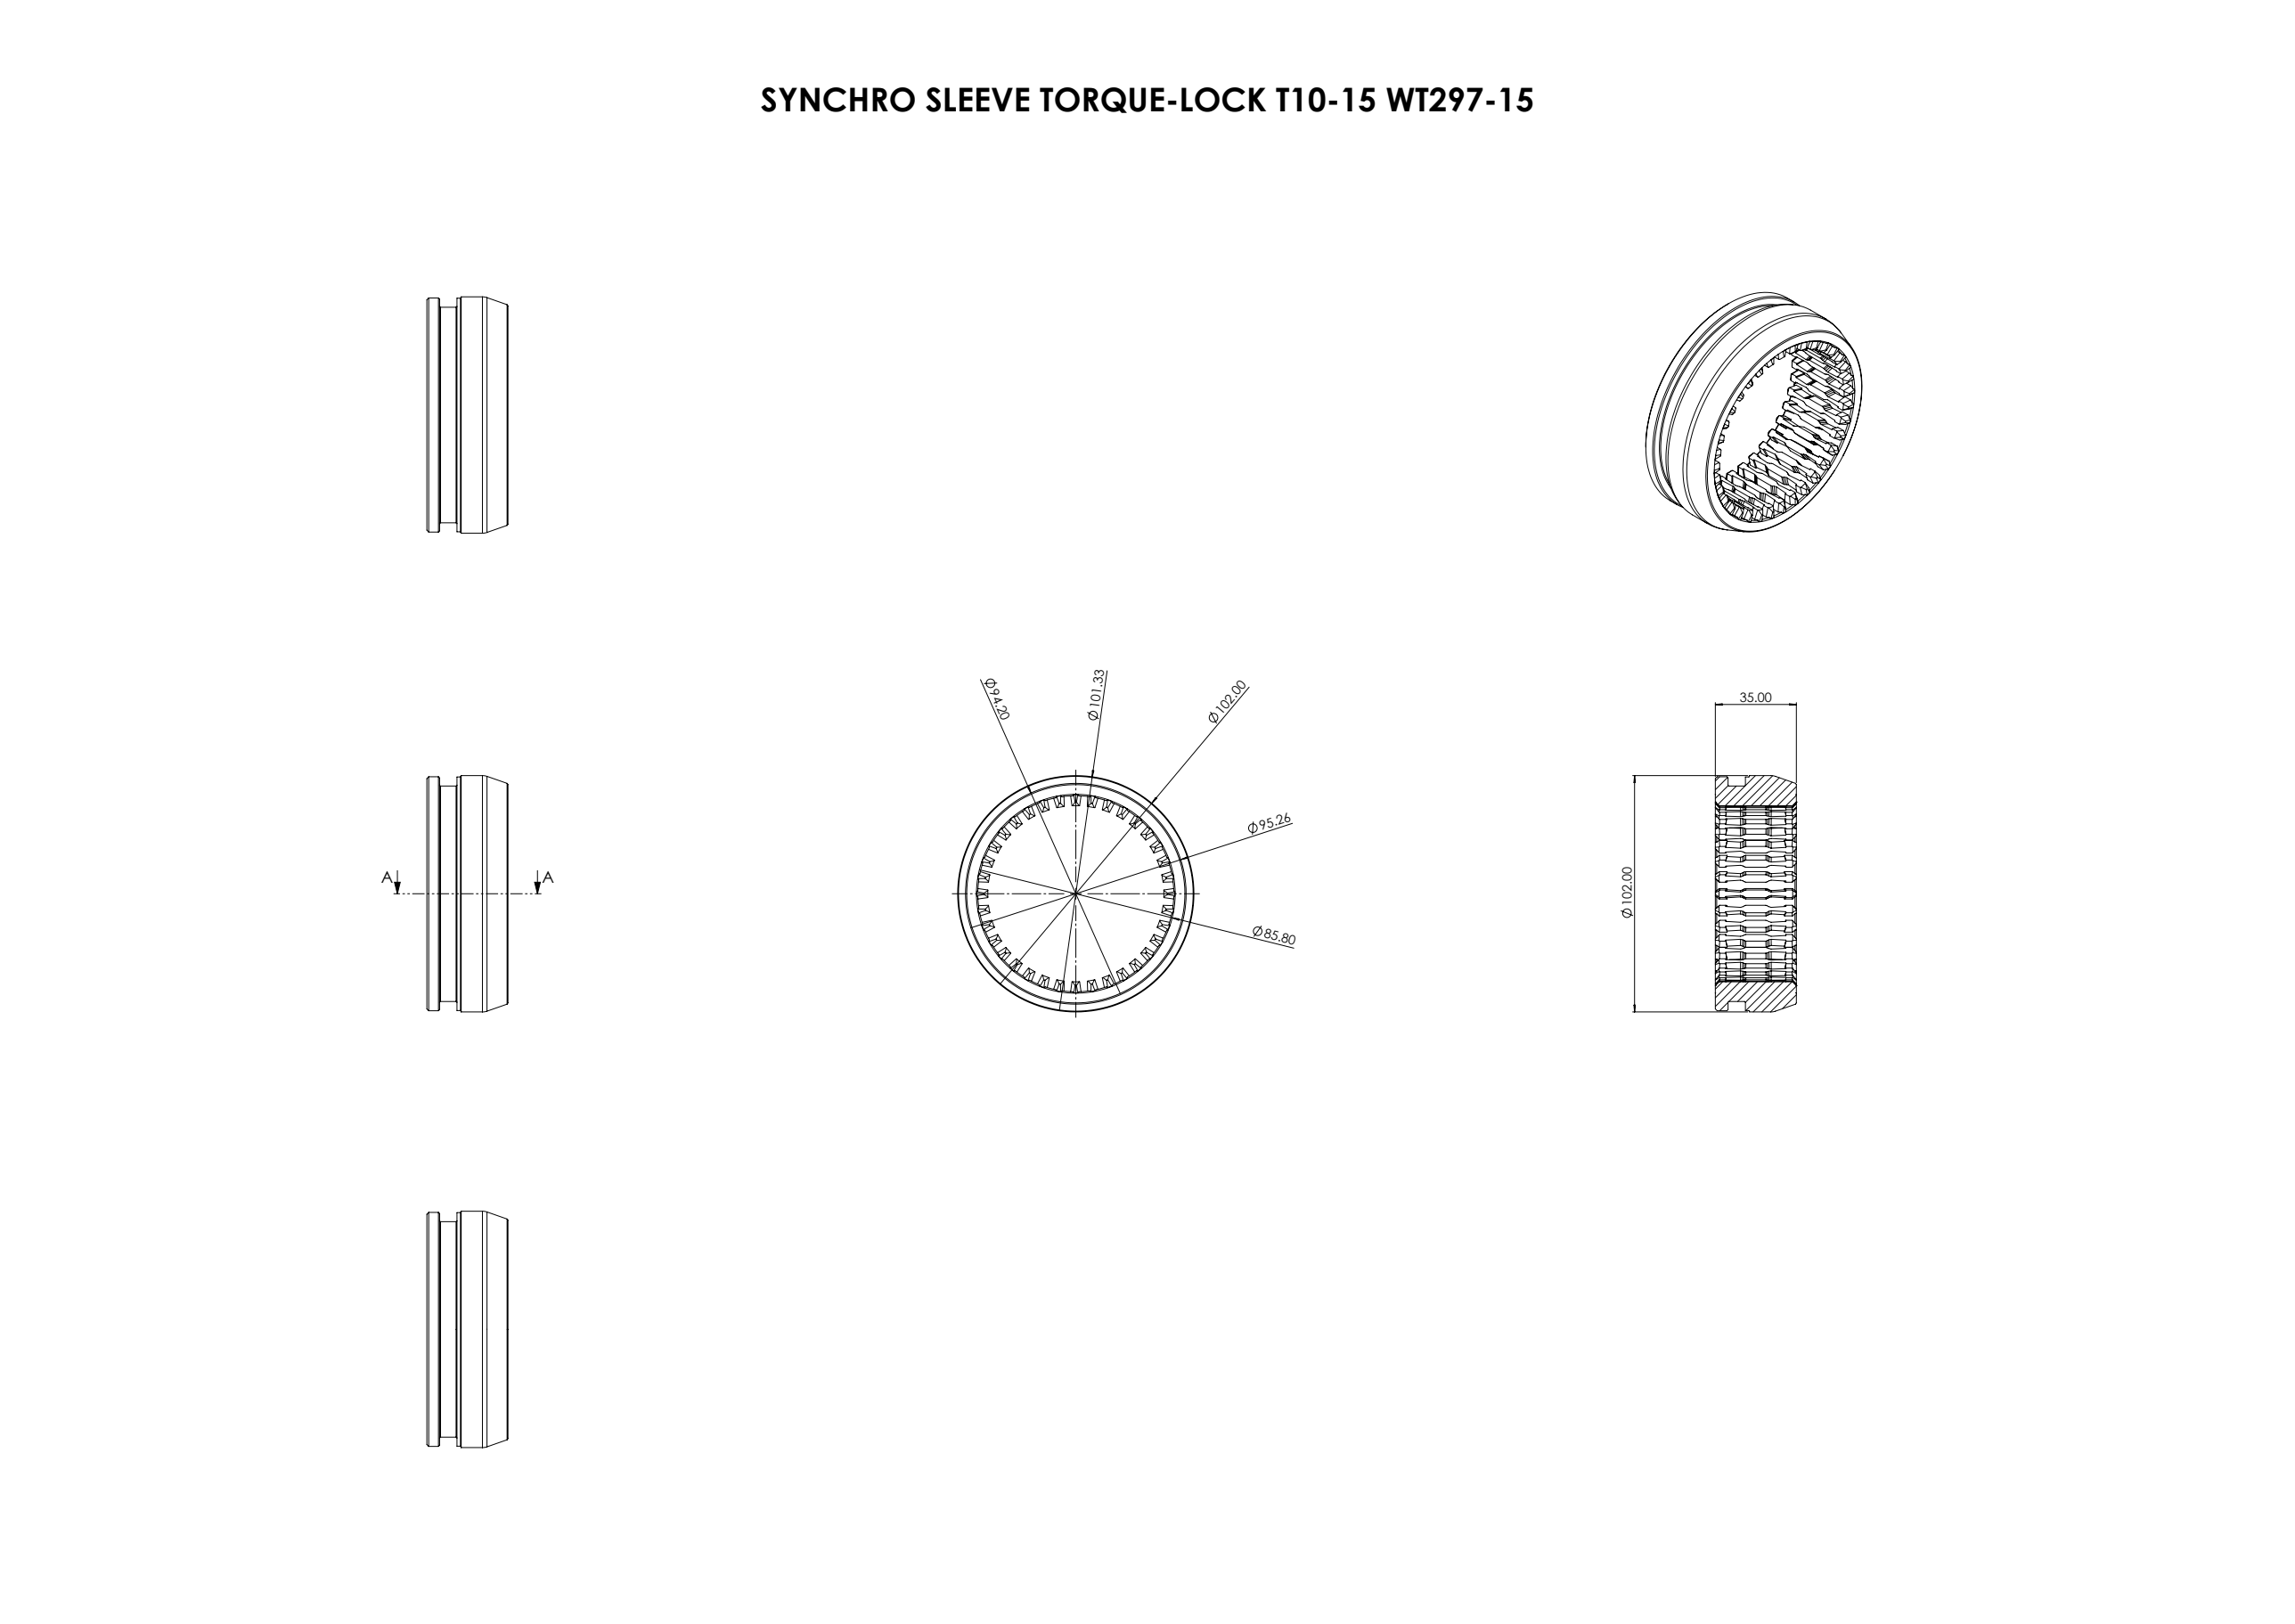
ISO-10303-21;
HEADER;
/* Generated by software containing ST-Developer
 * from STEP Tools, Inc. (www.steptools.com) 
 */

FILE_DESCRIPTION(
/* description */ (''),
/* implementation_level */ '2;1');

FILE_NAME(
/* name */ '01_Synchro_Sleeve_Torque-Lock_T10-15_WT297-15.step',
/* time_stamp */ '2026-10-11T08:27:52-07:00',
/* author */ (''),
/* organization */ (''),
/* preprocessor_version */ 'ST-DEVELOPER v20.2',
/* originating_system */ 'Autodesk Translation Framework v15.15.0.0',
/* authorisation */ '');

FILE_SCHEMA (('AUTOMOTIVE_DESIGN { 1 0 10303 214 3 1 1 }'));
ENDSEC;

DATA;
#10=MECHANICAL_DESIGN_GEOMETRIC_PRESENTATION_REPRESENTATION('',(#919),#94301);
#891=SHAPE_REPRESENTATION_RELATIONSHIP('SRR','None',#94371,#905);
#905=ADVANCED_BREP_SHAPE_REPRESENTATION('',(#933),#94287);
#919=STYLED_ITEM('',(#94567),#933);
#933=MANIFOLD_SOLID_BREP('Body1',#51018);
#947=TOROIDAL_SURFACE('',#53576,45.,6.);
#948=TOROIDAL_SURFACE('',#53582,46.9,0.4);
#949=TOROIDAL_SURFACE('',#53592,46.9,0.4);
#959=FACE_BOUND('',#17303,.T.);
#960=FACE_BOUND('',#17309,.T.);
#961=FACE_BOUND('',#17312,.T.);
#962=FACE_BOUND('',#17315,.T.);
#1044=CYLINDRICAL_SURFACE('',#51779,42.3);
#1045=CYLINDRICAL_SURFACE('',#51830,42.3);
#1046=CYLINDRICAL_SURFACE('',#51881,42.3);
#1047=CYLINDRICAL_SURFACE('',#51932,42.3);
#1048=CYLINDRICAL_SURFACE('',#51983,42.3);
#1049=CYLINDRICAL_SURFACE('',#52034,42.3);
#1050=CYLINDRICAL_SURFACE('',#52085,42.3);
#1051=CYLINDRICAL_SURFACE('',#52136,42.3);
#1052=CYLINDRICAL_SURFACE('',#52187,42.3);
#1053=CYLINDRICAL_SURFACE('',#52238,42.3);
#1054=CYLINDRICAL_SURFACE('',#52289,42.3);
#1055=CYLINDRICAL_SURFACE('',#52340,42.3);
#1056=CYLINDRICAL_SURFACE('',#52391,42.3);
#1057=CYLINDRICAL_SURFACE('',#52442,42.3);
#1058=CYLINDRICAL_SURFACE('',#52493,42.3);
#1059=CYLINDRICAL_SURFACE('',#52544,42.3);
#1060=CYLINDRICAL_SURFACE('',#52595,42.3);
#1061=CYLINDRICAL_SURFACE('',#52646,42.3);
#1062=CYLINDRICAL_SURFACE('',#52697,42.3);
#1063=CYLINDRICAL_SURFACE('',#52748,42.3);
#1064=CYLINDRICAL_SURFACE('',#52799,42.3);
#1065=CYLINDRICAL_SURFACE('',#52850,42.3);
#1066=CYLINDRICAL_SURFACE('',#52901,42.3);
#1067=CYLINDRICAL_SURFACE('',#52952,42.3);
#1068=CYLINDRICAL_SURFACE('',#53003,42.3);
#1069=CYLINDRICAL_SURFACE('',#53054,42.3);
#1070=CYLINDRICAL_SURFACE('',#53105,42.3);
#1071=CYLINDRICAL_SURFACE('',#53156,42.3);
#1072=CYLINDRICAL_SURFACE('',#53207,42.3);
#1073=CYLINDRICAL_SURFACE('',#53258,42.3);
#1074=CYLINDRICAL_SURFACE('',#53309,42.3);
#1075=CYLINDRICAL_SURFACE('',#53360,42.3);
#1076=CYLINDRICAL_SURFACE('',#53411,42.3);
#1077=CYLINDRICAL_SURFACE('',#53462,42.3);
#1078=CYLINDRICAL_SURFACE('',#53513,42.3);
#1079=CYLINDRICAL_SURFACE('',#53580,51.);
#1080=CYLINDRICAL_SURFACE('',#53587,46.5);
#1081=CYLINDRICAL_SURFACE('',#53597,42.3);
#1082=CYLINDRICAL_SURFACE('',#53602,50.5);
#1083=CYLINDRICAL_SURFACE('',#53605,50.4);
#1288=ELLIPSE('',#51263,65.1465238200804,42.3);
#1289=ELLIPSE('',#51266,65.1465238200804,42.3);
#1290=ELLIPSE('',#51269,65.1465238200804,42.3);
#1291=ELLIPSE('',#51272,65.1465238200804,42.3);
#1292=ELLIPSE('',#51275,65.1465238200804,42.3);
#1293=ELLIPSE('',#51278,65.1465238200804,42.3);
#1294=ELLIPSE('',#51281,65.1465238200804,42.3);
#1295=ELLIPSE('',#51284,65.1465238200804,42.3);
#1296=ELLIPSE('',#51287,65.1465238200804,42.3);
#1297=ELLIPSE('',#51290,65.1465238200804,42.3);
#1298=ELLIPSE('',#51293,65.1465238200804,42.3);
#1299=ELLIPSE('',#51296,65.1465238200804,42.3);
#1300=ELLIPSE('',#51299,65.1465238200804,42.3);
#1301=ELLIPSE('',#51302,65.1465238200804,42.3);
#1302=ELLIPSE('',#51305,65.1465238200804,42.3);
#1303=ELLIPSE('',#51308,65.1465238200804,42.3);
#1304=ELLIPSE('',#51311,65.1465238200804,42.3);
#1305=ELLIPSE('',#51314,65.1465238200804,42.3);
#1306=ELLIPSE('',#51317,65.1465238200804,42.3);
#1307=ELLIPSE('',#51320,65.1465238200804,42.3);
#1308=ELLIPSE('',#51323,65.1465238200804,42.3);
#1309=ELLIPSE('',#51326,65.1465238200804,42.3);
#1310=ELLIPSE('',#51329,65.1465238200804,42.3);
#1311=ELLIPSE('',#51332,65.1465238200804,42.3);
#1312=ELLIPSE('',#51335,65.1465238200804,42.3);
#1313=ELLIPSE('',#51338,65.1465238200804,42.3);
#1314=ELLIPSE('',#51341,65.1465238200804,42.3);
#1315=ELLIPSE('',#51344,65.1465238200804,42.3);
#1316=ELLIPSE('',#51347,65.1465238200804,42.3);
#1317=ELLIPSE('',#51350,65.1465238200804,42.3);
#1318=ELLIPSE('',#51353,65.1465238200804,42.3);
#1319=ELLIPSE('',#51356,65.1465238200804,42.3);
#1320=ELLIPSE('',#51359,65.1465238200804,42.3);
#1321=ELLIPSE('',#51362,65.1465238200804,42.3);
#1322=ELLIPSE('',#51365,65.1465238200804,42.3);
#1323=ELLIPSE('',#51368,65.1465238200804,42.3);
#1324=ELLIPSE('',#51442,65.1465238200804,42.3);
#1325=ELLIPSE('',#51444,65.1465238200804,42.3);
#1326=ELLIPSE('',#51446,65.1465238200804,42.3);
#1327=ELLIPSE('',#51448,65.1465238200804,42.3);
#1328=ELLIPSE('',#51450,65.1465238200804,42.3);
#1329=ELLIPSE('',#51452,65.1465238200804,42.3);
#1330=ELLIPSE('',#51454,65.1465238200804,42.3);
#1331=ELLIPSE('',#51456,65.1465238200804,42.3);
#1332=ELLIPSE('',#51458,65.1465238200804,42.3);
#1333=ELLIPSE('',#51460,65.1465238200804,42.3);
#1334=ELLIPSE('',#51462,65.1465238200804,42.3);
#1335=ELLIPSE('',#51464,65.1465238200804,42.3);
#1336=ELLIPSE('',#51466,65.1465238200804,42.3);
#1337=ELLIPSE('',#51468,65.1465238200804,42.3);
#1338=ELLIPSE('',#51470,65.1465238200804,42.3);
#1339=ELLIPSE('',#51472,65.1465238200804,42.3);
#1340=ELLIPSE('',#51474,65.1465238200804,42.3);
#1341=ELLIPSE('',#51476,65.1465238200804,42.3);
#1342=ELLIPSE('',#51478,65.1465238200804,42.3);
#1343=ELLIPSE('',#51480,65.1465238200804,42.3);
#1344=ELLIPSE('',#51482,65.1465238200804,42.3);
#1345=ELLIPSE('',#51484,65.1465238200804,42.3);
#1346=ELLIPSE('',#51486,65.1465238200804,42.3);
#1347=ELLIPSE('',#51488,65.1465238200804,42.3);
#1348=ELLIPSE('',#51490,65.1465238200804,42.3);
#1349=ELLIPSE('',#51492,65.1465238200804,42.3);
#1350=ELLIPSE('',#51494,65.1465238200804,42.3);
#1351=ELLIPSE('',#51496,65.1465238200804,42.3);
#1352=ELLIPSE('',#51498,65.1465238200804,42.3);
#1353=ELLIPSE('',#51500,65.1465238200804,42.3);
#1354=ELLIPSE('',#51502,65.1465238200804,42.3);
#1355=ELLIPSE('',#51504,65.1465238200804,42.3);
#1356=ELLIPSE('',#51506,65.1465238200804,42.3);
#1357=ELLIPSE('',#51508,65.1465238200804,42.3);
#1358=ELLIPSE('',#51510,65.1465238200804,42.3);
#1359=ELLIPSE('',#51512,65.1465238200804,42.3);
#1360=ELLIPSE('',#51550,65.1465238200804,42.3);
#1361=ELLIPSE('',#51552,65.1465238200804,42.3);
#1362=ELLIPSE('',#51554,65.1465238200804,42.3);
#1363=ELLIPSE('',#51556,65.1465238200804,42.3);
#1364=ELLIPSE('',#51558,65.1465238200804,42.3);
#1365=ELLIPSE('',#51560,65.1465238200804,42.3);
#1366=ELLIPSE('',#51562,65.1465238200804,42.3);
#1367=ELLIPSE('',#51564,65.1465238200804,42.3);
#1368=ELLIPSE('',#51566,65.1465238200804,42.3);
#1369=ELLIPSE('',#51568,65.1465238200804,42.3);
#1370=ELLIPSE('',#51570,65.1465238200804,42.3);
#1371=ELLIPSE('',#51572,65.1465238200804,42.3);
#1372=ELLIPSE('',#51574,65.1465238200804,42.3);
#1373=ELLIPSE('',#51576,65.1465238200804,42.3);
#1374=ELLIPSE('',#51578,65.1465238200804,42.3);
#1375=ELLIPSE('',#51580,65.1465238200804,42.3);
#1376=ELLIPSE('',#51582,65.1465238200804,42.3);
#1377=ELLIPSE('',#51584,65.1465238200804,42.3);
#1378=ELLIPSE('',#51586,65.1465238200804,42.3);
#1379=ELLIPSE('',#51588,65.1465238200804,42.3);
#1380=ELLIPSE('',#51590,65.1465238200804,42.3);
#1381=ELLIPSE('',#51592,65.1465238200804,42.3);
#1382=ELLIPSE('',#51594,65.1465238200804,42.3);
#1383=ELLIPSE('',#51596,65.1465238200804,42.3);
#1384=ELLIPSE('',#51598,65.1465238200804,42.3);
#1385=ELLIPSE('',#51600,65.1465238200804,42.3);
#1386=ELLIPSE('',#51602,65.1465238200804,42.3);
#1387=ELLIPSE('',#51604,65.1465238200804,42.3);
#1388=ELLIPSE('',#51606,65.1465238200804,42.3);
#1389=ELLIPSE('',#51608,65.1465238200804,42.3);
#1390=ELLIPSE('',#51610,65.1465238200804,42.3);
#1391=ELLIPSE('',#51612,65.1465238200804,42.3);
#1392=ELLIPSE('',#51614,65.1465238200804,42.3);
#1393=ELLIPSE('',#51616,65.1465238200804,42.3);
#1394=ELLIPSE('',#51618,65.1465238200804,42.3);
#1395=ELLIPSE('',#51694,42.7157063175375,42.3);
#1396=ELLIPSE('',#51696,684.784865862974,42.3);
#1397=ELLIPSE('',#51698,148.655022233233,42.3);
#1398=ELLIPSE('',#51700,86.0962585581534,42.3);
#1399=ELLIPSE('',#51702,135.078923826262,42.3);
#1400=ELLIPSE('',#51705,135.078923826262,42.3);
#1401=ELLIPSE('',#51707,86.0962585581532,42.3);
#1402=ELLIPSE('',#51709,148.655022233233,42.3);
#1403=ELLIPSE('',#51711,684.784865862975,42.3);
#1404=ELLIPSE('',#51713,42.7157063175375,42.3);
#1405=ELLIPSE('',#51716,65.1465238200804,42.3);
#1406=ELLIPSE('',#51719,42.7157063175375,42.3);
#1407=ELLIPSE('',#51721,684.784865862975,42.3);
#1408=ELLIPSE('',#51723,148.655022233233,42.3);
#1409=ELLIPSE('',#51725,86.0962585581532,42.3);
#1410=ELLIPSE('',#51727,135.078923826262,42.3);
#1411=ELLIPSE('',#51730,135.078923826262,42.3);
#1412=ELLIPSE('',#51732,86.0962585581534,42.3);
#1413=ELLIPSE('',#51734,148.655022233233,42.3);
#1414=ELLIPSE('',#51736,684.784865862974,42.3);
#1415=ELLIPSE('',#51738,42.7157063175375,42.3);
#1416=ELLIPSE('',#51781,65.1465238200804,42.3);
#1417=ELLIPSE('',#51782,42.7157063175375,42.3);
#1418=ELLIPSE('',#51783,684.784865862975,42.3);
#1419=ELLIPSE('',#51784,148.655022233233,42.3);
#1420=ELLIPSE('',#51785,86.0962585581532,42.3);
#1421=ELLIPSE('',#51786,135.078923826262,42.3);
#1422=ELLIPSE('',#51787,135.078923826262,42.3);
#1423=ELLIPSE('',#51788,86.0962585581534,42.3);
#1424=ELLIPSE('',#51789,148.655022233233,42.3);
#1425=ELLIPSE('',#51790,684.784865862974,42.3);
#1426=ELLIPSE('',#51791,42.7157063175375,42.3);
#1427=ELLIPSE('',#51808,42.7157063175375,42.3);
#1428=ELLIPSE('',#51810,684.784865862975,42.3);
#1429=ELLIPSE('',#51812,148.655022233233,42.3);
#1430=ELLIPSE('',#51814,86.0962585581532,42.3);
#1431=ELLIPSE('',#51816,135.078923826262,42.3);
#1432=ELLIPSE('',#51819,135.078923826262,42.3);
#1433=ELLIPSE('',#51821,86.0962585581534,42.3);
#1434=ELLIPSE('',#51823,148.655022233233,42.3);
#1435=ELLIPSE('',#51825,684.784865862974,42.3);
#1436=ELLIPSE('',#51827,42.7157063175375,42.3);
#1437=ELLIPSE('',#51832,65.1465238200804,42.3);
#1438=ELLIPSE('',#51833,42.7157063175375,42.3);
#1439=ELLIPSE('',#51834,684.784865862975,42.3);
#1440=ELLIPSE('',#51835,148.655022233233,42.3);
#1441=ELLIPSE('',#51836,86.0962585581532,42.3);
#1442=ELLIPSE('',#51837,135.078923826262,42.3);
#1443=ELLIPSE('',#51838,135.078923826262,42.3);
#1444=ELLIPSE('',#51839,86.0962585581534,42.3);
#1445=ELLIPSE('',#51840,148.655022233233,42.3);
#1446=ELLIPSE('',#51841,684.784865862974,42.3);
#1447=ELLIPSE('',#51842,42.7157063175375,42.3);
#1448=ELLIPSE('',#51859,42.7157063175375,42.3);
#1449=ELLIPSE('',#51861,684.784865862975,42.3);
#1450=ELLIPSE('',#51863,148.655022233233,42.3);
#1451=ELLIPSE('',#51865,86.0962585581532,42.3);
#1452=ELLIPSE('',#51867,135.078923826262,42.3);
#1453=ELLIPSE('',#51870,135.078923826262,42.3);
#1454=ELLIPSE('',#51872,86.0962585581534,42.3);
#1455=ELLIPSE('',#51874,148.655022233233,42.3);
#1456=ELLIPSE('',#51876,684.784865862974,42.3);
#1457=ELLIPSE('',#51878,42.7157063175375,42.3);
#1458=ELLIPSE('',#51883,65.1465238200804,42.3);
#1459=ELLIPSE('',#51884,42.7157063175375,42.3);
#1460=ELLIPSE('',#51885,684.784865862975,42.3);
#1461=ELLIPSE('',#51886,148.655022233233,42.3);
#1462=ELLIPSE('',#51887,86.0962585581532,42.3);
#1463=ELLIPSE('',#51888,135.078923826262,42.3);
#1464=ELLIPSE('',#51889,135.078923826262,42.3);
#1465=ELLIPSE('',#51890,86.0962585581534,42.3);
#1466=ELLIPSE('',#51891,148.655022233233,42.3);
#1467=ELLIPSE('',#51892,684.784865862974,42.3);
#1468=ELLIPSE('',#51893,42.7157063175375,42.3);
#1469=ELLIPSE('',#51910,42.7157063175375,42.3);
#1470=ELLIPSE('',#51912,684.784865862975,42.3);
#1471=ELLIPSE('',#51914,148.655022233233,42.3);
#1472=ELLIPSE('',#51916,86.0962585581532,42.3);
#1473=ELLIPSE('',#51918,135.078923826262,42.3);
#1474=ELLIPSE('',#51921,135.078923826262,42.3);
#1475=ELLIPSE('',#51923,86.0962585581534,42.3);
#1476=ELLIPSE('',#51925,148.655022233233,42.3);
#1477=ELLIPSE('',#51927,684.784865862974,42.3);
#1478=ELLIPSE('',#51929,42.7157063175375,42.3);
#1479=ELLIPSE('',#51934,65.1465238200804,42.3);
#1480=ELLIPSE('',#51935,42.7157063175375,42.3);
#1481=ELLIPSE('',#51936,684.784865862975,42.3);
#1482=ELLIPSE('',#51937,148.655022233233,42.3);
#1483=ELLIPSE('',#51938,86.0962585581532,42.3);
#1484=ELLIPSE('',#51939,135.078923826262,42.3);
#1485=ELLIPSE('',#51940,135.078923826262,42.3);
#1486=ELLIPSE('',#51941,86.0962585581534,42.3);
#1487=ELLIPSE('',#51942,148.655022233233,42.3);
#1488=ELLIPSE('',#51943,684.784865862974,42.3);
#1489=ELLIPSE('',#51944,42.7157063175375,42.3);
#1490=ELLIPSE('',#51961,42.7157063175375,42.3);
#1491=ELLIPSE('',#51963,684.784865862975,42.3);
#1492=ELLIPSE('',#51965,148.655022233233,42.3);
#1493=ELLIPSE('',#51967,86.0962585581532,42.3);
#1494=ELLIPSE('',#51969,135.078923826262,42.3);
#1495=ELLIPSE('',#51972,135.078923826262,42.3);
#1496=ELLIPSE('',#51974,86.0962585581534,42.3);
#1497=ELLIPSE('',#51976,148.655022233233,42.3);
#1498=ELLIPSE('',#51978,684.784865862974,42.3);
#1499=ELLIPSE('',#51980,42.7157063175375,42.3);
#1500=ELLIPSE('',#51985,65.1465238200804,42.3);
#1501=ELLIPSE('',#51986,42.7157063175375,42.3);
#1502=ELLIPSE('',#51987,684.784865862975,42.3);
#1503=ELLIPSE('',#51988,148.655022233233,42.3);
#1504=ELLIPSE('',#51989,86.0962585581532,42.3);
#1505=ELLIPSE('',#51990,135.078923826262,42.3);
#1506=ELLIPSE('',#51991,135.078923826262,42.3);
#1507=ELLIPSE('',#51992,86.0962585581534,42.3);
#1508=ELLIPSE('',#51993,148.655022233233,42.3);
#1509=ELLIPSE('',#51994,684.784865862974,42.3);
#1510=ELLIPSE('',#51995,42.7157063175375,42.3);
#1511=ELLIPSE('',#52012,42.7157063175375,42.3);
#1512=ELLIPSE('',#52014,684.784865862975,42.3);
#1513=ELLIPSE('',#52016,148.655022233233,42.3);
#1514=ELLIPSE('',#52018,86.0962585581532,42.3);
#1515=ELLIPSE('',#52020,135.078923826262,42.3);
#1516=ELLIPSE('',#52023,135.078923826262,42.3);
#1517=ELLIPSE('',#52025,86.0962585581534,42.3);
#1518=ELLIPSE('',#52027,148.655022233233,42.3);
#1519=ELLIPSE('',#52029,684.784865862974,42.3);
#1520=ELLIPSE('',#52031,42.7157063175375,42.3);
#1521=ELLIPSE('',#52036,65.1465238200804,42.3);
#1522=ELLIPSE('',#52037,42.7157063175375,42.3);
#1523=ELLIPSE('',#52038,684.784865862975,42.3);
#1524=ELLIPSE('',#52039,148.655022233233,42.3);
#1525=ELLIPSE('',#52040,86.0962585581532,42.3);
#1526=ELLIPSE('',#52041,135.078923826262,42.3);
#1527=ELLIPSE('',#52042,135.078923826262,42.3);
#1528=ELLIPSE('',#52043,86.0962585581534,42.3);
#1529=ELLIPSE('',#52044,148.655022233233,42.3);
#1530=ELLIPSE('',#52045,684.784865862974,42.3);
#1531=ELLIPSE('',#52046,42.7157063175375,42.3);
#1532=ELLIPSE('',#52063,42.7157063175375,42.3);
#1533=ELLIPSE('',#52065,684.784865862975,42.3);
#1534=ELLIPSE('',#52067,148.655022233233,42.3);
#1535=ELLIPSE('',#52069,86.0962585581532,42.3);
#1536=ELLIPSE('',#52071,135.078923826262,42.3);
#1537=ELLIPSE('',#52074,135.078923826262,42.3);
#1538=ELLIPSE('',#52076,86.0962585581534,42.3);
#1539=ELLIPSE('',#52078,148.655022233233,42.3);
#1540=ELLIPSE('',#52080,684.784865862974,42.3);
#1541=ELLIPSE('',#52082,42.7157063175375,42.3);
#1542=ELLIPSE('',#52087,65.1465238200804,42.3);
#1543=ELLIPSE('',#52088,42.7157063175375,42.3);
#1544=ELLIPSE('',#52089,684.784865862975,42.3);
#1545=ELLIPSE('',#52090,148.655022233233,42.3);
#1546=ELLIPSE('',#52091,86.0962585581532,42.3);
#1547=ELLIPSE('',#52092,135.078923826262,42.3);
#1548=ELLIPSE('',#52093,135.078923826262,42.3);
#1549=ELLIPSE('',#52094,86.0962585581534,42.3);
#1550=ELLIPSE('',#52095,148.655022233233,42.3);
#1551=ELLIPSE('',#52096,684.784865862974,42.3);
#1552=ELLIPSE('',#52097,42.7157063175375,42.3);
#1553=ELLIPSE('',#52114,42.7157063175375,42.3);
#1554=ELLIPSE('',#52116,684.784865862975,42.3);
#1555=ELLIPSE('',#52118,148.655022233233,42.3);
#1556=ELLIPSE('',#52120,86.0962585581532,42.3);
#1557=ELLIPSE('',#52122,135.078923826262,42.3);
#1558=ELLIPSE('',#52125,135.078923826262,42.3);
#1559=ELLIPSE('',#52127,86.0962585581534,42.3);
#1560=ELLIPSE('',#52129,148.655022233233,42.3);
#1561=ELLIPSE('',#52131,684.784865862974,42.3);
#1562=ELLIPSE('',#52133,42.7157063175375,42.3);
#1563=ELLIPSE('',#52138,65.1465238200804,42.3);
#1564=ELLIPSE('',#52139,42.7157063175375,42.3);
#1565=ELLIPSE('',#52140,684.784865862975,42.3);
#1566=ELLIPSE('',#52141,148.655022233233,42.3);
#1567=ELLIPSE('',#52142,86.0962585581532,42.3);
#1568=ELLIPSE('',#52143,135.078923826262,42.3);
#1569=ELLIPSE('',#52144,135.078923826262,42.3);
#1570=ELLIPSE('',#52145,86.0962585581534,42.3);
#1571=ELLIPSE('',#52146,148.655022233233,42.3);
#1572=ELLIPSE('',#52147,684.784865862974,42.3);
#1573=ELLIPSE('',#52148,42.7157063175375,42.3);
#1574=ELLIPSE('',#52165,42.7157063175375,42.3);
#1575=ELLIPSE('',#52167,684.784865862975,42.3);
#1576=ELLIPSE('',#52169,148.655022233233,42.3);
#1577=ELLIPSE('',#52171,86.0962585581532,42.3);
#1578=ELLIPSE('',#52173,135.078923826262,42.3);
#1579=ELLIPSE('',#52176,135.078923826262,42.3);
#1580=ELLIPSE('',#52178,86.0962585581534,42.3);
#1581=ELLIPSE('',#52180,148.655022233233,42.3);
#1582=ELLIPSE('',#52182,684.784865862974,42.3);
#1583=ELLIPSE('',#52184,42.7157063175375,42.3);
#1584=ELLIPSE('',#52189,65.1465238200804,42.3);
#1585=ELLIPSE('',#52190,42.7157063175375,42.3);
#1586=ELLIPSE('',#52191,684.784865862975,42.3);
#1587=ELLIPSE('',#52192,148.655022233233,42.3);
#1588=ELLIPSE('',#52193,86.0962585581532,42.3);
#1589=ELLIPSE('',#52194,135.078923826262,42.3);
#1590=ELLIPSE('',#52195,135.078923826262,42.3);
#1591=ELLIPSE('',#52196,86.0962585581534,42.3);
#1592=ELLIPSE('',#52197,148.655022233233,42.3);
#1593=ELLIPSE('',#52198,684.784865862974,42.3);
#1594=ELLIPSE('',#52199,42.7157063175375,42.3);
#1595=ELLIPSE('',#52216,42.7157063175375,42.3);
#1596=ELLIPSE('',#52218,684.784865862975,42.3);
#1597=ELLIPSE('',#52220,148.655022233233,42.3);
#1598=ELLIPSE('',#52222,86.0962585581532,42.3);
#1599=ELLIPSE('',#52224,135.078923826262,42.3);
#1600=ELLIPSE('',#52227,135.078923826262,42.3);
#1601=ELLIPSE('',#52229,86.0962585581534,42.3);
#1602=ELLIPSE('',#52231,148.655022233233,42.3);
#1603=ELLIPSE('',#52233,684.784865862974,42.3);
#1604=ELLIPSE('',#52235,42.7157063175375,42.3);
#1605=ELLIPSE('',#52240,65.1465238200804,42.3);
#1606=ELLIPSE('',#52241,42.7157063175375,42.3);
#1607=ELLIPSE('',#52242,684.784865862975,42.3);
#1608=ELLIPSE('',#52243,148.655022233233,42.3);
#1609=ELLIPSE('',#52244,86.0962585581532,42.3);
#1610=ELLIPSE('',#52245,135.078923826262,42.3);
#1611=ELLIPSE('',#52246,135.078923826262,42.3);
#1612=ELLIPSE('',#52247,86.0962585581534,42.3);
#1613=ELLIPSE('',#52248,148.655022233233,42.3);
#1614=ELLIPSE('',#52249,684.784865862974,42.3);
#1615=ELLIPSE('',#52250,42.7157063175375,42.3);
#1616=ELLIPSE('',#52267,42.7157063175375,42.3);
#1617=ELLIPSE('',#52269,684.784865862975,42.3);
#1618=ELLIPSE('',#52271,148.655022233233,42.3);
#1619=ELLIPSE('',#52273,86.0962585581532,42.3);
#1620=ELLIPSE('',#52275,135.078923826262,42.3);
#1621=ELLIPSE('',#52278,135.078923826262,42.3);
#1622=ELLIPSE('',#52280,86.0962585581534,42.3);
#1623=ELLIPSE('',#52282,148.655022233233,42.3);
#1624=ELLIPSE('',#52284,684.784865862974,42.3);
#1625=ELLIPSE('',#52286,42.7157063175375,42.3);
#1626=ELLIPSE('',#52291,65.1465238200804,42.3);
#1627=ELLIPSE('',#52292,42.7157063175375,42.3);
#1628=ELLIPSE('',#52293,684.784865862975,42.3);
#1629=ELLIPSE('',#52294,148.655022233233,42.3);
#1630=ELLIPSE('',#52295,86.0962585581532,42.3);
#1631=ELLIPSE('',#52296,135.078923826262,42.3);
#1632=ELLIPSE('',#52297,135.078923826262,42.3);
#1633=ELLIPSE('',#52298,86.0962585581534,42.3);
#1634=ELLIPSE('',#52299,148.655022233233,42.3);
#1635=ELLIPSE('',#52300,684.784865862974,42.3);
#1636=ELLIPSE('',#52301,42.7157063175375,42.3);
#1637=ELLIPSE('',#52318,42.7157063175375,42.3);
#1638=ELLIPSE('',#52320,684.784865862975,42.3);
#1639=ELLIPSE('',#52322,148.655022233233,42.3);
#1640=ELLIPSE('',#52324,86.0962585581532,42.3);
#1641=ELLIPSE('',#52326,135.078923826262,42.3);
#1642=ELLIPSE('',#52329,135.078923826262,42.3);
#1643=ELLIPSE('',#52331,86.0962585581534,42.3);
#1644=ELLIPSE('',#52333,148.655022233233,42.3);
#1645=ELLIPSE('',#52335,684.784865862974,42.3);
#1646=ELLIPSE('',#52337,42.7157063175375,42.3);
#1647=ELLIPSE('',#52342,65.1465238200804,42.3);
#1648=ELLIPSE('',#52343,42.7157063175375,42.3);
#1649=ELLIPSE('',#52344,684.784865862975,42.3);
#1650=ELLIPSE('',#52345,148.655022233233,42.3);
#1651=ELLIPSE('',#52346,86.0962585581532,42.3);
#1652=ELLIPSE('',#52347,135.078923826262,42.3);
#1653=ELLIPSE('',#52348,135.078923826262,42.3);
#1654=ELLIPSE('',#52349,86.0962585581534,42.3);
#1655=ELLIPSE('',#52350,148.655022233233,42.3);
#1656=ELLIPSE('',#52351,684.784865862974,42.3);
#1657=ELLIPSE('',#52352,42.7157063175375,42.3);
#1658=ELLIPSE('',#52369,42.7157063175375,42.3);
#1659=ELLIPSE('',#52371,684.784865862975,42.3);
#1660=ELLIPSE('',#52373,148.655022233233,42.3);
#1661=ELLIPSE('',#52375,86.0962585581532,42.3);
#1662=ELLIPSE('',#52377,135.078923826262,42.3);
#1663=ELLIPSE('',#52380,135.078923826262,42.3);
#1664=ELLIPSE('',#52382,86.0962585581534,42.3);
#1665=ELLIPSE('',#52384,148.655022233233,42.3);
#1666=ELLIPSE('',#52386,684.784865862974,42.3);
#1667=ELLIPSE('',#52388,42.7157063175375,42.3);
#1668=ELLIPSE('',#52393,65.1465238200804,42.3);
#1669=ELLIPSE('',#52394,42.7157063175375,42.3);
#1670=ELLIPSE('',#52395,684.784865862975,42.3);
#1671=ELLIPSE('',#52396,148.655022233233,42.3);
#1672=ELLIPSE('',#52397,86.0962585581532,42.3);
#1673=ELLIPSE('',#52398,135.078923826262,42.3);
#1674=ELLIPSE('',#52399,135.078923826262,42.3);
#1675=ELLIPSE('',#52400,86.0962585581534,42.3);
#1676=ELLIPSE('',#52401,148.655022233233,42.3);
#1677=ELLIPSE('',#52402,684.784865862974,42.3);
#1678=ELLIPSE('',#52403,42.7157063175375,42.3);
#1679=ELLIPSE('',#52420,42.7157063175375,42.3);
#1680=ELLIPSE('',#52422,684.784865862975,42.3);
#1681=ELLIPSE('',#52424,148.655022233233,42.3);
#1682=ELLIPSE('',#52426,86.0962585581532,42.3);
#1683=ELLIPSE('',#52428,135.078923826262,42.3);
#1684=ELLIPSE('',#52431,135.078923826262,42.3);
#1685=ELLIPSE('',#52433,86.0962585581534,42.3);
#1686=ELLIPSE('',#52435,148.655022233233,42.3);
#1687=ELLIPSE('',#52437,684.784865862974,42.3);
#1688=ELLIPSE('',#52439,42.7157063175375,42.3);
#1689=ELLIPSE('',#52444,65.1465238200804,42.3);
#1690=ELLIPSE('',#52445,42.7157063175375,42.3);
#1691=ELLIPSE('',#52446,684.784865862975,42.3);
#1692=ELLIPSE('',#52447,148.655022233233,42.3);
#1693=ELLIPSE('',#52448,86.0962585581532,42.3);
#1694=ELLIPSE('',#52449,135.078923826262,42.3);
#1695=ELLIPSE('',#52450,135.078923826262,42.3);
#1696=ELLIPSE('',#52451,86.0962585581534,42.3);
#1697=ELLIPSE('',#52452,148.655022233233,42.3);
#1698=ELLIPSE('',#52453,684.784865862974,42.3);
#1699=ELLIPSE('',#52454,42.7157063175375,42.3);
#1700=ELLIPSE('',#52471,42.7157063175375,42.3);
#1701=ELLIPSE('',#52473,684.784865862975,42.3);
#1702=ELLIPSE('',#52475,148.655022233233,42.3);
#1703=ELLIPSE('',#52477,86.0962585581532,42.3);
#1704=ELLIPSE('',#52479,135.078923826262,42.3);
#1705=ELLIPSE('',#52482,135.078923826262,42.3);
#1706=ELLIPSE('',#52484,86.0962585581534,42.3);
#1707=ELLIPSE('',#52486,148.655022233233,42.3);
#1708=ELLIPSE('',#52488,684.784865862974,42.3);
#1709=ELLIPSE('',#52490,42.7157063175375,42.3);
#1710=ELLIPSE('',#52495,65.1465238200804,42.3);
#1711=ELLIPSE('',#52496,42.7157063175375,42.3);
#1712=ELLIPSE('',#52497,684.784865862975,42.3);
#1713=ELLIPSE('',#52498,148.655022233233,42.3);
#1714=ELLIPSE('',#52499,86.0962585581532,42.3);
#1715=ELLIPSE('',#52500,135.078923826262,42.3);
#1716=ELLIPSE('',#52501,135.078923826262,42.3);
#1717=ELLIPSE('',#52502,86.0962585581534,42.3);
#1718=ELLIPSE('',#52503,148.655022233233,42.3);
#1719=ELLIPSE('',#52504,684.784865862974,42.3);
#1720=ELLIPSE('',#52505,42.7157063175375,42.3);
#1721=ELLIPSE('',#52522,42.7157063175375,42.3);
#1722=ELLIPSE('',#52524,684.784865862975,42.3);
#1723=ELLIPSE('',#52526,148.655022233233,42.3);
#1724=ELLIPSE('',#52528,86.0962585581532,42.3);
#1725=ELLIPSE('',#52530,135.078923826262,42.3);
#1726=ELLIPSE('',#52533,135.078923826262,42.3);
#1727=ELLIPSE('',#52535,86.0962585581534,42.3);
#1728=ELLIPSE('',#52537,148.655022233233,42.3);
#1729=ELLIPSE('',#52539,684.784865862974,42.3);
#1730=ELLIPSE('',#52541,42.7157063175375,42.3);
#1731=ELLIPSE('',#52546,65.1465238200804,42.3);
#1732=ELLIPSE('',#52547,42.7157063175375,42.3);
#1733=ELLIPSE('',#52548,684.784865862975,42.3);
#1734=ELLIPSE('',#52549,148.655022233233,42.3);
#1735=ELLIPSE('',#52550,86.0962585581532,42.3);
#1736=ELLIPSE('',#52551,135.078923826262,42.3);
#1737=ELLIPSE('',#52552,135.078923826262,42.3);
#1738=ELLIPSE('',#52553,86.0962585581534,42.3);
#1739=ELLIPSE('',#52554,148.655022233233,42.3);
#1740=ELLIPSE('',#52555,684.784865862974,42.3);
#1741=ELLIPSE('',#52556,42.7157063175375,42.3);
#1742=ELLIPSE('',#52573,42.7157063175375,42.3);
#1743=ELLIPSE('',#52575,684.784865862975,42.3);
#1744=ELLIPSE('',#52577,148.655022233233,42.3);
#1745=ELLIPSE('',#52579,86.0962585581532,42.3);
#1746=ELLIPSE('',#52581,135.078923826262,42.3);
#1747=ELLIPSE('',#52584,135.078923826262,42.3);
#1748=ELLIPSE('',#52586,86.0962585581534,42.3);
#1749=ELLIPSE('',#52588,148.655022233233,42.3);
#1750=ELLIPSE('',#52590,684.784865862974,42.3);
#1751=ELLIPSE('',#52592,42.7157063175375,42.3);
#1752=ELLIPSE('',#52597,65.1465238200804,42.3);
#1753=ELLIPSE('',#52598,42.7157063175375,42.3);
#1754=ELLIPSE('',#52599,684.784865862975,42.3);
#1755=ELLIPSE('',#52600,148.655022233233,42.3);
#1756=ELLIPSE('',#52601,86.0962585581532,42.3);
#1757=ELLIPSE('',#52602,135.078923826262,42.3);
#1758=ELLIPSE('',#52603,135.078923826262,42.3);
#1759=ELLIPSE('',#52604,86.0962585581534,42.3);
#1760=ELLIPSE('',#52605,148.655022233233,42.3);
#1761=ELLIPSE('',#52606,684.784865862974,42.3);
#1762=ELLIPSE('',#52607,42.7157063175375,42.3);
#1763=ELLIPSE('',#52624,42.7157063175375,42.3);
#1764=ELLIPSE('',#52626,684.784865862975,42.3);
#1765=ELLIPSE('',#52628,148.655022233233,42.3);
#1766=ELLIPSE('',#52630,86.0962585581532,42.3);
#1767=ELLIPSE('',#52632,135.078923826262,42.3);
#1768=ELLIPSE('',#52635,135.078923826262,42.3);
#1769=ELLIPSE('',#52637,86.0962585581534,42.3);
#1770=ELLIPSE('',#52639,148.655022233233,42.3);
#1771=ELLIPSE('',#52641,684.784865862974,42.3);
#1772=ELLIPSE('',#52643,42.7157063175375,42.3);
#1773=ELLIPSE('',#52648,65.1465238200804,42.3);
#1774=ELLIPSE('',#52649,42.7157063175375,42.3);
#1775=ELLIPSE('',#52650,684.784865862975,42.3);
#1776=ELLIPSE('',#52651,148.655022233233,42.3);
#1777=ELLIPSE('',#52652,86.0962585581532,42.3);
#1778=ELLIPSE('',#52653,135.078923826262,42.3);
#1779=ELLIPSE('',#52654,135.078923826262,42.3);
#1780=ELLIPSE('',#52655,86.0962585581534,42.3);
#1781=ELLIPSE('',#52656,148.655022233233,42.3);
#1782=ELLIPSE('',#52657,684.784865862974,42.3);
#1783=ELLIPSE('',#52658,42.7157063175375,42.3);
#1784=ELLIPSE('',#52675,42.7157063175375,42.3);
#1785=ELLIPSE('',#52677,684.784865862975,42.3);
#1786=ELLIPSE('',#52679,148.655022233233,42.3);
#1787=ELLIPSE('',#52681,86.0962585581532,42.3);
#1788=ELLIPSE('',#52683,135.078923826262,42.3);
#1789=ELLIPSE('',#52686,135.078923826262,42.3);
#1790=ELLIPSE('',#52688,86.0962585581534,42.3);
#1791=ELLIPSE('',#52690,148.655022233233,42.3);
#1792=ELLIPSE('',#52692,684.784865862974,42.3);
#1793=ELLIPSE('',#52694,42.7157063175375,42.3);
#1794=ELLIPSE('',#52699,65.1465238200804,42.3);
#1795=ELLIPSE('',#52700,42.7157063175375,42.3);
#1796=ELLIPSE('',#52701,684.784865862975,42.3);
#1797=ELLIPSE('',#52702,148.655022233233,42.3);
#1798=ELLIPSE('',#52703,86.0962585581532,42.3);
#1799=ELLIPSE('',#52704,135.078923826262,42.3);
#1800=ELLIPSE('',#52705,135.078923826262,42.3);
#1801=ELLIPSE('',#52706,86.0962585581534,42.3);
#1802=ELLIPSE('',#52707,148.655022233233,42.3);
#1803=ELLIPSE('',#52708,684.784865862974,42.3);
#1804=ELLIPSE('',#52709,42.7157063175375,42.3);
#1805=ELLIPSE('',#52726,42.7157063175375,42.3);
#1806=ELLIPSE('',#52728,684.784865862975,42.3);
#1807=ELLIPSE('',#52730,148.655022233233,42.3);
#1808=ELLIPSE('',#52732,86.0962585581532,42.3);
#1809=ELLIPSE('',#52734,135.078923826262,42.3);
#1810=ELLIPSE('',#52737,135.078923826262,42.3);
#1811=ELLIPSE('',#52739,86.0962585581534,42.3);
#1812=ELLIPSE('',#52741,148.655022233233,42.3);
#1813=ELLIPSE('',#52743,684.784865862974,42.3);
#1814=ELLIPSE('',#52745,42.7157063175375,42.3);
#1815=ELLIPSE('',#52750,65.1465238200804,42.3);
#1816=ELLIPSE('',#52751,42.7157063175375,42.3);
#1817=ELLIPSE('',#52752,684.784865862975,42.3);
#1818=ELLIPSE('',#52753,148.655022233233,42.3);
#1819=ELLIPSE('',#52754,86.0962585581532,42.3);
#1820=ELLIPSE('',#52755,135.078923826262,42.3);
#1821=ELLIPSE('',#52756,135.078923826262,42.3);
#1822=ELLIPSE('',#52757,86.0962585581534,42.3);
#1823=ELLIPSE('',#52758,148.655022233233,42.3);
#1824=ELLIPSE('',#52759,684.784865862974,42.3);
#1825=ELLIPSE('',#52760,42.7157063175375,42.3);
#1826=ELLIPSE('',#52777,42.7157063175375,42.3);
#1827=ELLIPSE('',#52779,684.784865862975,42.3);
#1828=ELLIPSE('',#52781,148.655022233233,42.3);
#1829=ELLIPSE('',#52783,86.0962585581532,42.3);
#1830=ELLIPSE('',#52785,135.078923826262,42.3);
#1831=ELLIPSE('',#52788,135.078923826262,42.3);
#1832=ELLIPSE('',#52790,86.0962585581534,42.3);
#1833=ELLIPSE('',#52792,148.655022233233,42.3);
#1834=ELLIPSE('',#52794,684.784865862974,42.3);
#1835=ELLIPSE('',#52796,42.7157063175375,42.3);
#1836=ELLIPSE('',#52801,65.1465238200804,42.3);
#1837=ELLIPSE('',#52802,42.7157063175375,42.3);
#1838=ELLIPSE('',#52803,684.784865862975,42.3);
#1839=ELLIPSE('',#52804,148.655022233233,42.3);
#1840=ELLIPSE('',#52805,86.0962585581532,42.3);
#1841=ELLIPSE('',#52806,135.078923826262,42.3);
#1842=ELLIPSE('',#52807,135.078923826262,42.3);
#1843=ELLIPSE('',#52808,86.0962585581534,42.3);
#1844=ELLIPSE('',#52809,148.655022233233,42.3);
#1845=ELLIPSE('',#52810,684.784865862974,42.3);
#1846=ELLIPSE('',#52811,42.7157063175375,42.3);
#1847=ELLIPSE('',#52828,42.7157063175375,42.3);
#1848=ELLIPSE('',#52830,684.784865862975,42.3);
#1849=ELLIPSE('',#52832,148.655022233233,42.3);
#1850=ELLIPSE('',#52834,86.0962585581532,42.3);
#1851=ELLIPSE('',#52836,135.078923826262,42.3);
#1852=ELLIPSE('',#52839,135.078923826262,42.3);
#1853=ELLIPSE('',#52841,86.0962585581534,42.3);
#1854=ELLIPSE('',#52843,148.655022233233,42.3);
#1855=ELLIPSE('',#52845,684.784865862974,42.3);
#1856=ELLIPSE('',#52847,42.7157063175375,42.3);
#1857=ELLIPSE('',#52852,65.1465238200804,42.3);
#1858=ELLIPSE('',#52853,42.7157063175375,42.3);
#1859=ELLIPSE('',#52854,684.784865862975,42.3);
#1860=ELLIPSE('',#52855,148.655022233233,42.3);
#1861=ELLIPSE('',#52856,86.0962585581532,42.3);
#1862=ELLIPSE('',#52857,135.078923826262,42.3);
#1863=ELLIPSE('',#52858,135.078923826262,42.3);
#1864=ELLIPSE('',#52859,86.0962585581534,42.3);
#1865=ELLIPSE('',#52860,148.655022233233,42.3);
#1866=ELLIPSE('',#52861,684.784865862974,42.3);
#1867=ELLIPSE('',#52862,42.7157063175375,42.3);
#1868=ELLIPSE('',#52879,42.7157063175375,42.3);
#1869=ELLIPSE('',#52881,684.784865862975,42.3);
#1870=ELLIPSE('',#52883,148.655022233233,42.3);
#1871=ELLIPSE('',#52885,86.0962585581532,42.3);
#1872=ELLIPSE('',#52887,135.078923826262,42.3);
#1873=ELLIPSE('',#52890,135.078923826262,42.3);
#1874=ELLIPSE('',#52892,86.0962585581534,42.3);
#1875=ELLIPSE('',#52894,148.655022233233,42.3);
#1876=ELLIPSE('',#52896,684.784865862974,42.3);
#1877=ELLIPSE('',#52898,42.7157063175375,42.3);
#1878=ELLIPSE('',#52903,65.1465238200804,42.3);
#1879=ELLIPSE('',#52904,42.7157063175375,42.3);
#1880=ELLIPSE('',#52905,684.784865862975,42.3);
#1881=ELLIPSE('',#52906,148.655022233233,42.3);
#1882=ELLIPSE('',#52907,86.0962585581532,42.3);
#1883=ELLIPSE('',#52908,135.078923826262,42.3);
#1884=ELLIPSE('',#52909,135.078923826262,42.3);
#1885=ELLIPSE('',#52910,86.0962585581534,42.3);
#1886=ELLIPSE('',#52911,148.655022233233,42.3);
#1887=ELLIPSE('',#52912,684.784865862974,42.3);
#1888=ELLIPSE('',#52913,42.7157063175375,42.3);
#1889=ELLIPSE('',#52930,42.7157063175375,42.3);
#1890=ELLIPSE('',#52932,684.784865862975,42.3);
#1891=ELLIPSE('',#52934,148.655022233233,42.3);
#1892=ELLIPSE('',#52936,86.0962585581532,42.3);
#1893=ELLIPSE('',#52938,135.078923826262,42.3);
#1894=ELLIPSE('',#52941,135.078923826262,42.3);
#1895=ELLIPSE('',#52943,86.0962585581534,42.3);
#1896=ELLIPSE('',#52945,148.655022233233,42.3);
#1897=ELLIPSE('',#52947,684.784865862974,42.3);
#1898=ELLIPSE('',#52949,42.7157063175375,42.3);
#1899=ELLIPSE('',#52954,65.1465238200804,42.3);
#1900=ELLIPSE('',#52955,42.7157063175375,42.3);
#1901=ELLIPSE('',#52956,684.784865862975,42.3);
#1902=ELLIPSE('',#52957,148.655022233233,42.3);
#1903=ELLIPSE('',#52958,86.0962585581532,42.3);
#1904=ELLIPSE('',#52959,135.078923826262,42.3);
#1905=ELLIPSE('',#52960,135.078923826262,42.3);
#1906=ELLIPSE('',#52961,86.0962585581534,42.3);
#1907=ELLIPSE('',#52962,148.655022233233,42.3);
#1908=ELLIPSE('',#52963,684.784865862974,42.3);
#1909=ELLIPSE('',#52964,42.7157063175375,42.3);
#1910=ELLIPSE('',#52981,42.7157063175375,42.3);
#1911=ELLIPSE('',#52983,684.784865862975,42.3);
#1912=ELLIPSE('',#52985,148.655022233233,42.3);
#1913=ELLIPSE('',#52987,86.0962585581532,42.3);
#1914=ELLIPSE('',#52989,135.078923826262,42.3);
#1915=ELLIPSE('',#52992,135.078923826262,42.3);
#1916=ELLIPSE('',#52994,86.0962585581534,42.3);
#1917=ELLIPSE('',#52996,148.655022233233,42.3);
#1918=ELLIPSE('',#52998,684.784865862974,42.3);
#1919=ELLIPSE('',#53000,42.7157063175375,42.3);
#1920=ELLIPSE('',#53005,65.1465238200804,42.3);
#1921=ELLIPSE('',#53006,42.7157063175375,42.3);
#1922=ELLIPSE('',#53007,684.784865862975,42.3);
#1923=ELLIPSE('',#53008,148.655022233233,42.3);
#1924=ELLIPSE('',#53009,86.0962585581532,42.3);
#1925=ELLIPSE('',#53010,135.078923826262,42.3);
#1926=ELLIPSE('',#53011,135.078923826262,42.3);
#1927=ELLIPSE('',#53012,86.0962585581534,42.3);
#1928=ELLIPSE('',#53013,148.655022233233,42.3);
#1929=ELLIPSE('',#53014,684.784865862974,42.3);
#1930=ELLIPSE('',#53015,42.7157063175375,42.3);
#1931=ELLIPSE('',#53032,42.7157063175375,42.3);
#1932=ELLIPSE('',#53034,684.784865862975,42.3);
#1933=ELLIPSE('',#53036,148.655022233233,42.3);
#1934=ELLIPSE('',#53038,86.0962585581532,42.3);
#1935=ELLIPSE('',#53040,135.078923826262,42.3);
#1936=ELLIPSE('',#53043,135.078923826262,42.3);
#1937=ELLIPSE('',#53045,86.0962585581534,42.3);
#1938=ELLIPSE('',#53047,148.655022233233,42.3);
#1939=ELLIPSE('',#53049,684.784865862974,42.3);
#1940=ELLIPSE('',#53051,42.7157063175375,42.3);
#1941=ELLIPSE('',#53056,65.1465238200804,42.3);
#1942=ELLIPSE('',#53057,42.7157063175375,42.3);
#1943=ELLIPSE('',#53058,684.784865862975,42.3);
#1944=ELLIPSE('',#53059,148.655022233233,42.3);
#1945=ELLIPSE('',#53060,86.0962585581532,42.3);
#1946=ELLIPSE('',#53061,135.078923826262,42.3);
#1947=ELLIPSE('',#53062,135.078923826262,42.3);
#1948=ELLIPSE('',#53063,86.0962585581534,42.3);
#1949=ELLIPSE('',#53064,148.655022233233,42.3);
#1950=ELLIPSE('',#53065,684.784865862974,42.3);
#1951=ELLIPSE('',#53066,42.7157063175375,42.3);
#1952=ELLIPSE('',#53083,42.7157063175375,42.3);
#1953=ELLIPSE('',#53085,684.784865862975,42.3);
#1954=ELLIPSE('',#53087,148.655022233233,42.3);
#1955=ELLIPSE('',#53089,86.0962585581532,42.3);
#1956=ELLIPSE('',#53091,135.078923826262,42.3);
#1957=ELLIPSE('',#53094,135.078923826262,42.3);
#1958=ELLIPSE('',#53096,86.0962585581534,42.3);
#1959=ELLIPSE('',#53098,148.655022233233,42.3);
#1960=ELLIPSE('',#53100,684.784865862974,42.3);
#1961=ELLIPSE('',#53102,42.7157063175375,42.3);
#1962=ELLIPSE('',#53107,65.1465238200804,42.3);
#1963=ELLIPSE('',#53108,42.7157063175375,42.3);
#1964=ELLIPSE('',#53109,684.784865862975,42.3);
#1965=ELLIPSE('',#53110,148.655022233233,42.3);
#1966=ELLIPSE('',#53111,86.0962585581532,42.3);
#1967=ELLIPSE('',#53112,135.078923826262,42.3);
#1968=ELLIPSE('',#53113,135.078923826262,42.3);
#1969=ELLIPSE('',#53114,86.0962585581534,42.3);
#1970=ELLIPSE('',#53115,148.655022233233,42.3);
#1971=ELLIPSE('',#53116,684.784865862974,42.3);
#1972=ELLIPSE('',#53117,42.7157063175375,42.3);
#1973=ELLIPSE('',#53134,42.7157063175375,42.3);
#1974=ELLIPSE('',#53136,684.784865862975,42.3);
#1975=ELLIPSE('',#53138,148.655022233233,42.3);
#1976=ELLIPSE('',#53140,86.0962585581532,42.3);
#1977=ELLIPSE('',#53142,135.078923826262,42.3);
#1978=ELLIPSE('',#53145,135.078923826262,42.3);
#1979=ELLIPSE('',#53147,86.0962585581534,42.3);
#1980=ELLIPSE('',#53149,148.655022233233,42.3);
#1981=ELLIPSE('',#53151,684.784865862974,42.3);
#1982=ELLIPSE('',#53153,42.7157063175375,42.3);
#1983=ELLIPSE('',#53158,65.1465238200804,42.3);
#1984=ELLIPSE('',#53159,42.7157063175375,42.3);
#1985=ELLIPSE('',#53160,684.784865862975,42.3);
#1986=ELLIPSE('',#53161,148.655022233233,42.3);
#1987=ELLIPSE('',#53162,86.0962585581532,42.3);
#1988=ELLIPSE('',#53163,135.078923826262,42.3);
#1989=ELLIPSE('',#53164,135.078923826262,42.3);
#1990=ELLIPSE('',#53165,86.0962585581534,42.3);
#1991=ELLIPSE('',#53166,148.655022233233,42.3);
#1992=ELLIPSE('',#53167,684.784865862974,42.3);
#1993=ELLIPSE('',#53168,42.7157063175375,42.3);
#1994=ELLIPSE('',#53185,42.7157063175375,42.3);
#1995=ELLIPSE('',#53187,684.784865862975,42.3);
#1996=ELLIPSE('',#53189,148.655022233233,42.3);
#1997=ELLIPSE('',#53191,86.0962585581532,42.3);
#1998=ELLIPSE('',#53193,135.078923826262,42.3);
#1999=ELLIPSE('',#53196,135.078923826262,42.3);
#2000=ELLIPSE('',#53198,86.0962585581534,42.3);
#2001=ELLIPSE('',#53200,148.655022233233,42.3);
#2002=ELLIPSE('',#53202,684.784865862974,42.3);
#2003=ELLIPSE('',#53204,42.7157063175375,42.3);
#2004=ELLIPSE('',#53209,65.1465238200804,42.3);
#2005=ELLIPSE('',#53210,42.7157063175375,42.3);
#2006=ELLIPSE('',#53211,684.784865862975,42.3);
#2007=ELLIPSE('',#53212,148.655022233233,42.3);
#2008=ELLIPSE('',#53213,86.0962585581532,42.3);
#2009=ELLIPSE('',#53214,135.078923826262,42.3);
#2010=ELLIPSE('',#53215,135.078923826262,42.3);
#2011=ELLIPSE('',#53216,86.0962585581534,42.3);
#2012=ELLIPSE('',#53217,148.655022233233,42.3);
#2013=ELLIPSE('',#53218,684.784865862974,42.3);
#2014=ELLIPSE('',#53219,42.7157063175375,42.3);
#2015=ELLIPSE('',#53236,42.7157063175375,42.3);
#2016=ELLIPSE('',#53238,684.784865862975,42.3);
#2017=ELLIPSE('',#53240,148.655022233233,42.3);
#2018=ELLIPSE('',#53242,86.0962585581532,42.3);
#2019=ELLIPSE('',#53244,135.078923826262,42.3);
#2020=ELLIPSE('',#53247,135.078923826262,42.3);
#2021=ELLIPSE('',#53249,86.0962585581534,42.3);
#2022=ELLIPSE('',#53251,148.655022233233,42.3);
#2023=ELLIPSE('',#53253,684.784865862974,42.3);
#2024=ELLIPSE('',#53255,42.7157063175375,42.3);
#2025=ELLIPSE('',#53260,65.1465238200804,42.3);
#2026=ELLIPSE('',#53261,42.7157063175375,42.3);
#2027=ELLIPSE('',#53262,684.784865862975,42.3);
#2028=ELLIPSE('',#53263,148.655022233233,42.3);
#2029=ELLIPSE('',#53264,86.0962585581532,42.3);
#2030=ELLIPSE('',#53265,135.078923826262,42.3);
#2031=ELLIPSE('',#53266,135.078923826262,42.3);
#2032=ELLIPSE('',#53267,86.0962585581534,42.3);
#2033=ELLIPSE('',#53268,148.655022233233,42.3);
#2034=ELLIPSE('',#53269,684.784865862974,42.3);
#2035=ELLIPSE('',#53270,42.7157063175375,42.3);
#2036=ELLIPSE('',#53287,42.7157063175375,42.3);
#2037=ELLIPSE('',#53289,684.784865862975,42.3);
#2038=ELLIPSE('',#53291,148.655022233233,42.3);
#2039=ELLIPSE('',#53293,86.0962585581532,42.3);
#2040=ELLIPSE('',#53295,135.078923826262,42.3);
#2041=ELLIPSE('',#53298,135.078923826262,42.3);
#2042=ELLIPSE('',#53300,86.0962585581534,42.3);
#2043=ELLIPSE('',#53302,148.655022233233,42.3);
#2044=ELLIPSE('',#53304,684.784865862974,42.3);
#2045=ELLIPSE('',#53306,42.7157063175375,42.3);
#2046=ELLIPSE('',#53311,65.1465238200804,42.3);
#2047=ELLIPSE('',#53312,42.7157063175375,42.3);
#2048=ELLIPSE('',#53313,684.784865862975,42.3);
#2049=ELLIPSE('',#53314,148.655022233233,42.3);
#2050=ELLIPSE('',#53315,86.0962585581532,42.3);
#2051=ELLIPSE('',#53316,135.078923826262,42.3);
#2052=ELLIPSE('',#53317,135.078923826262,42.3);
#2053=ELLIPSE('',#53318,86.0962585581534,42.3);
#2054=ELLIPSE('',#53319,148.655022233233,42.3);
#2055=ELLIPSE('',#53320,684.784865862974,42.3);
#2056=ELLIPSE('',#53321,42.7157063175375,42.3);
#2057=ELLIPSE('',#53338,42.7157063175375,42.3);
#2058=ELLIPSE('',#53340,684.784865862975,42.3);
#2059=ELLIPSE('',#53342,148.655022233233,42.3);
#2060=ELLIPSE('',#53344,86.0962585581532,42.3);
#2061=ELLIPSE('',#53346,135.078923826262,42.3);
#2062=ELLIPSE('',#53349,135.078923826262,42.3);
#2063=ELLIPSE('',#53351,86.0962585581534,42.3);
#2064=ELLIPSE('',#53353,148.655022233233,42.3);
#2065=ELLIPSE('',#53355,684.784865862974,42.3);
#2066=ELLIPSE('',#53357,42.7157063175375,42.3);
#2067=ELLIPSE('',#53362,65.1465238200804,42.3);
#2068=ELLIPSE('',#53363,42.7157063175375,42.3);
#2069=ELLIPSE('',#53364,684.784865862975,42.3);
#2070=ELLIPSE('',#53365,148.655022233233,42.3);
#2071=ELLIPSE('',#53366,86.0962585581532,42.3);
#2072=ELLIPSE('',#53367,135.078923826262,42.3);
#2073=ELLIPSE('',#53368,135.078923826262,42.3);
#2074=ELLIPSE('',#53369,86.0962585581534,42.3);
#2075=ELLIPSE('',#53370,148.655022233233,42.3);
#2076=ELLIPSE('',#53371,684.784865862974,42.3);
#2077=ELLIPSE('',#53372,42.7157063175375,42.3);
#2078=ELLIPSE('',#53389,42.7157063175375,42.3);
#2079=ELLIPSE('',#53391,684.784865862975,42.3);
#2080=ELLIPSE('',#53393,148.655022233233,42.3);
#2081=ELLIPSE('',#53395,86.0962585581532,42.3);
#2082=ELLIPSE('',#53397,135.078923826262,42.3);
#2083=ELLIPSE('',#53400,135.078923826262,42.3);
#2084=ELLIPSE('',#53402,86.0962585581534,42.3);
#2085=ELLIPSE('',#53404,148.655022233233,42.3);
#2086=ELLIPSE('',#53406,684.784865862974,42.3);
#2087=ELLIPSE('',#53408,42.7157063175375,42.3);
#2088=ELLIPSE('',#53413,65.1465238200804,42.3);
#2089=ELLIPSE('',#53414,42.7157063175375,42.3);
#2090=ELLIPSE('',#53415,684.784865862975,42.3);
#2091=ELLIPSE('',#53416,148.655022233233,42.3);
#2092=ELLIPSE('',#53417,86.0962585581532,42.3);
#2093=ELLIPSE('',#53418,135.078923826262,42.3);
#2094=ELLIPSE('',#53419,135.078923826262,42.3);
#2095=ELLIPSE('',#53420,86.0962585581534,42.3);
#2096=ELLIPSE('',#53421,148.655022233233,42.3);
#2097=ELLIPSE('',#53422,684.784865862974,42.3);
#2098=ELLIPSE('',#53423,42.7157063175375,42.3);
#2099=ELLIPSE('',#53440,42.7157063175375,42.3);
#2100=ELLIPSE('',#53442,684.784865862975,42.3);
#2101=ELLIPSE('',#53444,148.655022233233,42.3);
#2102=ELLIPSE('',#53446,86.0962585581532,42.3);
#2103=ELLIPSE('',#53448,135.078923826262,42.3);
#2104=ELLIPSE('',#53451,135.078923826262,42.3);
#2105=ELLIPSE('',#53453,86.0962585581534,42.3);
#2106=ELLIPSE('',#53455,148.655022233233,42.3);
#2107=ELLIPSE('',#53457,684.784865862974,42.3);
#2108=ELLIPSE('',#53459,42.7157063175375,42.3);
#2109=ELLIPSE('',#53464,65.1465238200804,42.3);
#2110=ELLIPSE('',#53465,42.7157063175375,42.3);
#2111=ELLIPSE('',#53466,684.784865862975,42.3);
#2112=ELLIPSE('',#53467,148.655022233233,42.3);
#2113=ELLIPSE('',#53468,86.0962585581532,42.3);
#2114=ELLIPSE('',#53469,135.078923826262,42.3);
#2115=ELLIPSE('',#53470,135.078923826262,42.3);
#2116=ELLIPSE('',#53471,86.0962585581534,42.3);
#2117=ELLIPSE('',#53472,148.655022233233,42.3);
#2118=ELLIPSE('',#53473,684.784865862974,42.3);
#2119=ELLIPSE('',#53474,42.7157063175375,42.3);
#2120=ELLIPSE('',#53491,42.7157063175375,42.3);
#2121=ELLIPSE('',#53493,684.784865862975,42.3);
#2122=ELLIPSE('',#53495,148.655022233233,42.3);
#2123=ELLIPSE('',#53497,86.0962585581532,42.3);
#2124=ELLIPSE('',#53499,135.078923826262,42.3);
#2125=ELLIPSE('',#53502,135.078923826262,42.3);
#2126=ELLIPSE('',#53504,86.0962585581534,42.3);
#2127=ELLIPSE('',#53506,148.655022233233,42.3);
#2128=ELLIPSE('',#53508,684.784865862974,42.3);
#2129=ELLIPSE('',#53510,42.7157063175375,42.3);
#2130=ELLIPSE('',#53515,65.1465238200804,42.3);
#2131=ELLIPSE('',#53516,42.7157063175375,42.3);
#2132=ELLIPSE('',#53517,684.784865862975,42.3);
#2133=ELLIPSE('',#53518,148.655022233233,42.3);
#2134=ELLIPSE('',#53519,86.0962585581532,42.3);
#2135=ELLIPSE('',#53520,135.078923826262,42.3);
#2136=ELLIPSE('',#53521,135.078923826262,42.3);
#2137=ELLIPSE('',#53522,86.0962585581534,42.3);
#2138=ELLIPSE('',#53523,148.655022233233,42.3);
#2139=ELLIPSE('',#53524,684.784865862974,42.3);
#2140=ELLIPSE('',#53525,42.7157063175375,42.3);
#2141=ELLIPSE('',#53528,42.7157063175375,42.3);
#2142=ELLIPSE('',#53530,684.784865862975,42.3);
#2143=ELLIPSE('',#53532,148.655022233233,42.3);
#2144=ELLIPSE('',#53534,86.0962585581532,42.3);
#2145=ELLIPSE('',#53536,135.078923826262,42.3);
#2146=ELLIPSE('',#53539,135.078923826262,42.3);
#2147=ELLIPSE('',#53541,86.0962585581534,42.3);
#2148=ELLIPSE('',#53543,148.655022233233,42.3);
#2149=ELLIPSE('',#53545,684.784865862974,42.3);
#2150=ELLIPSE('',#53547,42.7157063175375,42.3);
#2151=ELLIPSE('',#53550,65.1465238200804,42.3);
#2160=LINE('',#68802,#6688);
#2161=LINE('',#68804,#6689);
#2162=LINE('',#68806,#6690);
#2163=LINE('',#68808,#6691);
#2164=LINE('',#68810,#6692);
#2165=LINE('',#68812,#6693);
#2166=LINE('',#68814,#6694);
#2167=LINE('',#68816,#6695);
#2168=LINE('',#68818,#6696);
#2169=LINE('',#68820,#6697);
#2170=LINE('',#68822,#6698);
#2171=LINE('',#68824,#6699);
#2172=LINE('',#68826,#6700);
#2173=LINE('',#68828,#6701);
#2174=LINE('',#68830,#6702);
#2175=LINE('',#68836,#6703);
#2176=LINE('',#68838,#6704);
#2177=LINE('',#68840,#6705);
#2178=LINE('',#68842,#6706);
#2179=LINE('',#68844,#6707);
#2180=LINE('',#68846,#6708);
#2181=LINE('',#68848,#6709);
#2182=LINE('',#68850,#6710);
#2183=LINE('',#68852,#6711);
#2184=LINE('',#68854,#6712);
#2185=LINE('',#68856,#6713);
#2186=LINE('',#68858,#6714);
#2187=LINE('',#68860,#6715);
#2188=LINE('',#68862,#6716);
#2189=LINE('',#68863,#6717);
#2190=LINE('',#68866,#6718);
#2191=LINE('',#68868,#6719);
#2192=LINE('',#68875,#6720);
#2193=LINE('',#68878,#6721);
#2194=LINE('',#68880,#6722);
#2195=LINE('',#68882,#6723);
#2196=LINE('',#68884,#6724);
#2197=LINE('',#68886,#6725);
#2198=LINE('',#68888,#6726);
#2199=LINE('',#68890,#6727);
#2200=LINE('',#68892,#6728);
#2201=LINE('',#68894,#6729);
#2202=LINE('',#68896,#6730);
#2203=LINE('',#68898,#6731);
#2204=LINE('',#68900,#6732);
#2205=LINE('',#68902,#6733);
#2206=LINE('',#68904,#6734);
#2207=LINE('',#68906,#6735);
#2208=LINE('',#68912,#6736);
#2209=LINE('',#68914,#6737);
#2210=LINE('',#68916,#6738);
#2211=LINE('',#68918,#6739);
#2212=LINE('',#68920,#6740);
#2213=LINE('',#68922,#6741);
#2214=LINE('',#68924,#6742);
#2215=LINE('',#68926,#6743);
#2216=LINE('',#68928,#6744);
#2217=LINE('',#68930,#6745);
#2218=LINE('',#68932,#6746);
#2219=LINE('',#68934,#6747);
#2220=LINE('',#68936,#6748);
#2221=LINE('',#68938,#6749);
#2222=LINE('',#68939,#6750);
#2223=LINE('',#68942,#6751);
#2224=LINE('',#68944,#6752);
#2225=LINE('',#68951,#6753);
#2226=LINE('',#68954,#6754);
#2227=LINE('',#68956,#6755);
#2228=LINE('',#68958,#6756);
#2229=LINE('',#68960,#6757);
#2230=LINE('',#68962,#6758);
#2231=LINE('',#68964,#6759);
#2232=LINE('',#68966,#6760);
#2233=LINE('',#68968,#6761);
#2234=LINE('',#68970,#6762);
#2235=LINE('',#68972,#6763);
#2236=LINE('',#68974,#6764);
#2237=LINE('',#68976,#6765);
#2238=LINE('',#68978,#6766);
#2239=LINE('',#68980,#6767);
#2240=LINE('',#68982,#6768);
#2241=LINE('',#68988,#6769);
#2242=LINE('',#68990,#6770);
#2243=LINE('',#68992,#6771);
#2244=LINE('',#68994,#6772);
#2245=LINE('',#68996,#6773);
#2246=LINE('',#68998,#6774);
#2247=LINE('',#69000,#6775);
#2248=LINE('',#69002,#6776);
#2249=LINE('',#69004,#6777);
#2250=LINE('',#69006,#6778);
#2251=LINE('',#69008,#6779);
#2252=LINE('',#69010,#6780);
#2253=LINE('',#69012,#6781);
#2254=LINE('',#69014,#6782);
#2255=LINE('',#69015,#6783);
#2256=LINE('',#69018,#6784);
#2257=LINE('',#69020,#6785);
#2258=LINE('',#69027,#6786);
#2259=LINE('',#69030,#6787);
#2260=LINE('',#69032,#6788);
#2261=LINE('',#69034,#6789);
#2262=LINE('',#69036,#6790);
#2263=LINE('',#69038,#6791);
#2264=LINE('',#69040,#6792);
#2265=LINE('',#69042,#6793);
#2266=LINE('',#69044,#6794);
#2267=LINE('',#69046,#6795);
#2268=LINE('',#69048,#6796);
#2269=LINE('',#69050,#6797);
#2270=LINE('',#69052,#6798);
#2271=LINE('',#69054,#6799);
#2272=LINE('',#69056,#6800);
#2273=LINE('',#69058,#6801);
#2274=LINE('',#69064,#6802);
#2275=LINE('',#69066,#6803);
#2276=LINE('',#69068,#6804);
#2277=LINE('',#69070,#6805);
#2278=LINE('',#69072,#6806);
#2279=LINE('',#69074,#6807);
#2280=LINE('',#69076,#6808);
#2281=LINE('',#69078,#6809);
#2282=LINE('',#69080,#6810);
#2283=LINE('',#69082,#6811);
#2284=LINE('',#69084,#6812);
#2285=LINE('',#69086,#6813);
#2286=LINE('',#69088,#6814);
#2287=LINE('',#69090,#6815);
#2288=LINE('',#69091,#6816);
#2289=LINE('',#69094,#6817);
#2290=LINE('',#69096,#6818);
#2291=LINE('',#69103,#6819);
#2292=LINE('',#69106,#6820);
#2293=LINE('',#69108,#6821);
#2294=LINE('',#69110,#6822);
#2295=LINE('',#69112,#6823);
#2296=LINE('',#69114,#6824);
#2297=LINE('',#69116,#6825);
#2298=LINE('',#69118,#6826);
#2299=LINE('',#69120,#6827);
#2300=LINE('',#69122,#6828);
#2301=LINE('',#69124,#6829);
#2302=LINE('',#69126,#6830);
#2303=LINE('',#69128,#6831);
#2304=LINE('',#69130,#6832);
#2305=LINE('',#69132,#6833);
#2306=LINE('',#69134,#6834);
#2307=LINE('',#69140,#6835);
#2308=LINE('',#69142,#6836);
#2309=LINE('',#69144,#6837);
#2310=LINE('',#69146,#6838);
#2311=LINE('',#69148,#6839);
#2312=LINE('',#69150,#6840);
#2313=LINE('',#69152,#6841);
#2314=LINE('',#69154,#6842);
#2315=LINE('',#69156,#6843);
#2316=LINE('',#69158,#6844);
#2317=LINE('',#69160,#6845);
#2318=LINE('',#69162,#6846);
#2319=LINE('',#69164,#6847);
#2320=LINE('',#69166,#6848);
#2321=LINE('',#69167,#6849);
#2322=LINE('',#69170,#6850);
#2323=LINE('',#69172,#6851);
#2324=LINE('',#69179,#6852);
#2325=LINE('',#69182,#6853);
#2326=LINE('',#69184,#6854);
#2327=LINE('',#69186,#6855);
#2328=LINE('',#69188,#6856);
#2329=LINE('',#69190,#6857);
#2330=LINE('',#69192,#6858);
#2331=LINE('',#69194,#6859);
#2332=LINE('',#69196,#6860);
#2333=LINE('',#69198,#6861);
#2334=LINE('',#69200,#6862);
#2335=LINE('',#69202,#6863);
#2336=LINE('',#69204,#6864);
#2337=LINE('',#69206,#6865);
#2338=LINE('',#69208,#6866);
#2339=LINE('',#69210,#6867);
#2340=LINE('',#69216,#6868);
#2341=LINE('',#69218,#6869);
#2342=LINE('',#69220,#6870);
#2343=LINE('',#69222,#6871);
#2344=LINE('',#69224,#6872);
#2345=LINE('',#69226,#6873);
#2346=LINE('',#69228,#6874);
#2347=LINE('',#69230,#6875);
#2348=LINE('',#69232,#6876);
#2349=LINE('',#69234,#6877);
#2350=LINE('',#69236,#6878);
#2351=LINE('',#69238,#6879);
#2352=LINE('',#69240,#6880);
#2353=LINE('',#69242,#6881);
#2354=LINE('',#69243,#6882);
#2355=LINE('',#69246,#6883);
#2356=LINE('',#69248,#6884);
#2357=LINE('',#69255,#6885);
#2358=LINE('',#69258,#6886);
#2359=LINE('',#69260,#6887);
#2360=LINE('',#69262,#6888);
#2361=LINE('',#69264,#6889);
#2362=LINE('',#69266,#6890);
#2363=LINE('',#69268,#6891);
#2364=LINE('',#69270,#6892);
#2365=LINE('',#69272,#6893);
#2366=LINE('',#69274,#6894);
#2367=LINE('',#69276,#6895);
#2368=LINE('',#69278,#6896);
#2369=LINE('',#69280,#6897);
#2370=LINE('',#69282,#6898);
#2371=LINE('',#69284,#6899);
#2372=LINE('',#69286,#6900);
#2373=LINE('',#69292,#6901);
#2374=LINE('',#69294,#6902);
#2375=LINE('',#69296,#6903);
#2376=LINE('',#69298,#6904);
#2377=LINE('',#69300,#6905);
#2378=LINE('',#69302,#6906);
#2379=LINE('',#69304,#6907);
#2380=LINE('',#69306,#6908);
#2381=LINE('',#69308,#6909);
#2382=LINE('',#69310,#6910);
#2383=LINE('',#69312,#6911);
#2384=LINE('',#69314,#6912);
#2385=LINE('',#69316,#6913);
#2386=LINE('',#69318,#6914);
#2387=LINE('',#69319,#6915);
#2388=LINE('',#69322,#6916);
#2389=LINE('',#69324,#6917);
#2390=LINE('',#69331,#6918);
#2391=LINE('',#69334,#6919);
#2392=LINE('',#69336,#6920);
#2393=LINE('',#69338,#6921);
#2394=LINE('',#69340,#6922);
#2395=LINE('',#69342,#6923);
#2396=LINE('',#69344,#6924);
#2397=LINE('',#69346,#6925);
#2398=LINE('',#69348,#6926);
#2399=LINE('',#69350,#6927);
#2400=LINE('',#69352,#6928);
#2401=LINE('',#69354,#6929);
#2402=LINE('',#69356,#6930);
#2403=LINE('',#69358,#6931);
#2404=LINE('',#69360,#6932);
#2405=LINE('',#69362,#6933);
#2406=LINE('',#69368,#6934);
#2407=LINE('',#69370,#6935);
#2408=LINE('',#69372,#6936);
#2409=LINE('',#69374,#6937);
#2410=LINE('',#69376,#6938);
#2411=LINE('',#69378,#6939);
#2412=LINE('',#69380,#6940);
#2413=LINE('',#69382,#6941);
#2414=LINE('',#69384,#6942);
#2415=LINE('',#69386,#6943);
#2416=LINE('',#69388,#6944);
#2417=LINE('',#69390,#6945);
#2418=LINE('',#69392,#6946);
#2419=LINE('',#69394,#6947);
#2420=LINE('',#69395,#6948);
#2421=LINE('',#69398,#6949);
#2422=LINE('',#69400,#6950);
#2423=LINE('',#69407,#6951);
#2424=LINE('',#69410,#6952);
#2425=LINE('',#69412,#6953);
#2426=LINE('',#69414,#6954);
#2427=LINE('',#69416,#6955);
#2428=LINE('',#69418,#6956);
#2429=LINE('',#69420,#6957);
#2430=LINE('',#69422,#6958);
#2431=LINE('',#69424,#6959);
#2432=LINE('',#69426,#6960);
#2433=LINE('',#69428,#6961);
#2434=LINE('',#69430,#6962);
#2435=LINE('',#69432,#6963);
#2436=LINE('',#69434,#6964);
#2437=LINE('',#69436,#6965);
#2438=LINE('',#69438,#6966);
#2439=LINE('',#69444,#6967);
#2440=LINE('',#69446,#6968);
#2441=LINE('',#69448,#6969);
#2442=LINE('',#69450,#6970);
#2443=LINE('',#69452,#6971);
#2444=LINE('',#69454,#6972);
#2445=LINE('',#69456,#6973);
#2446=LINE('',#69458,#6974);
#2447=LINE('',#69460,#6975);
#2448=LINE('',#69462,#6976);
#2449=LINE('',#69464,#6977);
#2450=LINE('',#69466,#6978);
#2451=LINE('',#69468,#6979);
#2452=LINE('',#69470,#6980);
#2453=LINE('',#69471,#6981);
#2454=LINE('',#69474,#6982);
#2455=LINE('',#69476,#6983);
#2456=LINE('',#69483,#6984);
#2457=LINE('',#69486,#6985);
#2458=LINE('',#69488,#6986);
#2459=LINE('',#69490,#6987);
#2460=LINE('',#69492,#6988);
#2461=LINE('',#69494,#6989);
#2462=LINE('',#69496,#6990);
#2463=LINE('',#69498,#6991);
#2464=LINE('',#69500,#6992);
#2465=LINE('',#69502,#6993);
#2466=LINE('',#69504,#6994);
#2467=LINE('',#69506,#6995);
#2468=LINE('',#69508,#6996);
#2469=LINE('',#69510,#6997);
#2470=LINE('',#69512,#6998);
#2471=LINE('',#69514,#6999);
#2472=LINE('',#69520,#7000);
#2473=LINE('',#69522,#7001);
#2474=LINE('',#69524,#7002);
#2475=LINE('',#69526,#7003);
#2476=LINE('',#69528,#7004);
#2477=LINE('',#69530,#7005);
#2478=LINE('',#69532,#7006);
#2479=LINE('',#69534,#7007);
#2480=LINE('',#69536,#7008);
#2481=LINE('',#69538,#7009);
#2482=LINE('',#69540,#7010);
#2483=LINE('',#69542,#7011);
#2484=LINE('',#69544,#7012);
#2485=LINE('',#69546,#7013);
#2486=LINE('',#69547,#7014);
#2487=LINE('',#69550,#7015);
#2488=LINE('',#69552,#7016);
#2489=LINE('',#69559,#7017);
#2490=LINE('',#69562,#7018);
#2491=LINE('',#69564,#7019);
#2492=LINE('',#69566,#7020);
#2493=LINE('',#69568,#7021);
#2494=LINE('',#69570,#7022);
#2495=LINE('',#69572,#7023);
#2496=LINE('',#69574,#7024);
#2497=LINE('',#69576,#7025);
#2498=LINE('',#69578,#7026);
#2499=LINE('',#69580,#7027);
#2500=LINE('',#69582,#7028);
#2501=LINE('',#69584,#7029);
#2502=LINE('',#69586,#7030);
#2503=LINE('',#69588,#7031);
#2504=LINE('',#69590,#7032);
#2505=LINE('',#69596,#7033);
#2506=LINE('',#69598,#7034);
#2507=LINE('',#69600,#7035);
#2508=LINE('',#69602,#7036);
#2509=LINE('',#69604,#7037);
#2510=LINE('',#69606,#7038);
#2511=LINE('',#69608,#7039);
#2512=LINE('',#69610,#7040);
#2513=LINE('',#69612,#7041);
#2514=LINE('',#69614,#7042);
#2515=LINE('',#69616,#7043);
#2516=LINE('',#69618,#7044);
#2517=LINE('',#69620,#7045);
#2518=LINE('',#69622,#7046);
#2519=LINE('',#69623,#7047);
#2520=LINE('',#69626,#7048);
#2521=LINE('',#69628,#7049);
#2522=LINE('',#69635,#7050);
#2523=LINE('',#69638,#7051);
#2524=LINE('',#69640,#7052);
#2525=LINE('',#69642,#7053);
#2526=LINE('',#69644,#7054);
#2527=LINE('',#69646,#7055);
#2528=LINE('',#69648,#7056);
#2529=LINE('',#69650,#7057);
#2530=LINE('',#69652,#7058);
#2531=LINE('',#69654,#7059);
#2532=LINE('',#69656,#7060);
#2533=LINE('',#69658,#7061);
#2534=LINE('',#69660,#7062);
#2535=LINE('',#69662,#7063);
#2536=LINE('',#69664,#7064);
#2537=LINE('',#69666,#7065);
#2538=LINE('',#69672,#7066);
#2539=LINE('',#69674,#7067);
#2540=LINE('',#69676,#7068);
#2541=LINE('',#69678,#7069);
#2542=LINE('',#69680,#7070);
#2543=LINE('',#69682,#7071);
#2544=LINE('',#69684,#7072);
#2545=LINE('',#69686,#7073);
#2546=LINE('',#69688,#7074);
#2547=LINE('',#69690,#7075);
#2548=LINE('',#69692,#7076);
#2549=LINE('',#69694,#7077);
#2550=LINE('',#69696,#7078);
#2551=LINE('',#69698,#7079);
#2552=LINE('',#69699,#7080);
#2553=LINE('',#69702,#7081);
#2554=LINE('',#69704,#7082);
#2555=LINE('',#69711,#7083);
#2556=LINE('',#69714,#7084);
#2557=LINE('',#69716,#7085);
#2558=LINE('',#69718,#7086);
#2559=LINE('',#69720,#7087);
#2560=LINE('',#69722,#7088);
#2561=LINE('',#69724,#7089);
#2562=LINE('',#69726,#7090);
#2563=LINE('',#69728,#7091);
#2564=LINE('',#69730,#7092);
#2565=LINE('',#69732,#7093);
#2566=LINE('',#69734,#7094);
#2567=LINE('',#69736,#7095);
#2568=LINE('',#69738,#7096);
#2569=LINE('',#69740,#7097);
#2570=LINE('',#69742,#7098);
#2571=LINE('',#69748,#7099);
#2572=LINE('',#69750,#7100);
#2573=LINE('',#69752,#7101);
#2574=LINE('',#69754,#7102);
#2575=LINE('',#69756,#7103);
#2576=LINE('',#69758,#7104);
#2577=LINE('',#69760,#7105);
#2578=LINE('',#69762,#7106);
#2579=LINE('',#69764,#7107);
#2580=LINE('',#69766,#7108);
#2581=LINE('',#69768,#7109);
#2582=LINE('',#69770,#7110);
#2583=LINE('',#69772,#7111);
#2584=LINE('',#69774,#7112);
#2585=LINE('',#69775,#7113);
#2586=LINE('',#69778,#7114);
#2587=LINE('',#69780,#7115);
#2588=LINE('',#69787,#7116);
#2589=LINE('',#69790,#7117);
#2590=LINE('',#69792,#7118);
#2591=LINE('',#69794,#7119);
#2592=LINE('',#69796,#7120);
#2593=LINE('',#69798,#7121);
#2594=LINE('',#69800,#7122);
#2595=LINE('',#69802,#7123);
#2596=LINE('',#69804,#7124);
#2597=LINE('',#69806,#7125);
#2598=LINE('',#69808,#7126);
#2599=LINE('',#69810,#7127);
#2600=LINE('',#69812,#7128);
#2601=LINE('',#69814,#7129);
#2602=LINE('',#69816,#7130);
#2603=LINE('',#69818,#7131);
#2604=LINE('',#69824,#7132);
#2605=LINE('',#69826,#7133);
#2606=LINE('',#69828,#7134);
#2607=LINE('',#69830,#7135);
#2608=LINE('',#69832,#7136);
#2609=LINE('',#69834,#7137);
#2610=LINE('',#69836,#7138);
#2611=LINE('',#69838,#7139);
#2612=LINE('',#69840,#7140);
#2613=LINE('',#69842,#7141);
#2614=LINE('',#69844,#7142);
#2615=LINE('',#69846,#7143);
#2616=LINE('',#69848,#7144);
#2617=LINE('',#69850,#7145);
#2618=LINE('',#69851,#7146);
#2619=LINE('',#69854,#7147);
#2620=LINE('',#69856,#7148);
#2621=LINE('',#69863,#7149);
#2622=LINE('',#69866,#7150);
#2623=LINE('',#69868,#7151);
#2624=LINE('',#69870,#7152);
#2625=LINE('',#69872,#7153);
#2626=LINE('',#69874,#7154);
#2627=LINE('',#69876,#7155);
#2628=LINE('',#69878,#7156);
#2629=LINE('',#69880,#7157);
#2630=LINE('',#69882,#7158);
#2631=LINE('',#69884,#7159);
#2632=LINE('',#69886,#7160);
#2633=LINE('',#69888,#7161);
#2634=LINE('',#69890,#7162);
#2635=LINE('',#69892,#7163);
#2636=LINE('',#69894,#7164);
#2637=LINE('',#69900,#7165);
#2638=LINE('',#69902,#7166);
#2639=LINE('',#69904,#7167);
#2640=LINE('',#69906,#7168);
#2641=LINE('',#69908,#7169);
#2642=LINE('',#69910,#7170);
#2643=LINE('',#69912,#7171);
#2644=LINE('',#69914,#7172);
#2645=LINE('',#69916,#7173);
#2646=LINE('',#69918,#7174);
#2647=LINE('',#69920,#7175);
#2648=LINE('',#69922,#7176);
#2649=LINE('',#69924,#7177);
#2650=LINE('',#69926,#7178);
#2651=LINE('',#69927,#7179);
#2652=LINE('',#69930,#7180);
#2653=LINE('',#69932,#7181);
#2654=LINE('',#69939,#7182);
#2655=LINE('',#69942,#7183);
#2656=LINE('',#69944,#7184);
#2657=LINE('',#69946,#7185);
#2658=LINE('',#69948,#7186);
#2659=LINE('',#69950,#7187);
#2660=LINE('',#69952,#7188);
#2661=LINE('',#69954,#7189);
#2662=LINE('',#69956,#7190);
#2663=LINE('',#69958,#7191);
#2664=LINE('',#69960,#7192);
#2665=LINE('',#69962,#7193);
#2666=LINE('',#69964,#7194);
#2667=LINE('',#69966,#7195);
#2668=LINE('',#69968,#7196);
#2669=LINE('',#69970,#7197);
#2670=LINE('',#69976,#7198);
#2671=LINE('',#69978,#7199);
#2672=LINE('',#69980,#7200);
#2673=LINE('',#69982,#7201);
#2674=LINE('',#69984,#7202);
#2675=LINE('',#69986,#7203);
#2676=LINE('',#69988,#7204);
#2677=LINE('',#69990,#7205);
#2678=LINE('',#69992,#7206);
#2679=LINE('',#69994,#7207);
#2680=LINE('',#69996,#7208);
#2681=LINE('',#69998,#7209);
#2682=LINE('',#70000,#7210);
#2683=LINE('',#70002,#7211);
#2684=LINE('',#70003,#7212);
#2685=LINE('',#70006,#7213);
#2686=LINE('',#70008,#7214);
#2687=LINE('',#70015,#7215);
#2688=LINE('',#70018,#7216);
#2689=LINE('',#70020,#7217);
#2690=LINE('',#70022,#7218);
#2691=LINE('',#70024,#7219);
#2692=LINE('',#70026,#7220);
#2693=LINE('',#70028,#7221);
#2694=LINE('',#70030,#7222);
#2695=LINE('',#70032,#7223);
#2696=LINE('',#70034,#7224);
#2697=LINE('',#70036,#7225);
#2698=LINE('',#70038,#7226);
#2699=LINE('',#70040,#7227);
#2700=LINE('',#70042,#7228);
#2701=LINE('',#70044,#7229);
#2702=LINE('',#70046,#7230);
#2703=LINE('',#70052,#7231);
#2704=LINE('',#70054,#7232);
#2705=LINE('',#70056,#7233);
#2706=LINE('',#70058,#7234);
#2707=LINE('',#70060,#7235);
#2708=LINE('',#70062,#7236);
#2709=LINE('',#70064,#7237);
#2710=LINE('',#70066,#7238);
#2711=LINE('',#70068,#7239);
#2712=LINE('',#70070,#7240);
#2713=LINE('',#70072,#7241);
#2714=LINE('',#70074,#7242);
#2715=LINE('',#70076,#7243);
#2716=LINE('',#70078,#7244);
#2717=LINE('',#70079,#7245);
#2718=LINE('',#70082,#7246);
#2719=LINE('',#70084,#7247);
#2720=LINE('',#70091,#7248);
#2721=LINE('',#70094,#7249);
#2722=LINE('',#70096,#7250);
#2723=LINE('',#70098,#7251);
#2724=LINE('',#70100,#7252);
#2725=LINE('',#70102,#7253);
#2726=LINE('',#70104,#7254);
#2727=LINE('',#70106,#7255);
#2728=LINE('',#70108,#7256);
#2729=LINE('',#70110,#7257);
#2730=LINE('',#70112,#7258);
#2731=LINE('',#70114,#7259);
#2732=LINE('',#70116,#7260);
#2733=LINE('',#70118,#7261);
#2734=LINE('',#70120,#7262);
#2735=LINE('',#70122,#7263);
#2736=LINE('',#70128,#7264);
#2737=LINE('',#70130,#7265);
#2738=LINE('',#70132,#7266);
#2739=LINE('',#70134,#7267);
#2740=LINE('',#70136,#7268);
#2741=LINE('',#70138,#7269);
#2742=LINE('',#70140,#7270);
#2743=LINE('',#70142,#7271);
#2744=LINE('',#70144,#7272);
#2745=LINE('',#70146,#7273);
#2746=LINE('',#70148,#7274);
#2747=LINE('',#70150,#7275);
#2748=LINE('',#70152,#7276);
#2749=LINE('',#70154,#7277);
#2750=LINE('',#70155,#7278);
#2751=LINE('',#70158,#7279);
#2752=LINE('',#70160,#7280);
#2753=LINE('',#70167,#7281);
#2754=LINE('',#70170,#7282);
#2755=LINE('',#70172,#7283);
#2756=LINE('',#70174,#7284);
#2757=LINE('',#70176,#7285);
#2758=LINE('',#70178,#7286);
#2759=LINE('',#70180,#7287);
#2760=LINE('',#70182,#7288);
#2761=LINE('',#70184,#7289);
#2762=LINE('',#70186,#7290);
#2763=LINE('',#70188,#7291);
#2764=LINE('',#70190,#7292);
#2765=LINE('',#70192,#7293);
#2766=LINE('',#70194,#7294);
#2767=LINE('',#70196,#7295);
#2768=LINE('',#70198,#7296);
#2769=LINE('',#70204,#7297);
#2770=LINE('',#70206,#7298);
#2771=LINE('',#70208,#7299);
#2772=LINE('',#70210,#7300);
#2773=LINE('',#70212,#7301);
#2774=LINE('',#70214,#7302);
#2775=LINE('',#70216,#7303);
#2776=LINE('',#70218,#7304);
#2777=LINE('',#70220,#7305);
#2778=LINE('',#70222,#7306);
#2779=LINE('',#70224,#7307);
#2780=LINE('',#70226,#7308);
#2781=LINE('',#70228,#7309);
#2782=LINE('',#70230,#7310);
#2783=LINE('',#70231,#7311);
#2784=LINE('',#70234,#7312);
#2785=LINE('',#70236,#7313);
#2786=LINE('',#70243,#7314);
#2787=LINE('',#70246,#7315);
#2788=LINE('',#70248,#7316);
#2789=LINE('',#70250,#7317);
#2790=LINE('',#70252,#7318);
#2791=LINE('',#70254,#7319);
#2792=LINE('',#70256,#7320);
#2793=LINE('',#70258,#7321);
#2794=LINE('',#70260,#7322);
#2795=LINE('',#70262,#7323);
#2796=LINE('',#70264,#7324);
#2797=LINE('',#70266,#7325);
#2798=LINE('',#70268,#7326);
#2799=LINE('',#70270,#7327);
#2800=LINE('',#70272,#7328);
#2801=LINE('',#70274,#7329);
#2802=LINE('',#70280,#7330);
#2803=LINE('',#70282,#7331);
#2804=LINE('',#70284,#7332);
#2805=LINE('',#70286,#7333);
#2806=LINE('',#70288,#7334);
#2807=LINE('',#70290,#7335);
#2808=LINE('',#70292,#7336);
#2809=LINE('',#70294,#7337);
#2810=LINE('',#70296,#7338);
#2811=LINE('',#70298,#7339);
#2812=LINE('',#70300,#7340);
#2813=LINE('',#70302,#7341);
#2814=LINE('',#70304,#7342);
#2815=LINE('',#70306,#7343);
#2816=LINE('',#70307,#7344);
#2817=LINE('',#70310,#7345);
#2818=LINE('',#70312,#7346);
#2819=LINE('',#70319,#7347);
#2820=LINE('',#70322,#7348);
#2821=LINE('',#70324,#7349);
#2822=LINE('',#70326,#7350);
#2823=LINE('',#70328,#7351);
#2824=LINE('',#70330,#7352);
#2825=LINE('',#70332,#7353);
#2826=LINE('',#70334,#7354);
#2827=LINE('',#70336,#7355);
#2828=LINE('',#70338,#7356);
#2829=LINE('',#70340,#7357);
#2830=LINE('',#70342,#7358);
#2831=LINE('',#70344,#7359);
#2832=LINE('',#70346,#7360);
#2833=LINE('',#70348,#7361);
#2834=LINE('',#70350,#7362);
#2835=LINE('',#70356,#7363);
#2836=LINE('',#70358,#7364);
#2837=LINE('',#70360,#7365);
#2838=LINE('',#70362,#7366);
#2839=LINE('',#70364,#7367);
#2840=LINE('',#70366,#7368);
#2841=LINE('',#70368,#7369);
#2842=LINE('',#70370,#7370);
#2843=LINE('',#70372,#7371);
#2844=LINE('',#70374,#7372);
#2845=LINE('',#70376,#7373);
#2846=LINE('',#70378,#7374);
#2847=LINE('',#70380,#7375);
#2848=LINE('',#70382,#7376);
#2849=LINE('',#70383,#7377);
#2850=LINE('',#70386,#7378);
#2851=LINE('',#70388,#7379);
#2852=LINE('',#70395,#7380);
#2853=LINE('',#70398,#7381);
#2854=LINE('',#70400,#7382);
#2855=LINE('',#70402,#7383);
#2856=LINE('',#70404,#7384);
#2857=LINE('',#70406,#7385);
#2858=LINE('',#70408,#7386);
#2859=LINE('',#70410,#7387);
#2860=LINE('',#70412,#7388);
#2861=LINE('',#70414,#7389);
#2862=LINE('',#70416,#7390);
#2863=LINE('',#70418,#7391);
#2864=LINE('',#70420,#7392);
#2865=LINE('',#70422,#7393);
#2866=LINE('',#70424,#7394);
#2867=LINE('',#70426,#7395);
#2868=LINE('',#70432,#7396);
#2869=LINE('',#70434,#7397);
#2870=LINE('',#70436,#7398);
#2871=LINE('',#70438,#7399);
#2872=LINE('',#70440,#7400);
#2873=LINE('',#70442,#7401);
#2874=LINE('',#70444,#7402);
#2875=LINE('',#70446,#7403);
#2876=LINE('',#70448,#7404);
#2877=LINE('',#70450,#7405);
#2878=LINE('',#70452,#7406);
#2879=LINE('',#70454,#7407);
#2880=LINE('',#70456,#7408);
#2881=LINE('',#70458,#7409);
#2882=LINE('',#70459,#7410);
#2883=LINE('',#70462,#7411);
#2884=LINE('',#70464,#7412);
#2885=LINE('',#70471,#7413);
#2886=LINE('',#70474,#7414);
#2887=LINE('',#70476,#7415);
#2888=LINE('',#70478,#7416);
#2889=LINE('',#70480,#7417);
#2890=LINE('',#70482,#7418);
#2891=LINE('',#70484,#7419);
#2892=LINE('',#70486,#7420);
#2893=LINE('',#70488,#7421);
#2894=LINE('',#70490,#7422);
#2895=LINE('',#70492,#7423);
#2896=LINE('',#70494,#7424);
#2897=LINE('',#70496,#7425);
#2898=LINE('',#70498,#7426);
#2899=LINE('',#70500,#7427);
#2900=LINE('',#70502,#7428);
#2901=LINE('',#70508,#7429);
#2902=LINE('',#70510,#7430);
#2903=LINE('',#70512,#7431);
#2904=LINE('',#70514,#7432);
#2905=LINE('',#70516,#7433);
#2906=LINE('',#70518,#7434);
#2907=LINE('',#70520,#7435);
#2908=LINE('',#70522,#7436);
#2909=LINE('',#70524,#7437);
#2910=LINE('',#70526,#7438);
#2911=LINE('',#70528,#7439);
#2912=LINE('',#70530,#7440);
#2913=LINE('',#70532,#7441);
#2914=LINE('',#70534,#7442);
#2915=LINE('',#70535,#7443);
#2916=LINE('',#70538,#7444);
#2917=LINE('',#70540,#7445);
#2918=LINE('',#70547,#7446);
#2919=LINE('',#70550,#7447);
#2920=LINE('',#70552,#7448);
#2921=LINE('',#70554,#7449);
#2922=LINE('',#70556,#7450);
#2923=LINE('',#70558,#7451);
#2924=LINE('',#70560,#7452);
#2925=LINE('',#70562,#7453);
#2926=LINE('',#70564,#7454);
#2927=LINE('',#70566,#7455);
#2928=LINE('',#70568,#7456);
#2929=LINE('',#70570,#7457);
#2930=LINE('',#70572,#7458);
#2931=LINE('',#70574,#7459);
#2932=LINE('',#70576,#7460);
#2933=LINE('',#70578,#7461);
#2934=LINE('',#70584,#7462);
#2935=LINE('',#70586,#7463);
#2936=LINE('',#70588,#7464);
#2937=LINE('',#70590,#7465);
#2938=LINE('',#70592,#7466);
#2939=LINE('',#70594,#7467);
#2940=LINE('',#70596,#7468);
#2941=LINE('',#70598,#7469);
#2942=LINE('',#70600,#7470);
#2943=LINE('',#70602,#7471);
#2944=LINE('',#70604,#7472);
#2945=LINE('',#70606,#7473);
#2946=LINE('',#70608,#7474);
#2947=LINE('',#70610,#7475);
#2948=LINE('',#70611,#7476);
#2949=LINE('',#70614,#7477);
#2950=LINE('',#70616,#7478);
#2951=LINE('',#70623,#7479);
#2952=LINE('',#70626,#7480);
#2953=LINE('',#70628,#7481);
#2954=LINE('',#70630,#7482);
#2955=LINE('',#70632,#7483);
#2956=LINE('',#70634,#7484);
#2957=LINE('',#70636,#7485);
#2958=LINE('',#70638,#7486);
#2959=LINE('',#70640,#7487);
#2960=LINE('',#70642,#7488);
#2961=LINE('',#70644,#7489);
#2962=LINE('',#70646,#7490);
#2963=LINE('',#70648,#7491);
#2964=LINE('',#70650,#7492);
#2965=LINE('',#70652,#7493);
#2966=LINE('',#70654,#7494);
#2967=LINE('',#70660,#7495);
#2968=LINE('',#70662,#7496);
#2969=LINE('',#70664,#7497);
#2970=LINE('',#70666,#7498);
#2971=LINE('',#70668,#7499);
#2972=LINE('',#70670,#7500);
#2973=LINE('',#70672,#7501);
#2974=LINE('',#70674,#7502);
#2975=LINE('',#70676,#7503);
#2976=LINE('',#70678,#7504);
#2977=LINE('',#70680,#7505);
#2978=LINE('',#70682,#7506);
#2979=LINE('',#70684,#7507);
#2980=LINE('',#70686,#7508);
#2981=LINE('',#70687,#7509);
#2982=LINE('',#70690,#7510);
#2983=LINE('',#70692,#7511);
#2984=LINE('',#70699,#7512);
#2985=LINE('',#70702,#7513);
#2986=LINE('',#70704,#7514);
#2987=LINE('',#70706,#7515);
#2988=LINE('',#70708,#7516);
#2989=LINE('',#70710,#7517);
#2990=LINE('',#70712,#7518);
#2991=LINE('',#70714,#7519);
#2992=LINE('',#70716,#7520);
#2993=LINE('',#70718,#7521);
#2994=LINE('',#70720,#7522);
#2995=LINE('',#70722,#7523);
#2996=LINE('',#70724,#7524);
#2997=LINE('',#70726,#7525);
#2998=LINE('',#70728,#7526);
#2999=LINE('',#70730,#7527);
#3000=LINE('',#70736,#7528);
#3001=LINE('',#70738,#7529);
#3002=LINE('',#70740,#7530);
#3003=LINE('',#70742,#7531);
#3004=LINE('',#70744,#7532);
#3005=LINE('',#70746,#7533);
#3006=LINE('',#70748,#7534);
#3007=LINE('',#70750,#7535);
#3008=LINE('',#70752,#7536);
#3009=LINE('',#70754,#7537);
#3010=LINE('',#70756,#7538);
#3011=LINE('',#70758,#7539);
#3012=LINE('',#70760,#7540);
#3013=LINE('',#70762,#7541);
#3014=LINE('',#70763,#7542);
#3015=LINE('',#70766,#7543);
#3016=LINE('',#70768,#7544);
#3017=LINE('',#70775,#7545);
#3018=LINE('',#70778,#7546);
#3019=LINE('',#70780,#7547);
#3020=LINE('',#70782,#7548);
#3021=LINE('',#70784,#7549);
#3022=LINE('',#70786,#7550);
#3023=LINE('',#70788,#7551);
#3024=LINE('',#70790,#7552);
#3025=LINE('',#70792,#7553);
#3026=LINE('',#70794,#7554);
#3027=LINE('',#70796,#7555);
#3028=LINE('',#70798,#7556);
#3029=LINE('',#70800,#7557);
#3030=LINE('',#70802,#7558);
#3031=LINE('',#70804,#7559);
#3032=LINE('',#70806,#7560);
#3033=LINE('',#70812,#7561);
#3034=LINE('',#70814,#7562);
#3035=LINE('',#70816,#7563);
#3036=LINE('',#70818,#7564);
#3037=LINE('',#70820,#7565);
#3038=LINE('',#70822,#7566);
#3039=LINE('',#70824,#7567);
#3040=LINE('',#70826,#7568);
#3041=LINE('',#70828,#7569);
#3042=LINE('',#70830,#7570);
#3043=LINE('',#70832,#7571);
#3044=LINE('',#70834,#7572);
#3045=LINE('',#70836,#7573);
#3046=LINE('',#70838,#7574);
#3047=LINE('',#70839,#7575);
#3048=LINE('',#70842,#7576);
#3049=LINE('',#70844,#7577);
#3050=LINE('',#70851,#7578);
#3051=LINE('',#70854,#7579);
#3052=LINE('',#70856,#7580);
#3053=LINE('',#70858,#7581);
#3054=LINE('',#70860,#7582);
#3055=LINE('',#70862,#7583);
#3056=LINE('',#70864,#7584);
#3057=LINE('',#70866,#7585);
#3058=LINE('',#70868,#7586);
#3059=LINE('',#70870,#7587);
#3060=LINE('',#70872,#7588);
#3061=LINE('',#70874,#7589);
#3062=LINE('',#70876,#7590);
#3063=LINE('',#70878,#7591);
#3064=LINE('',#70880,#7592);
#3065=LINE('',#70882,#7593);
#3066=LINE('',#70888,#7594);
#3067=LINE('',#70890,#7595);
#3068=LINE('',#70892,#7596);
#3069=LINE('',#70894,#7597);
#3070=LINE('',#70896,#7598);
#3071=LINE('',#70898,#7599);
#3072=LINE('',#70900,#7600);
#3073=LINE('',#70902,#7601);
#3074=LINE('',#70904,#7602);
#3075=LINE('',#70906,#7603);
#3076=LINE('',#70908,#7604);
#3077=LINE('',#70910,#7605);
#3078=LINE('',#70912,#7606);
#3079=LINE('',#70914,#7607);
#3080=LINE('',#70915,#7608);
#3081=LINE('',#70918,#7609);
#3082=LINE('',#70920,#7610);
#3083=LINE('',#70927,#7611);
#3084=LINE('',#70930,#7612);
#3085=LINE('',#70932,#7613);
#3086=LINE('',#70934,#7614);
#3087=LINE('',#70936,#7615);
#3088=LINE('',#70938,#7616);
#3089=LINE('',#70940,#7617);
#3090=LINE('',#70942,#7618);
#3091=LINE('',#70944,#7619);
#3092=LINE('',#70946,#7620);
#3093=LINE('',#70948,#7621);
#3094=LINE('',#70950,#7622);
#3095=LINE('',#70952,#7623);
#3096=LINE('',#70954,#7624);
#3097=LINE('',#70956,#7625);
#3098=LINE('',#70958,#7626);
#3099=LINE('',#70964,#7627);
#3100=LINE('',#70966,#7628);
#3101=LINE('',#70968,#7629);
#3102=LINE('',#70970,#7630);
#3103=LINE('',#70972,#7631);
#3104=LINE('',#70974,#7632);
#3105=LINE('',#70976,#7633);
#3106=LINE('',#70978,#7634);
#3107=LINE('',#70980,#7635);
#3108=LINE('',#70982,#7636);
#3109=LINE('',#70984,#7637);
#3110=LINE('',#70986,#7638);
#3111=LINE('',#70988,#7639);
#3112=LINE('',#70990,#7640);
#3113=LINE('',#70991,#7641);
#3114=LINE('',#70994,#7642);
#3115=LINE('',#70996,#7643);
#3116=LINE('',#71003,#7644);
#3117=LINE('',#71006,#7645);
#3118=LINE('',#71008,#7646);
#3119=LINE('',#71010,#7647);
#3120=LINE('',#71012,#7648);
#3121=LINE('',#71014,#7649);
#3122=LINE('',#71016,#7650);
#3123=LINE('',#71018,#7651);
#3124=LINE('',#71020,#7652);
#3125=LINE('',#71022,#7653);
#3126=LINE('',#71024,#7654);
#3127=LINE('',#71026,#7655);
#3128=LINE('',#71028,#7656);
#3129=LINE('',#71030,#7657);
#3130=LINE('',#71032,#7658);
#3131=LINE('',#71034,#7659);
#3132=LINE('',#71040,#7660);
#3133=LINE('',#71042,#7661);
#3134=LINE('',#71044,#7662);
#3135=LINE('',#71046,#7663);
#3136=LINE('',#71048,#7664);
#3137=LINE('',#71050,#7665);
#3138=LINE('',#71052,#7666);
#3139=LINE('',#71054,#7667);
#3140=LINE('',#71056,#7668);
#3141=LINE('',#71058,#7669);
#3142=LINE('',#71060,#7670);
#3143=LINE('',#71062,#7671);
#3144=LINE('',#71064,#7672);
#3145=LINE('',#71066,#7673);
#3146=LINE('',#71067,#7674);
#3147=LINE('',#71070,#7675);
#3148=LINE('',#71072,#7676);
#3149=LINE('',#71079,#7677);
#3150=LINE('',#71082,#7678);
#3151=LINE('',#71084,#7679);
#3152=LINE('',#71086,#7680);
#3153=LINE('',#71088,#7681);
#3154=LINE('',#71090,#7682);
#3155=LINE('',#71092,#7683);
#3156=LINE('',#71094,#7684);
#3157=LINE('',#71096,#7685);
#3158=LINE('',#71098,#7686);
#3159=LINE('',#71100,#7687);
#3160=LINE('',#71102,#7688);
#3161=LINE('',#71104,#7689);
#3162=LINE('',#71106,#7690);
#3163=LINE('',#71108,#7691);
#3164=LINE('',#71110,#7692);
#3165=LINE('',#71116,#7693);
#3166=LINE('',#71118,#7694);
#3167=LINE('',#71120,#7695);
#3168=LINE('',#71122,#7696);
#3169=LINE('',#71124,#7697);
#3170=LINE('',#71126,#7698);
#3171=LINE('',#71128,#7699);
#3172=LINE('',#71130,#7700);
#3173=LINE('',#71132,#7701);
#3174=LINE('',#71134,#7702);
#3175=LINE('',#71136,#7703);
#3176=LINE('',#71138,#7704);
#3177=LINE('',#71140,#7705);
#3178=LINE('',#71142,#7706);
#3179=LINE('',#71143,#7707);
#3180=LINE('',#71146,#7708);
#3181=LINE('',#71148,#7709);
#3182=LINE('',#71155,#7710);
#3183=LINE('',#71158,#7711);
#3184=LINE('',#71160,#7712);
#3185=LINE('',#71162,#7713);
#3186=LINE('',#71164,#7714);
#3187=LINE('',#71166,#7715);
#3188=LINE('',#71168,#7716);
#3189=LINE('',#71170,#7717);
#3190=LINE('',#71172,#7718);
#3191=LINE('',#71174,#7719);
#3192=LINE('',#71176,#7720);
#3193=LINE('',#71178,#7721);
#3194=LINE('',#71180,#7722);
#3195=LINE('',#71182,#7723);
#3196=LINE('',#71184,#7724);
#3197=LINE('',#71186,#7725);
#3198=LINE('',#71192,#7726);
#3199=LINE('',#71194,#7727);
#3200=LINE('',#71196,#7728);
#3201=LINE('',#71198,#7729);
#3202=LINE('',#71200,#7730);
#3203=LINE('',#71202,#7731);
#3204=LINE('',#71204,#7732);
#3205=LINE('',#71206,#7733);
#3206=LINE('',#71208,#7734);
#3207=LINE('',#71210,#7735);
#3208=LINE('',#71212,#7736);
#3209=LINE('',#71214,#7737);
#3210=LINE('',#71216,#7738);
#3211=LINE('',#71218,#7739);
#3212=LINE('',#71219,#7740);
#3213=LINE('',#71222,#7741);
#3214=LINE('',#71224,#7742);
#3215=LINE('',#71231,#7743);
#3216=LINE('',#71234,#7744);
#3217=LINE('',#71236,#7745);
#3218=LINE('',#71238,#7746);
#3219=LINE('',#71240,#7747);
#3220=LINE('',#71242,#7748);
#3221=LINE('',#71244,#7749);
#3222=LINE('',#71246,#7750);
#3223=LINE('',#71248,#7751);
#3224=LINE('',#71250,#7752);
#3225=LINE('',#71252,#7753);
#3226=LINE('',#71254,#7754);
#3227=LINE('',#71256,#7755);
#3228=LINE('',#71258,#7756);
#3229=LINE('',#71260,#7757);
#3230=LINE('',#71262,#7758);
#3231=LINE('',#71268,#7759);
#3232=LINE('',#71270,#7760);
#3233=LINE('',#71272,#7761);
#3234=LINE('',#71274,#7762);
#3235=LINE('',#71276,#7763);
#3236=LINE('',#71278,#7764);
#3237=LINE('',#71280,#7765);
#3238=LINE('',#71282,#7766);
#3239=LINE('',#71284,#7767);
#3240=LINE('',#71286,#7768);
#3241=LINE('',#71288,#7769);
#3242=LINE('',#71290,#7770);
#3243=LINE('',#71292,#7771);
#3244=LINE('',#71294,#7772);
#3245=LINE('',#71295,#7773);
#3246=LINE('',#71298,#7774);
#3247=LINE('',#71300,#7775);
#3248=LINE('',#71307,#7776);
#3249=LINE('',#71310,#7777);
#3250=LINE('',#71312,#7778);
#3251=LINE('',#71314,#7779);
#3252=LINE('',#71316,#7780);
#3253=LINE('',#71318,#7781);
#3254=LINE('',#71320,#7782);
#3255=LINE('',#71322,#7783);
#3256=LINE('',#71324,#7784);
#3257=LINE('',#71326,#7785);
#3258=LINE('',#71328,#7786);
#3259=LINE('',#71330,#7787);
#3260=LINE('',#71332,#7788);
#3261=LINE('',#71334,#7789);
#3262=LINE('',#71336,#7790);
#3263=LINE('',#71338,#7791);
#3264=LINE('',#71344,#7792);
#3265=LINE('',#71346,#7793);
#3266=LINE('',#71348,#7794);
#3267=LINE('',#71350,#7795);
#3268=LINE('',#71352,#7796);
#3269=LINE('',#71354,#7797);
#3270=LINE('',#71356,#7798);
#3271=LINE('',#71358,#7799);
#3272=LINE('',#71360,#7800);
#3273=LINE('',#71362,#7801);
#3274=LINE('',#71364,#7802);
#3275=LINE('',#71366,#7803);
#3276=LINE('',#71368,#7804);
#3277=LINE('',#71370,#7805);
#3278=LINE('',#71371,#7806);
#3279=LINE('',#71374,#7807);
#3280=LINE('',#71376,#7808);
#3281=LINE('',#71383,#7809);
#3282=LINE('',#71386,#7810);
#3283=LINE('',#71388,#7811);
#3284=LINE('',#71390,#7812);
#3285=LINE('',#71392,#7813);
#3286=LINE('',#71394,#7814);
#3287=LINE('',#71396,#7815);
#3288=LINE('',#71398,#7816);
#3289=LINE('',#71400,#7817);
#3290=LINE('',#71402,#7818);
#3291=LINE('',#71404,#7819);
#3292=LINE('',#71406,#7820);
#3293=LINE('',#71408,#7821);
#3294=LINE('',#71410,#7822);
#3295=LINE('',#71412,#7823);
#3296=LINE('',#71414,#7824);
#3297=LINE('',#71420,#7825);
#3298=LINE('',#71422,#7826);
#3299=LINE('',#71424,#7827);
#3300=LINE('',#71426,#7828);
#3301=LINE('',#71428,#7829);
#3302=LINE('',#71430,#7830);
#3303=LINE('',#71432,#7831);
#3304=LINE('',#71434,#7832);
#3305=LINE('',#71436,#7833);
#3306=LINE('',#71438,#7834);
#3307=LINE('',#71440,#7835);
#3308=LINE('',#71442,#7836);
#3309=LINE('',#71444,#7837);
#3310=LINE('',#71446,#7838);
#3311=LINE('',#71447,#7839);
#3312=LINE('',#71450,#7840);
#3313=LINE('',#71452,#7841);
#3314=LINE('',#71459,#7842);
#3315=LINE('',#71462,#7843);
#3316=LINE('',#71464,#7844);
#3317=LINE('',#71466,#7845);
#3318=LINE('',#71468,#7846);
#3319=LINE('',#71470,#7847);
#3320=LINE('',#71472,#7848);
#3321=LINE('',#71474,#7849);
#3322=LINE('',#71476,#7850);
#3323=LINE('',#71478,#7851);
#3324=LINE('',#71480,#7852);
#3325=LINE('',#71482,#7853);
#3326=LINE('',#71484,#7854);
#3327=LINE('',#71486,#7855);
#3328=LINE('',#71488,#7856);
#3329=LINE('',#71490,#7857);
#3330=LINE('',#71496,#7858);
#3331=LINE('',#71498,#7859);
#3332=LINE('',#71500,#7860);
#3333=LINE('',#71502,#7861);
#3334=LINE('',#71504,#7862);
#3335=LINE('',#71506,#7863);
#3336=LINE('',#71508,#7864);
#3337=LINE('',#71510,#7865);
#3338=LINE('',#71512,#7866);
#3339=LINE('',#71514,#7867);
#3340=LINE('',#71516,#7868);
#3341=LINE('',#71518,#7869);
#3342=LINE('',#71520,#7870);
#3343=LINE('',#71522,#7871);
#3344=LINE('',#71523,#7872);
#3345=LINE('',#71526,#7873);
#3346=LINE('',#71528,#7874);
#3347=LINE('',#71535,#7875);
#3348=LINE('',#71898,#7876);
#3349=LINE('',#71900,#7877);
#3350=LINE('',#71907,#7878);
#3351=LINE('',#71910,#7879);
#3352=LINE('',#71912,#7880);
#3353=LINE('',#71919,#7881);
#3354=LINE('',#71922,#7882);
#3355=LINE('',#71924,#7883);
#3356=LINE('',#71931,#7884);
#3357=LINE('',#71934,#7885);
#3358=LINE('',#71936,#7886);
#3359=LINE('',#71943,#7887);
#3360=LINE('',#71946,#7888);
#3361=LINE('',#71948,#7889);
#3362=LINE('',#71955,#7890);
#3363=LINE('',#71958,#7891);
#3364=LINE('',#71960,#7892);
#3365=LINE('',#71967,#7893);
#3366=LINE('',#71970,#7894);
#3367=LINE('',#71972,#7895);
#3368=LINE('',#71979,#7896);
#3369=LINE('',#71982,#7897);
#3370=LINE('',#71984,#7898);
#3371=LINE('',#71991,#7899);
#3372=LINE('',#71994,#7900);
#3373=LINE('',#71996,#7901);
#3374=LINE('',#72003,#7902);
#3375=LINE('',#72006,#7903);
#3376=LINE('',#72008,#7904);
#3377=LINE('',#72015,#7905);
#3378=LINE('',#72018,#7906);
#3379=LINE('',#72020,#7907);
#3380=LINE('',#72027,#7908);
#3381=LINE('',#72030,#7909);
#3382=LINE('',#72032,#7910);
#3383=LINE('',#72039,#7911);
#3384=LINE('',#72042,#7912);
#3385=LINE('',#72044,#7913);
#3386=LINE('',#72051,#7914);
#3387=LINE('',#72054,#7915);
#3388=LINE('',#72056,#7916);
#3389=LINE('',#72063,#7917);
#3390=LINE('',#72066,#7918);
#3391=LINE('',#72068,#7919);
#3392=LINE('',#72075,#7920);
#3393=LINE('',#72078,#7921);
#3394=LINE('',#72080,#7922);
#3395=LINE('',#72087,#7923);
#3396=LINE('',#72090,#7924);
#3397=LINE('',#72092,#7925);
#3398=LINE('',#72099,#7926);
#3399=LINE('',#72102,#7927);
#3400=LINE('',#72104,#7928);
#3401=LINE('',#72111,#7929);
#3402=LINE('',#72114,#7930);
#3403=LINE('',#72116,#7931);
#3404=LINE('',#72123,#7932);
#3405=LINE('',#72126,#7933);
#3406=LINE('',#72128,#7934);
#3407=LINE('',#72135,#7935);
#3408=LINE('',#72138,#7936);
#3409=LINE('',#72140,#7937);
#3410=LINE('',#72147,#7938);
#3411=LINE('',#72150,#7939);
#3412=LINE('',#72152,#7940);
#3413=LINE('',#72159,#7941);
#3414=LINE('',#72162,#7942);
#3415=LINE('',#72164,#7943);
#3416=LINE('',#72171,#7944);
#3417=LINE('',#72174,#7945);
#3418=LINE('',#72176,#7946);
#3419=LINE('',#72183,#7947);
#3420=LINE('',#72186,#7948);
#3421=LINE('',#72188,#7949);
#3422=LINE('',#72195,#7950);
#3423=LINE('',#72198,#7951);
#3424=LINE('',#72200,#7952);
#3425=LINE('',#72207,#7953);
#3426=LINE('',#72210,#7954);
#3427=LINE('',#72212,#7955);
#3428=LINE('',#72219,#7956);
#3429=LINE('',#72222,#7957);
#3430=LINE('',#72224,#7958);
#3431=LINE('',#72231,#7959);
#3432=LINE('',#72234,#7960);
#3433=LINE('',#72236,#7961);
#3434=LINE('',#72243,#7962);
#3435=LINE('',#72246,#7963);
#3436=LINE('',#72248,#7964);
#3437=LINE('',#72255,#7965);
#3438=LINE('',#72258,#7966);
#3439=LINE('',#72260,#7967);
#3440=LINE('',#72267,#7968);
#3441=LINE('',#72270,#7969);
#3442=LINE('',#72272,#7970);
#3443=LINE('',#72279,#7971);
#3444=LINE('',#72282,#7972);
#3445=LINE('',#72284,#7973);
#3446=LINE('',#72291,#7974);
#3447=LINE('',#72294,#7975);
#3448=LINE('',#72296,#7976);
#3449=LINE('',#72303,#7977);
#3450=LINE('',#72306,#7978);
#3451=LINE('',#72308,#7979);
#3452=LINE('',#72315,#7980);
#3453=LINE('',#72318,#7981);
#3454=LINE('',#72320,#7982);
#3455=LINE('',#72327,#7983);
#3456=LINE('',#72330,#7984);
#3457=LINE('',#72331,#7985);
#3458=LINE('',#72334,#7986);
#3459=LINE('',#72335,#7987);
#3460=LINE('',#72338,#7988);
#3461=LINE('',#72339,#7989);
#3462=LINE('',#72342,#7990);
#3463=LINE('',#72343,#7991);
#3464=LINE('',#72346,#7992);
#3465=LINE('',#72347,#7993);
#3466=LINE('',#72350,#7994);
#3467=LINE('',#72351,#7995);
#3468=LINE('',#72354,#7996);
#3469=LINE('',#72355,#7997);
#3470=LINE('',#72358,#7998);
#3471=LINE('',#72359,#7999);
#3472=LINE('',#72362,#8000);
#3473=LINE('',#72363,#8001);
#3474=LINE('',#72366,#8002);
#3475=LINE('',#72367,#8003);
#3476=LINE('',#72370,#8004);
#3477=LINE('',#72371,#8005);
#3478=LINE('',#72374,#8006);
#3479=LINE('',#72375,#8007);
#3480=LINE('',#72378,#8008);
#3481=LINE('',#72379,#8009);
#3482=LINE('',#72382,#8010);
#3483=LINE('',#72383,#8011);
#3484=LINE('',#72386,#8012);
#3485=LINE('',#72387,#8013);
#3486=LINE('',#72390,#8014);
#3487=LINE('',#72391,#8015);
#3488=LINE('',#72394,#8016);
#3489=LINE('',#72395,#8017);
#3490=LINE('',#72398,#8018);
#3491=LINE('',#72399,#8019);
#3492=LINE('',#72402,#8020);
#3493=LINE('',#72403,#8021);
#3494=LINE('',#72406,#8022);
#3495=LINE('',#72407,#8023);
#3496=LINE('',#72410,#8024);
#3497=LINE('',#72411,#8025);
#3498=LINE('',#72414,#8026);
#3499=LINE('',#72415,#8027);
#3500=LINE('',#72418,#8028);
#3501=LINE('',#72419,#8029);
#3502=LINE('',#72422,#8030);
#3503=LINE('',#72423,#8031);
#3504=LINE('',#72426,#8032);
#3505=LINE('',#72427,#8033);
#3506=LINE('',#72430,#8034);
#3507=LINE('',#72431,#8035);
#3508=LINE('',#72434,#8036);
#3509=LINE('',#72435,#8037);
#3510=LINE('',#72438,#8038);
#3511=LINE('',#72439,#8039);
#3512=LINE('',#72442,#8040);
#3513=LINE('',#72443,#8041);
#3514=LINE('',#72446,#8042);
#3515=LINE('',#72447,#8043);
#3516=LINE('',#72450,#8044);
#3517=LINE('',#72451,#8045);
#3518=LINE('',#72454,#8046);
#3519=LINE('',#72455,#8047);
#3520=LINE('',#72458,#8048);
#3521=LINE('',#72459,#8049);
#3522=LINE('',#72462,#8050);
#3523=LINE('',#72463,#8051);
#3524=LINE('',#72466,#8052);
#3525=LINE('',#72467,#8053);
#3526=LINE('',#72470,#8054);
#3527=LINE('',#72471,#8055);
#3528=LINE('',#72474,#8056);
#3529=LINE('',#72481,#8057);
#3530=LINE('',#72484,#8058);
#3531=LINE('',#72491,#8059);
#3532=LINE('',#72494,#8060);
#3533=LINE('',#72501,#8061);
#3534=LINE('',#72504,#8062);
#3535=LINE('',#72511,#8063);
#3536=LINE('',#72514,#8064);
#3537=LINE('',#72521,#8065);
#3538=LINE('',#72524,#8066);
#3539=LINE('',#72531,#8067);
#3540=LINE('',#72534,#8068);
#3541=LINE('',#72541,#8069);
#3542=LINE('',#72544,#8070);
#3543=LINE('',#72551,#8071);
#3544=LINE('',#72554,#8072);
#3545=LINE('',#72561,#8073);
#3546=LINE('',#72564,#8074);
#3547=LINE('',#72571,#8075);
#3548=LINE('',#72574,#8076);
#3549=LINE('',#72581,#8077);
#3550=LINE('',#72584,#8078);
#3551=LINE('',#72591,#8079);
#3552=LINE('',#72594,#8080);
#3553=LINE('',#72601,#8081);
#3554=LINE('',#72604,#8082);
#3555=LINE('',#72611,#8083);
#3556=LINE('',#72614,#8084);
#3557=LINE('',#72621,#8085);
#3558=LINE('',#72624,#8086);
#3559=LINE('',#72631,#8087);
#3560=LINE('',#72634,#8088);
#3561=LINE('',#72641,#8089);
#3562=LINE('',#72644,#8090);
#3563=LINE('',#72651,#8091);
#3564=LINE('',#72654,#8092);
#3565=LINE('',#72661,#8093);
#3566=LINE('',#72664,#8094);
#3567=LINE('',#72671,#8095);
#3568=LINE('',#72674,#8096);
#3569=LINE('',#72681,#8097);
#3570=LINE('',#72684,#8098);
#3571=LINE('',#72691,#8099);
#3572=LINE('',#72694,#8100);
#3573=LINE('',#72701,#8101);
#3574=LINE('',#72704,#8102);
#3575=LINE('',#72711,#8103);
#3576=LINE('',#72714,#8104);
#3577=LINE('',#72721,#8105);
#3578=LINE('',#72724,#8106);
#3579=LINE('',#72731,#8107);
#3580=LINE('',#72734,#8108);
#3581=LINE('',#72741,#8109);
#3582=LINE('',#72744,#8110);
#3583=LINE('',#72751,#8111);
#3584=LINE('',#72754,#8112);
#3585=LINE('',#72761,#8113);
#3586=LINE('',#72764,#8114);
#3587=LINE('',#72771,#8115);
#3588=LINE('',#72774,#8116);
#3589=LINE('',#72781,#8117);
#3590=LINE('',#72784,#8118);
#3591=LINE('',#72791,#8119);
#3592=LINE('',#72794,#8120);
#3593=LINE('',#72801,#8121);
#3594=LINE('',#72804,#8122);
#3595=LINE('',#72811,#8123);
#3596=LINE('',#72814,#8124);
#3597=LINE('',#72821,#8125);
#3598=LINE('',#72824,#8126);
#3599=LINE('',#72830,#8127);
#3600=LINE('',#72831,#8128);
#3601=LINE('',#72834,#8129);
#3602=LINE('',#72835,#8130);
#3603=LINE('',#72838,#8131);
#3604=LINE('',#72839,#8132);
#3605=LINE('',#72842,#8133);
#3606=LINE('',#72843,#8134);
#3607=LINE('',#72846,#8135);
#3608=LINE('',#72847,#8136);
#3609=LINE('',#72850,#8137);
#3610=LINE('',#72851,#8138);
#3611=LINE('',#72854,#8139);
#3612=LINE('',#72855,#8140);
#3613=LINE('',#72858,#8141);
#3614=LINE('',#72859,#8142);
#3615=LINE('',#72862,#8143);
#3616=LINE('',#72863,#8144);
#3617=LINE('',#72866,#8145);
#3618=LINE('',#72867,#8146);
#3619=LINE('',#72870,#8147);
#3620=LINE('',#72871,#8148);
#3621=LINE('',#72874,#8149);
#3622=LINE('',#72875,#8150);
#3623=LINE('',#72878,#8151);
#3624=LINE('',#72879,#8152);
#3625=LINE('',#72882,#8153);
#3626=LINE('',#72883,#8154);
#3627=LINE('',#72886,#8155);
#3628=LINE('',#72887,#8156);
#3629=LINE('',#72890,#8157);
#3630=LINE('',#72891,#8158);
#3631=LINE('',#72894,#8159);
#3632=LINE('',#72895,#8160);
#3633=LINE('',#72898,#8161);
#3634=LINE('',#72899,#8162);
#3635=LINE('',#72902,#8163);
#3636=LINE('',#72903,#8164);
#3637=LINE('',#72906,#8165);
#3638=LINE('',#72907,#8166);
#3639=LINE('',#72910,#8167);
#3640=LINE('',#72911,#8168);
#3641=LINE('',#72914,#8169);
#3642=LINE('',#72915,#8170);
#3643=LINE('',#72918,#8171);
#3644=LINE('',#72919,#8172);
#3645=LINE('',#72922,#8173);
#3646=LINE('',#72923,#8174);
#3647=LINE('',#72926,#8175);
#3648=LINE('',#72927,#8176);
#3649=LINE('',#72930,#8177);
#3650=LINE('',#72931,#8178);
#3651=LINE('',#72934,#8179);
#3652=LINE('',#72935,#8180);
#3653=LINE('',#72938,#8181);
#3654=LINE('',#72939,#8182);
#3655=LINE('',#72942,#8183);
#3656=LINE('',#72943,#8184);
#3657=LINE('',#72946,#8185);
#3658=LINE('',#72947,#8186);
#3659=LINE('',#72950,#8187);
#3660=LINE('',#72951,#8188);
#3661=LINE('',#72954,#8189);
#3662=LINE('',#72955,#8190);
#3663=LINE('',#72958,#8191);
#3664=LINE('',#72959,#8192);
#3665=LINE('',#72962,#8193);
#3666=LINE('',#72963,#8194);
#3667=LINE('',#72966,#8195);
#3668=LINE('',#72967,#8196);
#3669=LINE('',#72970,#8197);
#3670=LINE('',#72971,#8198);
#3671=LINE('',#72974,#8199);
#3672=LINE('',#72980,#8200);
#3673=LINE('',#72986,#8201);
#3674=LINE('',#72992,#8202);
#3675=LINE('',#72998,#8203);
#3676=LINE('',#73004,#8204);
#3677=LINE('',#73010,#8205);
#3678=LINE('',#73016,#8206);
#3679=LINE('',#73022,#8207);
#3680=LINE('',#73028,#8208);
#3681=LINE('',#73034,#8209);
#3682=LINE('',#73040,#8210);
#3683=LINE('',#73046,#8211);
#3684=LINE('',#73052,#8212);
#3685=LINE('',#73058,#8213);
#3686=LINE('',#73064,#8214);
#3687=LINE('',#73070,#8215);
#3688=LINE('',#73076,#8216);
#3689=LINE('',#73086,#8217);
#3690=LINE('',#73092,#8218);
#3691=LINE('',#73098,#8219);
#3692=LINE('',#73104,#8220);
#3693=LINE('',#73110,#8221);
#3694=LINE('',#73116,#8222);
#3695=LINE('',#73122,#8223);
#3696=LINE('',#73128,#8224);
#3697=LINE('',#73134,#8225);
#3698=LINE('',#73140,#8226);
#3699=LINE('',#73146,#8227);
#3700=LINE('',#73152,#8228);
#3701=LINE('',#73158,#8229);
#3702=LINE('',#73164,#8230);
#3703=LINE('',#73170,#8231);
#3704=LINE('',#73176,#8232);
#3705=LINE('',#73182,#8233);
#3706=LINE('',#73188,#8234);
#3707=LINE('',#73194,#8235);
#3708=LINE('',#73195,#8236);
#3709=LINE('',#73199,#8237);
#3710=LINE('',#73203,#8238);
#3711=LINE('',#73207,#8239);
#3712=LINE('',#73211,#8240);
#3713=LINE('',#73215,#8241);
#3714=LINE('',#73218,#8242);
#3715=LINE('',#73219,#8243);
#3716=LINE('',#73223,#8244);
#3717=LINE('',#73227,#8245);
#3718=LINE('',#73231,#8246);
#3719=LINE('',#73235,#8247);
#3720=LINE('',#73239,#8248);
#3721=LINE('',#73242,#8249);
#3722=LINE('',#73243,#8250);
#3723=LINE('',#73252,#8251);
#3724=LINE('',#73253,#8252);
#3725=LINE('',#73257,#8253);
#3726=LINE('',#73261,#8254);
#3727=LINE('',#73265,#8255);
#3728=LINE('',#73269,#8256);
#3729=LINE('',#73273,#8257);
#3730=LINE('',#73276,#8258);
#3731=LINE('',#73277,#8259);
#3732=LINE('',#73281,#8260);
#3733=LINE('',#73285,#8261);
#3734=LINE('',#73289,#8262);
#3735=LINE('',#73293,#8263);
#3736=LINE('',#73297,#8264);
#3737=LINE('',#73299,#8265);
#3738=LINE('',#73308,#8266);
#3739=LINE('',#73460,#8267);
#3740=LINE('',#73472,#8268);
#3741=LINE('',#73483,#8269);
#3742=LINE('',#73485,#8270);
#3743=LINE('',#73487,#8271);
#3744=LINE('',#73489,#8272);
#3745=LINE('',#73491,#8273);
#3746=LINE('',#73493,#8274);
#3747=LINE('',#73495,#8275);
#3748=LINE('',#73497,#8276);
#3749=LINE('',#73499,#8277);
#3750=LINE('',#73501,#8278);
#3751=LINE('',#73503,#8279);
#3752=LINE('',#73505,#8280);
#3753=LINE('',#73507,#8281);
#3754=LINE('',#73509,#8282);
#3755=LINE('',#73516,#8283);
#3756=LINE('',#73517,#8284);
#3757=LINE('',#73521,#8285);
#3758=LINE('',#73525,#8286);
#3759=LINE('',#73529,#8287);
#3760=LINE('',#73533,#8288);
#3761=LINE('',#73537,#8289);
#3762=LINE('',#73540,#8290);
#3763=LINE('',#73541,#8291);
#3764=LINE('',#73545,#8292);
#3765=LINE('',#73549,#8293);
#3766=LINE('',#73553,#8294);
#3767=LINE('',#73557,#8295);
#3768=LINE('',#73561,#8296);
#3769=LINE('',#73563,#8297);
#3770=LINE('',#73571,#8298);
#3771=LINE('',#73583,#8299);
#3772=LINE('',#73594,#8300);
#3773=LINE('',#73596,#8301);
#3774=LINE('',#73598,#8302);
#3775=LINE('',#73600,#8303);
#3776=LINE('',#73602,#8304);
#3777=LINE('',#73604,#8305);
#3778=LINE('',#73606,#8306);
#3779=LINE('',#73608,#8307);
#3780=LINE('',#73610,#8308);
#3781=LINE('',#73612,#8309);
#3782=LINE('',#73614,#8310);
#3783=LINE('',#73616,#8311);
#3784=LINE('',#73618,#8312);
#3785=LINE('',#73620,#8313);
#3786=LINE('',#73627,#8314);
#3787=LINE('',#73628,#8315);
#3788=LINE('',#73632,#8316);
#3789=LINE('',#73636,#8317);
#3790=LINE('',#73640,#8318);
#3791=LINE('',#73644,#8319);
#3792=LINE('',#73648,#8320);
#3793=LINE('',#73651,#8321);
#3794=LINE('',#73652,#8322);
#3795=LINE('',#73656,#8323);
#3796=LINE('',#73660,#8324);
#3797=LINE('',#73664,#8325);
#3798=LINE('',#73668,#8326);
#3799=LINE('',#73672,#8327);
#3800=LINE('',#73674,#8328);
#3801=LINE('',#73682,#8329);
#3802=LINE('',#73694,#8330);
#3803=LINE('',#73705,#8331);
#3804=LINE('',#73707,#8332);
#3805=LINE('',#73709,#8333);
#3806=LINE('',#73711,#8334);
#3807=LINE('',#73713,#8335);
#3808=LINE('',#73715,#8336);
#3809=LINE('',#73717,#8337);
#3810=LINE('',#73719,#8338);
#3811=LINE('',#73721,#8339);
#3812=LINE('',#73723,#8340);
#3813=LINE('',#73725,#8341);
#3814=LINE('',#73727,#8342);
#3815=LINE('',#73729,#8343);
#3816=LINE('',#73731,#8344);
#3817=LINE('',#73738,#8345);
#3818=LINE('',#73739,#8346);
#3819=LINE('',#73743,#8347);
#3820=LINE('',#73747,#8348);
#3821=LINE('',#73751,#8349);
#3822=LINE('',#73755,#8350);
#3823=LINE('',#73759,#8351);
#3824=LINE('',#73762,#8352);
#3825=LINE('',#73763,#8353);
#3826=LINE('',#73767,#8354);
#3827=LINE('',#73771,#8355);
#3828=LINE('',#73775,#8356);
#3829=LINE('',#73779,#8357);
#3830=LINE('',#73783,#8358);
#3831=LINE('',#73785,#8359);
#3832=LINE('',#73793,#8360);
#3833=LINE('',#73805,#8361);
#3834=LINE('',#73816,#8362);
#3835=LINE('',#73818,#8363);
#3836=LINE('',#73820,#8364);
#3837=LINE('',#73822,#8365);
#3838=LINE('',#73824,#8366);
#3839=LINE('',#73826,#8367);
#3840=LINE('',#73828,#8368);
#3841=LINE('',#73830,#8369);
#3842=LINE('',#73832,#8370);
#3843=LINE('',#73834,#8371);
#3844=LINE('',#73836,#8372);
#3845=LINE('',#73838,#8373);
#3846=LINE('',#73840,#8374);
#3847=LINE('',#73842,#8375);
#3848=LINE('',#73849,#8376);
#3849=LINE('',#73850,#8377);
#3850=LINE('',#73854,#8378);
#3851=LINE('',#73858,#8379);
#3852=LINE('',#73862,#8380);
#3853=LINE('',#73866,#8381);
#3854=LINE('',#73870,#8382);
#3855=LINE('',#73873,#8383);
#3856=LINE('',#73874,#8384);
#3857=LINE('',#73878,#8385);
#3858=LINE('',#73882,#8386);
#3859=LINE('',#73886,#8387);
#3860=LINE('',#73890,#8388);
#3861=LINE('',#73894,#8389);
#3862=LINE('',#73896,#8390);
#3863=LINE('',#73904,#8391);
#3864=LINE('',#73916,#8392);
#3865=LINE('',#73927,#8393);
#3866=LINE('',#73929,#8394);
#3867=LINE('',#73931,#8395);
#3868=LINE('',#73933,#8396);
#3869=LINE('',#73935,#8397);
#3870=LINE('',#73937,#8398);
#3871=LINE('',#73939,#8399);
#3872=LINE('',#73941,#8400);
#3873=LINE('',#73943,#8401);
#3874=LINE('',#73945,#8402);
#3875=LINE('',#73947,#8403);
#3876=LINE('',#73949,#8404);
#3877=LINE('',#73951,#8405);
#3878=LINE('',#73953,#8406);
#3879=LINE('',#73960,#8407);
#3880=LINE('',#73961,#8408);
#3881=LINE('',#73965,#8409);
#3882=LINE('',#73969,#8410);
#3883=LINE('',#73973,#8411);
#3884=LINE('',#73977,#8412);
#3885=LINE('',#73981,#8413);
#3886=LINE('',#73984,#8414);
#3887=LINE('',#73985,#8415);
#3888=LINE('',#73989,#8416);
#3889=LINE('',#73993,#8417);
#3890=LINE('',#73997,#8418);
#3891=LINE('',#74001,#8419);
#3892=LINE('',#74005,#8420);
#3893=LINE('',#74007,#8421);
#3894=LINE('',#74015,#8422);
#3895=LINE('',#74027,#8423);
#3896=LINE('',#74038,#8424);
#3897=LINE('',#74040,#8425);
#3898=LINE('',#74042,#8426);
#3899=LINE('',#74044,#8427);
#3900=LINE('',#74046,#8428);
#3901=LINE('',#74048,#8429);
#3902=LINE('',#74050,#8430);
#3903=LINE('',#74052,#8431);
#3904=LINE('',#74054,#8432);
#3905=LINE('',#74056,#8433);
#3906=LINE('',#74058,#8434);
#3907=LINE('',#74060,#8435);
#3908=LINE('',#74062,#8436);
#3909=LINE('',#74064,#8437);
#3910=LINE('',#74071,#8438);
#3911=LINE('',#74072,#8439);
#3912=LINE('',#74076,#8440);
#3913=LINE('',#74080,#8441);
#3914=LINE('',#74084,#8442);
#3915=LINE('',#74088,#8443);
#3916=LINE('',#74092,#8444);
#3917=LINE('',#74095,#8445);
#3918=LINE('',#74096,#8446);
#3919=LINE('',#74100,#8447);
#3920=LINE('',#74104,#8448);
#3921=LINE('',#74108,#8449);
#3922=LINE('',#74112,#8450);
#3923=LINE('',#74116,#8451);
#3924=LINE('',#74118,#8452);
#3925=LINE('',#74126,#8453);
#3926=LINE('',#74138,#8454);
#3927=LINE('',#74149,#8455);
#3928=LINE('',#74151,#8456);
#3929=LINE('',#74153,#8457);
#3930=LINE('',#74155,#8458);
#3931=LINE('',#74157,#8459);
#3932=LINE('',#74159,#8460);
#3933=LINE('',#74161,#8461);
#3934=LINE('',#74163,#8462);
#3935=LINE('',#74165,#8463);
#3936=LINE('',#74167,#8464);
#3937=LINE('',#74169,#8465);
#3938=LINE('',#74171,#8466);
#3939=LINE('',#74173,#8467);
#3940=LINE('',#74175,#8468);
#3941=LINE('',#74182,#8469);
#3942=LINE('',#74183,#8470);
#3943=LINE('',#74187,#8471);
#3944=LINE('',#74191,#8472);
#3945=LINE('',#74195,#8473);
#3946=LINE('',#74199,#8474);
#3947=LINE('',#74203,#8475);
#3948=LINE('',#74206,#8476);
#3949=LINE('',#74207,#8477);
#3950=LINE('',#74211,#8478);
#3951=LINE('',#74215,#8479);
#3952=LINE('',#74219,#8480);
#3953=LINE('',#74223,#8481);
#3954=LINE('',#74227,#8482);
#3955=LINE('',#74229,#8483);
#3956=LINE('',#74237,#8484);
#3957=LINE('',#74249,#8485);
#3958=LINE('',#74260,#8486);
#3959=LINE('',#74262,#8487);
#3960=LINE('',#74264,#8488);
#3961=LINE('',#74266,#8489);
#3962=LINE('',#74268,#8490);
#3963=LINE('',#74270,#8491);
#3964=LINE('',#74272,#8492);
#3965=LINE('',#74274,#8493);
#3966=LINE('',#74276,#8494);
#3967=LINE('',#74278,#8495);
#3968=LINE('',#74280,#8496);
#3969=LINE('',#74282,#8497);
#3970=LINE('',#74284,#8498);
#3971=LINE('',#74286,#8499);
#3972=LINE('',#74293,#8500);
#3973=LINE('',#74294,#8501);
#3974=LINE('',#74298,#8502);
#3975=LINE('',#74302,#8503);
#3976=LINE('',#74306,#8504);
#3977=LINE('',#74310,#8505);
#3978=LINE('',#74314,#8506);
#3979=LINE('',#74317,#8507);
#3980=LINE('',#74318,#8508);
#3981=LINE('',#74322,#8509);
#3982=LINE('',#74326,#8510);
#3983=LINE('',#74330,#8511);
#3984=LINE('',#74334,#8512);
#3985=LINE('',#74338,#8513);
#3986=LINE('',#74340,#8514);
#3987=LINE('',#74348,#8515);
#3988=LINE('',#74360,#8516);
#3989=LINE('',#74371,#8517);
#3990=LINE('',#74373,#8518);
#3991=LINE('',#74375,#8519);
#3992=LINE('',#74377,#8520);
#3993=LINE('',#74379,#8521);
#3994=LINE('',#74381,#8522);
#3995=LINE('',#74383,#8523);
#3996=LINE('',#74385,#8524);
#3997=LINE('',#74387,#8525);
#3998=LINE('',#74389,#8526);
#3999=LINE('',#74391,#8527);
#4000=LINE('',#74393,#8528);
#4001=LINE('',#74395,#8529);
#4002=LINE('',#74397,#8530);
#4003=LINE('',#74404,#8531);
#4004=LINE('',#74405,#8532);
#4005=LINE('',#74409,#8533);
#4006=LINE('',#74413,#8534);
#4007=LINE('',#74417,#8535);
#4008=LINE('',#74421,#8536);
#4009=LINE('',#74425,#8537);
#4010=LINE('',#74428,#8538);
#4011=LINE('',#74429,#8539);
#4012=LINE('',#74433,#8540);
#4013=LINE('',#74437,#8541);
#4014=LINE('',#74441,#8542);
#4015=LINE('',#74445,#8543);
#4016=LINE('',#74449,#8544);
#4017=LINE('',#74451,#8545);
#4018=LINE('',#74459,#8546);
#4019=LINE('',#74471,#8547);
#4020=LINE('',#74482,#8548);
#4021=LINE('',#74484,#8549);
#4022=LINE('',#74486,#8550);
#4023=LINE('',#74488,#8551);
#4024=LINE('',#74490,#8552);
#4025=LINE('',#74492,#8553);
#4026=LINE('',#74494,#8554);
#4027=LINE('',#74496,#8555);
#4028=LINE('',#74498,#8556);
#4029=LINE('',#74500,#8557);
#4030=LINE('',#74502,#8558);
#4031=LINE('',#74504,#8559);
#4032=LINE('',#74506,#8560);
#4033=LINE('',#74508,#8561);
#4034=LINE('',#74515,#8562);
#4035=LINE('',#74516,#8563);
#4036=LINE('',#74520,#8564);
#4037=LINE('',#74524,#8565);
#4038=LINE('',#74528,#8566);
#4039=LINE('',#74532,#8567);
#4040=LINE('',#74536,#8568);
#4041=LINE('',#74539,#8569);
#4042=LINE('',#74540,#8570);
#4043=LINE('',#74544,#8571);
#4044=LINE('',#74548,#8572);
#4045=LINE('',#74552,#8573);
#4046=LINE('',#74556,#8574);
#4047=LINE('',#74560,#8575);
#4048=LINE('',#74562,#8576);
#4049=LINE('',#74570,#8577);
#4050=LINE('',#74582,#8578);
#4051=LINE('',#74593,#8579);
#4052=LINE('',#74595,#8580);
#4053=LINE('',#74597,#8581);
#4054=LINE('',#74599,#8582);
#4055=LINE('',#74601,#8583);
#4056=LINE('',#74603,#8584);
#4057=LINE('',#74605,#8585);
#4058=LINE('',#74607,#8586);
#4059=LINE('',#74609,#8587);
#4060=LINE('',#74611,#8588);
#4061=LINE('',#74613,#8589);
#4062=LINE('',#74615,#8590);
#4063=LINE('',#74617,#8591);
#4064=LINE('',#74619,#8592);
#4065=LINE('',#74626,#8593);
#4066=LINE('',#74627,#8594);
#4067=LINE('',#74631,#8595);
#4068=LINE('',#74635,#8596);
#4069=LINE('',#74639,#8597);
#4070=LINE('',#74643,#8598);
#4071=LINE('',#74647,#8599);
#4072=LINE('',#74650,#8600);
#4073=LINE('',#74651,#8601);
#4074=LINE('',#74655,#8602);
#4075=LINE('',#74659,#8603);
#4076=LINE('',#74663,#8604);
#4077=LINE('',#74667,#8605);
#4078=LINE('',#74671,#8606);
#4079=LINE('',#74673,#8607);
#4080=LINE('',#74681,#8608);
#4081=LINE('',#74693,#8609);
#4082=LINE('',#74704,#8610);
#4083=LINE('',#74706,#8611);
#4084=LINE('',#74708,#8612);
#4085=LINE('',#74710,#8613);
#4086=LINE('',#74712,#8614);
#4087=LINE('',#74714,#8615);
#4088=LINE('',#74716,#8616);
#4089=LINE('',#74718,#8617);
#4090=LINE('',#74720,#8618);
#4091=LINE('',#74722,#8619);
#4092=LINE('',#74724,#8620);
#4093=LINE('',#74726,#8621);
#4094=LINE('',#74728,#8622);
#4095=LINE('',#74730,#8623);
#4096=LINE('',#74737,#8624);
#4097=LINE('',#74738,#8625);
#4098=LINE('',#74742,#8626);
#4099=LINE('',#74746,#8627);
#4100=LINE('',#74750,#8628);
#4101=LINE('',#74754,#8629);
#4102=LINE('',#74758,#8630);
#4103=LINE('',#74761,#8631);
#4104=LINE('',#74762,#8632);
#4105=LINE('',#74766,#8633);
#4106=LINE('',#74770,#8634);
#4107=LINE('',#74774,#8635);
#4108=LINE('',#74778,#8636);
#4109=LINE('',#74782,#8637);
#4110=LINE('',#74784,#8638);
#4111=LINE('',#74792,#8639);
#4112=LINE('',#74804,#8640);
#4113=LINE('',#74815,#8641);
#4114=LINE('',#74817,#8642);
#4115=LINE('',#74819,#8643);
#4116=LINE('',#74821,#8644);
#4117=LINE('',#74823,#8645);
#4118=LINE('',#74825,#8646);
#4119=LINE('',#74827,#8647);
#4120=LINE('',#74829,#8648);
#4121=LINE('',#74831,#8649);
#4122=LINE('',#74833,#8650);
#4123=LINE('',#74835,#8651);
#4124=LINE('',#74837,#8652);
#4125=LINE('',#74839,#8653);
#4126=LINE('',#74841,#8654);
#4127=LINE('',#74848,#8655);
#4128=LINE('',#74849,#8656);
#4129=LINE('',#74853,#8657);
#4130=LINE('',#74857,#8658);
#4131=LINE('',#74861,#8659);
#4132=LINE('',#74865,#8660);
#4133=LINE('',#74869,#8661);
#4134=LINE('',#74872,#8662);
#4135=LINE('',#74873,#8663);
#4136=LINE('',#74877,#8664);
#4137=LINE('',#74881,#8665);
#4138=LINE('',#74885,#8666);
#4139=LINE('',#74889,#8667);
#4140=LINE('',#74893,#8668);
#4141=LINE('',#74895,#8669);
#4142=LINE('',#74903,#8670);
#4143=LINE('',#74915,#8671);
#4144=LINE('',#74926,#8672);
#4145=LINE('',#74928,#8673);
#4146=LINE('',#74930,#8674);
#4147=LINE('',#74932,#8675);
#4148=LINE('',#74934,#8676);
#4149=LINE('',#74936,#8677);
#4150=LINE('',#74938,#8678);
#4151=LINE('',#74940,#8679);
#4152=LINE('',#74942,#8680);
#4153=LINE('',#74944,#8681);
#4154=LINE('',#74946,#8682);
#4155=LINE('',#74948,#8683);
#4156=LINE('',#74950,#8684);
#4157=LINE('',#74952,#8685);
#4158=LINE('',#74959,#8686);
#4159=LINE('',#74960,#8687);
#4160=LINE('',#74964,#8688);
#4161=LINE('',#74968,#8689);
#4162=LINE('',#74972,#8690);
#4163=LINE('',#74976,#8691);
#4164=LINE('',#74980,#8692);
#4165=LINE('',#74983,#8693);
#4166=LINE('',#74984,#8694);
#4167=LINE('',#74988,#8695);
#4168=LINE('',#74992,#8696);
#4169=LINE('',#74996,#8697);
#4170=LINE('',#75000,#8698);
#4171=LINE('',#75004,#8699);
#4172=LINE('',#75006,#8700);
#4173=LINE('',#75014,#8701);
#4174=LINE('',#75026,#8702);
#4175=LINE('',#75037,#8703);
#4176=LINE('',#75039,#8704);
#4177=LINE('',#75041,#8705);
#4178=LINE('',#75043,#8706);
#4179=LINE('',#75045,#8707);
#4180=LINE('',#75047,#8708);
#4181=LINE('',#75049,#8709);
#4182=LINE('',#75051,#8710);
#4183=LINE('',#75053,#8711);
#4184=LINE('',#75055,#8712);
#4185=LINE('',#75057,#8713);
#4186=LINE('',#75059,#8714);
#4187=LINE('',#75061,#8715);
#4188=LINE('',#75063,#8716);
#4189=LINE('',#75070,#8717);
#4190=LINE('',#75071,#8718);
#4191=LINE('',#75075,#8719);
#4192=LINE('',#75079,#8720);
#4193=LINE('',#75083,#8721);
#4194=LINE('',#75087,#8722);
#4195=LINE('',#75091,#8723);
#4196=LINE('',#75094,#8724);
#4197=LINE('',#75095,#8725);
#4198=LINE('',#75099,#8726);
#4199=LINE('',#75103,#8727);
#4200=LINE('',#75107,#8728);
#4201=LINE('',#75111,#8729);
#4202=LINE('',#75115,#8730);
#4203=LINE('',#75117,#8731);
#4204=LINE('',#75125,#8732);
#4205=LINE('',#75137,#8733);
#4206=LINE('',#75148,#8734);
#4207=LINE('',#75150,#8735);
#4208=LINE('',#75152,#8736);
#4209=LINE('',#75154,#8737);
#4210=LINE('',#75156,#8738);
#4211=LINE('',#75158,#8739);
#4212=LINE('',#75160,#8740);
#4213=LINE('',#75162,#8741);
#4214=LINE('',#75164,#8742);
#4215=LINE('',#75166,#8743);
#4216=LINE('',#75168,#8744);
#4217=LINE('',#75170,#8745);
#4218=LINE('',#75172,#8746);
#4219=LINE('',#75174,#8747);
#4220=LINE('',#75181,#8748);
#4221=LINE('',#75182,#8749);
#4222=LINE('',#75186,#8750);
#4223=LINE('',#75190,#8751);
#4224=LINE('',#75194,#8752);
#4225=LINE('',#75198,#8753);
#4226=LINE('',#75202,#8754);
#4227=LINE('',#75205,#8755);
#4228=LINE('',#75206,#8756);
#4229=LINE('',#75210,#8757);
#4230=LINE('',#75214,#8758);
#4231=LINE('',#75218,#8759);
#4232=LINE('',#75222,#8760);
#4233=LINE('',#75226,#8761);
#4234=LINE('',#75228,#8762);
#4235=LINE('',#75236,#8763);
#4236=LINE('',#75248,#8764);
#4237=LINE('',#75259,#8765);
#4238=LINE('',#75261,#8766);
#4239=LINE('',#75263,#8767);
#4240=LINE('',#75265,#8768);
#4241=LINE('',#75267,#8769);
#4242=LINE('',#75269,#8770);
#4243=LINE('',#75271,#8771);
#4244=LINE('',#75273,#8772);
#4245=LINE('',#75275,#8773);
#4246=LINE('',#75277,#8774);
#4247=LINE('',#75279,#8775);
#4248=LINE('',#75281,#8776);
#4249=LINE('',#75283,#8777);
#4250=LINE('',#75285,#8778);
#4251=LINE('',#75292,#8779);
#4252=LINE('',#75293,#8780);
#4253=LINE('',#75297,#8781);
#4254=LINE('',#75301,#8782);
#4255=LINE('',#75305,#8783);
#4256=LINE('',#75309,#8784);
#4257=LINE('',#75313,#8785);
#4258=LINE('',#75316,#8786);
#4259=LINE('',#75317,#8787);
#4260=LINE('',#75321,#8788);
#4261=LINE('',#75325,#8789);
#4262=LINE('',#75329,#8790);
#4263=LINE('',#75333,#8791);
#4264=LINE('',#75337,#8792);
#4265=LINE('',#75339,#8793);
#4266=LINE('',#75347,#8794);
#4267=LINE('',#75359,#8795);
#4268=LINE('',#75370,#8796);
#4269=LINE('',#75372,#8797);
#4270=LINE('',#75374,#8798);
#4271=LINE('',#75376,#8799);
#4272=LINE('',#75378,#8800);
#4273=LINE('',#75380,#8801);
#4274=LINE('',#75382,#8802);
#4275=LINE('',#75384,#8803);
#4276=LINE('',#75386,#8804);
#4277=LINE('',#75388,#8805);
#4278=LINE('',#75390,#8806);
#4279=LINE('',#75392,#8807);
#4280=LINE('',#75394,#8808);
#4281=LINE('',#75396,#8809);
#4282=LINE('',#75403,#8810);
#4283=LINE('',#75404,#8811);
#4284=LINE('',#75408,#8812);
#4285=LINE('',#75412,#8813);
#4286=LINE('',#75416,#8814);
#4287=LINE('',#75420,#8815);
#4288=LINE('',#75424,#8816);
#4289=LINE('',#75427,#8817);
#4290=LINE('',#75428,#8818);
#4291=LINE('',#75432,#8819);
#4292=LINE('',#75436,#8820);
#4293=LINE('',#75440,#8821);
#4294=LINE('',#75444,#8822);
#4295=LINE('',#75448,#8823);
#4296=LINE('',#75450,#8824);
#4297=LINE('',#75458,#8825);
#4298=LINE('',#75470,#8826);
#4299=LINE('',#75481,#8827);
#4300=LINE('',#75483,#8828);
#4301=LINE('',#75485,#8829);
#4302=LINE('',#75487,#8830);
#4303=LINE('',#75489,#8831);
#4304=LINE('',#75491,#8832);
#4305=LINE('',#75493,#8833);
#4306=LINE('',#75495,#8834);
#4307=LINE('',#75497,#8835);
#4308=LINE('',#75499,#8836);
#4309=LINE('',#75501,#8837);
#4310=LINE('',#75503,#8838);
#4311=LINE('',#75505,#8839);
#4312=LINE('',#75507,#8840);
#4313=LINE('',#75514,#8841);
#4314=LINE('',#75515,#8842);
#4315=LINE('',#75519,#8843);
#4316=LINE('',#75523,#8844);
#4317=LINE('',#75527,#8845);
#4318=LINE('',#75531,#8846);
#4319=LINE('',#75535,#8847);
#4320=LINE('',#75538,#8848);
#4321=LINE('',#75539,#8849);
#4322=LINE('',#75543,#8850);
#4323=LINE('',#75547,#8851);
#4324=LINE('',#75551,#8852);
#4325=LINE('',#75555,#8853);
#4326=LINE('',#75559,#8854);
#4327=LINE('',#75561,#8855);
#4328=LINE('',#75569,#8856);
#4329=LINE('',#75581,#8857);
#4330=LINE('',#75592,#8858);
#4331=LINE('',#75594,#8859);
#4332=LINE('',#75596,#8860);
#4333=LINE('',#75598,#8861);
#4334=LINE('',#75600,#8862);
#4335=LINE('',#75602,#8863);
#4336=LINE('',#75604,#8864);
#4337=LINE('',#75606,#8865);
#4338=LINE('',#75608,#8866);
#4339=LINE('',#75610,#8867);
#4340=LINE('',#75612,#8868);
#4341=LINE('',#75614,#8869);
#4342=LINE('',#75616,#8870);
#4343=LINE('',#75618,#8871);
#4344=LINE('',#75625,#8872);
#4345=LINE('',#75626,#8873);
#4346=LINE('',#75630,#8874);
#4347=LINE('',#75634,#8875);
#4348=LINE('',#75638,#8876);
#4349=LINE('',#75642,#8877);
#4350=LINE('',#75646,#8878);
#4351=LINE('',#75649,#8879);
#4352=LINE('',#75650,#8880);
#4353=LINE('',#75654,#8881);
#4354=LINE('',#75658,#8882);
#4355=LINE('',#75662,#8883);
#4356=LINE('',#75666,#8884);
#4357=LINE('',#75670,#8885);
#4358=LINE('',#75672,#8886);
#4359=LINE('',#75680,#8887);
#4360=LINE('',#75692,#8888);
#4361=LINE('',#75703,#8889);
#4362=LINE('',#75705,#8890);
#4363=LINE('',#75707,#8891);
#4364=LINE('',#75709,#8892);
#4365=LINE('',#75711,#8893);
#4366=LINE('',#75713,#8894);
#4367=LINE('',#75715,#8895);
#4368=LINE('',#75717,#8896);
#4369=LINE('',#75719,#8897);
#4370=LINE('',#75721,#8898);
#4371=LINE('',#75723,#8899);
#4372=LINE('',#75725,#8900);
#4373=LINE('',#75727,#8901);
#4374=LINE('',#75729,#8902);
#4375=LINE('',#75736,#8903);
#4376=LINE('',#75737,#8904);
#4377=LINE('',#75741,#8905);
#4378=LINE('',#75745,#8906);
#4379=LINE('',#75749,#8907);
#4380=LINE('',#75753,#8908);
#4381=LINE('',#75757,#8909);
#4382=LINE('',#75760,#8910);
#4383=LINE('',#75761,#8911);
#4384=LINE('',#75765,#8912);
#4385=LINE('',#75769,#8913);
#4386=LINE('',#75773,#8914);
#4387=LINE('',#75777,#8915);
#4388=LINE('',#75781,#8916);
#4389=LINE('',#75783,#8917);
#4390=LINE('',#75791,#8918);
#4391=LINE('',#75803,#8919);
#4392=LINE('',#75814,#8920);
#4393=LINE('',#75816,#8921);
#4394=LINE('',#75818,#8922);
#4395=LINE('',#75820,#8923);
#4396=LINE('',#75822,#8924);
#4397=LINE('',#75824,#8925);
#4398=LINE('',#75826,#8926);
#4399=LINE('',#75828,#8927);
#4400=LINE('',#75830,#8928);
#4401=LINE('',#75832,#8929);
#4402=LINE('',#75834,#8930);
#4403=LINE('',#75836,#8931);
#4404=LINE('',#75838,#8932);
#4405=LINE('',#75840,#8933);
#4406=LINE('',#75847,#8934);
#4407=LINE('',#75848,#8935);
#4408=LINE('',#75852,#8936);
#4409=LINE('',#75856,#8937);
#4410=LINE('',#75860,#8938);
#4411=LINE('',#75864,#8939);
#4412=LINE('',#75868,#8940);
#4413=LINE('',#75871,#8941);
#4414=LINE('',#75872,#8942);
#4415=LINE('',#75876,#8943);
#4416=LINE('',#75880,#8944);
#4417=LINE('',#75884,#8945);
#4418=LINE('',#75888,#8946);
#4419=LINE('',#75892,#8947);
#4420=LINE('',#75894,#8948);
#4421=LINE('',#75902,#8949);
#4422=LINE('',#75914,#8950);
#4423=LINE('',#75925,#8951);
#4424=LINE('',#75927,#8952);
#4425=LINE('',#75929,#8953);
#4426=LINE('',#75931,#8954);
#4427=LINE('',#75933,#8955);
#4428=LINE('',#75935,#8956);
#4429=LINE('',#75937,#8957);
#4430=LINE('',#75939,#8958);
#4431=LINE('',#75941,#8959);
#4432=LINE('',#75943,#8960);
#4433=LINE('',#75945,#8961);
#4434=LINE('',#75947,#8962);
#4435=LINE('',#75949,#8963);
#4436=LINE('',#75951,#8964);
#4437=LINE('',#75958,#8965);
#4438=LINE('',#75959,#8966);
#4439=LINE('',#75963,#8967);
#4440=LINE('',#75967,#8968);
#4441=LINE('',#75971,#8969);
#4442=LINE('',#75975,#8970);
#4443=LINE('',#75979,#8971);
#4444=LINE('',#75982,#8972);
#4445=LINE('',#75983,#8973);
#4446=LINE('',#75987,#8974);
#4447=LINE('',#75991,#8975);
#4448=LINE('',#75995,#8976);
#4449=LINE('',#75999,#8977);
#4450=LINE('',#76003,#8978);
#4451=LINE('',#76005,#8979);
#4452=LINE('',#76013,#8980);
#4453=LINE('',#76025,#8981);
#4454=LINE('',#76036,#8982);
#4455=LINE('',#76038,#8983);
#4456=LINE('',#76040,#8984);
#4457=LINE('',#76042,#8985);
#4458=LINE('',#76044,#8986);
#4459=LINE('',#76046,#8987);
#4460=LINE('',#76048,#8988);
#4461=LINE('',#76050,#8989);
#4462=LINE('',#76052,#8990);
#4463=LINE('',#76054,#8991);
#4464=LINE('',#76056,#8992);
#4465=LINE('',#76058,#8993);
#4466=LINE('',#76060,#8994);
#4467=LINE('',#76062,#8995);
#4468=LINE('',#76069,#8996);
#4469=LINE('',#76070,#8997);
#4470=LINE('',#76074,#8998);
#4471=LINE('',#76078,#8999);
#4472=LINE('',#76082,#9000);
#4473=LINE('',#76086,#9001);
#4474=LINE('',#76090,#9002);
#4475=LINE('',#76093,#9003);
#4476=LINE('',#76094,#9004);
#4477=LINE('',#76098,#9005);
#4478=LINE('',#76102,#9006);
#4479=LINE('',#76106,#9007);
#4480=LINE('',#76110,#9008);
#4481=LINE('',#76114,#9009);
#4482=LINE('',#76116,#9010);
#4483=LINE('',#76124,#9011);
#4484=LINE('',#76136,#9012);
#4485=LINE('',#76147,#9013);
#4486=LINE('',#76149,#9014);
#4487=LINE('',#76151,#9015);
#4488=LINE('',#76153,#9016);
#4489=LINE('',#76155,#9017);
#4490=LINE('',#76157,#9018);
#4491=LINE('',#76159,#9019);
#4492=LINE('',#76161,#9020);
#4493=LINE('',#76163,#9021);
#4494=LINE('',#76165,#9022);
#4495=LINE('',#76167,#9023);
#4496=LINE('',#76169,#9024);
#4497=LINE('',#76171,#9025);
#4498=LINE('',#76173,#9026);
#4499=LINE('',#76180,#9027);
#4500=LINE('',#76181,#9028);
#4501=LINE('',#76185,#9029);
#4502=LINE('',#76189,#9030);
#4503=LINE('',#76193,#9031);
#4504=LINE('',#76197,#9032);
#4505=LINE('',#76201,#9033);
#4506=LINE('',#76204,#9034);
#4507=LINE('',#76205,#9035);
#4508=LINE('',#76209,#9036);
#4509=LINE('',#76213,#9037);
#4510=LINE('',#76217,#9038);
#4511=LINE('',#76221,#9039);
#4512=LINE('',#76225,#9040);
#4513=LINE('',#76227,#9041);
#4514=LINE('',#76235,#9042);
#4515=LINE('',#76247,#9043);
#4516=LINE('',#76258,#9044);
#4517=LINE('',#76260,#9045);
#4518=LINE('',#76262,#9046);
#4519=LINE('',#76264,#9047);
#4520=LINE('',#76266,#9048);
#4521=LINE('',#76268,#9049);
#4522=LINE('',#76270,#9050);
#4523=LINE('',#76272,#9051);
#4524=LINE('',#76274,#9052);
#4525=LINE('',#76276,#9053);
#4526=LINE('',#76278,#9054);
#4527=LINE('',#76280,#9055);
#4528=LINE('',#76282,#9056);
#4529=LINE('',#76284,#9057);
#4530=LINE('',#76291,#9058);
#4531=LINE('',#76292,#9059);
#4532=LINE('',#76296,#9060);
#4533=LINE('',#76300,#9061);
#4534=LINE('',#76304,#9062);
#4535=LINE('',#76308,#9063);
#4536=LINE('',#76312,#9064);
#4537=LINE('',#76315,#9065);
#4538=LINE('',#76316,#9066);
#4539=LINE('',#76320,#9067);
#4540=LINE('',#76324,#9068);
#4541=LINE('',#76328,#9069);
#4542=LINE('',#76332,#9070);
#4543=LINE('',#76336,#9071);
#4544=LINE('',#76338,#9072);
#4545=LINE('',#76346,#9073);
#4546=LINE('',#76358,#9074);
#4547=LINE('',#76369,#9075);
#4548=LINE('',#76371,#9076);
#4549=LINE('',#76373,#9077);
#4550=LINE('',#76375,#9078);
#4551=LINE('',#76377,#9079);
#4552=LINE('',#76379,#9080);
#4553=LINE('',#76381,#9081);
#4554=LINE('',#76383,#9082);
#4555=LINE('',#76385,#9083);
#4556=LINE('',#76387,#9084);
#4557=LINE('',#76389,#9085);
#4558=LINE('',#76391,#9086);
#4559=LINE('',#76393,#9087);
#4560=LINE('',#76395,#9088);
#4561=LINE('',#76402,#9089);
#4562=LINE('',#76403,#9090);
#4563=LINE('',#76407,#9091);
#4564=LINE('',#76411,#9092);
#4565=LINE('',#76415,#9093);
#4566=LINE('',#76419,#9094);
#4567=LINE('',#76423,#9095);
#4568=LINE('',#76426,#9096);
#4569=LINE('',#76427,#9097);
#4570=LINE('',#76431,#9098);
#4571=LINE('',#76435,#9099);
#4572=LINE('',#76439,#9100);
#4573=LINE('',#76443,#9101);
#4574=LINE('',#76447,#9102);
#4575=LINE('',#76449,#9103);
#4576=LINE('',#76457,#9104);
#4577=LINE('',#76469,#9105);
#4578=LINE('',#76480,#9106);
#4579=LINE('',#76482,#9107);
#4580=LINE('',#76484,#9108);
#4581=LINE('',#76486,#9109);
#4582=LINE('',#76488,#9110);
#4583=LINE('',#76490,#9111);
#4584=LINE('',#76492,#9112);
#4585=LINE('',#76494,#9113);
#4586=LINE('',#76496,#9114);
#4587=LINE('',#76498,#9115);
#4588=LINE('',#76500,#9116);
#4589=LINE('',#76502,#9117);
#4590=LINE('',#76504,#9118);
#4591=LINE('',#76506,#9119);
#4592=LINE('',#76513,#9120);
#4593=LINE('',#76514,#9121);
#4594=LINE('',#76518,#9122);
#4595=LINE('',#76522,#9123);
#4596=LINE('',#76526,#9124);
#4597=LINE('',#76530,#9125);
#4598=LINE('',#76534,#9126);
#4599=LINE('',#76537,#9127);
#4600=LINE('',#76538,#9128);
#4601=LINE('',#76542,#9129);
#4602=LINE('',#76546,#9130);
#4603=LINE('',#76550,#9131);
#4604=LINE('',#76554,#9132);
#4605=LINE('',#76558,#9133);
#4606=LINE('',#76560,#9134);
#4607=LINE('',#76568,#9135);
#4608=LINE('',#76580,#9136);
#4609=LINE('',#76591,#9137);
#4610=LINE('',#76593,#9138);
#4611=LINE('',#76595,#9139);
#4612=LINE('',#76597,#9140);
#4613=LINE('',#76599,#9141);
#4614=LINE('',#76601,#9142);
#4615=LINE('',#76603,#9143);
#4616=LINE('',#76605,#9144);
#4617=LINE('',#76607,#9145);
#4618=LINE('',#76609,#9146);
#4619=LINE('',#76611,#9147);
#4620=LINE('',#76613,#9148);
#4621=LINE('',#76615,#9149);
#4622=LINE('',#76617,#9150);
#4623=LINE('',#76624,#9151);
#4624=LINE('',#76625,#9152);
#4625=LINE('',#76629,#9153);
#4626=LINE('',#76633,#9154);
#4627=LINE('',#76637,#9155);
#4628=LINE('',#76641,#9156);
#4629=LINE('',#76645,#9157);
#4630=LINE('',#76648,#9158);
#4631=LINE('',#76649,#9159);
#4632=LINE('',#76653,#9160);
#4633=LINE('',#76657,#9161);
#4634=LINE('',#76661,#9162);
#4635=LINE('',#76665,#9163);
#4636=LINE('',#76669,#9164);
#4637=LINE('',#76671,#9165);
#4638=LINE('',#76679,#9166);
#4639=LINE('',#76691,#9167);
#4640=LINE('',#76702,#9168);
#4641=LINE('',#76704,#9169);
#4642=LINE('',#76706,#9170);
#4643=LINE('',#76708,#9171);
#4644=LINE('',#76710,#9172);
#4645=LINE('',#76712,#9173);
#4646=LINE('',#76714,#9174);
#4647=LINE('',#76716,#9175);
#4648=LINE('',#76718,#9176);
#4649=LINE('',#76720,#9177);
#4650=LINE('',#76722,#9178);
#4651=LINE('',#76724,#9179);
#4652=LINE('',#76726,#9180);
#4653=LINE('',#76728,#9181);
#4654=LINE('',#76735,#9182);
#4655=LINE('',#76736,#9183);
#4656=LINE('',#76740,#9184);
#4657=LINE('',#76744,#9185);
#4658=LINE('',#76748,#9186);
#4659=LINE('',#76752,#9187);
#4660=LINE('',#76756,#9188);
#4661=LINE('',#76759,#9189);
#4662=LINE('',#76760,#9190);
#4663=LINE('',#76764,#9191);
#4664=LINE('',#76768,#9192);
#4665=LINE('',#76772,#9193);
#4666=LINE('',#76776,#9194);
#4667=LINE('',#76780,#9195);
#4668=LINE('',#76782,#9196);
#4669=LINE('',#76790,#9197);
#4670=LINE('',#76802,#9198);
#4671=LINE('',#76813,#9199);
#4672=LINE('',#76815,#9200);
#4673=LINE('',#76817,#9201);
#4674=LINE('',#76819,#9202);
#4675=LINE('',#76821,#9203);
#4676=LINE('',#76823,#9204);
#4677=LINE('',#76825,#9205);
#4678=LINE('',#76827,#9206);
#4679=LINE('',#76829,#9207);
#4680=LINE('',#76831,#9208);
#4681=LINE('',#76833,#9209);
#4682=LINE('',#76835,#9210);
#4683=LINE('',#76837,#9211);
#4684=LINE('',#76839,#9212);
#4685=LINE('',#76846,#9213);
#4686=LINE('',#76847,#9214);
#4687=LINE('',#76851,#9215);
#4688=LINE('',#76855,#9216);
#4689=LINE('',#76859,#9217);
#4690=LINE('',#76863,#9218);
#4691=LINE('',#76867,#9219);
#4692=LINE('',#76870,#9220);
#4693=LINE('',#76871,#9221);
#4694=LINE('',#76875,#9222);
#4695=LINE('',#76879,#9223);
#4696=LINE('',#76883,#9224);
#4697=LINE('',#76887,#9225);
#4698=LINE('',#76891,#9226);
#4699=LINE('',#76893,#9227);
#4700=LINE('',#76901,#9228);
#4701=LINE('',#76913,#9229);
#4702=LINE('',#76924,#9230);
#4703=LINE('',#76926,#9231);
#4704=LINE('',#76928,#9232);
#4705=LINE('',#76930,#9233);
#4706=LINE('',#76932,#9234);
#4707=LINE('',#76934,#9235);
#4708=LINE('',#76936,#9236);
#4709=LINE('',#76938,#9237);
#4710=LINE('',#76940,#9238);
#4711=LINE('',#76942,#9239);
#4712=LINE('',#76944,#9240);
#4713=LINE('',#76946,#9241);
#4714=LINE('',#76948,#9242);
#4715=LINE('',#76950,#9243);
#4716=LINE('',#76957,#9244);
#4717=LINE('',#76958,#9245);
#4718=LINE('',#76962,#9246);
#4719=LINE('',#76966,#9247);
#4720=LINE('',#76970,#9248);
#4721=LINE('',#76974,#9249);
#4722=LINE('',#76978,#9250);
#4723=LINE('',#76981,#9251);
#4724=LINE('',#76982,#9252);
#4725=LINE('',#76986,#9253);
#4726=LINE('',#76990,#9254);
#4727=LINE('',#76994,#9255);
#4728=LINE('',#76998,#9256);
#4729=LINE('',#77002,#9257);
#4730=LINE('',#77004,#9258);
#4731=LINE('',#77012,#9259);
#4732=LINE('',#77024,#9260);
#4733=LINE('',#77035,#9261);
#4734=LINE('',#77037,#9262);
#4735=LINE('',#77039,#9263);
#4736=LINE('',#77041,#9264);
#4737=LINE('',#77043,#9265);
#4738=LINE('',#77045,#9266);
#4739=LINE('',#77047,#9267);
#4740=LINE('',#77049,#9268);
#4741=LINE('',#77051,#9269);
#4742=LINE('',#77053,#9270);
#4743=LINE('',#77055,#9271);
#4744=LINE('',#77057,#9272);
#4745=LINE('',#77059,#9273);
#4746=LINE('',#77061,#9274);
#4747=LINE('',#77068,#9275);
#4748=LINE('',#77069,#9276);
#4749=LINE('',#77073,#9277);
#4750=LINE('',#77077,#9278);
#4751=LINE('',#77081,#9279);
#4752=LINE('',#77085,#9280);
#4753=LINE('',#77089,#9281);
#4754=LINE('',#77092,#9282);
#4755=LINE('',#77093,#9283);
#4756=LINE('',#77097,#9284);
#4757=LINE('',#77101,#9285);
#4758=LINE('',#77105,#9286);
#4759=LINE('',#77109,#9287);
#4760=LINE('',#77113,#9288);
#4761=LINE('',#77115,#9289);
#4762=LINE('',#77123,#9290);
#4763=LINE('',#77135,#9291);
#4764=LINE('',#77146,#9292);
#4765=LINE('',#77148,#9293);
#4766=LINE('',#77150,#9294);
#4767=LINE('',#77152,#9295);
#4768=LINE('',#77154,#9296);
#4769=LINE('',#77156,#9297);
#4770=LINE('',#77158,#9298);
#4771=LINE('',#77160,#9299);
#4772=LINE('',#77162,#9300);
#4773=LINE('',#77164,#9301);
#4774=LINE('',#77166,#9302);
#4775=LINE('',#77168,#9303);
#4776=LINE('',#77170,#9304);
#4777=LINE('',#77172,#9305);
#4778=LINE('',#77179,#9306);
#4779=LINE('',#77180,#9307);
#4780=LINE('',#77184,#9308);
#4781=LINE('',#77188,#9309);
#4782=LINE('',#77192,#9310);
#4783=LINE('',#77196,#9311);
#4784=LINE('',#77200,#9312);
#4785=LINE('',#77203,#9313);
#4786=LINE('',#77204,#9314);
#4787=LINE('',#77208,#9315);
#4788=LINE('',#77212,#9316);
#4789=LINE('',#77216,#9317);
#4790=LINE('',#77220,#9318);
#4791=LINE('',#77224,#9319);
#4792=LINE('',#77226,#9320);
#4793=LINE('',#77234,#9321);
#4794=LINE('',#77246,#9322);
#4795=LINE('',#77257,#9323);
#4796=LINE('',#77260,#9324);
#4797=LINE('',#77261,#9325);
#4798=LINE('',#77265,#9326);
#4799=LINE('',#77269,#9327);
#4800=LINE('',#77273,#9328);
#4801=LINE('',#77277,#9329);
#4802=LINE('',#77281,#9330);
#4803=LINE('',#77284,#9331);
#4804=LINE('',#77285,#9332);
#4805=LINE('',#77289,#9333);
#4806=LINE('',#77293,#9334);
#4807=LINE('',#77297,#9335);
#4808=LINE('',#77301,#9336);
#4809=LINE('',#77305,#9337);
#4810=LINE('',#77308,#9338);
#4811=LINE('',#77309,#9339);
#4812=LINE('',#77313,#9340);
#4813=LINE('',#77315,#9341);
#4814=LINE('',#77317,#9342);
#4815=LINE('',#77319,#9343);
#4816=LINE('',#77321,#9344);
#4817=LINE('',#77323,#9345);
#4818=LINE('',#77325,#9346);
#4819=LINE('',#77327,#9347);
#4820=LINE('',#77329,#9348);
#4821=LINE('',#77331,#9349);
#4822=LINE('',#77333,#9350);
#4823=LINE('',#77335,#9351);
#4824=LINE('',#77337,#9352);
#4825=LINE('',#77345,#9353);
#4826=LINE('',#77351,#9354);
#4827=LINE('',#77357,#9355);
#4828=LINE('',#77370,#9356);
#4829=LINE('',#77382,#9357);
#4830=LINE('',#77403,#9358);
#4831=LINE('',#77407,#9359);
#4832=LINE('',#77409,#9360);
#4833=LINE('',#77413,#9361);
#4834=LINE('',#77415,#9362);
#6688=VECTOR('',#55518,10.);
#6689=VECTOR('',#55519,10.);
#6690=VECTOR('',#55520,10.);
#6691=VECTOR('',#55521,10.);
#6692=VECTOR('',#55522,10.);
#6693=VECTOR('',#55523,10.);
#6694=VECTOR('',#55524,10.);
#6695=VECTOR('',#55525,10.);
#6696=VECTOR('',#55526,10.);
#6697=VECTOR('',#55527,10.);
#6698=VECTOR('',#55528,10.);
#6699=VECTOR('',#55529,10.);
#6700=VECTOR('',#55530,10.);
#6701=VECTOR('',#55531,10.);
#6702=VECTOR('',#55532,10.);
#6703=VECTOR('',#55533,10.);
#6704=VECTOR('',#55534,10.);
#6705=VECTOR('',#55535,10.);
#6706=VECTOR('',#55536,10.);
#6707=VECTOR('',#55537,10.);
#6708=VECTOR('',#55538,10.);
#6709=VECTOR('',#55539,10.);
#6710=VECTOR('',#55540,10.);
#6711=VECTOR('',#55541,10.);
#6712=VECTOR('',#55542,10.);
#6713=VECTOR('',#55543,10.);
#6714=VECTOR('',#55544,10.);
#6715=VECTOR('',#55545,10.);
#6716=VECTOR('',#55546,10.);
#6717=VECTOR('',#55547,10.);
#6718=VECTOR('',#55550,10.);
#6719=VECTOR('',#55551,10.);
#6720=VECTOR('',#55554,10.);
#6721=VECTOR('',#55557,10.);
#6722=VECTOR('',#55558,10.);
#6723=VECTOR('',#55559,10.);
#6724=VECTOR('',#55560,10.);
#6725=VECTOR('',#55561,10.);
#6726=VECTOR('',#55562,10.);
#6727=VECTOR('',#55563,10.);
#6728=VECTOR('',#55564,10.);
#6729=VECTOR('',#55565,10.);
#6730=VECTOR('',#55566,10.);
#6731=VECTOR('',#55567,10.);
#6732=VECTOR('',#55568,10.);
#6733=VECTOR('',#55569,10.);
#6734=VECTOR('',#55570,10.);
#6735=VECTOR('',#55571,10.);
#6736=VECTOR('',#55572,10.);
#6737=VECTOR('',#55573,10.);
#6738=VECTOR('',#55574,10.);
#6739=VECTOR('',#55575,10.);
#6740=VECTOR('',#55576,10.);
#6741=VECTOR('',#55577,10.);
#6742=VECTOR('',#55578,10.);
#6743=VECTOR('',#55579,10.);
#6744=VECTOR('',#55580,10.);
#6745=VECTOR('',#55581,10.);
#6746=VECTOR('',#55582,10.);
#6747=VECTOR('',#55583,10.);
#6748=VECTOR('',#55584,10.);
#6749=VECTOR('',#55585,10.);
#6750=VECTOR('',#55586,10.);
#6751=VECTOR('',#55589,10.);
#6752=VECTOR('',#55590,10.);
#6753=VECTOR('',#55593,10.);
#6754=VECTOR('',#55596,10.);
#6755=VECTOR('',#55597,10.);
#6756=VECTOR('',#55598,10.);
#6757=VECTOR('',#55599,10.);
#6758=VECTOR('',#55600,10.);
#6759=VECTOR('',#55601,10.);
#6760=VECTOR('',#55602,10.);
#6761=VECTOR('',#55603,10.);
#6762=VECTOR('',#55604,10.);
#6763=VECTOR('',#55605,10.);
#6764=VECTOR('',#55606,10.);
#6765=VECTOR('',#55607,10.);
#6766=VECTOR('',#55608,10.);
#6767=VECTOR('',#55609,10.);
#6768=VECTOR('',#55610,10.);
#6769=VECTOR('',#55611,10.);
#6770=VECTOR('',#55612,10.);
#6771=VECTOR('',#55613,10.);
#6772=VECTOR('',#55614,10.);
#6773=VECTOR('',#55615,10.);
#6774=VECTOR('',#55616,10.);
#6775=VECTOR('',#55617,10.);
#6776=VECTOR('',#55618,10.);
#6777=VECTOR('',#55619,10.);
#6778=VECTOR('',#55620,10.);
#6779=VECTOR('',#55621,10.);
#6780=VECTOR('',#55622,10.);
#6781=VECTOR('',#55623,10.);
#6782=VECTOR('',#55624,10.);
#6783=VECTOR('',#55625,10.);
#6784=VECTOR('',#55628,10.);
#6785=VECTOR('',#55629,10.);
#6786=VECTOR('',#55632,10.);
#6787=VECTOR('',#55635,10.);
#6788=VECTOR('',#55636,10.);
#6789=VECTOR('',#55637,10.);
#6790=VECTOR('',#55638,10.);
#6791=VECTOR('',#55639,10.);
#6792=VECTOR('',#55640,10.);
#6793=VECTOR('',#55641,10.);
#6794=VECTOR('',#55642,10.);
#6795=VECTOR('',#55643,10.);
#6796=VECTOR('',#55644,10.);
#6797=VECTOR('',#55645,10.);
#6798=VECTOR('',#55646,10.);
#6799=VECTOR('',#55647,10.);
#6800=VECTOR('',#55648,10.);
#6801=VECTOR('',#55649,10.);
#6802=VECTOR('',#55650,10.);
#6803=VECTOR('',#55651,10.);
#6804=VECTOR('',#55652,10.);
#6805=VECTOR('',#55653,10.);
#6806=VECTOR('',#55654,10.);
#6807=VECTOR('',#55655,10.);
#6808=VECTOR('',#55656,10.);
#6809=VECTOR('',#55657,10.);
#6810=VECTOR('',#55658,10.);
#6811=VECTOR('',#55659,10.);
#6812=VECTOR('',#55660,10.);
#6813=VECTOR('',#55661,10.);
#6814=VECTOR('',#55662,10.);
#6815=VECTOR('',#55663,10.);
#6816=VECTOR('',#55664,10.);
#6817=VECTOR('',#55667,10.);
#6818=VECTOR('',#55668,10.);
#6819=VECTOR('',#55671,10.);
#6820=VECTOR('',#55674,10.);
#6821=VECTOR('',#55675,10.);
#6822=VECTOR('',#55676,10.);
#6823=VECTOR('',#55677,10.);
#6824=VECTOR('',#55678,10.);
#6825=VECTOR('',#55679,10.);
#6826=VECTOR('',#55680,10.);
#6827=VECTOR('',#55681,10.);
#6828=VECTOR('',#55682,10.);
#6829=VECTOR('',#55683,10.);
#6830=VECTOR('',#55684,10.);
#6831=VECTOR('',#55685,10.);
#6832=VECTOR('',#55686,10.);
#6833=VECTOR('',#55687,10.);
#6834=VECTOR('',#55688,10.);
#6835=VECTOR('',#55689,10.);
#6836=VECTOR('',#55690,10.);
#6837=VECTOR('',#55691,10.);
#6838=VECTOR('',#55692,10.);
#6839=VECTOR('',#55693,10.);
#6840=VECTOR('',#55694,10.);
#6841=VECTOR('',#55695,10.);
#6842=VECTOR('',#55696,10.);
#6843=VECTOR('',#55697,10.);
#6844=VECTOR('',#55698,10.);
#6845=VECTOR('',#55699,10.);
#6846=VECTOR('',#55700,10.);
#6847=VECTOR('',#55701,10.);
#6848=VECTOR('',#55702,10.);
#6849=VECTOR('',#55703,10.);
#6850=VECTOR('',#55706,10.);
#6851=VECTOR('',#55707,10.);
#6852=VECTOR('',#55710,10.);
#6853=VECTOR('',#55713,10.);
#6854=VECTOR('',#55714,10.);
#6855=VECTOR('',#55715,10.);
#6856=VECTOR('',#55716,10.);
#6857=VECTOR('',#55717,10.);
#6858=VECTOR('',#55718,10.);
#6859=VECTOR('',#55719,10.);
#6860=VECTOR('',#55720,10.);
#6861=VECTOR('',#55721,10.);
#6862=VECTOR('',#55722,10.);
#6863=VECTOR('',#55723,10.);
#6864=VECTOR('',#55724,10.);
#6865=VECTOR('',#55725,10.);
#6866=VECTOR('',#55726,10.);
#6867=VECTOR('',#55727,10.);
#6868=VECTOR('',#55728,10.);
#6869=VECTOR('',#55729,10.);
#6870=VECTOR('',#55730,10.);
#6871=VECTOR('',#55731,10.);
#6872=VECTOR('',#55732,10.);
#6873=VECTOR('',#55733,10.);
#6874=VECTOR('',#55734,10.);
#6875=VECTOR('',#55735,10.);
#6876=VECTOR('',#55736,10.);
#6877=VECTOR('',#55737,10.);
#6878=VECTOR('',#55738,10.);
#6879=VECTOR('',#55739,10.);
#6880=VECTOR('',#55740,10.);
#6881=VECTOR('',#55741,10.);
#6882=VECTOR('',#55742,10.);
#6883=VECTOR('',#55745,10.);
#6884=VECTOR('',#55746,10.);
#6885=VECTOR('',#55749,10.);
#6886=VECTOR('',#55752,10.);
#6887=VECTOR('',#55753,10.);
#6888=VECTOR('',#55754,10.);
#6889=VECTOR('',#55755,10.);
#6890=VECTOR('',#55756,10.);
#6891=VECTOR('',#55757,10.);
#6892=VECTOR('',#55758,10.);
#6893=VECTOR('',#55759,10.);
#6894=VECTOR('',#55760,10.);
#6895=VECTOR('',#55761,10.);
#6896=VECTOR('',#55762,10.);
#6897=VECTOR('',#55763,10.);
#6898=VECTOR('',#55764,10.);
#6899=VECTOR('',#55765,10.);
#6900=VECTOR('',#55766,10.);
#6901=VECTOR('',#55767,10.);
#6902=VECTOR('',#55768,10.);
#6903=VECTOR('',#55769,10.);
#6904=VECTOR('',#55770,10.);
#6905=VECTOR('',#55771,10.);
#6906=VECTOR('',#55772,10.);
#6907=VECTOR('',#55773,10.);
#6908=VECTOR('',#55774,10.);
#6909=VECTOR('',#55775,10.);
#6910=VECTOR('',#55776,10.);
#6911=VECTOR('',#55777,10.);
#6912=VECTOR('',#55778,10.);
#6913=VECTOR('',#55779,10.);
#6914=VECTOR('',#55780,10.);
#6915=VECTOR('',#55781,10.);
#6916=VECTOR('',#55784,10.);
#6917=VECTOR('',#55785,10.);
#6918=VECTOR('',#55788,10.);
#6919=VECTOR('',#55791,10.);
#6920=VECTOR('',#55792,10.);
#6921=VECTOR('',#55793,10.);
#6922=VECTOR('',#55794,10.);
#6923=VECTOR('',#55795,10.);
#6924=VECTOR('',#55796,10.);
#6925=VECTOR('',#55797,10.);
#6926=VECTOR('',#55798,10.);
#6927=VECTOR('',#55799,10.);
#6928=VECTOR('',#55800,10.);
#6929=VECTOR('',#55801,10.);
#6930=VECTOR('',#55802,10.);
#6931=VECTOR('',#55803,10.);
#6932=VECTOR('',#55804,10.);
#6933=VECTOR('',#55805,10.);
#6934=VECTOR('',#55806,10.);
#6935=VECTOR('',#55807,10.);
#6936=VECTOR('',#55808,10.);
#6937=VECTOR('',#55809,10.);
#6938=VECTOR('',#55810,10.);
#6939=VECTOR('',#55811,10.);
#6940=VECTOR('',#55812,10.);
#6941=VECTOR('',#55813,10.);
#6942=VECTOR('',#55814,10.);
#6943=VECTOR('',#55815,10.);
#6944=VECTOR('',#55816,10.);
#6945=VECTOR('',#55817,10.);
#6946=VECTOR('',#55818,10.);
#6947=VECTOR('',#55819,10.);
#6948=VECTOR('',#55820,10.);
#6949=VECTOR('',#55823,10.);
#6950=VECTOR('',#55824,10.);
#6951=VECTOR('',#55827,10.);
#6952=VECTOR('',#55830,10.);
#6953=VECTOR('',#55831,10.);
#6954=VECTOR('',#55832,10.);
#6955=VECTOR('',#55833,10.);
#6956=VECTOR('',#55834,10.);
#6957=VECTOR('',#55835,10.);
#6958=VECTOR('',#55836,10.);
#6959=VECTOR('',#55837,10.);
#6960=VECTOR('',#55838,10.);
#6961=VECTOR('',#55839,10.);
#6962=VECTOR('',#55840,10.);
#6963=VECTOR('',#55841,10.);
#6964=VECTOR('',#55842,10.);
#6965=VECTOR('',#55843,10.);
#6966=VECTOR('',#55844,10.);
#6967=VECTOR('',#55845,10.);
#6968=VECTOR('',#55846,10.);
#6969=VECTOR('',#55847,10.);
#6970=VECTOR('',#55848,10.);
#6971=VECTOR('',#55849,10.);
#6972=VECTOR('',#55850,10.);
#6973=VECTOR('',#55851,10.);
#6974=VECTOR('',#55852,10.);
#6975=VECTOR('',#55853,10.);
#6976=VECTOR('',#55854,10.);
#6977=VECTOR('',#55855,10.);
#6978=VECTOR('',#55856,10.);
#6979=VECTOR('',#55857,10.);
#6980=VECTOR('',#55858,10.);
#6981=VECTOR('',#55859,10.);
#6982=VECTOR('',#55862,10.);
#6983=VECTOR('',#55863,10.);
#6984=VECTOR('',#55866,10.);
#6985=VECTOR('',#55869,10.);
#6986=VECTOR('',#55870,10.);
#6987=VECTOR('',#55871,10.);
#6988=VECTOR('',#55872,10.);
#6989=VECTOR('',#55873,10.);
#6990=VECTOR('',#55874,10.);
#6991=VECTOR('',#55875,10.);
#6992=VECTOR('',#55876,10.);
#6993=VECTOR('',#55877,10.);
#6994=VECTOR('',#55878,10.);
#6995=VECTOR('',#55879,10.);
#6996=VECTOR('',#55880,10.);
#6997=VECTOR('',#55881,10.);
#6998=VECTOR('',#55882,10.);
#6999=VECTOR('',#55883,10.);
#7000=VECTOR('',#55884,10.);
#7001=VECTOR('',#55885,10.);
#7002=VECTOR('',#55886,10.);
#7003=VECTOR('',#55887,10.);
#7004=VECTOR('',#55888,10.);
#7005=VECTOR('',#55889,10.);
#7006=VECTOR('',#55890,10.);
#7007=VECTOR('',#55891,10.);
#7008=VECTOR('',#55892,10.);
#7009=VECTOR('',#55893,10.);
#7010=VECTOR('',#55894,10.);
#7011=VECTOR('',#55895,10.);
#7012=VECTOR('',#55896,10.);
#7013=VECTOR('',#55897,10.);
#7014=VECTOR('',#55898,10.);
#7015=VECTOR('',#55901,10.);
#7016=VECTOR('',#55902,10.);
#7017=VECTOR('',#55905,10.);
#7018=VECTOR('',#55908,10.);
#7019=VECTOR('',#55909,10.);
#7020=VECTOR('',#55910,10.);
#7021=VECTOR('',#55911,10.);
#7022=VECTOR('',#55912,10.);
#7023=VECTOR('',#55913,10.);
#7024=VECTOR('',#55914,10.);
#7025=VECTOR('',#55915,10.);
#7026=VECTOR('',#55916,10.);
#7027=VECTOR('',#55917,10.);
#7028=VECTOR('',#55918,10.);
#7029=VECTOR('',#55919,10.);
#7030=VECTOR('',#55920,10.);
#7031=VECTOR('',#55921,10.);
#7032=VECTOR('',#55922,10.);
#7033=VECTOR('',#55923,10.);
#7034=VECTOR('',#55924,10.);
#7035=VECTOR('',#55925,10.);
#7036=VECTOR('',#55926,10.);
#7037=VECTOR('',#55927,10.);
#7038=VECTOR('',#55928,10.);
#7039=VECTOR('',#55929,10.);
#7040=VECTOR('',#55930,10.);
#7041=VECTOR('',#55931,10.);
#7042=VECTOR('',#55932,10.);
#7043=VECTOR('',#55933,10.);
#7044=VECTOR('',#55934,10.);
#7045=VECTOR('',#55935,10.);
#7046=VECTOR('',#55936,10.);
#7047=VECTOR('',#55937,10.);
#7048=VECTOR('',#55940,10.);
#7049=VECTOR('',#55941,10.);
#7050=VECTOR('',#55944,10.);
#7051=VECTOR('',#55947,10.);
#7052=VECTOR('',#55948,10.);
#7053=VECTOR('',#55949,10.);
#7054=VECTOR('',#55950,10.);
#7055=VECTOR('',#55951,10.);
#7056=VECTOR('',#55952,10.);
#7057=VECTOR('',#55953,10.);
#7058=VECTOR('',#55954,10.);
#7059=VECTOR('',#55955,10.);
#7060=VECTOR('',#55956,10.);
#7061=VECTOR('',#55957,10.);
#7062=VECTOR('',#55958,10.);
#7063=VECTOR('',#55959,10.);
#7064=VECTOR('',#55960,10.);
#7065=VECTOR('',#55961,10.);
#7066=VECTOR('',#55962,10.);
#7067=VECTOR('',#55963,10.);
#7068=VECTOR('',#55964,10.);
#7069=VECTOR('',#55965,10.);
#7070=VECTOR('',#55966,10.);
#7071=VECTOR('',#55967,10.);
#7072=VECTOR('',#55968,10.);
#7073=VECTOR('',#55969,10.);
#7074=VECTOR('',#55970,10.);
#7075=VECTOR('',#55971,10.);
#7076=VECTOR('',#55972,10.);
#7077=VECTOR('',#55973,10.);
#7078=VECTOR('',#55974,10.);
#7079=VECTOR('',#55975,10.);
#7080=VECTOR('',#55976,10.);
#7081=VECTOR('',#55979,10.);
#7082=VECTOR('',#55980,10.);
#7083=VECTOR('',#55983,10.);
#7084=VECTOR('',#55986,10.);
#7085=VECTOR('',#55987,10.);
#7086=VECTOR('',#55988,10.);
#7087=VECTOR('',#55989,10.);
#7088=VECTOR('',#55990,10.);
#7089=VECTOR('',#55991,10.);
#7090=VECTOR('',#55992,10.);
#7091=VECTOR('',#55993,10.);
#7092=VECTOR('',#55994,10.);
#7093=VECTOR('',#55995,10.);
#7094=VECTOR('',#55996,10.);
#7095=VECTOR('',#55997,10.);
#7096=VECTOR('',#55998,10.);
#7097=VECTOR('',#55999,10.);
#7098=VECTOR('',#56000,10.);
#7099=VECTOR('',#56001,10.);
#7100=VECTOR('',#56002,10.);
#7101=VECTOR('',#56003,10.);
#7102=VECTOR('',#56004,10.);
#7103=VECTOR('',#56005,10.);
#7104=VECTOR('',#56006,10.);
#7105=VECTOR('',#56007,10.);
#7106=VECTOR('',#56008,10.);
#7107=VECTOR('',#56009,10.);
#7108=VECTOR('',#56010,10.);
#7109=VECTOR('',#56011,10.);
#7110=VECTOR('',#56012,10.);
#7111=VECTOR('',#56013,10.);
#7112=VECTOR('',#56014,10.);
#7113=VECTOR('',#56015,10.);
#7114=VECTOR('',#56018,10.);
#7115=VECTOR('',#56019,10.);
#7116=VECTOR('',#56022,10.);
#7117=VECTOR('',#56025,10.);
#7118=VECTOR('',#56026,10.);
#7119=VECTOR('',#56027,10.);
#7120=VECTOR('',#56028,10.);
#7121=VECTOR('',#56029,10.);
#7122=VECTOR('',#56030,10.);
#7123=VECTOR('',#56031,10.);
#7124=VECTOR('',#56032,10.);
#7125=VECTOR('',#56033,10.);
#7126=VECTOR('',#56034,10.);
#7127=VECTOR('',#56035,10.);
#7128=VECTOR('',#56036,10.);
#7129=VECTOR('',#56037,10.);
#7130=VECTOR('',#56038,10.);
#7131=VECTOR('',#56039,10.);
#7132=VECTOR('',#56040,10.);
#7133=VECTOR('',#56041,10.);
#7134=VECTOR('',#56042,10.);
#7135=VECTOR('',#56043,10.);
#7136=VECTOR('',#56044,10.);
#7137=VECTOR('',#56045,10.);
#7138=VECTOR('',#56046,10.);
#7139=VECTOR('',#56047,10.);
#7140=VECTOR('',#56048,10.);
#7141=VECTOR('',#56049,10.);
#7142=VECTOR('',#56050,10.);
#7143=VECTOR('',#56051,10.);
#7144=VECTOR('',#56052,10.);
#7145=VECTOR('',#56053,10.);
#7146=VECTOR('',#56054,10.);
#7147=VECTOR('',#56057,10.);
#7148=VECTOR('',#56058,10.);
#7149=VECTOR('',#56061,10.);
#7150=VECTOR('',#56064,10.);
#7151=VECTOR('',#56065,10.);
#7152=VECTOR('',#56066,10.);
#7153=VECTOR('',#56067,10.);
#7154=VECTOR('',#56068,10.);
#7155=VECTOR('',#56069,10.);
#7156=VECTOR('',#56070,10.);
#7157=VECTOR('',#56071,10.);
#7158=VECTOR('',#56072,10.);
#7159=VECTOR('',#56073,10.);
#7160=VECTOR('',#56074,10.);
#7161=VECTOR('',#56075,10.);
#7162=VECTOR('',#56076,10.);
#7163=VECTOR('',#56077,10.);
#7164=VECTOR('',#56078,10.);
#7165=VECTOR('',#56079,10.);
#7166=VECTOR('',#56080,10.);
#7167=VECTOR('',#56081,10.);
#7168=VECTOR('',#56082,10.);
#7169=VECTOR('',#56083,10.);
#7170=VECTOR('',#56084,10.);
#7171=VECTOR('',#56085,10.);
#7172=VECTOR('',#56086,10.);
#7173=VECTOR('',#56087,10.);
#7174=VECTOR('',#56088,10.);
#7175=VECTOR('',#56089,10.);
#7176=VECTOR('',#56090,10.);
#7177=VECTOR('',#56091,10.);
#7178=VECTOR('',#56092,10.);
#7179=VECTOR('',#56093,10.);
#7180=VECTOR('',#56096,10.);
#7181=VECTOR('',#56097,10.);
#7182=VECTOR('',#56100,10.);
#7183=VECTOR('',#56103,10.);
#7184=VECTOR('',#56104,10.);
#7185=VECTOR('',#56105,10.);
#7186=VECTOR('',#56106,10.);
#7187=VECTOR('',#56107,10.);
#7188=VECTOR('',#56108,10.);
#7189=VECTOR('',#56109,10.);
#7190=VECTOR('',#56110,10.);
#7191=VECTOR('',#56111,10.);
#7192=VECTOR('',#56112,10.);
#7193=VECTOR('',#56113,10.);
#7194=VECTOR('',#56114,10.);
#7195=VECTOR('',#56115,10.);
#7196=VECTOR('',#56116,10.);
#7197=VECTOR('',#56117,10.);
#7198=VECTOR('',#56118,10.);
#7199=VECTOR('',#56119,10.);
#7200=VECTOR('',#56120,10.);
#7201=VECTOR('',#56121,10.);
#7202=VECTOR('',#56122,10.);
#7203=VECTOR('',#56123,10.);
#7204=VECTOR('',#56124,10.);
#7205=VECTOR('',#56125,10.);
#7206=VECTOR('',#56126,10.);
#7207=VECTOR('',#56127,10.);
#7208=VECTOR('',#56128,10.);
#7209=VECTOR('',#56129,10.);
#7210=VECTOR('',#56130,10.);
#7211=VECTOR('',#56131,10.);
#7212=VECTOR('',#56132,10.);
#7213=VECTOR('',#56135,10.);
#7214=VECTOR('',#56136,10.);
#7215=VECTOR('',#56139,10.);
#7216=VECTOR('',#56142,10.);
#7217=VECTOR('',#56143,10.);
#7218=VECTOR('',#56144,10.);
#7219=VECTOR('',#56145,10.);
#7220=VECTOR('',#56146,10.);
#7221=VECTOR('',#56147,10.);
#7222=VECTOR('',#56148,10.);
#7223=VECTOR('',#56149,10.);
#7224=VECTOR('',#56150,10.);
#7225=VECTOR('',#56151,10.);
#7226=VECTOR('',#56152,10.);
#7227=VECTOR('',#56153,10.);
#7228=VECTOR('',#56154,10.);
#7229=VECTOR('',#56155,10.);
#7230=VECTOR('',#56156,10.);
#7231=VECTOR('',#56157,10.);
#7232=VECTOR('',#56158,10.);
#7233=VECTOR('',#56159,10.);
#7234=VECTOR('',#56160,10.);
#7235=VECTOR('',#56161,10.);
#7236=VECTOR('',#56162,10.);
#7237=VECTOR('',#56163,10.);
#7238=VECTOR('',#56164,10.);
#7239=VECTOR('',#56165,10.);
#7240=VECTOR('',#56166,10.);
#7241=VECTOR('',#56167,10.);
#7242=VECTOR('',#56168,10.);
#7243=VECTOR('',#56169,10.);
#7244=VECTOR('',#56170,10.);
#7245=VECTOR('',#56171,10.);
#7246=VECTOR('',#56174,10.);
#7247=VECTOR('',#56175,10.);
#7248=VECTOR('',#56178,10.);
#7249=VECTOR('',#56181,10.);
#7250=VECTOR('',#56182,10.);
#7251=VECTOR('',#56183,10.);
#7252=VECTOR('',#56184,10.);
#7253=VECTOR('',#56185,10.);
#7254=VECTOR('',#56186,10.);
#7255=VECTOR('',#56187,10.);
#7256=VECTOR('',#56188,10.);
#7257=VECTOR('',#56189,10.);
#7258=VECTOR('',#56190,10.);
#7259=VECTOR('',#56191,10.);
#7260=VECTOR('',#56192,10.);
#7261=VECTOR('',#56193,10.);
#7262=VECTOR('',#56194,10.);
#7263=VECTOR('',#56195,10.);
#7264=VECTOR('',#56196,10.);
#7265=VECTOR('',#56197,10.);
#7266=VECTOR('',#56198,10.);
#7267=VECTOR('',#56199,10.);
#7268=VECTOR('',#56200,10.);
#7269=VECTOR('',#56201,10.);
#7270=VECTOR('',#56202,10.);
#7271=VECTOR('',#56203,10.);
#7272=VECTOR('',#56204,10.);
#7273=VECTOR('',#56205,10.);
#7274=VECTOR('',#56206,10.);
#7275=VECTOR('',#56207,10.);
#7276=VECTOR('',#56208,10.);
#7277=VECTOR('',#56209,10.);
#7278=VECTOR('',#56210,10.);
#7279=VECTOR('',#56213,10.);
#7280=VECTOR('',#56214,10.);
#7281=VECTOR('',#56217,10.);
#7282=VECTOR('',#56220,10.);
#7283=VECTOR('',#56221,10.);
#7284=VECTOR('',#56222,10.);
#7285=VECTOR('',#56223,10.);
#7286=VECTOR('',#56224,10.);
#7287=VECTOR('',#56225,10.);
#7288=VECTOR('',#56226,10.);
#7289=VECTOR('',#56227,10.);
#7290=VECTOR('',#56228,10.);
#7291=VECTOR('',#56229,10.);
#7292=VECTOR('',#56230,10.);
#7293=VECTOR('',#56231,10.);
#7294=VECTOR('',#56232,10.);
#7295=VECTOR('',#56233,10.);
#7296=VECTOR('',#56234,10.);
#7297=VECTOR('',#56235,10.);
#7298=VECTOR('',#56236,10.);
#7299=VECTOR('',#56237,10.);
#7300=VECTOR('',#56238,10.);
#7301=VECTOR('',#56239,10.);
#7302=VECTOR('',#56240,10.);
#7303=VECTOR('',#56241,10.);
#7304=VECTOR('',#56242,10.);
#7305=VECTOR('',#56243,10.);
#7306=VECTOR('',#56244,10.);
#7307=VECTOR('',#56245,10.);
#7308=VECTOR('',#56246,10.);
#7309=VECTOR('',#56247,10.);
#7310=VECTOR('',#56248,10.);
#7311=VECTOR('',#56249,10.);
#7312=VECTOR('',#56252,10.);
#7313=VECTOR('',#56253,10.);
#7314=VECTOR('',#56256,10.);
#7315=VECTOR('',#56259,10.);
#7316=VECTOR('',#56260,10.);
#7317=VECTOR('',#56261,10.);
#7318=VECTOR('',#56262,10.);
#7319=VECTOR('',#56263,10.);
#7320=VECTOR('',#56264,10.);
#7321=VECTOR('',#56265,10.);
#7322=VECTOR('',#56266,10.);
#7323=VECTOR('',#56267,10.);
#7324=VECTOR('',#56268,10.);
#7325=VECTOR('',#56269,10.);
#7326=VECTOR('',#56270,10.);
#7327=VECTOR('',#56271,10.);
#7328=VECTOR('',#56272,10.);
#7329=VECTOR('',#56273,10.);
#7330=VECTOR('',#56274,10.);
#7331=VECTOR('',#56275,10.);
#7332=VECTOR('',#56276,10.);
#7333=VECTOR('',#56277,10.);
#7334=VECTOR('',#56278,10.);
#7335=VECTOR('',#56279,10.);
#7336=VECTOR('',#56280,10.);
#7337=VECTOR('',#56281,10.);
#7338=VECTOR('',#56282,10.);
#7339=VECTOR('',#56283,10.);
#7340=VECTOR('',#56284,10.);
#7341=VECTOR('',#56285,10.);
#7342=VECTOR('',#56286,10.);
#7343=VECTOR('',#56287,10.);
#7344=VECTOR('',#56288,10.);
#7345=VECTOR('',#56291,10.);
#7346=VECTOR('',#56292,10.);
#7347=VECTOR('',#56295,10.);
#7348=VECTOR('',#56298,10.);
#7349=VECTOR('',#56299,10.);
#7350=VECTOR('',#56300,10.);
#7351=VECTOR('',#56301,10.);
#7352=VECTOR('',#56302,10.);
#7353=VECTOR('',#56303,10.);
#7354=VECTOR('',#56304,10.);
#7355=VECTOR('',#56305,10.);
#7356=VECTOR('',#56306,10.);
#7357=VECTOR('',#56307,10.);
#7358=VECTOR('',#56308,10.);
#7359=VECTOR('',#56309,10.);
#7360=VECTOR('',#56310,10.);
#7361=VECTOR('',#56311,10.);
#7362=VECTOR('',#56312,10.);
#7363=VECTOR('',#56313,10.);
#7364=VECTOR('',#56314,10.);
#7365=VECTOR('',#56315,10.);
#7366=VECTOR('',#56316,10.);
#7367=VECTOR('',#56317,10.);
#7368=VECTOR('',#56318,10.);
#7369=VECTOR('',#56319,10.);
#7370=VECTOR('',#56320,10.);
#7371=VECTOR('',#56321,10.);
#7372=VECTOR('',#56322,10.);
#7373=VECTOR('',#56323,10.);
#7374=VECTOR('',#56324,10.);
#7375=VECTOR('',#56325,10.);
#7376=VECTOR('',#56326,10.);
#7377=VECTOR('',#56327,10.);
#7378=VECTOR('',#56330,10.);
#7379=VECTOR('',#56331,10.);
#7380=VECTOR('',#56334,10.);
#7381=VECTOR('',#56337,10.);
#7382=VECTOR('',#56338,10.);
#7383=VECTOR('',#56339,10.);
#7384=VECTOR('',#56340,10.);
#7385=VECTOR('',#56341,10.);
#7386=VECTOR('',#56342,10.);
#7387=VECTOR('',#56343,10.);
#7388=VECTOR('',#56344,10.);
#7389=VECTOR('',#56345,10.);
#7390=VECTOR('',#56346,10.);
#7391=VECTOR('',#56347,10.);
#7392=VECTOR('',#56348,10.);
#7393=VECTOR('',#56349,10.);
#7394=VECTOR('',#56350,10.);
#7395=VECTOR('',#56351,10.);
#7396=VECTOR('',#56352,10.);
#7397=VECTOR('',#56353,10.);
#7398=VECTOR('',#56354,10.);
#7399=VECTOR('',#56355,10.);
#7400=VECTOR('',#56356,10.);
#7401=VECTOR('',#56357,10.);
#7402=VECTOR('',#56358,10.);
#7403=VECTOR('',#56359,10.);
#7404=VECTOR('',#56360,10.);
#7405=VECTOR('',#56361,10.);
#7406=VECTOR('',#56362,10.);
#7407=VECTOR('',#56363,10.);
#7408=VECTOR('',#56364,10.);
#7409=VECTOR('',#56365,10.);
#7410=VECTOR('',#56366,10.);
#7411=VECTOR('',#56369,10.);
#7412=VECTOR('',#56370,10.);
#7413=VECTOR('',#56373,10.);
#7414=VECTOR('',#56376,10.);
#7415=VECTOR('',#56377,10.);
#7416=VECTOR('',#56378,10.);
#7417=VECTOR('',#56379,10.);
#7418=VECTOR('',#56380,10.);
#7419=VECTOR('',#56381,10.);
#7420=VECTOR('',#56382,10.);
#7421=VECTOR('',#56383,10.);
#7422=VECTOR('',#56384,10.);
#7423=VECTOR('',#56385,10.);
#7424=VECTOR('',#56386,10.);
#7425=VECTOR('',#56387,10.);
#7426=VECTOR('',#56388,10.);
#7427=VECTOR('',#56389,10.);
#7428=VECTOR('',#56390,10.);
#7429=VECTOR('',#56391,10.);
#7430=VECTOR('',#56392,10.);
#7431=VECTOR('',#56393,10.);
#7432=VECTOR('',#56394,10.);
#7433=VECTOR('',#56395,10.);
#7434=VECTOR('',#56396,10.);
#7435=VECTOR('',#56397,10.);
#7436=VECTOR('',#56398,10.);
#7437=VECTOR('',#56399,10.);
#7438=VECTOR('',#56400,10.);
#7439=VECTOR('',#56401,10.);
#7440=VECTOR('',#56402,10.);
#7441=VECTOR('',#56403,10.);
#7442=VECTOR('',#56404,10.);
#7443=VECTOR('',#56405,10.);
#7444=VECTOR('',#56408,10.);
#7445=VECTOR('',#56409,10.);
#7446=VECTOR('',#56412,10.);
#7447=VECTOR('',#56415,10.);
#7448=VECTOR('',#56416,10.);
#7449=VECTOR('',#56417,10.);
#7450=VECTOR('',#56418,10.);
#7451=VECTOR('',#56419,10.);
#7452=VECTOR('',#56420,10.);
#7453=VECTOR('',#56421,10.);
#7454=VECTOR('',#56422,10.);
#7455=VECTOR('',#56423,10.);
#7456=VECTOR('',#56424,10.);
#7457=VECTOR('',#56425,10.);
#7458=VECTOR('',#56426,10.);
#7459=VECTOR('',#56427,10.);
#7460=VECTOR('',#56428,10.);
#7461=VECTOR('',#56429,10.);
#7462=VECTOR('',#56430,10.);
#7463=VECTOR('',#56431,10.);
#7464=VECTOR('',#56432,10.);
#7465=VECTOR('',#56433,10.);
#7466=VECTOR('',#56434,10.);
#7467=VECTOR('',#56435,10.);
#7468=VECTOR('',#56436,10.);
#7469=VECTOR('',#56437,10.);
#7470=VECTOR('',#56438,10.);
#7471=VECTOR('',#56439,10.);
#7472=VECTOR('',#56440,10.);
#7473=VECTOR('',#56441,10.);
#7474=VECTOR('',#56442,10.);
#7475=VECTOR('',#56443,10.);
#7476=VECTOR('',#56444,10.);
#7477=VECTOR('',#56447,10.);
#7478=VECTOR('',#56448,10.);
#7479=VECTOR('',#56451,10.);
#7480=VECTOR('',#56454,10.);
#7481=VECTOR('',#56455,10.);
#7482=VECTOR('',#56456,10.);
#7483=VECTOR('',#56457,10.);
#7484=VECTOR('',#56458,10.);
#7485=VECTOR('',#56459,10.);
#7486=VECTOR('',#56460,10.);
#7487=VECTOR('',#56461,10.);
#7488=VECTOR('',#56462,10.);
#7489=VECTOR('',#56463,10.);
#7490=VECTOR('',#56464,10.);
#7491=VECTOR('',#56465,10.);
#7492=VECTOR('',#56466,10.);
#7493=VECTOR('',#56467,10.);
#7494=VECTOR('',#56468,10.);
#7495=VECTOR('',#56469,10.);
#7496=VECTOR('',#56470,10.);
#7497=VECTOR('',#56471,10.);
#7498=VECTOR('',#56472,10.);
#7499=VECTOR('',#56473,10.);
#7500=VECTOR('',#56474,10.);
#7501=VECTOR('',#56475,10.);
#7502=VECTOR('',#56476,10.);
#7503=VECTOR('',#56477,10.);
#7504=VECTOR('',#56478,10.);
#7505=VECTOR('',#56479,10.);
#7506=VECTOR('',#56480,10.);
#7507=VECTOR('',#56481,10.);
#7508=VECTOR('',#56482,10.);
#7509=VECTOR('',#56483,10.);
#7510=VECTOR('',#56486,10.);
#7511=VECTOR('',#56487,10.);
#7512=VECTOR('',#56490,10.);
#7513=VECTOR('',#56493,10.);
#7514=VECTOR('',#56494,10.);
#7515=VECTOR('',#56495,10.);
#7516=VECTOR('',#56496,10.);
#7517=VECTOR('',#56497,10.);
#7518=VECTOR('',#56498,10.);
#7519=VECTOR('',#56499,10.);
#7520=VECTOR('',#56500,10.);
#7521=VECTOR('',#56501,10.);
#7522=VECTOR('',#56502,10.);
#7523=VECTOR('',#56503,10.);
#7524=VECTOR('',#56504,10.);
#7525=VECTOR('',#56505,10.);
#7526=VECTOR('',#56506,10.);
#7527=VECTOR('',#56507,10.);
#7528=VECTOR('',#56508,10.);
#7529=VECTOR('',#56509,10.);
#7530=VECTOR('',#56510,10.);
#7531=VECTOR('',#56511,10.);
#7532=VECTOR('',#56512,10.);
#7533=VECTOR('',#56513,10.);
#7534=VECTOR('',#56514,10.);
#7535=VECTOR('',#56515,10.);
#7536=VECTOR('',#56516,10.);
#7537=VECTOR('',#56517,10.);
#7538=VECTOR('',#56518,10.);
#7539=VECTOR('',#56519,10.);
#7540=VECTOR('',#56520,10.);
#7541=VECTOR('',#56521,10.);
#7542=VECTOR('',#56522,10.);
#7543=VECTOR('',#56525,10.);
#7544=VECTOR('',#56526,10.);
#7545=VECTOR('',#56529,10.);
#7546=VECTOR('',#56532,10.);
#7547=VECTOR('',#56533,10.);
#7548=VECTOR('',#56534,10.);
#7549=VECTOR('',#56535,10.);
#7550=VECTOR('',#56536,10.);
#7551=VECTOR('',#56537,10.);
#7552=VECTOR('',#56538,10.);
#7553=VECTOR('',#56539,10.);
#7554=VECTOR('',#56540,10.);
#7555=VECTOR('',#56541,10.);
#7556=VECTOR('',#56542,10.);
#7557=VECTOR('',#56543,10.);
#7558=VECTOR('',#56544,10.);
#7559=VECTOR('',#56545,10.);
#7560=VECTOR('',#56546,10.);
#7561=VECTOR('',#56547,10.);
#7562=VECTOR('',#56548,10.);
#7563=VECTOR('',#56549,10.);
#7564=VECTOR('',#56550,10.);
#7565=VECTOR('',#56551,10.);
#7566=VECTOR('',#56552,10.);
#7567=VECTOR('',#56553,10.);
#7568=VECTOR('',#56554,10.);
#7569=VECTOR('',#56555,10.);
#7570=VECTOR('',#56556,10.);
#7571=VECTOR('',#56557,10.);
#7572=VECTOR('',#56558,10.);
#7573=VECTOR('',#56559,10.);
#7574=VECTOR('',#56560,10.);
#7575=VECTOR('',#56561,10.);
#7576=VECTOR('',#56564,10.);
#7577=VECTOR('',#56565,10.);
#7578=VECTOR('',#56568,10.);
#7579=VECTOR('',#56571,10.);
#7580=VECTOR('',#56572,10.);
#7581=VECTOR('',#56573,10.);
#7582=VECTOR('',#56574,10.);
#7583=VECTOR('',#56575,10.);
#7584=VECTOR('',#56576,10.);
#7585=VECTOR('',#56577,10.);
#7586=VECTOR('',#56578,10.);
#7587=VECTOR('',#56579,10.);
#7588=VECTOR('',#56580,10.);
#7589=VECTOR('',#56581,10.);
#7590=VECTOR('',#56582,10.);
#7591=VECTOR('',#56583,10.);
#7592=VECTOR('',#56584,10.);
#7593=VECTOR('',#56585,10.);
#7594=VECTOR('',#56586,10.);
#7595=VECTOR('',#56587,10.);
#7596=VECTOR('',#56588,10.);
#7597=VECTOR('',#56589,10.);
#7598=VECTOR('',#56590,10.);
#7599=VECTOR('',#56591,10.);
#7600=VECTOR('',#56592,10.);
#7601=VECTOR('',#56593,10.);
#7602=VECTOR('',#56594,10.);
#7603=VECTOR('',#56595,10.);
#7604=VECTOR('',#56596,10.);
#7605=VECTOR('',#56597,10.);
#7606=VECTOR('',#56598,10.);
#7607=VECTOR('',#56599,10.);
#7608=VECTOR('',#56600,10.);
#7609=VECTOR('',#56603,10.);
#7610=VECTOR('',#56604,10.);
#7611=VECTOR('',#56607,10.);
#7612=VECTOR('',#56610,10.);
#7613=VECTOR('',#56611,10.);
#7614=VECTOR('',#56612,10.);
#7615=VECTOR('',#56613,10.);
#7616=VECTOR('',#56614,10.);
#7617=VECTOR('',#56615,10.);
#7618=VECTOR('',#56616,10.);
#7619=VECTOR('',#56617,10.);
#7620=VECTOR('',#56618,10.);
#7621=VECTOR('',#56619,10.);
#7622=VECTOR('',#56620,10.);
#7623=VECTOR('',#56621,10.);
#7624=VECTOR('',#56622,10.);
#7625=VECTOR('',#56623,10.);
#7626=VECTOR('',#56624,10.);
#7627=VECTOR('',#56625,10.);
#7628=VECTOR('',#56626,10.);
#7629=VECTOR('',#56627,10.);
#7630=VECTOR('',#56628,10.);
#7631=VECTOR('',#56629,10.);
#7632=VECTOR('',#56630,10.);
#7633=VECTOR('',#56631,10.);
#7634=VECTOR('',#56632,10.);
#7635=VECTOR('',#56633,10.);
#7636=VECTOR('',#56634,10.);
#7637=VECTOR('',#56635,10.);
#7638=VECTOR('',#56636,10.);
#7639=VECTOR('',#56637,10.);
#7640=VECTOR('',#56638,10.);
#7641=VECTOR('',#56639,10.);
#7642=VECTOR('',#56642,10.);
#7643=VECTOR('',#56643,10.);
#7644=VECTOR('',#56646,10.);
#7645=VECTOR('',#56649,10.);
#7646=VECTOR('',#56650,10.);
#7647=VECTOR('',#56651,10.);
#7648=VECTOR('',#56652,10.);
#7649=VECTOR('',#56653,10.);
#7650=VECTOR('',#56654,10.);
#7651=VECTOR('',#56655,10.);
#7652=VECTOR('',#56656,10.);
#7653=VECTOR('',#56657,10.);
#7654=VECTOR('',#56658,10.);
#7655=VECTOR('',#56659,10.);
#7656=VECTOR('',#56660,10.);
#7657=VECTOR('',#56661,10.);
#7658=VECTOR('',#56662,10.);
#7659=VECTOR('',#56663,10.);
#7660=VECTOR('',#56664,10.);
#7661=VECTOR('',#56665,10.);
#7662=VECTOR('',#56666,10.);
#7663=VECTOR('',#56667,10.);
#7664=VECTOR('',#56668,10.);
#7665=VECTOR('',#56669,10.);
#7666=VECTOR('',#56670,10.);
#7667=VECTOR('',#56671,10.);
#7668=VECTOR('',#56672,10.);
#7669=VECTOR('',#56673,10.);
#7670=VECTOR('',#56674,10.);
#7671=VECTOR('',#56675,10.);
#7672=VECTOR('',#56676,10.);
#7673=VECTOR('',#56677,10.);
#7674=VECTOR('',#56678,10.);
#7675=VECTOR('',#56681,10.);
#7676=VECTOR('',#56682,10.);
#7677=VECTOR('',#56685,10.);
#7678=VECTOR('',#56688,10.);
#7679=VECTOR('',#56689,10.);
#7680=VECTOR('',#56690,10.);
#7681=VECTOR('',#56691,10.);
#7682=VECTOR('',#56692,10.);
#7683=VECTOR('',#56693,10.);
#7684=VECTOR('',#56694,10.);
#7685=VECTOR('',#56695,10.);
#7686=VECTOR('',#56696,10.);
#7687=VECTOR('',#56697,10.);
#7688=VECTOR('',#56698,10.);
#7689=VECTOR('',#56699,10.);
#7690=VECTOR('',#56700,10.);
#7691=VECTOR('',#56701,10.);
#7692=VECTOR('',#56702,10.);
#7693=VECTOR('',#56703,10.);
#7694=VECTOR('',#56704,10.);
#7695=VECTOR('',#56705,10.);
#7696=VECTOR('',#56706,10.);
#7697=VECTOR('',#56707,10.);
#7698=VECTOR('',#56708,10.);
#7699=VECTOR('',#56709,10.);
#7700=VECTOR('',#56710,10.);
#7701=VECTOR('',#56711,10.);
#7702=VECTOR('',#56712,10.);
#7703=VECTOR('',#56713,10.);
#7704=VECTOR('',#56714,10.);
#7705=VECTOR('',#56715,10.);
#7706=VECTOR('',#56716,10.);
#7707=VECTOR('',#56717,10.);
#7708=VECTOR('',#56720,10.);
#7709=VECTOR('',#56721,10.);
#7710=VECTOR('',#56724,10.);
#7711=VECTOR('',#56727,10.);
#7712=VECTOR('',#56728,10.);
#7713=VECTOR('',#56729,10.);
#7714=VECTOR('',#56730,10.);
#7715=VECTOR('',#56731,10.);
#7716=VECTOR('',#56732,10.);
#7717=VECTOR('',#56733,10.);
#7718=VECTOR('',#56734,10.);
#7719=VECTOR('',#56735,10.);
#7720=VECTOR('',#56736,10.);
#7721=VECTOR('',#56737,10.);
#7722=VECTOR('',#56738,10.);
#7723=VECTOR('',#56739,10.);
#7724=VECTOR('',#56740,10.);
#7725=VECTOR('',#56741,10.);
#7726=VECTOR('',#56742,10.);
#7727=VECTOR('',#56743,10.);
#7728=VECTOR('',#56744,10.);
#7729=VECTOR('',#56745,10.);
#7730=VECTOR('',#56746,10.);
#7731=VECTOR('',#56747,10.);
#7732=VECTOR('',#56748,10.);
#7733=VECTOR('',#56749,10.);
#7734=VECTOR('',#56750,10.);
#7735=VECTOR('',#56751,10.);
#7736=VECTOR('',#56752,10.);
#7737=VECTOR('',#56753,10.);
#7738=VECTOR('',#56754,10.);
#7739=VECTOR('',#56755,10.);
#7740=VECTOR('',#56756,10.);
#7741=VECTOR('',#56759,10.);
#7742=VECTOR('',#56760,10.);
#7743=VECTOR('',#56763,10.);
#7744=VECTOR('',#56766,10.);
#7745=VECTOR('',#56767,10.);
#7746=VECTOR('',#56768,10.);
#7747=VECTOR('',#56769,10.);
#7748=VECTOR('',#56770,10.);
#7749=VECTOR('',#56771,10.);
#7750=VECTOR('',#56772,10.);
#7751=VECTOR('',#56773,10.);
#7752=VECTOR('',#56774,10.);
#7753=VECTOR('',#56775,10.);
#7754=VECTOR('',#56776,10.);
#7755=VECTOR('',#56777,10.);
#7756=VECTOR('',#56778,10.);
#7757=VECTOR('',#56779,10.);
#7758=VECTOR('',#56780,10.);
#7759=VECTOR('',#56781,10.);
#7760=VECTOR('',#56782,10.);
#7761=VECTOR('',#56783,10.);
#7762=VECTOR('',#56784,10.);
#7763=VECTOR('',#56785,10.);
#7764=VECTOR('',#56786,10.);
#7765=VECTOR('',#56787,10.);
#7766=VECTOR('',#56788,10.);
#7767=VECTOR('',#56789,10.);
#7768=VECTOR('',#56790,10.);
#7769=VECTOR('',#56791,10.);
#7770=VECTOR('',#56792,10.);
#7771=VECTOR('',#56793,10.);
#7772=VECTOR('',#56794,10.);
#7773=VECTOR('',#56795,10.);
#7774=VECTOR('',#56798,10.);
#7775=VECTOR('',#56799,10.);
#7776=VECTOR('',#56802,10.);
#7777=VECTOR('',#56805,10.);
#7778=VECTOR('',#56806,10.);
#7779=VECTOR('',#56807,10.);
#7780=VECTOR('',#56808,10.);
#7781=VECTOR('',#56809,10.);
#7782=VECTOR('',#56810,10.);
#7783=VECTOR('',#56811,10.);
#7784=VECTOR('',#56812,10.);
#7785=VECTOR('',#56813,10.);
#7786=VECTOR('',#56814,10.);
#7787=VECTOR('',#56815,10.);
#7788=VECTOR('',#56816,10.);
#7789=VECTOR('',#56817,10.);
#7790=VECTOR('',#56818,10.);
#7791=VECTOR('',#56819,10.);
#7792=VECTOR('',#56820,10.);
#7793=VECTOR('',#56821,10.);
#7794=VECTOR('',#56822,10.);
#7795=VECTOR('',#56823,10.);
#7796=VECTOR('',#56824,10.);
#7797=VECTOR('',#56825,10.);
#7798=VECTOR('',#56826,10.);
#7799=VECTOR('',#56827,10.);
#7800=VECTOR('',#56828,10.);
#7801=VECTOR('',#56829,10.);
#7802=VECTOR('',#56830,10.);
#7803=VECTOR('',#56831,10.);
#7804=VECTOR('',#56832,10.);
#7805=VECTOR('',#56833,10.);
#7806=VECTOR('',#56834,10.);
#7807=VECTOR('',#56837,10.);
#7808=VECTOR('',#56838,10.);
#7809=VECTOR('',#56841,10.);
#7810=VECTOR('',#56844,10.);
#7811=VECTOR('',#56845,10.);
#7812=VECTOR('',#56846,10.);
#7813=VECTOR('',#56847,10.);
#7814=VECTOR('',#56848,10.);
#7815=VECTOR('',#56849,10.);
#7816=VECTOR('',#56850,10.);
#7817=VECTOR('',#56851,10.);
#7818=VECTOR('',#56852,10.);
#7819=VECTOR('',#56853,10.);
#7820=VECTOR('',#56854,10.);
#7821=VECTOR('',#56855,10.);
#7822=VECTOR('',#56856,10.);
#7823=VECTOR('',#56857,10.);
#7824=VECTOR('',#56858,10.);
#7825=VECTOR('',#56859,10.);
#7826=VECTOR('',#56860,10.);
#7827=VECTOR('',#56861,10.);
#7828=VECTOR('',#56862,10.);
#7829=VECTOR('',#56863,10.);
#7830=VECTOR('',#56864,10.);
#7831=VECTOR('',#56865,10.);
#7832=VECTOR('',#56866,10.);
#7833=VECTOR('',#56867,10.);
#7834=VECTOR('',#56868,10.);
#7835=VECTOR('',#56869,10.);
#7836=VECTOR('',#56870,10.);
#7837=VECTOR('',#56871,10.);
#7838=VECTOR('',#56872,10.);
#7839=VECTOR('',#56873,10.);
#7840=VECTOR('',#56876,10.);
#7841=VECTOR('',#56877,10.);
#7842=VECTOR('',#56880,10.);
#7843=VECTOR('',#56883,10.);
#7844=VECTOR('',#56884,10.);
#7845=VECTOR('',#56885,10.);
#7846=VECTOR('',#56886,10.);
#7847=VECTOR('',#56887,10.);
#7848=VECTOR('',#56888,10.);
#7849=VECTOR('',#56889,10.);
#7850=VECTOR('',#56890,10.);
#7851=VECTOR('',#56891,10.);
#7852=VECTOR('',#56892,10.);
#7853=VECTOR('',#56893,10.);
#7854=VECTOR('',#56894,10.);
#7855=VECTOR('',#56895,10.);
#7856=VECTOR('',#56896,10.);
#7857=VECTOR('',#56897,10.);
#7858=VECTOR('',#56898,10.);
#7859=VECTOR('',#56899,10.);
#7860=VECTOR('',#56900,10.);
#7861=VECTOR('',#56901,10.);
#7862=VECTOR('',#56902,10.);
#7863=VECTOR('',#56903,10.);
#7864=VECTOR('',#56904,10.);
#7865=VECTOR('',#56905,10.);
#7866=VECTOR('',#56906,10.);
#7867=VECTOR('',#56907,10.);
#7868=VECTOR('',#56908,10.);
#7869=VECTOR('',#56909,10.);
#7870=VECTOR('',#56910,10.);
#7871=VECTOR('',#56911,10.);
#7872=VECTOR('',#56912,10.);
#7873=VECTOR('',#56915,10.);
#7874=VECTOR('',#56916,10.);
#7875=VECTOR('',#56919,10.);
#7876=VECTOR('',#57066,10.);
#7877=VECTOR('',#57067,10.);
#7878=VECTOR('',#57070,10.);
#7879=VECTOR('',#57073,10.);
#7880=VECTOR('',#57074,10.);
#7881=VECTOR('',#57077,10.);
#7882=VECTOR('',#57080,10.);
#7883=VECTOR('',#57081,10.);
#7884=VECTOR('',#57084,10.);
#7885=VECTOR('',#57087,10.);
#7886=VECTOR('',#57088,10.);
#7887=VECTOR('',#57091,10.);
#7888=VECTOR('',#57094,10.);
#7889=VECTOR('',#57095,10.);
#7890=VECTOR('',#57098,10.);
#7891=VECTOR('',#57101,10.);
#7892=VECTOR('',#57102,10.);
#7893=VECTOR('',#57105,10.);
#7894=VECTOR('',#57108,10.);
#7895=VECTOR('',#57109,10.);
#7896=VECTOR('',#57112,10.);
#7897=VECTOR('',#57115,10.);
#7898=VECTOR('',#57116,10.);
#7899=VECTOR('',#57119,10.);
#7900=VECTOR('',#57122,10.);
#7901=VECTOR('',#57123,10.);
#7902=VECTOR('',#57126,10.);
#7903=VECTOR('',#57129,10.);
#7904=VECTOR('',#57130,10.);
#7905=VECTOR('',#57133,10.);
#7906=VECTOR('',#57136,10.);
#7907=VECTOR('',#57137,10.);
#7908=VECTOR('',#57140,10.);
#7909=VECTOR('',#57143,10.);
#7910=VECTOR('',#57144,10.);
#7911=VECTOR('',#57147,10.);
#7912=VECTOR('',#57150,10.);
#7913=VECTOR('',#57151,10.);
#7914=VECTOR('',#57154,10.);
#7915=VECTOR('',#57157,10.);
#7916=VECTOR('',#57158,10.);
#7917=VECTOR('',#57161,10.);
#7918=VECTOR('',#57164,10.);
#7919=VECTOR('',#57165,10.);
#7920=VECTOR('',#57168,10.);
#7921=VECTOR('',#57171,10.);
#7922=VECTOR('',#57172,10.);
#7923=VECTOR('',#57175,10.);
#7924=VECTOR('',#57178,10.);
#7925=VECTOR('',#57179,10.);
#7926=VECTOR('',#57182,10.);
#7927=VECTOR('',#57185,10.);
#7928=VECTOR('',#57186,10.);
#7929=VECTOR('',#57189,10.);
#7930=VECTOR('',#57192,10.);
#7931=VECTOR('',#57193,10.);
#7932=VECTOR('',#57196,10.);
#7933=VECTOR('',#57199,10.);
#7934=VECTOR('',#57200,10.);
#7935=VECTOR('',#57203,10.);
#7936=VECTOR('',#57206,10.);
#7937=VECTOR('',#57207,10.);
#7938=VECTOR('',#57210,10.);
#7939=VECTOR('',#57213,10.);
#7940=VECTOR('',#57214,10.);
#7941=VECTOR('',#57217,10.);
#7942=VECTOR('',#57220,10.);
#7943=VECTOR('',#57221,10.);
#7944=VECTOR('',#57224,10.);
#7945=VECTOR('',#57227,10.);
#7946=VECTOR('',#57228,10.);
#7947=VECTOR('',#57231,10.);
#7948=VECTOR('',#57234,10.);
#7949=VECTOR('',#57235,10.);
#7950=VECTOR('',#57238,10.);
#7951=VECTOR('',#57241,10.);
#7952=VECTOR('',#57242,10.);
#7953=VECTOR('',#57245,10.);
#7954=VECTOR('',#57248,10.);
#7955=VECTOR('',#57249,10.);
#7956=VECTOR('',#57252,10.);
#7957=VECTOR('',#57255,10.);
#7958=VECTOR('',#57256,10.);
#7959=VECTOR('',#57259,10.);
#7960=VECTOR('',#57262,10.);
#7961=VECTOR('',#57263,10.);
#7962=VECTOR('',#57266,10.);
#7963=VECTOR('',#57269,10.);
#7964=VECTOR('',#57270,10.);
#7965=VECTOR('',#57273,10.);
#7966=VECTOR('',#57276,10.);
#7967=VECTOR('',#57277,10.);
#7968=VECTOR('',#57280,10.);
#7969=VECTOR('',#57283,10.);
#7970=VECTOR('',#57284,10.);
#7971=VECTOR('',#57287,10.);
#7972=VECTOR('',#57290,10.);
#7973=VECTOR('',#57291,10.);
#7974=VECTOR('',#57294,10.);
#7975=VECTOR('',#57297,10.);
#7976=VECTOR('',#57298,10.);
#7977=VECTOR('',#57301,10.);
#7978=VECTOR('',#57304,10.);
#7979=VECTOR('',#57305,10.);
#7980=VECTOR('',#57308,10.);
#7981=VECTOR('',#57311,10.);
#7982=VECTOR('',#57312,10.);
#7983=VECTOR('',#57315,10.);
#7984=VECTOR('',#57318,10.);
#7985=VECTOR('',#57319,10.);
#7986=VECTOR('',#57322,10.);
#7987=VECTOR('',#57323,10.);
#7988=VECTOR('',#57326,10.);
#7989=VECTOR('',#57327,10.);
#7990=VECTOR('',#57330,10.);
#7991=VECTOR('',#57331,10.);
#7992=VECTOR('',#57334,10.);
#7993=VECTOR('',#57335,10.);
#7994=VECTOR('',#57338,10.);
#7995=VECTOR('',#57339,10.);
#7996=VECTOR('',#57342,10.);
#7997=VECTOR('',#57343,10.);
#7998=VECTOR('',#57346,10.);
#7999=VECTOR('',#57347,10.);
#8000=VECTOR('',#57350,10.);
#8001=VECTOR('',#57351,10.);
#8002=VECTOR('',#57354,10.);
#8003=VECTOR('',#57355,10.);
#8004=VECTOR('',#57358,10.);
#8005=VECTOR('',#57359,10.);
#8006=VECTOR('',#57362,10.);
#8007=VECTOR('',#57363,10.);
#8008=VECTOR('',#57366,10.);
#8009=VECTOR('',#57367,10.);
#8010=VECTOR('',#57370,10.);
#8011=VECTOR('',#57371,10.);
#8012=VECTOR('',#57374,10.);
#8013=VECTOR('',#57375,10.);
#8014=VECTOR('',#57378,10.);
#8015=VECTOR('',#57379,10.);
#8016=VECTOR('',#57382,10.);
#8017=VECTOR('',#57383,10.);
#8018=VECTOR('',#57386,10.);
#8019=VECTOR('',#57387,10.);
#8020=VECTOR('',#57390,10.);
#8021=VECTOR('',#57391,10.);
#8022=VECTOR('',#57394,10.);
#8023=VECTOR('',#57395,10.);
#8024=VECTOR('',#57398,10.);
#8025=VECTOR('',#57399,10.);
#8026=VECTOR('',#57402,10.);
#8027=VECTOR('',#57403,10.);
#8028=VECTOR('',#57406,10.);
#8029=VECTOR('',#57407,10.);
#8030=VECTOR('',#57410,10.);
#8031=VECTOR('',#57411,10.);
#8032=VECTOR('',#57414,10.);
#8033=VECTOR('',#57415,10.);
#8034=VECTOR('',#57418,10.);
#8035=VECTOR('',#57419,10.);
#8036=VECTOR('',#57422,10.);
#8037=VECTOR('',#57423,10.);
#8038=VECTOR('',#57426,10.);
#8039=VECTOR('',#57427,10.);
#8040=VECTOR('',#57430,10.);
#8041=VECTOR('',#57431,10.);
#8042=VECTOR('',#57434,10.);
#8043=VECTOR('',#57435,10.);
#8044=VECTOR('',#57438,10.);
#8045=VECTOR('',#57439,10.);
#8046=VECTOR('',#57442,10.);
#8047=VECTOR('',#57443,10.);
#8048=VECTOR('',#57446,10.);
#8049=VECTOR('',#57447,10.);
#8050=VECTOR('',#57450,10.);
#8051=VECTOR('',#57451,10.);
#8052=VECTOR('',#57454,10.);
#8053=VECTOR('',#57455,10.);
#8054=VECTOR('',#57458,10.);
#8055=VECTOR('',#57459,10.);
#8056=VECTOR('',#57462,10.);
#8057=VECTOR('',#57465,10.);
#8058=VECTOR('',#57468,10.);
#8059=VECTOR('',#57471,10.);
#8060=VECTOR('',#57474,10.);
#8061=VECTOR('',#57477,10.);
#8062=VECTOR('',#57480,10.);
#8063=VECTOR('',#57483,10.);
#8064=VECTOR('',#57486,10.);
#8065=VECTOR('',#57489,10.);
#8066=VECTOR('',#57492,10.);
#8067=VECTOR('',#57495,10.);
#8068=VECTOR('',#57498,10.);
#8069=VECTOR('',#57501,10.);
#8070=VECTOR('',#57504,10.);
#8071=VECTOR('',#57507,10.);
#8072=VECTOR('',#57510,10.);
#8073=VECTOR('',#57513,10.);
#8074=VECTOR('',#57516,10.);
#8075=VECTOR('',#57519,10.);
#8076=VECTOR('',#57522,10.);
#8077=VECTOR('',#57525,10.);
#8078=VECTOR('',#57528,10.);
#8079=VECTOR('',#57531,10.);
#8080=VECTOR('',#57534,10.);
#8081=VECTOR('',#57537,10.);
#8082=VECTOR('',#57540,10.);
#8083=VECTOR('',#57543,10.);
#8084=VECTOR('',#57546,10.);
#8085=VECTOR('',#57549,10.);
#8086=VECTOR('',#57552,10.);
#8087=VECTOR('',#57555,10.);
#8088=VECTOR('',#57558,10.);
#8089=VECTOR('',#57561,10.);
#8090=VECTOR('',#57564,10.);
#8091=VECTOR('',#57567,10.);
#8092=VECTOR('',#57570,10.);
#8093=VECTOR('',#57573,10.);
#8094=VECTOR('',#57576,10.);
#8095=VECTOR('',#57579,10.);
#8096=VECTOR('',#57582,10.);
#8097=VECTOR('',#57585,10.);
#8098=VECTOR('',#57588,10.);
#8099=VECTOR('',#57591,10.);
#8100=VECTOR('',#57594,10.);
#8101=VECTOR('',#57597,10.);
#8102=VECTOR('',#57600,10.);
#8103=VECTOR('',#57603,10.);
#8104=VECTOR('',#57606,10.);
#8105=VECTOR('',#57609,10.);
#8106=VECTOR('',#57612,10.);
#8107=VECTOR('',#57615,10.);
#8108=VECTOR('',#57618,10.);
#8109=VECTOR('',#57621,10.);
#8110=VECTOR('',#57624,10.);
#8111=VECTOR('',#57627,10.);
#8112=VECTOR('',#57630,10.);
#8113=VECTOR('',#57633,10.);
#8114=VECTOR('',#57636,10.);
#8115=VECTOR('',#57639,10.);
#8116=VECTOR('',#57642,10.);
#8117=VECTOR('',#57645,10.);
#8118=VECTOR('',#57648,10.);
#8119=VECTOR('',#57651,10.);
#8120=VECTOR('',#57654,10.);
#8121=VECTOR('',#57657,10.);
#8122=VECTOR('',#57660,10.);
#8123=VECTOR('',#57663,10.);
#8124=VECTOR('',#57666,10.);
#8125=VECTOR('',#57669,10.);
#8126=VECTOR('',#57672,10.);
#8127=VECTOR('',#57675,10.);
#8128=VECTOR('',#57676,10.);
#8129=VECTOR('',#57679,10.);
#8130=VECTOR('',#57680,10.);
#8131=VECTOR('',#57683,10.);
#8132=VECTOR('',#57684,10.);
#8133=VECTOR('',#57687,10.);
#8134=VECTOR('',#57688,10.);
#8135=VECTOR('',#57691,10.);
#8136=VECTOR('',#57692,10.);
#8137=VECTOR('',#57695,10.);
#8138=VECTOR('',#57696,10.);
#8139=VECTOR('',#57699,10.);
#8140=VECTOR('',#57700,10.);
#8141=VECTOR('',#57703,10.);
#8142=VECTOR('',#57704,10.);
#8143=VECTOR('',#57707,10.);
#8144=VECTOR('',#57708,10.);
#8145=VECTOR('',#57711,10.);
#8146=VECTOR('',#57712,10.);
#8147=VECTOR('',#57715,10.);
#8148=VECTOR('',#57716,10.);
#8149=VECTOR('',#57719,10.);
#8150=VECTOR('',#57720,10.);
#8151=VECTOR('',#57723,10.);
#8152=VECTOR('',#57724,10.);
#8153=VECTOR('',#57727,10.);
#8154=VECTOR('',#57728,10.);
#8155=VECTOR('',#57731,10.);
#8156=VECTOR('',#57732,10.);
#8157=VECTOR('',#57735,10.);
#8158=VECTOR('',#57736,10.);
#8159=VECTOR('',#57739,10.);
#8160=VECTOR('',#57740,10.);
#8161=VECTOR('',#57743,10.);
#8162=VECTOR('',#57744,10.);
#8163=VECTOR('',#57747,10.);
#8164=VECTOR('',#57748,10.);
#8165=VECTOR('',#57751,10.);
#8166=VECTOR('',#57752,10.);
#8167=VECTOR('',#57755,10.);
#8168=VECTOR('',#57756,10.);
#8169=VECTOR('',#57759,10.);
#8170=VECTOR('',#57760,10.);
#8171=VECTOR('',#57763,10.);
#8172=VECTOR('',#57764,10.);
#8173=VECTOR('',#57767,10.);
#8174=VECTOR('',#57768,10.);
#8175=VECTOR('',#57771,10.);
#8176=VECTOR('',#57772,10.);
#8177=VECTOR('',#57775,10.);
#8178=VECTOR('',#57776,10.);
#8179=VECTOR('',#57779,10.);
#8180=VECTOR('',#57780,10.);
#8181=VECTOR('',#57783,10.);
#8182=VECTOR('',#57784,10.);
#8183=VECTOR('',#57787,10.);
#8184=VECTOR('',#57788,10.);
#8185=VECTOR('',#57791,10.);
#8186=VECTOR('',#57792,10.);
#8187=VECTOR('',#57795,10.);
#8188=VECTOR('',#57796,10.);
#8189=VECTOR('',#57799,10.);
#8190=VECTOR('',#57800,10.);
#8191=VECTOR('',#57803,10.);
#8192=VECTOR('',#57804,10.);
#8193=VECTOR('',#57807,10.);
#8194=VECTOR('',#57808,10.);
#8195=VECTOR('',#57811,10.);
#8196=VECTOR('',#57812,10.);
#8197=VECTOR('',#57815,10.);
#8198=VECTOR('',#57816,10.);
#8199=VECTOR('',#57819,10.);
#8200=VECTOR('',#57822,10.);
#8201=VECTOR('',#57825,10.);
#8202=VECTOR('',#57828,10.);
#8203=VECTOR('',#57831,10.);
#8204=VECTOR('',#57834,10.);
#8205=VECTOR('',#57837,10.);
#8206=VECTOR('',#57840,10.);
#8207=VECTOR('',#57843,10.);
#8208=VECTOR('',#57846,10.);
#8209=VECTOR('',#57849,10.);
#8210=VECTOR('',#57852,10.);
#8211=VECTOR('',#57855,10.);
#8212=VECTOR('',#57858,10.);
#8213=VECTOR('',#57861,10.);
#8214=VECTOR('',#57864,10.);
#8215=VECTOR('',#57867,10.);
#8216=VECTOR('',#57870,10.);
#8217=VECTOR('',#57873,10.);
#8218=VECTOR('',#57876,10.);
#8219=VECTOR('',#57879,10.);
#8220=VECTOR('',#57882,10.);
#8221=VECTOR('',#57885,10.);
#8222=VECTOR('',#57888,10.);
#8223=VECTOR('',#57891,10.);
#8224=VECTOR('',#57894,10.);
#8225=VECTOR('',#57897,10.);
#8226=VECTOR('',#57900,10.);
#8227=VECTOR('',#57903,10.);
#8228=VECTOR('',#57906,10.);
#8229=VECTOR('',#57909,10.);
#8230=VECTOR('',#57912,10.);
#8231=VECTOR('',#57915,10.);
#8232=VECTOR('',#57918,10.);
#8233=VECTOR('',#57921,10.);
#8234=VECTOR('',#57924,10.);
#8235=VECTOR('',#57927,10.);
#8236=VECTOR('',#57928,10.);
#8237=VECTOR('',#57933,10.);
#8238=VECTOR('',#57938,10.);
#8239=VECTOR('',#57943,10.);
#8240=VECTOR('',#57948,10.);
#8241=VECTOR('',#57953,10.);
#8242=VECTOR('',#57956,10.);
#8243=VECTOR('',#57957,10.);
#8244=VECTOR('',#57962,10.);
#8245=VECTOR('',#57967,10.);
#8246=VECTOR('',#57972,10.);
#8247=VECTOR('',#57977,10.);
#8248=VECTOR('',#57982,10.);
#8249=VECTOR('',#57985,10.);
#8250=VECTOR('',#57986,10.);
#8251=VECTOR('',#57993,10.);
#8252=VECTOR('',#57994,10.);
#8253=VECTOR('',#57999,10.);
#8254=VECTOR('',#58004,10.);
#8255=VECTOR('',#58009,10.);
#8256=VECTOR('',#58014,10.);
#8257=VECTOR('',#58019,10.);
#8258=VECTOR('',#58022,10.);
#8259=VECTOR('',#58023,10.);
#8260=VECTOR('',#58028,10.);
#8261=VECTOR('',#58033,10.);
#8262=VECTOR('',#58038,10.);
#8263=VECTOR('',#58043,10.);
#8264=VECTOR('',#58048,10.);
#8265=VECTOR('',#58051,10.);
#8266=VECTOR('',#58058,42.6);
#8267=VECTOR('',#58137,10.);
#8268=VECTOR('',#58148,10.);
#8269=VECTOR('',#58159,10.);
#8270=VECTOR('',#58162,10.);
#8271=VECTOR('',#58165,10.);
#8272=VECTOR('',#58168,10.);
#8273=VECTOR('',#58171,10.);
#8274=VECTOR('',#58174,10.);
#8275=VECTOR('',#58177,10.);
#8276=VECTOR('',#58180,10.);
#8277=VECTOR('',#58183,10.);
#8278=VECTOR('',#58186,10.);
#8279=VECTOR('',#58189,10.);
#8280=VECTOR('',#58192,10.);
#8281=VECTOR('',#58195,10.);
#8282=VECTOR('',#58198,10.);
#8283=VECTOR('',#58203,10.);
#8284=VECTOR('',#58204,10.);
#8285=VECTOR('',#58209,10.);
#8286=VECTOR('',#58214,10.);
#8287=VECTOR('',#58219,10.);
#8288=VECTOR('',#58224,10.);
#8289=VECTOR('',#58229,10.);
#8290=VECTOR('',#58232,10.);
#8291=VECTOR('',#58233,10.);
#8292=VECTOR('',#58238,10.);
#8293=VECTOR('',#58243,10.);
#8294=VECTOR('',#58248,10.);
#8295=VECTOR('',#58253,10.);
#8296=VECTOR('',#58258,10.);
#8297=VECTOR('',#58261,10.);
#8298=VECTOR('',#58270,10.);
#8299=VECTOR('',#58281,10.);
#8300=VECTOR('',#58292,10.);
#8301=VECTOR('',#58295,10.);
#8302=VECTOR('',#58298,10.);
#8303=VECTOR('',#58301,10.);
#8304=VECTOR('',#58304,10.);
#8305=VECTOR('',#58307,10.);
#8306=VECTOR('',#58310,10.);
#8307=VECTOR('',#58313,10.);
#8308=VECTOR('',#58316,10.);
#8309=VECTOR('',#58319,10.);
#8310=VECTOR('',#58322,10.);
#8311=VECTOR('',#58325,10.);
#8312=VECTOR('',#58328,10.);
#8313=VECTOR('',#58331,10.);
#8314=VECTOR('',#58336,10.);
#8315=VECTOR('',#58337,10.);
#8316=VECTOR('',#58342,10.);
#8317=VECTOR('',#58347,10.);
#8318=VECTOR('',#58352,10.);
#8319=VECTOR('',#58357,10.);
#8320=VECTOR('',#58362,10.);
#8321=VECTOR('',#58365,10.);
#8322=VECTOR('',#58366,10.);
#8323=VECTOR('',#58371,10.);
#8324=VECTOR('',#58376,10.);
#8325=VECTOR('',#58381,10.);
#8326=VECTOR('',#58386,10.);
#8327=VECTOR('',#58391,10.);
#8328=VECTOR('',#58394,10.);
#8329=VECTOR('',#58403,10.);
#8330=VECTOR('',#58414,10.);
#8331=VECTOR('',#58425,10.);
#8332=VECTOR('',#58428,10.);
#8333=VECTOR('',#58431,10.);
#8334=VECTOR('',#58434,10.);
#8335=VECTOR('',#58437,10.);
#8336=VECTOR('',#58440,10.);
#8337=VECTOR('',#58443,10.);
#8338=VECTOR('',#58446,10.);
#8339=VECTOR('',#58449,10.);
#8340=VECTOR('',#58452,10.);
#8341=VECTOR('',#58455,10.);
#8342=VECTOR('',#58458,10.);
#8343=VECTOR('',#58461,10.);
#8344=VECTOR('',#58464,10.);
#8345=VECTOR('',#58469,10.);
#8346=VECTOR('',#58470,10.);
#8347=VECTOR('',#58475,10.);
#8348=VECTOR('',#58480,10.);
#8349=VECTOR('',#58485,10.);
#8350=VECTOR('',#58490,10.);
#8351=VECTOR('',#58495,10.);
#8352=VECTOR('',#58498,10.);
#8353=VECTOR('',#58499,10.);
#8354=VECTOR('',#58504,10.);
#8355=VECTOR('',#58509,10.);
#8356=VECTOR('',#58514,10.);
#8357=VECTOR('',#58519,10.);
#8358=VECTOR('',#58524,10.);
#8359=VECTOR('',#58527,10.);
#8360=VECTOR('',#58536,10.);
#8361=VECTOR('',#58547,10.);
#8362=VECTOR('',#58558,10.);
#8363=VECTOR('',#58561,10.);
#8364=VECTOR('',#58564,10.);
#8365=VECTOR('',#58567,10.);
#8366=VECTOR('',#58570,10.);
#8367=VECTOR('',#58573,10.);
#8368=VECTOR('',#58576,10.);
#8369=VECTOR('',#58579,10.);
#8370=VECTOR('',#58582,10.);
#8371=VECTOR('',#58585,10.);
#8372=VECTOR('',#58588,10.);
#8373=VECTOR('',#58591,10.);
#8374=VECTOR('',#58594,10.);
#8375=VECTOR('',#58597,10.);
#8376=VECTOR('',#58602,10.);
#8377=VECTOR('',#58603,10.);
#8378=VECTOR('',#58608,10.);
#8379=VECTOR('',#58613,10.);
#8380=VECTOR('',#58618,10.);
#8381=VECTOR('',#58623,10.);
#8382=VECTOR('',#58628,10.);
#8383=VECTOR('',#58631,10.);
#8384=VECTOR('',#58632,10.);
#8385=VECTOR('',#58637,10.);
#8386=VECTOR('',#58642,10.);
#8387=VECTOR('',#58647,10.);
#8388=VECTOR('',#58652,10.);
#8389=VECTOR('',#58657,10.);
#8390=VECTOR('',#58660,10.);
#8391=VECTOR('',#58669,10.);
#8392=VECTOR('',#58680,10.);
#8393=VECTOR('',#58691,10.);
#8394=VECTOR('',#58694,10.);
#8395=VECTOR('',#58697,10.);
#8396=VECTOR('',#58700,10.);
#8397=VECTOR('',#58703,10.);
#8398=VECTOR('',#58706,10.);
#8399=VECTOR('',#58709,10.);
#8400=VECTOR('',#58712,10.);
#8401=VECTOR('',#58715,10.);
#8402=VECTOR('',#58718,10.);
#8403=VECTOR('',#58721,10.);
#8404=VECTOR('',#58724,10.);
#8405=VECTOR('',#58727,10.);
#8406=VECTOR('',#58730,10.);
#8407=VECTOR('',#58735,10.);
#8408=VECTOR('',#58736,10.);
#8409=VECTOR('',#58741,10.);
#8410=VECTOR('',#58746,10.);
#8411=VECTOR('',#58751,10.);
#8412=VECTOR('',#58756,10.);
#8413=VECTOR('',#58761,10.);
#8414=VECTOR('',#58764,10.);
#8415=VECTOR('',#58765,10.);
#8416=VECTOR('',#58770,10.);
#8417=VECTOR('',#58775,10.);
#8418=VECTOR('',#58780,10.);
#8419=VECTOR('',#58785,10.);
#8420=VECTOR('',#58790,10.);
#8421=VECTOR('',#58793,10.);
#8422=VECTOR('',#58802,10.);
#8423=VECTOR('',#58813,10.);
#8424=VECTOR('',#58824,10.);
#8425=VECTOR('',#58827,10.);
#8426=VECTOR('',#58830,10.);
#8427=VECTOR('',#58833,10.);
#8428=VECTOR('',#58836,10.);
#8429=VECTOR('',#58839,10.);
#8430=VECTOR('',#58842,10.);
#8431=VECTOR('',#58845,10.);
#8432=VECTOR('',#58848,10.);
#8433=VECTOR('',#58851,10.);
#8434=VECTOR('',#58854,10.);
#8435=VECTOR('',#58857,10.);
#8436=VECTOR('',#58860,10.);
#8437=VECTOR('',#58863,10.);
#8438=VECTOR('',#58868,10.);
#8439=VECTOR('',#58869,10.);
#8440=VECTOR('',#58874,10.);
#8441=VECTOR('',#58879,10.);
#8442=VECTOR('',#58884,10.);
#8443=VECTOR('',#58889,10.);
#8444=VECTOR('',#58894,10.);
#8445=VECTOR('',#58897,10.);
#8446=VECTOR('',#58898,10.);
#8447=VECTOR('',#58903,10.);
#8448=VECTOR('',#58908,10.);
#8449=VECTOR('',#58913,10.);
#8450=VECTOR('',#58918,10.);
#8451=VECTOR('',#58923,10.);
#8452=VECTOR('',#58926,10.);
#8453=VECTOR('',#58935,10.);
#8454=VECTOR('',#58946,10.);
#8455=VECTOR('',#58957,10.);
#8456=VECTOR('',#58960,10.);
#8457=VECTOR('',#58963,10.);
#8458=VECTOR('',#58966,10.);
#8459=VECTOR('',#58969,10.);
#8460=VECTOR('',#58972,10.);
#8461=VECTOR('',#58975,10.);
#8462=VECTOR('',#58978,10.);
#8463=VECTOR('',#58981,10.);
#8464=VECTOR('',#58984,10.);
#8465=VECTOR('',#58987,10.);
#8466=VECTOR('',#58990,10.);
#8467=VECTOR('',#58993,10.);
#8468=VECTOR('',#58996,10.);
#8469=VECTOR('',#59001,10.);
#8470=VECTOR('',#59002,10.);
#8471=VECTOR('',#59007,10.);
#8472=VECTOR('',#59012,10.);
#8473=VECTOR('',#59017,10.);
#8474=VECTOR('',#59022,10.);
#8475=VECTOR('',#59027,10.);
#8476=VECTOR('',#59030,10.);
#8477=VECTOR('',#59031,10.);
#8478=VECTOR('',#59036,10.);
#8479=VECTOR('',#59041,10.);
#8480=VECTOR('',#59046,10.);
#8481=VECTOR('',#59051,10.);
#8482=VECTOR('',#59056,10.);
#8483=VECTOR('',#59059,10.);
#8484=VECTOR('',#59068,10.);
#8485=VECTOR('',#59079,10.);
#8486=VECTOR('',#59090,10.);
#8487=VECTOR('',#59093,10.);
#8488=VECTOR('',#59096,10.);
#8489=VECTOR('',#59099,10.);
#8490=VECTOR('',#59102,10.);
#8491=VECTOR('',#59105,10.);
#8492=VECTOR('',#59108,10.);
#8493=VECTOR('',#59111,10.);
#8494=VECTOR('',#59114,10.);
#8495=VECTOR('',#59117,10.);
#8496=VECTOR('',#59120,10.);
#8497=VECTOR('',#59123,10.);
#8498=VECTOR('',#59126,10.);
#8499=VECTOR('',#59129,10.);
#8500=VECTOR('',#59134,10.);
#8501=VECTOR('',#59135,10.);
#8502=VECTOR('',#59140,10.);
#8503=VECTOR('',#59145,10.);
#8504=VECTOR('',#59150,10.);
#8505=VECTOR('',#59155,10.);
#8506=VECTOR('',#59160,10.);
#8507=VECTOR('',#59163,10.);
#8508=VECTOR('',#59164,10.);
#8509=VECTOR('',#59169,10.);
#8510=VECTOR('',#59174,10.);
#8511=VECTOR('',#59179,10.);
#8512=VECTOR('',#59184,10.);
#8513=VECTOR('',#59189,10.);
#8514=VECTOR('',#59192,10.);
#8515=VECTOR('',#59201,10.);
#8516=VECTOR('',#59212,10.);
#8517=VECTOR('',#59223,10.);
#8518=VECTOR('',#59226,10.);
#8519=VECTOR('',#59229,10.);
#8520=VECTOR('',#59232,10.);
#8521=VECTOR('',#59235,10.);
#8522=VECTOR('',#59238,10.);
#8523=VECTOR('',#59241,10.);
#8524=VECTOR('',#59244,10.);
#8525=VECTOR('',#59247,10.);
#8526=VECTOR('',#59250,10.);
#8527=VECTOR('',#59253,10.);
#8528=VECTOR('',#59256,10.);
#8529=VECTOR('',#59259,10.);
#8530=VECTOR('',#59262,10.);
#8531=VECTOR('',#59267,10.);
#8532=VECTOR('',#59268,10.);
#8533=VECTOR('',#59273,10.);
#8534=VECTOR('',#59278,10.);
#8535=VECTOR('',#59283,10.);
#8536=VECTOR('',#59288,10.);
#8537=VECTOR('',#59293,10.);
#8538=VECTOR('',#59296,10.);
#8539=VECTOR('',#59297,10.);
#8540=VECTOR('',#59302,10.);
#8541=VECTOR('',#59307,10.);
#8542=VECTOR('',#59312,10.);
#8543=VECTOR('',#59317,10.);
#8544=VECTOR('',#59322,10.);
#8545=VECTOR('',#59325,10.);
#8546=VECTOR('',#59334,10.);
#8547=VECTOR('',#59345,10.);
#8548=VECTOR('',#59356,10.);
#8549=VECTOR('',#59359,10.);
#8550=VECTOR('',#59362,10.);
#8551=VECTOR('',#59365,10.);
#8552=VECTOR('',#59368,10.);
#8553=VECTOR('',#59371,10.);
#8554=VECTOR('',#59374,10.);
#8555=VECTOR('',#59377,10.);
#8556=VECTOR('',#59380,10.);
#8557=VECTOR('',#59383,10.);
#8558=VECTOR('',#59386,10.);
#8559=VECTOR('',#59389,10.);
#8560=VECTOR('',#59392,10.);
#8561=VECTOR('',#59395,10.);
#8562=VECTOR('',#59400,10.);
#8563=VECTOR('',#59401,10.);
#8564=VECTOR('',#59406,10.);
#8565=VECTOR('',#59411,10.);
#8566=VECTOR('',#59416,10.);
#8567=VECTOR('',#59421,10.);
#8568=VECTOR('',#59426,10.);
#8569=VECTOR('',#59429,10.);
#8570=VECTOR('',#59430,10.);
#8571=VECTOR('',#59435,10.);
#8572=VECTOR('',#59440,10.);
#8573=VECTOR('',#59445,10.);
#8574=VECTOR('',#59450,10.);
#8575=VECTOR('',#59455,10.);
#8576=VECTOR('',#59458,10.);
#8577=VECTOR('',#59467,10.);
#8578=VECTOR('',#59478,10.);
#8579=VECTOR('',#59489,10.);
#8580=VECTOR('',#59492,10.);
#8581=VECTOR('',#59495,10.);
#8582=VECTOR('',#59498,10.);
#8583=VECTOR('',#59501,10.);
#8584=VECTOR('',#59504,10.);
#8585=VECTOR('',#59507,10.);
#8586=VECTOR('',#59510,10.);
#8587=VECTOR('',#59513,10.);
#8588=VECTOR('',#59516,10.);
#8589=VECTOR('',#59519,10.);
#8590=VECTOR('',#59522,10.);
#8591=VECTOR('',#59525,10.);
#8592=VECTOR('',#59528,10.);
#8593=VECTOR('',#59533,10.);
#8594=VECTOR('',#59534,10.);
#8595=VECTOR('',#59539,10.);
#8596=VECTOR('',#59544,10.);
#8597=VECTOR('',#59549,10.);
#8598=VECTOR('',#59554,10.);
#8599=VECTOR('',#59559,10.);
#8600=VECTOR('',#59562,10.);
#8601=VECTOR('',#59563,10.);
#8602=VECTOR('',#59568,10.);
#8603=VECTOR('',#59573,10.);
#8604=VECTOR('',#59578,10.);
#8605=VECTOR('',#59583,10.);
#8606=VECTOR('',#59588,10.);
#8607=VECTOR('',#59591,10.);
#8608=VECTOR('',#59600,10.);
#8609=VECTOR('',#59611,10.);
#8610=VECTOR('',#59622,10.);
#8611=VECTOR('',#59625,10.);
#8612=VECTOR('',#59628,10.);
#8613=VECTOR('',#59631,10.);
#8614=VECTOR('',#59634,10.);
#8615=VECTOR('',#59637,10.);
#8616=VECTOR('',#59640,10.);
#8617=VECTOR('',#59643,10.);
#8618=VECTOR('',#59646,10.);
#8619=VECTOR('',#59649,10.);
#8620=VECTOR('',#59652,10.);
#8621=VECTOR('',#59655,10.);
#8622=VECTOR('',#59658,10.);
#8623=VECTOR('',#59661,10.);
#8624=VECTOR('',#59666,10.);
#8625=VECTOR('',#59667,10.);
#8626=VECTOR('',#59672,10.);
#8627=VECTOR('',#59677,10.);
#8628=VECTOR('',#59682,10.);
#8629=VECTOR('',#59687,10.);
#8630=VECTOR('',#59692,10.);
#8631=VECTOR('',#59695,10.);
#8632=VECTOR('',#59696,10.);
#8633=VECTOR('',#59701,10.);
#8634=VECTOR('',#59706,10.);
#8635=VECTOR('',#59711,10.);
#8636=VECTOR('',#59716,10.);
#8637=VECTOR('',#59721,10.);
#8638=VECTOR('',#59724,10.);
#8639=VECTOR('',#59733,10.);
#8640=VECTOR('',#59744,10.);
#8641=VECTOR('',#59755,10.);
#8642=VECTOR('',#59758,10.);
#8643=VECTOR('',#59761,10.);
#8644=VECTOR('',#59764,10.);
#8645=VECTOR('',#59767,10.);
#8646=VECTOR('',#59770,10.);
#8647=VECTOR('',#59773,10.);
#8648=VECTOR('',#59776,10.);
#8649=VECTOR('',#59779,10.);
#8650=VECTOR('',#59782,10.);
#8651=VECTOR('',#59785,10.);
#8652=VECTOR('',#59788,10.);
#8653=VECTOR('',#59791,10.);
#8654=VECTOR('',#59794,10.);
#8655=VECTOR('',#59799,10.);
#8656=VECTOR('',#59800,10.);
#8657=VECTOR('',#59805,10.);
#8658=VECTOR('',#59810,10.);
#8659=VECTOR('',#59815,10.);
#8660=VECTOR('',#59820,10.);
#8661=VECTOR('',#59825,10.);
#8662=VECTOR('',#59828,10.);
#8663=VECTOR('',#59829,10.);
#8664=VECTOR('',#59834,10.);
#8665=VECTOR('',#59839,10.);
#8666=VECTOR('',#59844,10.);
#8667=VECTOR('',#59849,10.);
#8668=VECTOR('',#59854,10.);
#8669=VECTOR('',#59857,10.);
#8670=VECTOR('',#59866,10.);
#8671=VECTOR('',#59877,10.);
#8672=VECTOR('',#59888,10.);
#8673=VECTOR('',#59891,10.);
#8674=VECTOR('',#59894,10.);
#8675=VECTOR('',#59897,10.);
#8676=VECTOR('',#59900,10.);
#8677=VECTOR('',#59903,10.);
#8678=VECTOR('',#59906,10.);
#8679=VECTOR('',#59909,10.);
#8680=VECTOR('',#59912,10.);
#8681=VECTOR('',#59915,10.);
#8682=VECTOR('',#59918,10.);
#8683=VECTOR('',#59921,10.);
#8684=VECTOR('',#59924,10.);
#8685=VECTOR('',#59927,10.);
#8686=VECTOR('',#59932,10.);
#8687=VECTOR('',#59933,10.);
#8688=VECTOR('',#59938,10.);
#8689=VECTOR('',#59943,10.);
#8690=VECTOR('',#59948,10.);
#8691=VECTOR('',#59953,10.);
#8692=VECTOR('',#59958,10.);
#8693=VECTOR('',#59961,10.);
#8694=VECTOR('',#59962,10.);
#8695=VECTOR('',#59967,10.);
#8696=VECTOR('',#59972,10.);
#8697=VECTOR('',#59977,10.);
#8698=VECTOR('',#59982,10.);
#8699=VECTOR('',#59987,10.);
#8700=VECTOR('',#59990,10.);
#8701=VECTOR('',#59999,10.);
#8702=VECTOR('',#60010,10.);
#8703=VECTOR('',#60021,10.);
#8704=VECTOR('',#60024,10.);
#8705=VECTOR('',#60027,10.);
#8706=VECTOR('',#60030,10.);
#8707=VECTOR('',#60033,10.);
#8708=VECTOR('',#60036,10.);
#8709=VECTOR('',#60039,10.);
#8710=VECTOR('',#60042,10.);
#8711=VECTOR('',#60045,10.);
#8712=VECTOR('',#60048,10.);
#8713=VECTOR('',#60051,10.);
#8714=VECTOR('',#60054,10.);
#8715=VECTOR('',#60057,10.);
#8716=VECTOR('',#60060,10.);
#8717=VECTOR('',#60065,10.);
#8718=VECTOR('',#60066,10.);
#8719=VECTOR('',#60071,10.);
#8720=VECTOR('',#60076,10.);
#8721=VECTOR('',#60081,10.);
#8722=VECTOR('',#60086,10.);
#8723=VECTOR('',#60091,10.);
#8724=VECTOR('',#60094,10.);
#8725=VECTOR('',#60095,10.);
#8726=VECTOR('',#60100,10.);
#8727=VECTOR('',#60105,10.);
#8728=VECTOR('',#60110,10.);
#8729=VECTOR('',#60115,10.);
#8730=VECTOR('',#60120,10.);
#8731=VECTOR('',#60123,10.);
#8732=VECTOR('',#60132,10.);
#8733=VECTOR('',#60143,10.);
#8734=VECTOR('',#60154,10.);
#8735=VECTOR('',#60157,10.);
#8736=VECTOR('',#60160,10.);
#8737=VECTOR('',#60163,10.);
#8738=VECTOR('',#60166,10.);
#8739=VECTOR('',#60169,10.);
#8740=VECTOR('',#60172,10.);
#8741=VECTOR('',#60175,10.);
#8742=VECTOR('',#60178,10.);
#8743=VECTOR('',#60181,10.);
#8744=VECTOR('',#60184,10.);
#8745=VECTOR('',#60187,10.);
#8746=VECTOR('',#60190,10.);
#8747=VECTOR('',#60193,10.);
#8748=VECTOR('',#60198,10.);
#8749=VECTOR('',#60199,10.);
#8750=VECTOR('',#60204,10.);
#8751=VECTOR('',#60209,10.);
#8752=VECTOR('',#60214,10.);
#8753=VECTOR('',#60219,10.);
#8754=VECTOR('',#60224,10.);
#8755=VECTOR('',#60227,10.);
#8756=VECTOR('',#60228,10.);
#8757=VECTOR('',#60233,10.);
#8758=VECTOR('',#60238,10.);
#8759=VECTOR('',#60243,10.);
#8760=VECTOR('',#60248,10.);
#8761=VECTOR('',#60253,10.);
#8762=VECTOR('',#60256,10.);
#8763=VECTOR('',#60265,10.);
#8764=VECTOR('',#60276,10.);
#8765=VECTOR('',#60287,10.);
#8766=VECTOR('',#60290,10.);
#8767=VECTOR('',#60293,10.);
#8768=VECTOR('',#60296,10.);
#8769=VECTOR('',#60299,10.);
#8770=VECTOR('',#60302,10.);
#8771=VECTOR('',#60305,10.);
#8772=VECTOR('',#60308,10.);
#8773=VECTOR('',#60311,10.);
#8774=VECTOR('',#60314,10.);
#8775=VECTOR('',#60317,10.);
#8776=VECTOR('',#60320,10.);
#8777=VECTOR('',#60323,10.);
#8778=VECTOR('',#60326,10.);
#8779=VECTOR('',#60331,10.);
#8780=VECTOR('',#60332,10.);
#8781=VECTOR('',#60337,10.);
#8782=VECTOR('',#60342,10.);
#8783=VECTOR('',#60347,10.);
#8784=VECTOR('',#60352,10.);
#8785=VECTOR('',#60357,10.);
#8786=VECTOR('',#60360,10.);
#8787=VECTOR('',#60361,10.);
#8788=VECTOR('',#60366,10.);
#8789=VECTOR('',#60371,10.);
#8790=VECTOR('',#60376,10.);
#8791=VECTOR('',#60381,10.);
#8792=VECTOR('',#60386,10.);
#8793=VECTOR('',#60389,10.);
#8794=VECTOR('',#60398,10.);
#8795=VECTOR('',#60409,10.);
#8796=VECTOR('',#60420,10.);
#8797=VECTOR('',#60423,10.);
#8798=VECTOR('',#60426,10.);
#8799=VECTOR('',#60429,10.);
#8800=VECTOR('',#60432,10.);
#8801=VECTOR('',#60435,10.);
#8802=VECTOR('',#60438,10.);
#8803=VECTOR('',#60441,10.);
#8804=VECTOR('',#60444,10.);
#8805=VECTOR('',#60447,10.);
#8806=VECTOR('',#60450,10.);
#8807=VECTOR('',#60453,10.);
#8808=VECTOR('',#60456,10.);
#8809=VECTOR('',#60459,10.);
#8810=VECTOR('',#60464,10.);
#8811=VECTOR('',#60465,10.);
#8812=VECTOR('',#60470,10.);
#8813=VECTOR('',#60475,10.);
#8814=VECTOR('',#60480,10.);
#8815=VECTOR('',#60485,10.);
#8816=VECTOR('',#60490,10.);
#8817=VECTOR('',#60493,10.);
#8818=VECTOR('',#60494,10.);
#8819=VECTOR('',#60499,10.);
#8820=VECTOR('',#60504,10.);
#8821=VECTOR('',#60509,10.);
#8822=VECTOR('',#60514,10.);
#8823=VECTOR('',#60519,10.);
#8824=VECTOR('',#60522,10.);
#8825=VECTOR('',#60531,10.);
#8826=VECTOR('',#60542,10.);
#8827=VECTOR('',#60553,10.);
#8828=VECTOR('',#60556,10.);
#8829=VECTOR('',#60559,10.);
#8830=VECTOR('',#60562,10.);
#8831=VECTOR('',#60565,10.);
#8832=VECTOR('',#60568,10.);
#8833=VECTOR('',#60571,10.);
#8834=VECTOR('',#60574,10.);
#8835=VECTOR('',#60577,10.);
#8836=VECTOR('',#60580,10.);
#8837=VECTOR('',#60583,10.);
#8838=VECTOR('',#60586,10.);
#8839=VECTOR('',#60589,10.);
#8840=VECTOR('',#60592,10.);
#8841=VECTOR('',#60597,10.);
#8842=VECTOR('',#60598,10.);
#8843=VECTOR('',#60603,10.);
#8844=VECTOR('',#60608,10.);
#8845=VECTOR('',#60613,10.);
#8846=VECTOR('',#60618,10.);
#8847=VECTOR('',#60623,10.);
#8848=VECTOR('',#60626,10.);
#8849=VECTOR('',#60627,10.);
#8850=VECTOR('',#60632,10.);
#8851=VECTOR('',#60637,10.);
#8852=VECTOR('',#60642,10.);
#8853=VECTOR('',#60647,10.);
#8854=VECTOR('',#60652,10.);
#8855=VECTOR('',#60655,10.);
#8856=VECTOR('',#60664,10.);
#8857=VECTOR('',#60675,10.);
#8858=VECTOR('',#60686,10.);
#8859=VECTOR('',#60689,10.);
#8860=VECTOR('',#60692,10.);
#8861=VECTOR('',#60695,10.);
#8862=VECTOR('',#60698,10.);
#8863=VECTOR('',#60701,10.);
#8864=VECTOR('',#60704,10.);
#8865=VECTOR('',#60707,10.);
#8866=VECTOR('',#60710,10.);
#8867=VECTOR('',#60713,10.);
#8868=VECTOR('',#60716,10.);
#8869=VECTOR('',#60719,10.);
#8870=VECTOR('',#60722,10.);
#8871=VECTOR('',#60725,10.);
#8872=VECTOR('',#60730,10.);
#8873=VECTOR('',#60731,10.);
#8874=VECTOR('',#60736,10.);
#8875=VECTOR('',#60741,10.);
#8876=VECTOR('',#60746,10.);
#8877=VECTOR('',#60751,10.);
#8878=VECTOR('',#60756,10.);
#8879=VECTOR('',#60759,10.);
#8880=VECTOR('',#60760,10.);
#8881=VECTOR('',#60765,10.);
#8882=VECTOR('',#60770,10.);
#8883=VECTOR('',#60775,10.);
#8884=VECTOR('',#60780,10.);
#8885=VECTOR('',#60785,10.);
#8886=VECTOR('',#60788,10.);
#8887=VECTOR('',#60797,10.);
#8888=VECTOR('',#60808,10.);
#8889=VECTOR('',#60819,10.);
#8890=VECTOR('',#60822,10.);
#8891=VECTOR('',#60825,10.);
#8892=VECTOR('',#60828,10.);
#8893=VECTOR('',#60831,10.);
#8894=VECTOR('',#60834,10.);
#8895=VECTOR('',#60837,10.);
#8896=VECTOR('',#60840,10.);
#8897=VECTOR('',#60843,10.);
#8898=VECTOR('',#60846,10.);
#8899=VECTOR('',#60849,10.);
#8900=VECTOR('',#60852,10.);
#8901=VECTOR('',#60855,10.);
#8902=VECTOR('',#60858,10.);
#8903=VECTOR('',#60863,10.);
#8904=VECTOR('',#60864,10.);
#8905=VECTOR('',#60869,10.);
#8906=VECTOR('',#60874,10.);
#8907=VECTOR('',#60879,10.);
#8908=VECTOR('',#60884,10.);
#8909=VECTOR('',#60889,10.);
#8910=VECTOR('',#60892,10.);
#8911=VECTOR('',#60893,10.);
#8912=VECTOR('',#60898,10.);
#8913=VECTOR('',#60903,10.);
#8914=VECTOR('',#60908,10.);
#8915=VECTOR('',#60913,10.);
#8916=VECTOR('',#60918,10.);
#8917=VECTOR('',#60921,10.);
#8918=VECTOR('',#60930,10.);
#8919=VECTOR('',#60941,10.);
#8920=VECTOR('',#60952,10.);
#8921=VECTOR('',#60955,10.);
#8922=VECTOR('',#60958,10.);
#8923=VECTOR('',#60961,10.);
#8924=VECTOR('',#60964,10.);
#8925=VECTOR('',#60967,10.);
#8926=VECTOR('',#60970,10.);
#8927=VECTOR('',#60973,10.);
#8928=VECTOR('',#60976,10.);
#8929=VECTOR('',#60979,10.);
#8930=VECTOR('',#60982,10.);
#8931=VECTOR('',#60985,10.);
#8932=VECTOR('',#60988,10.);
#8933=VECTOR('',#60991,10.);
#8934=VECTOR('',#60996,10.);
#8935=VECTOR('',#60997,10.);
#8936=VECTOR('',#61002,10.);
#8937=VECTOR('',#61007,10.);
#8938=VECTOR('',#61012,10.);
#8939=VECTOR('',#61017,10.);
#8940=VECTOR('',#61022,10.);
#8941=VECTOR('',#61025,10.);
#8942=VECTOR('',#61026,10.);
#8943=VECTOR('',#61031,10.);
#8944=VECTOR('',#61036,10.);
#8945=VECTOR('',#61041,10.);
#8946=VECTOR('',#61046,10.);
#8947=VECTOR('',#61051,10.);
#8948=VECTOR('',#61054,10.);
#8949=VECTOR('',#61063,10.);
#8950=VECTOR('',#61074,10.);
#8951=VECTOR('',#61085,10.);
#8952=VECTOR('',#61088,10.);
#8953=VECTOR('',#61091,10.);
#8954=VECTOR('',#61094,10.);
#8955=VECTOR('',#61097,10.);
#8956=VECTOR('',#61100,10.);
#8957=VECTOR('',#61103,10.);
#8958=VECTOR('',#61106,10.);
#8959=VECTOR('',#61109,10.);
#8960=VECTOR('',#61112,10.);
#8961=VECTOR('',#61115,10.);
#8962=VECTOR('',#61118,10.);
#8963=VECTOR('',#61121,10.);
#8964=VECTOR('',#61124,10.);
#8965=VECTOR('',#61129,10.);
#8966=VECTOR('',#61130,10.);
#8967=VECTOR('',#61135,10.);
#8968=VECTOR('',#61140,10.);
#8969=VECTOR('',#61145,10.);
#8970=VECTOR('',#61150,10.);
#8971=VECTOR('',#61155,10.);
#8972=VECTOR('',#61158,10.);
#8973=VECTOR('',#61159,10.);
#8974=VECTOR('',#61164,10.);
#8975=VECTOR('',#61169,10.);
#8976=VECTOR('',#61174,10.);
#8977=VECTOR('',#61179,10.);
#8978=VECTOR('',#61184,10.);
#8979=VECTOR('',#61187,10.);
#8980=VECTOR('',#61196,10.);
#8981=VECTOR('',#61207,10.);
#8982=VECTOR('',#61218,10.);
#8983=VECTOR('',#61221,10.);
#8984=VECTOR('',#61224,10.);
#8985=VECTOR('',#61227,10.);
#8986=VECTOR('',#61230,10.);
#8987=VECTOR('',#61233,10.);
#8988=VECTOR('',#61236,10.);
#8989=VECTOR('',#61239,10.);
#8990=VECTOR('',#61242,10.);
#8991=VECTOR('',#61245,10.);
#8992=VECTOR('',#61248,10.);
#8993=VECTOR('',#61251,10.);
#8994=VECTOR('',#61254,10.);
#8995=VECTOR('',#61257,10.);
#8996=VECTOR('',#61262,10.);
#8997=VECTOR('',#61263,10.);
#8998=VECTOR('',#61268,10.);
#8999=VECTOR('',#61273,10.);
#9000=VECTOR('',#61278,10.);
#9001=VECTOR('',#61283,10.);
#9002=VECTOR('',#61288,10.);
#9003=VECTOR('',#61291,10.);
#9004=VECTOR('',#61292,10.);
#9005=VECTOR('',#61297,10.);
#9006=VECTOR('',#61302,10.);
#9007=VECTOR('',#61307,10.);
#9008=VECTOR('',#61312,10.);
#9009=VECTOR('',#61317,10.);
#9010=VECTOR('',#61320,10.);
#9011=VECTOR('',#61329,10.);
#9012=VECTOR('',#61340,10.);
#9013=VECTOR('',#61351,10.);
#9014=VECTOR('',#61354,10.);
#9015=VECTOR('',#61357,10.);
#9016=VECTOR('',#61360,10.);
#9017=VECTOR('',#61363,10.);
#9018=VECTOR('',#61366,10.);
#9019=VECTOR('',#61369,10.);
#9020=VECTOR('',#61372,10.);
#9021=VECTOR('',#61375,10.);
#9022=VECTOR('',#61378,10.);
#9023=VECTOR('',#61381,10.);
#9024=VECTOR('',#61384,10.);
#9025=VECTOR('',#61387,10.);
#9026=VECTOR('',#61390,10.);
#9027=VECTOR('',#61395,10.);
#9028=VECTOR('',#61396,10.);
#9029=VECTOR('',#61401,10.);
#9030=VECTOR('',#61406,10.);
#9031=VECTOR('',#61411,10.);
#9032=VECTOR('',#61416,10.);
#9033=VECTOR('',#61421,10.);
#9034=VECTOR('',#61424,10.);
#9035=VECTOR('',#61425,10.);
#9036=VECTOR('',#61430,10.);
#9037=VECTOR('',#61435,10.);
#9038=VECTOR('',#61440,10.);
#9039=VECTOR('',#61445,10.);
#9040=VECTOR('',#61450,10.);
#9041=VECTOR('',#61453,10.);
#9042=VECTOR('',#61462,10.);
#9043=VECTOR('',#61473,10.);
#9044=VECTOR('',#61484,10.);
#9045=VECTOR('',#61487,10.);
#9046=VECTOR('',#61490,10.);
#9047=VECTOR('',#61493,10.);
#9048=VECTOR('',#61496,10.);
#9049=VECTOR('',#61499,10.);
#9050=VECTOR('',#61502,10.);
#9051=VECTOR('',#61505,10.);
#9052=VECTOR('',#61508,10.);
#9053=VECTOR('',#61511,10.);
#9054=VECTOR('',#61514,10.);
#9055=VECTOR('',#61517,10.);
#9056=VECTOR('',#61520,10.);
#9057=VECTOR('',#61523,10.);
#9058=VECTOR('',#61528,10.);
#9059=VECTOR('',#61529,10.);
#9060=VECTOR('',#61534,10.);
#9061=VECTOR('',#61539,10.);
#9062=VECTOR('',#61544,10.);
#9063=VECTOR('',#61549,10.);
#9064=VECTOR('',#61554,10.);
#9065=VECTOR('',#61557,10.);
#9066=VECTOR('',#61558,10.);
#9067=VECTOR('',#61563,10.);
#9068=VECTOR('',#61568,10.);
#9069=VECTOR('',#61573,10.);
#9070=VECTOR('',#61578,10.);
#9071=VECTOR('',#61583,10.);
#9072=VECTOR('',#61586,10.);
#9073=VECTOR('',#61595,10.);
#9074=VECTOR('',#61606,10.);
#9075=VECTOR('',#61617,10.);
#9076=VECTOR('',#61620,10.);
#9077=VECTOR('',#61623,10.);
#9078=VECTOR('',#61626,10.);
#9079=VECTOR('',#61629,10.);
#9080=VECTOR('',#61632,10.);
#9081=VECTOR('',#61635,10.);
#9082=VECTOR('',#61638,10.);
#9083=VECTOR('',#61641,10.);
#9084=VECTOR('',#61644,10.);
#9085=VECTOR('',#61647,10.);
#9086=VECTOR('',#61650,10.);
#9087=VECTOR('',#61653,10.);
#9088=VECTOR('',#61656,10.);
#9089=VECTOR('',#61661,10.);
#9090=VECTOR('',#61662,10.);
#9091=VECTOR('',#61667,10.);
#9092=VECTOR('',#61672,10.);
#9093=VECTOR('',#61677,10.);
#9094=VECTOR('',#61682,10.);
#9095=VECTOR('',#61687,10.);
#9096=VECTOR('',#61690,10.);
#9097=VECTOR('',#61691,10.);
#9098=VECTOR('',#61696,10.);
#9099=VECTOR('',#61701,10.);
#9100=VECTOR('',#61706,10.);
#9101=VECTOR('',#61711,10.);
#9102=VECTOR('',#61716,10.);
#9103=VECTOR('',#61719,10.);
#9104=VECTOR('',#61728,10.);
#9105=VECTOR('',#61739,10.);
#9106=VECTOR('',#61750,10.);
#9107=VECTOR('',#61753,10.);
#9108=VECTOR('',#61756,10.);
#9109=VECTOR('',#61759,10.);
#9110=VECTOR('',#61762,10.);
#9111=VECTOR('',#61765,10.);
#9112=VECTOR('',#61768,10.);
#9113=VECTOR('',#61771,10.);
#9114=VECTOR('',#61774,10.);
#9115=VECTOR('',#61777,10.);
#9116=VECTOR('',#61780,10.);
#9117=VECTOR('',#61783,10.);
#9118=VECTOR('',#61786,10.);
#9119=VECTOR('',#61789,10.);
#9120=VECTOR('',#61794,10.);
#9121=VECTOR('',#61795,10.);
#9122=VECTOR('',#61800,10.);
#9123=VECTOR('',#61805,10.);
#9124=VECTOR('',#61810,10.);
#9125=VECTOR('',#61815,10.);
#9126=VECTOR('',#61820,10.);
#9127=VECTOR('',#61823,10.);
#9128=VECTOR('',#61824,10.);
#9129=VECTOR('',#61829,10.);
#9130=VECTOR('',#61834,10.);
#9131=VECTOR('',#61839,10.);
#9132=VECTOR('',#61844,10.);
#9133=VECTOR('',#61849,10.);
#9134=VECTOR('',#61852,10.);
#9135=VECTOR('',#61861,10.);
#9136=VECTOR('',#61872,10.);
#9137=VECTOR('',#61883,10.);
#9138=VECTOR('',#61886,10.);
#9139=VECTOR('',#61889,10.);
#9140=VECTOR('',#61892,10.);
#9141=VECTOR('',#61895,10.);
#9142=VECTOR('',#61898,10.);
#9143=VECTOR('',#61901,10.);
#9144=VECTOR('',#61904,10.);
#9145=VECTOR('',#61907,10.);
#9146=VECTOR('',#61910,10.);
#9147=VECTOR('',#61913,10.);
#9148=VECTOR('',#61916,10.);
#9149=VECTOR('',#61919,10.);
#9150=VECTOR('',#61922,10.);
#9151=VECTOR('',#61927,10.);
#9152=VECTOR('',#61928,10.);
#9153=VECTOR('',#61933,10.);
#9154=VECTOR('',#61938,10.);
#9155=VECTOR('',#61943,10.);
#9156=VECTOR('',#61948,10.);
#9157=VECTOR('',#61953,10.);
#9158=VECTOR('',#61956,10.);
#9159=VECTOR('',#61957,10.);
#9160=VECTOR('',#61962,10.);
#9161=VECTOR('',#61967,10.);
#9162=VECTOR('',#61972,10.);
#9163=VECTOR('',#61977,10.);
#9164=VECTOR('',#61982,10.);
#9165=VECTOR('',#61985,10.);
#9166=VECTOR('',#61994,10.);
#9167=VECTOR('',#62005,10.);
#9168=VECTOR('',#62016,10.);
#9169=VECTOR('',#62019,10.);
#9170=VECTOR('',#62022,10.);
#9171=VECTOR('',#62025,10.);
#9172=VECTOR('',#62028,10.);
#9173=VECTOR('',#62031,10.);
#9174=VECTOR('',#62034,10.);
#9175=VECTOR('',#62037,10.);
#9176=VECTOR('',#62040,10.);
#9177=VECTOR('',#62043,10.);
#9178=VECTOR('',#62046,10.);
#9179=VECTOR('',#62049,10.);
#9180=VECTOR('',#62052,10.);
#9181=VECTOR('',#62055,10.);
#9182=VECTOR('',#62060,10.);
#9183=VECTOR('',#62061,10.);
#9184=VECTOR('',#62066,10.);
#9185=VECTOR('',#62071,10.);
#9186=VECTOR('',#62076,10.);
#9187=VECTOR('',#62081,10.);
#9188=VECTOR('',#62086,10.);
#9189=VECTOR('',#62089,10.);
#9190=VECTOR('',#62090,10.);
#9191=VECTOR('',#62095,10.);
#9192=VECTOR('',#62100,10.);
#9193=VECTOR('',#62105,10.);
#9194=VECTOR('',#62110,10.);
#9195=VECTOR('',#62115,10.);
#9196=VECTOR('',#62118,10.);
#9197=VECTOR('',#62127,10.);
#9198=VECTOR('',#62138,10.);
#9199=VECTOR('',#62149,10.);
#9200=VECTOR('',#62152,10.);
#9201=VECTOR('',#62155,10.);
#9202=VECTOR('',#62158,10.);
#9203=VECTOR('',#62161,10.);
#9204=VECTOR('',#62164,10.);
#9205=VECTOR('',#62167,10.);
#9206=VECTOR('',#62170,10.);
#9207=VECTOR('',#62173,10.);
#9208=VECTOR('',#62176,10.);
#9209=VECTOR('',#62179,10.);
#9210=VECTOR('',#62182,10.);
#9211=VECTOR('',#62185,10.);
#9212=VECTOR('',#62188,10.);
#9213=VECTOR('',#62193,10.);
#9214=VECTOR('',#62194,10.);
#9215=VECTOR('',#62199,10.);
#9216=VECTOR('',#62204,10.);
#9217=VECTOR('',#62209,10.);
#9218=VECTOR('',#62214,10.);
#9219=VECTOR('',#62219,10.);
#9220=VECTOR('',#62222,10.);
#9221=VECTOR('',#62223,10.);
#9222=VECTOR('',#62228,10.);
#9223=VECTOR('',#62233,10.);
#9224=VECTOR('',#62238,10.);
#9225=VECTOR('',#62243,10.);
#9226=VECTOR('',#62248,10.);
#9227=VECTOR('',#62251,10.);
#9228=VECTOR('',#62260,10.);
#9229=VECTOR('',#62271,10.);
#9230=VECTOR('',#62282,10.);
#9231=VECTOR('',#62285,10.);
#9232=VECTOR('',#62288,10.);
#9233=VECTOR('',#62291,10.);
#9234=VECTOR('',#62294,10.);
#9235=VECTOR('',#62297,10.);
#9236=VECTOR('',#62300,10.);
#9237=VECTOR('',#62303,10.);
#9238=VECTOR('',#62306,10.);
#9239=VECTOR('',#62309,10.);
#9240=VECTOR('',#62312,10.);
#9241=VECTOR('',#62315,10.);
#9242=VECTOR('',#62318,10.);
#9243=VECTOR('',#62321,10.);
#9244=VECTOR('',#62326,10.);
#9245=VECTOR('',#62327,10.);
#9246=VECTOR('',#62332,10.);
#9247=VECTOR('',#62337,10.);
#9248=VECTOR('',#62342,10.);
#9249=VECTOR('',#62347,10.);
#9250=VECTOR('',#62352,10.);
#9251=VECTOR('',#62355,10.);
#9252=VECTOR('',#62356,10.);
#9253=VECTOR('',#62361,10.);
#9254=VECTOR('',#62366,10.);
#9255=VECTOR('',#62371,10.);
#9256=VECTOR('',#62376,10.);
#9257=VECTOR('',#62381,10.);
#9258=VECTOR('',#62384,10.);
#9259=VECTOR('',#62393,10.);
#9260=VECTOR('',#62404,10.);
#9261=VECTOR('',#62415,10.);
#9262=VECTOR('',#62418,10.);
#9263=VECTOR('',#62421,10.);
#9264=VECTOR('',#62424,10.);
#9265=VECTOR('',#62427,10.);
#9266=VECTOR('',#62430,10.);
#9267=VECTOR('',#62433,10.);
#9268=VECTOR('',#62436,10.);
#9269=VECTOR('',#62439,10.);
#9270=VECTOR('',#62442,10.);
#9271=VECTOR('',#62445,10.);
#9272=VECTOR('',#62448,10.);
#9273=VECTOR('',#62451,10.);
#9274=VECTOR('',#62454,10.);
#9275=VECTOR('',#62459,10.);
#9276=VECTOR('',#62460,10.);
#9277=VECTOR('',#62465,10.);
#9278=VECTOR('',#62470,10.);
#9279=VECTOR('',#62475,10.);
#9280=VECTOR('',#62480,10.);
#9281=VECTOR('',#62485,10.);
#9282=VECTOR('',#62488,10.);
#9283=VECTOR('',#62489,10.);
#9284=VECTOR('',#62494,10.);
#9285=VECTOR('',#62499,10.);
#9286=VECTOR('',#62504,10.);
#9287=VECTOR('',#62509,10.);
#9288=VECTOR('',#62514,10.);
#9289=VECTOR('',#62517,10.);
#9290=VECTOR('',#62526,10.);
#9291=VECTOR('',#62537,10.);
#9292=VECTOR('',#62548,10.);
#9293=VECTOR('',#62551,10.);
#9294=VECTOR('',#62554,10.);
#9295=VECTOR('',#62557,10.);
#9296=VECTOR('',#62560,10.);
#9297=VECTOR('',#62563,10.);
#9298=VECTOR('',#62566,10.);
#9299=VECTOR('',#62569,10.);
#9300=VECTOR('',#62572,10.);
#9301=VECTOR('',#62575,10.);
#9302=VECTOR('',#62578,10.);
#9303=VECTOR('',#62581,10.);
#9304=VECTOR('',#62584,10.);
#9305=VECTOR('',#62587,10.);
#9306=VECTOR('',#62592,10.);
#9307=VECTOR('',#62593,10.);
#9308=VECTOR('',#62598,10.);
#9309=VECTOR('',#62603,10.);
#9310=VECTOR('',#62608,10.);
#9311=VECTOR('',#62613,10.);
#9312=VECTOR('',#62618,10.);
#9313=VECTOR('',#62621,10.);
#9314=VECTOR('',#62622,10.);
#9315=VECTOR('',#62627,10.);
#9316=VECTOR('',#62632,10.);
#9317=VECTOR('',#62637,10.);
#9318=VECTOR('',#62642,10.);
#9319=VECTOR('',#62647,10.);
#9320=VECTOR('',#62650,10.);
#9321=VECTOR('',#62659,10.);
#9322=VECTOR('',#62670,10.);
#9323=VECTOR('',#62681,10.);
#9324=VECTOR('',#62684,10.);
#9325=VECTOR('',#62685,10.);
#9326=VECTOR('',#62690,10.);
#9327=VECTOR('',#62695,10.);
#9328=VECTOR('',#62700,10.);
#9329=VECTOR('',#62705,10.);
#9330=VECTOR('',#62710,10.);
#9331=VECTOR('',#62713,10.);
#9332=VECTOR('',#62714,10.);
#9333=VECTOR('',#62719,10.);
#9334=VECTOR('',#62724,10.);
#9335=VECTOR('',#62729,10.);
#9336=VECTOR('',#62734,10.);
#9337=VECTOR('',#62739,10.);
#9338=VECTOR('',#62742,10.);
#9339=VECTOR('',#62743,10.);
#9340=VECTOR('',#62750,10.);
#9341=VECTOR('',#62753,10.);
#9342=VECTOR('',#62756,10.);
#9343=VECTOR('',#62759,10.);
#9344=VECTOR('',#62762,10.);
#9345=VECTOR('',#62765,10.);
#9346=VECTOR('',#62768,10.);
#9347=VECTOR('',#62771,10.);
#9348=VECTOR('',#62774,10.);
#9349=VECTOR('',#62777,10.);
#9350=VECTOR('',#62780,10.);
#9351=VECTOR('',#62783,10.);
#9352=VECTOR('',#62786,10.);
#9353=VECTOR('',#62793,42.6);
#9354=VECTOR('',#62800,47.3660700849456);
#9355=VECTOR('',#62807,49.25);
#9356=VECTOR('',#62824,51.);
#9357=VECTOR('',#62839,46.5);
#9358=VECTOR('',#62868,50.1);
#9359=VECTOR('',#62873,50.5);
#9360=VECTOR('',#62876,50.25);
#9361=VECTOR('',#62881,50.4);
#9362=VECTOR('',#62884,50.7);
#11216=PLANE('',#51261);
#11217=PLANE('',#51262);
#11218=PLANE('',#51264);
#11219=PLANE('',#51265);
#11220=PLANE('',#51267);
#11221=PLANE('',#51268);
#11222=PLANE('',#51270);
#11223=PLANE('',#51271);
#11224=PLANE('',#51273);
#11225=PLANE('',#51274);
#11226=PLANE('',#51276);
#11227=PLANE('',#51277);
#11228=PLANE('',#51279);
#11229=PLANE('',#51280);
#11230=PLANE('',#51282);
#11231=PLANE('',#51283);
#11232=PLANE('',#51285);
#11233=PLANE('',#51286);
#11234=PLANE('',#51288);
#11235=PLANE('',#51289);
#11236=PLANE('',#51291);
#11237=PLANE('',#51292);
#11238=PLANE('',#51294);
#11239=PLANE('',#51295);
#11240=PLANE('',#51297);
#11241=PLANE('',#51298);
#11242=PLANE('',#51300);
#11243=PLANE('',#51301);
#11244=PLANE('',#51303);
#11245=PLANE('',#51304);
#11246=PLANE('',#51306);
#11247=PLANE('',#51307);
#11248=PLANE('',#51309);
#11249=PLANE('',#51310);
#11250=PLANE('',#51312);
#11251=PLANE('',#51313);
#11252=PLANE('',#51315);
#11253=PLANE('',#51316);
#11254=PLANE('',#51318);
#11255=PLANE('',#51319);
#11256=PLANE('',#51321);
#11257=PLANE('',#51322);
#11258=PLANE('',#51324);
#11259=PLANE('',#51325);
#11260=PLANE('',#51327);
#11261=PLANE('',#51328);
#11262=PLANE('',#51330);
#11263=PLANE('',#51331);
#11264=PLANE('',#51333);
#11265=PLANE('',#51334);
#11266=PLANE('',#51336);
#11267=PLANE('',#51337);
#11268=PLANE('',#51339);
#11269=PLANE('',#51340);
#11270=PLANE('',#51342);
#11271=PLANE('',#51343);
#11272=PLANE('',#51345);
#11273=PLANE('',#51346);
#11274=PLANE('',#51348);
#11275=PLANE('',#51349);
#11276=PLANE('',#51351);
#11277=PLANE('',#51352);
#11278=PLANE('',#51354);
#11279=PLANE('',#51355);
#11280=PLANE('',#51357);
#11281=PLANE('',#51358);
#11282=PLANE('',#51360);
#11283=PLANE('',#51361);
#11284=PLANE('',#51363);
#11285=PLANE('',#51364);
#11286=PLANE('',#51366);
#11287=PLANE('',#51367);
#11288=PLANE('',#51441);
#11289=PLANE('',#51443);
#11290=PLANE('',#51445);
#11291=PLANE('',#51447);
#11292=PLANE('',#51449);
#11293=PLANE('',#51451);
#11294=PLANE('',#51453);
#11295=PLANE('',#51455);
#11296=PLANE('',#51457);
#11297=PLANE('',#51459);
#11298=PLANE('',#51461);
#11299=PLANE('',#51463);
#11300=PLANE('',#51465);
#11301=PLANE('',#51467);
#11302=PLANE('',#51469);
#11303=PLANE('',#51471);
#11304=PLANE('',#51473);
#11305=PLANE('',#51475);
#11306=PLANE('',#51477);
#11307=PLANE('',#51479);
#11308=PLANE('',#51481);
#11309=PLANE('',#51483);
#11310=PLANE('',#51485);
#11311=PLANE('',#51487);
#11312=PLANE('',#51489);
#11313=PLANE('',#51491);
#11314=PLANE('',#51493);
#11315=PLANE('',#51495);
#11316=PLANE('',#51497);
#11317=PLANE('',#51499);
#11318=PLANE('',#51501);
#11319=PLANE('',#51503);
#11320=PLANE('',#51505);
#11321=PLANE('',#51507);
#11322=PLANE('',#51509);
#11323=PLANE('',#51511);
#11324=PLANE('',#51513);
#11325=PLANE('',#51514);
#11326=PLANE('',#51515);
#11327=PLANE('',#51516);
#11328=PLANE('',#51517);
#11329=PLANE('',#51518);
#11330=PLANE('',#51519);
#11331=PLANE('',#51520);
#11332=PLANE('',#51521);
#11333=PLANE('',#51522);
#11334=PLANE('',#51523);
#11335=PLANE('',#51524);
#11336=PLANE('',#51525);
#11337=PLANE('',#51526);
#11338=PLANE('',#51527);
#11339=PLANE('',#51528);
#11340=PLANE('',#51529);
#11341=PLANE('',#51530);
#11342=PLANE('',#51531);
#11343=PLANE('',#51532);
#11344=PLANE('',#51533);
#11345=PLANE('',#51534);
#11346=PLANE('',#51535);
#11347=PLANE('',#51536);
#11348=PLANE('',#51537);
#11349=PLANE('',#51538);
#11350=PLANE('',#51539);
#11351=PLANE('',#51540);
#11352=PLANE('',#51541);
#11353=PLANE('',#51542);
#11354=PLANE('',#51543);
#11355=PLANE('',#51544);
#11356=PLANE('',#51545);
#11357=PLANE('',#51546);
#11358=PLANE('',#51547);
#11359=PLANE('',#51548);
#11360=PLANE('',#51549);
#11361=PLANE('',#51551);
#11362=PLANE('',#51553);
#11363=PLANE('',#51555);
#11364=PLANE('',#51557);
#11365=PLANE('',#51559);
#11366=PLANE('',#51561);
#11367=PLANE('',#51563);
#11368=PLANE('',#51565);
#11369=PLANE('',#51567);
#11370=PLANE('',#51569);
#11371=PLANE('',#51571);
#11372=PLANE('',#51573);
#11373=PLANE('',#51575);
#11374=PLANE('',#51577);
#11375=PLANE('',#51579);
#11376=PLANE('',#51581);
#11377=PLANE('',#51583);
#11378=PLANE('',#51585);
#11379=PLANE('',#51587);
#11380=PLANE('',#51589);
#11381=PLANE('',#51591);
#11382=PLANE('',#51593);
#11383=PLANE('',#51595);
#11384=PLANE('',#51597);
#11385=PLANE('',#51599);
#11386=PLANE('',#51601);
#11387=PLANE('',#51603);
#11388=PLANE('',#51605);
#11389=PLANE('',#51607);
#11390=PLANE('',#51609);
#11391=PLANE('',#51611);
#11392=PLANE('',#51613);
#11393=PLANE('',#51615);
#11394=PLANE('',#51617);
#11395=PLANE('',#51619);
#11396=PLANE('',#51620);
#11397=PLANE('',#51621);
#11398=PLANE('',#51622);
#11399=PLANE('',#51623);
#11400=PLANE('',#51624);
#11401=PLANE('',#51625);
#11402=PLANE('',#51626);
#11403=PLANE('',#51627);
#11404=PLANE('',#51628);
#11405=PLANE('',#51629);
#11406=PLANE('',#51630);
#11407=PLANE('',#51631);
#11408=PLANE('',#51632);
#11409=PLANE('',#51633);
#11410=PLANE('',#51634);
#11411=PLANE('',#51635);
#11412=PLANE('',#51636);
#11413=PLANE('',#51637);
#11414=PLANE('',#51638);
#11415=PLANE('',#51639);
#11416=PLANE('',#51640);
#11417=PLANE('',#51641);
#11418=PLANE('',#51642);
#11419=PLANE('',#51643);
#11420=PLANE('',#51644);
#11421=PLANE('',#51645);
#11422=PLANE('',#51646);
#11423=PLANE('',#51647);
#11424=PLANE('',#51648);
#11425=PLANE('',#51649);
#11426=PLANE('',#51650);
#11427=PLANE('',#51651);
#11428=PLANE('',#51652);
#11429=PLANE('',#51653);
#11430=PLANE('',#51654);
#11431=PLANE('',#51655);
#11432=PLANE('',#51656);
#11433=PLANE('',#51657);
#11434=PLANE('',#51658);
#11435=PLANE('',#51659);
#11436=PLANE('',#51660);
#11437=PLANE('',#51661);
#11438=PLANE('',#51662);
#11439=PLANE('',#51663);
#11440=PLANE('',#51664);
#11441=PLANE('',#51665);
#11442=PLANE('',#51666);
#11443=PLANE('',#51667);
#11444=PLANE('',#51668);
#11445=PLANE('',#51669);
#11446=PLANE('',#51670);
#11447=PLANE('',#51671);
#11448=PLANE('',#51672);
#11449=PLANE('',#51673);
#11450=PLANE('',#51674);
#11451=PLANE('',#51675);
#11452=PLANE('',#51676);
#11453=PLANE('',#51677);
#11454=PLANE('',#51678);
#11455=PLANE('',#51679);
#11456=PLANE('',#51680);
#11457=PLANE('',#51681);
#11458=PLANE('',#51682);
#11459=PLANE('',#51683);
#11460=PLANE('',#51684);
#11461=PLANE('',#51685);
#11462=PLANE('',#51686);
#11463=PLANE('',#51687);
#11464=PLANE('',#51688);
#11465=PLANE('',#51689);
#11466=PLANE('',#51690);
#11467=PLANE('',#51691);
#11468=PLANE('',#51692);
#11469=PLANE('',#51693);
#11470=PLANE('',#51695);
#11471=PLANE('',#51697);
#11472=PLANE('',#51699);
#11473=PLANE('',#51701);
#11474=PLANE('',#51703);
#11475=PLANE('',#51704);
#11476=PLANE('',#51706);
#11477=PLANE('',#51708);
#11478=PLANE('',#51710);
#11479=PLANE('',#51712);
#11480=PLANE('',#51714);
#11481=PLANE('',#51715);
#11482=PLANE('',#51717);
#11483=PLANE('',#51718);
#11484=PLANE('',#51720);
#11485=PLANE('',#51722);
#11486=PLANE('',#51724);
#11487=PLANE('',#51726);
#11488=PLANE('',#51728);
#11489=PLANE('',#51729);
#11490=PLANE('',#51731);
#11491=PLANE('',#51733);
#11492=PLANE('',#51735);
#11493=PLANE('',#51737);
#11494=PLANE('',#51739);
#11495=PLANE('',#51740);
#11496=PLANE('',#51792);
#11497=PLANE('',#51793);
#11498=PLANE('',#51794);
#11499=PLANE('',#51795);
#11500=PLANE('',#51796);
#11501=PLANE('',#51797);
#11502=PLANE('',#51798);
#11503=PLANE('',#51799);
#11504=PLANE('',#51800);
#11505=PLANE('',#51801);
#11506=PLANE('',#51802);
#11507=PLANE('',#51803);
#11508=PLANE('',#51804);
#11509=PLANE('',#51805);
#11510=PLANE('',#51806);
#11511=PLANE('',#51807);
#11512=PLANE('',#51809);
#11513=PLANE('',#51811);
#11514=PLANE('',#51813);
#11515=PLANE('',#51815);
#11516=PLANE('',#51817);
#11517=PLANE('',#51818);
#11518=PLANE('',#51820);
#11519=PLANE('',#51822);
#11520=PLANE('',#51824);
#11521=PLANE('',#51826);
#11522=PLANE('',#51828);
#11523=PLANE('',#51829);
#11524=PLANE('',#51843);
#11525=PLANE('',#51844);
#11526=PLANE('',#51845);
#11527=PLANE('',#51846);
#11528=PLANE('',#51847);
#11529=PLANE('',#51848);
#11530=PLANE('',#51849);
#11531=PLANE('',#51850);
#11532=PLANE('',#51851);
#11533=PLANE('',#51852);
#11534=PLANE('',#51853);
#11535=PLANE('',#51854);
#11536=PLANE('',#51855);
#11537=PLANE('',#51856);
#11538=PLANE('',#51857);
#11539=PLANE('',#51858);
#11540=PLANE('',#51860);
#11541=PLANE('',#51862);
#11542=PLANE('',#51864);
#11543=PLANE('',#51866);
#11544=PLANE('',#51868);
#11545=PLANE('',#51869);
#11546=PLANE('',#51871);
#11547=PLANE('',#51873);
#11548=PLANE('',#51875);
#11549=PLANE('',#51877);
#11550=PLANE('',#51879);
#11551=PLANE('',#51880);
#11552=PLANE('',#51894);
#11553=PLANE('',#51895);
#11554=PLANE('',#51896);
#11555=PLANE('',#51897);
#11556=PLANE('',#51898);
#11557=PLANE('',#51899);
#11558=PLANE('',#51900);
#11559=PLANE('',#51901);
#11560=PLANE('',#51902);
#11561=PLANE('',#51903);
#11562=PLANE('',#51904);
#11563=PLANE('',#51905);
#11564=PLANE('',#51906);
#11565=PLANE('',#51907);
#11566=PLANE('',#51908);
#11567=PLANE('',#51909);
#11568=PLANE('',#51911);
#11569=PLANE('',#51913);
#11570=PLANE('',#51915);
#11571=PLANE('',#51917);
#11572=PLANE('',#51919);
#11573=PLANE('',#51920);
#11574=PLANE('',#51922);
#11575=PLANE('',#51924);
#11576=PLANE('',#51926);
#11577=PLANE('',#51928);
#11578=PLANE('',#51930);
#11579=PLANE('',#51931);
#11580=PLANE('',#51945);
#11581=PLANE('',#51946);
#11582=PLANE('',#51947);
#11583=PLANE('',#51948);
#11584=PLANE('',#51949);
#11585=PLANE('',#51950);
#11586=PLANE('',#51951);
#11587=PLANE('',#51952);
#11588=PLANE('',#51953);
#11589=PLANE('',#51954);
#11590=PLANE('',#51955);
#11591=PLANE('',#51956);
#11592=PLANE('',#51957);
#11593=PLANE('',#51958);
#11594=PLANE('',#51959);
#11595=PLANE('',#51960);
#11596=PLANE('',#51962);
#11597=PLANE('',#51964);
#11598=PLANE('',#51966);
#11599=PLANE('',#51968);
#11600=PLANE('',#51970);
#11601=PLANE('',#51971);
#11602=PLANE('',#51973);
#11603=PLANE('',#51975);
#11604=PLANE('',#51977);
#11605=PLANE('',#51979);
#11606=PLANE('',#51981);
#11607=PLANE('',#51982);
#11608=PLANE('',#51996);
#11609=PLANE('',#51997);
#11610=PLANE('',#51998);
#11611=PLANE('',#51999);
#11612=PLANE('',#52000);
#11613=PLANE('',#52001);
#11614=PLANE('',#52002);
#11615=PLANE('',#52003);
#11616=PLANE('',#52004);
#11617=PLANE('',#52005);
#11618=PLANE('',#52006);
#11619=PLANE('',#52007);
#11620=PLANE('',#52008);
#11621=PLANE('',#52009);
#11622=PLANE('',#52010);
#11623=PLANE('',#52011);
#11624=PLANE('',#52013);
#11625=PLANE('',#52015);
#11626=PLANE('',#52017);
#11627=PLANE('',#52019);
#11628=PLANE('',#52021);
#11629=PLANE('',#52022);
#11630=PLANE('',#52024);
#11631=PLANE('',#52026);
#11632=PLANE('',#52028);
#11633=PLANE('',#52030);
#11634=PLANE('',#52032);
#11635=PLANE('',#52033);
#11636=PLANE('',#52047);
#11637=PLANE('',#52048);
#11638=PLANE('',#52049);
#11639=PLANE('',#52050);
#11640=PLANE('',#52051);
#11641=PLANE('',#52052);
#11642=PLANE('',#52053);
#11643=PLANE('',#52054);
#11644=PLANE('',#52055);
#11645=PLANE('',#52056);
#11646=PLANE('',#52057);
#11647=PLANE('',#52058);
#11648=PLANE('',#52059);
#11649=PLANE('',#52060);
#11650=PLANE('',#52061);
#11651=PLANE('',#52062);
#11652=PLANE('',#52064);
#11653=PLANE('',#52066);
#11654=PLANE('',#52068);
#11655=PLANE('',#52070);
#11656=PLANE('',#52072);
#11657=PLANE('',#52073);
#11658=PLANE('',#52075);
#11659=PLANE('',#52077);
#11660=PLANE('',#52079);
#11661=PLANE('',#52081);
#11662=PLANE('',#52083);
#11663=PLANE('',#52084);
#11664=PLANE('',#52098);
#11665=PLANE('',#52099);
#11666=PLANE('',#52100);
#11667=PLANE('',#52101);
#11668=PLANE('',#52102);
#11669=PLANE('',#52103);
#11670=PLANE('',#52104);
#11671=PLANE('',#52105);
#11672=PLANE('',#52106);
#11673=PLANE('',#52107);
#11674=PLANE('',#52108);
#11675=PLANE('',#52109);
#11676=PLANE('',#52110);
#11677=PLANE('',#52111);
#11678=PLANE('',#52112);
#11679=PLANE('',#52113);
#11680=PLANE('',#52115);
#11681=PLANE('',#52117);
#11682=PLANE('',#52119);
#11683=PLANE('',#52121);
#11684=PLANE('',#52123);
#11685=PLANE('',#52124);
#11686=PLANE('',#52126);
#11687=PLANE('',#52128);
#11688=PLANE('',#52130);
#11689=PLANE('',#52132);
#11690=PLANE('',#52134);
#11691=PLANE('',#52135);
#11692=PLANE('',#52149);
#11693=PLANE('',#52150);
#11694=PLANE('',#52151);
#11695=PLANE('',#52152);
#11696=PLANE('',#52153);
#11697=PLANE('',#52154);
#11698=PLANE('',#52155);
#11699=PLANE('',#52156);
#11700=PLANE('',#52157);
#11701=PLANE('',#52158);
#11702=PLANE('',#52159);
#11703=PLANE('',#52160);
#11704=PLANE('',#52161);
#11705=PLANE('',#52162);
#11706=PLANE('',#52163);
#11707=PLANE('',#52164);
#11708=PLANE('',#52166);
#11709=PLANE('',#52168);
#11710=PLANE('',#52170);
#11711=PLANE('',#52172);
#11712=PLANE('',#52174);
#11713=PLANE('',#52175);
#11714=PLANE('',#52177);
#11715=PLANE('',#52179);
#11716=PLANE('',#52181);
#11717=PLANE('',#52183);
#11718=PLANE('',#52185);
#11719=PLANE('',#52186);
#11720=PLANE('',#52200);
#11721=PLANE('',#52201);
#11722=PLANE('',#52202);
#11723=PLANE('',#52203);
#11724=PLANE('',#52204);
#11725=PLANE('',#52205);
#11726=PLANE('',#52206);
#11727=PLANE('',#52207);
#11728=PLANE('',#52208);
#11729=PLANE('',#52209);
#11730=PLANE('',#52210);
#11731=PLANE('',#52211);
#11732=PLANE('',#52212);
#11733=PLANE('',#52213);
#11734=PLANE('',#52214);
#11735=PLANE('',#52215);
#11736=PLANE('',#52217);
#11737=PLANE('',#52219);
#11738=PLANE('',#52221);
#11739=PLANE('',#52223);
#11740=PLANE('',#52225);
#11741=PLANE('',#52226);
#11742=PLANE('',#52228);
#11743=PLANE('',#52230);
#11744=PLANE('',#52232);
#11745=PLANE('',#52234);
#11746=PLANE('',#52236);
#11747=PLANE('',#52237);
#11748=PLANE('',#52251);
#11749=PLANE('',#52252);
#11750=PLANE('',#52253);
#11751=PLANE('',#52254);
#11752=PLANE('',#52255);
#11753=PLANE('',#52256);
#11754=PLANE('',#52257);
#11755=PLANE('',#52258);
#11756=PLANE('',#52259);
#11757=PLANE('',#52260);
#11758=PLANE('',#52261);
#11759=PLANE('',#52262);
#11760=PLANE('',#52263);
#11761=PLANE('',#52264);
#11762=PLANE('',#52265);
#11763=PLANE('',#52266);
#11764=PLANE('',#52268);
#11765=PLANE('',#52270);
#11766=PLANE('',#52272);
#11767=PLANE('',#52274);
#11768=PLANE('',#52276);
#11769=PLANE('',#52277);
#11770=PLANE('',#52279);
#11771=PLANE('',#52281);
#11772=PLANE('',#52283);
#11773=PLANE('',#52285);
#11774=PLANE('',#52287);
#11775=PLANE('',#52288);
#11776=PLANE('',#52302);
#11777=PLANE('',#52303);
#11778=PLANE('',#52304);
#11779=PLANE('',#52305);
#11780=PLANE('',#52306);
#11781=PLANE('',#52307);
#11782=PLANE('',#52308);
#11783=PLANE('',#52309);
#11784=PLANE('',#52310);
#11785=PLANE('',#52311);
#11786=PLANE('',#52312);
#11787=PLANE('',#52313);
#11788=PLANE('',#52314);
#11789=PLANE('',#52315);
#11790=PLANE('',#52316);
#11791=PLANE('',#52317);
#11792=PLANE('',#52319);
#11793=PLANE('',#52321);
#11794=PLANE('',#52323);
#11795=PLANE('',#52325);
#11796=PLANE('',#52327);
#11797=PLANE('',#52328);
#11798=PLANE('',#52330);
#11799=PLANE('',#52332);
#11800=PLANE('',#52334);
#11801=PLANE('',#52336);
#11802=PLANE('',#52338);
#11803=PLANE('',#52339);
#11804=PLANE('',#52353);
#11805=PLANE('',#52354);
#11806=PLANE('',#52355);
#11807=PLANE('',#52356);
#11808=PLANE('',#52357);
#11809=PLANE('',#52358);
#11810=PLANE('',#52359);
#11811=PLANE('',#52360);
#11812=PLANE('',#52361);
#11813=PLANE('',#52362);
#11814=PLANE('',#52363);
#11815=PLANE('',#52364);
#11816=PLANE('',#52365);
#11817=PLANE('',#52366);
#11818=PLANE('',#52367);
#11819=PLANE('',#52368);
#11820=PLANE('',#52370);
#11821=PLANE('',#52372);
#11822=PLANE('',#52374);
#11823=PLANE('',#52376);
#11824=PLANE('',#52378);
#11825=PLANE('',#52379);
#11826=PLANE('',#52381);
#11827=PLANE('',#52383);
#11828=PLANE('',#52385);
#11829=PLANE('',#52387);
#11830=PLANE('',#52389);
#11831=PLANE('',#52390);
#11832=PLANE('',#52404);
#11833=PLANE('',#52405);
#11834=PLANE('',#52406);
#11835=PLANE('',#52407);
#11836=PLANE('',#52408);
#11837=PLANE('',#52409);
#11838=PLANE('',#52410);
#11839=PLANE('',#52411);
#11840=PLANE('',#52412);
#11841=PLANE('',#52413);
#11842=PLANE('',#52414);
#11843=PLANE('',#52415);
#11844=PLANE('',#52416);
#11845=PLANE('',#52417);
#11846=PLANE('',#52418);
#11847=PLANE('',#52419);
#11848=PLANE('',#52421);
#11849=PLANE('',#52423);
#11850=PLANE('',#52425);
#11851=PLANE('',#52427);
#11852=PLANE('',#52429);
#11853=PLANE('',#52430);
#11854=PLANE('',#52432);
#11855=PLANE('',#52434);
#11856=PLANE('',#52436);
#11857=PLANE('',#52438);
#11858=PLANE('',#52440);
#11859=PLANE('',#52441);
#11860=PLANE('',#52455);
#11861=PLANE('',#52456);
#11862=PLANE('',#52457);
#11863=PLANE('',#52458);
#11864=PLANE('',#52459);
#11865=PLANE('',#52460);
#11866=PLANE('',#52461);
#11867=PLANE('',#52462);
#11868=PLANE('',#52463);
#11869=PLANE('',#52464);
#11870=PLANE('',#52465);
#11871=PLANE('',#52466);
#11872=PLANE('',#52467);
#11873=PLANE('',#52468);
#11874=PLANE('',#52469);
#11875=PLANE('',#52470);
#11876=PLANE('',#52472);
#11877=PLANE('',#52474);
#11878=PLANE('',#52476);
#11879=PLANE('',#52478);
#11880=PLANE('',#52480);
#11881=PLANE('',#52481);
#11882=PLANE('',#52483);
#11883=PLANE('',#52485);
#11884=PLANE('',#52487);
#11885=PLANE('',#52489);
#11886=PLANE('',#52491);
#11887=PLANE('',#52492);
#11888=PLANE('',#52506);
#11889=PLANE('',#52507);
#11890=PLANE('',#52508);
#11891=PLANE('',#52509);
#11892=PLANE('',#52510);
#11893=PLANE('',#52511);
#11894=PLANE('',#52512);
#11895=PLANE('',#52513);
#11896=PLANE('',#52514);
#11897=PLANE('',#52515);
#11898=PLANE('',#52516);
#11899=PLANE('',#52517);
#11900=PLANE('',#52518);
#11901=PLANE('',#52519);
#11902=PLANE('',#52520);
#11903=PLANE('',#52521);
#11904=PLANE('',#52523);
#11905=PLANE('',#52525);
#11906=PLANE('',#52527);
#11907=PLANE('',#52529);
#11908=PLANE('',#52531);
#11909=PLANE('',#52532);
#11910=PLANE('',#52534);
#11911=PLANE('',#52536);
#11912=PLANE('',#52538);
#11913=PLANE('',#52540);
#11914=PLANE('',#52542);
#11915=PLANE('',#52543);
#11916=PLANE('',#52557);
#11917=PLANE('',#52558);
#11918=PLANE('',#52559);
#11919=PLANE('',#52560);
#11920=PLANE('',#52561);
#11921=PLANE('',#52562);
#11922=PLANE('',#52563);
#11923=PLANE('',#52564);
#11924=PLANE('',#52565);
#11925=PLANE('',#52566);
#11926=PLANE('',#52567);
#11927=PLANE('',#52568);
#11928=PLANE('',#52569);
#11929=PLANE('',#52570);
#11930=PLANE('',#52571);
#11931=PLANE('',#52572);
#11932=PLANE('',#52574);
#11933=PLANE('',#52576);
#11934=PLANE('',#52578);
#11935=PLANE('',#52580);
#11936=PLANE('',#52582);
#11937=PLANE('',#52583);
#11938=PLANE('',#52585);
#11939=PLANE('',#52587);
#11940=PLANE('',#52589);
#11941=PLANE('',#52591);
#11942=PLANE('',#52593);
#11943=PLANE('',#52594);
#11944=PLANE('',#52608);
#11945=PLANE('',#52609);
#11946=PLANE('',#52610);
#11947=PLANE('',#52611);
#11948=PLANE('',#52612);
#11949=PLANE('',#52613);
#11950=PLANE('',#52614);
#11951=PLANE('',#52615);
#11952=PLANE('',#52616);
#11953=PLANE('',#52617);
#11954=PLANE('',#52618);
#11955=PLANE('',#52619);
#11956=PLANE('',#52620);
#11957=PLANE('',#52621);
#11958=PLANE('',#52622);
#11959=PLANE('',#52623);
#11960=PLANE('',#52625);
#11961=PLANE('',#52627);
#11962=PLANE('',#52629);
#11963=PLANE('',#52631);
#11964=PLANE('',#52633);
#11965=PLANE('',#52634);
#11966=PLANE('',#52636);
#11967=PLANE('',#52638);
#11968=PLANE('',#52640);
#11969=PLANE('',#52642);
#11970=PLANE('',#52644);
#11971=PLANE('',#52645);
#11972=PLANE('',#52659);
#11973=PLANE('',#52660);
#11974=PLANE('',#52661);
#11975=PLANE('',#52662);
#11976=PLANE('',#52663);
#11977=PLANE('',#52664);
#11978=PLANE('',#52665);
#11979=PLANE('',#52666);
#11980=PLANE('',#52667);
#11981=PLANE('',#52668);
#11982=PLANE('',#52669);
#11983=PLANE('',#52670);
#11984=PLANE('',#52671);
#11985=PLANE('',#52672);
#11986=PLANE('',#52673);
#11987=PLANE('',#52674);
#11988=PLANE('',#52676);
#11989=PLANE('',#52678);
#11990=PLANE('',#52680);
#11991=PLANE('',#52682);
#11992=PLANE('',#52684);
#11993=PLANE('',#52685);
#11994=PLANE('',#52687);
#11995=PLANE('',#52689);
#11996=PLANE('',#52691);
#11997=PLANE('',#52693);
#11998=PLANE('',#52695);
#11999=PLANE('',#52696);
#12000=PLANE('',#52710);
#12001=PLANE('',#52711);
#12002=PLANE('',#52712);
#12003=PLANE('',#52713);
#12004=PLANE('',#52714);
#12005=PLANE('',#52715);
#12006=PLANE('',#52716);
#12007=PLANE('',#52717);
#12008=PLANE('',#52718);
#12009=PLANE('',#52719);
#12010=PLANE('',#52720);
#12011=PLANE('',#52721);
#12012=PLANE('',#52722);
#12013=PLANE('',#52723);
#12014=PLANE('',#52724);
#12015=PLANE('',#52725);
#12016=PLANE('',#52727);
#12017=PLANE('',#52729);
#12018=PLANE('',#52731);
#12019=PLANE('',#52733);
#12020=PLANE('',#52735);
#12021=PLANE('',#52736);
#12022=PLANE('',#52738);
#12023=PLANE('',#52740);
#12024=PLANE('',#52742);
#12025=PLANE('',#52744);
#12026=PLANE('',#52746);
#12027=PLANE('',#52747);
#12028=PLANE('',#52761);
#12029=PLANE('',#52762);
#12030=PLANE('',#52763);
#12031=PLANE('',#52764);
#12032=PLANE('',#52765);
#12033=PLANE('',#52766);
#12034=PLANE('',#52767);
#12035=PLANE('',#52768);
#12036=PLANE('',#52769);
#12037=PLANE('',#52770);
#12038=PLANE('',#52771);
#12039=PLANE('',#52772);
#12040=PLANE('',#52773);
#12041=PLANE('',#52774);
#12042=PLANE('',#52775);
#12043=PLANE('',#52776);
#12044=PLANE('',#52778);
#12045=PLANE('',#52780);
#12046=PLANE('',#52782);
#12047=PLANE('',#52784);
#12048=PLANE('',#52786);
#12049=PLANE('',#52787);
#12050=PLANE('',#52789);
#12051=PLANE('',#52791);
#12052=PLANE('',#52793);
#12053=PLANE('',#52795);
#12054=PLANE('',#52797);
#12055=PLANE('',#52798);
#12056=PLANE('',#52812);
#12057=PLANE('',#52813);
#12058=PLANE('',#52814);
#12059=PLANE('',#52815);
#12060=PLANE('',#52816);
#12061=PLANE('',#52817);
#12062=PLANE('',#52818);
#12063=PLANE('',#52819);
#12064=PLANE('',#52820);
#12065=PLANE('',#52821);
#12066=PLANE('',#52822);
#12067=PLANE('',#52823);
#12068=PLANE('',#52824);
#12069=PLANE('',#52825);
#12070=PLANE('',#52826);
#12071=PLANE('',#52827);
#12072=PLANE('',#52829);
#12073=PLANE('',#52831);
#12074=PLANE('',#52833);
#12075=PLANE('',#52835);
#12076=PLANE('',#52837);
#12077=PLANE('',#52838);
#12078=PLANE('',#52840);
#12079=PLANE('',#52842);
#12080=PLANE('',#52844);
#12081=PLANE('',#52846);
#12082=PLANE('',#52848);
#12083=PLANE('',#52849);
#12084=PLANE('',#52863);
#12085=PLANE('',#52864);
#12086=PLANE('',#52865);
#12087=PLANE('',#52866);
#12088=PLANE('',#52867);
#12089=PLANE('',#52868);
#12090=PLANE('',#52869);
#12091=PLANE('',#52870);
#12092=PLANE('',#52871);
#12093=PLANE('',#52872);
#12094=PLANE('',#52873);
#12095=PLANE('',#52874);
#12096=PLANE('',#52875);
#12097=PLANE('',#52876);
#12098=PLANE('',#52877);
#12099=PLANE('',#52878);
#12100=PLANE('',#52880);
#12101=PLANE('',#52882);
#12102=PLANE('',#52884);
#12103=PLANE('',#52886);
#12104=PLANE('',#52888);
#12105=PLANE('',#52889);
#12106=PLANE('',#52891);
#12107=PLANE('',#52893);
#12108=PLANE('',#52895);
#12109=PLANE('',#52897);
#12110=PLANE('',#52899);
#12111=PLANE('',#52900);
#12112=PLANE('',#52914);
#12113=PLANE('',#52915);
#12114=PLANE('',#52916);
#12115=PLANE('',#52917);
#12116=PLANE('',#52918);
#12117=PLANE('',#52919);
#12118=PLANE('',#52920);
#12119=PLANE('',#52921);
#12120=PLANE('',#52922);
#12121=PLANE('',#52923);
#12122=PLANE('',#52924);
#12123=PLANE('',#52925);
#12124=PLANE('',#52926);
#12125=PLANE('',#52927);
#12126=PLANE('',#52928);
#12127=PLANE('',#52929);
#12128=PLANE('',#52931);
#12129=PLANE('',#52933);
#12130=PLANE('',#52935);
#12131=PLANE('',#52937);
#12132=PLANE('',#52939);
#12133=PLANE('',#52940);
#12134=PLANE('',#52942);
#12135=PLANE('',#52944);
#12136=PLANE('',#52946);
#12137=PLANE('',#52948);
#12138=PLANE('',#52950);
#12139=PLANE('',#52951);
#12140=PLANE('',#52965);
#12141=PLANE('',#52966);
#12142=PLANE('',#52967);
#12143=PLANE('',#52968);
#12144=PLANE('',#52969);
#12145=PLANE('',#52970);
#12146=PLANE('',#52971);
#12147=PLANE('',#52972);
#12148=PLANE('',#52973);
#12149=PLANE('',#52974);
#12150=PLANE('',#52975);
#12151=PLANE('',#52976);
#12152=PLANE('',#52977);
#12153=PLANE('',#52978);
#12154=PLANE('',#52979);
#12155=PLANE('',#52980);
#12156=PLANE('',#52982);
#12157=PLANE('',#52984);
#12158=PLANE('',#52986);
#12159=PLANE('',#52988);
#12160=PLANE('',#52990);
#12161=PLANE('',#52991);
#12162=PLANE('',#52993);
#12163=PLANE('',#52995);
#12164=PLANE('',#52997);
#12165=PLANE('',#52999);
#12166=PLANE('',#53001);
#12167=PLANE('',#53002);
#12168=PLANE('',#53016);
#12169=PLANE('',#53017);
#12170=PLANE('',#53018);
#12171=PLANE('',#53019);
#12172=PLANE('',#53020);
#12173=PLANE('',#53021);
#12174=PLANE('',#53022);
#12175=PLANE('',#53023);
#12176=PLANE('',#53024);
#12177=PLANE('',#53025);
#12178=PLANE('',#53026);
#12179=PLANE('',#53027);
#12180=PLANE('',#53028);
#12181=PLANE('',#53029);
#12182=PLANE('',#53030);
#12183=PLANE('',#53031);
#12184=PLANE('',#53033);
#12185=PLANE('',#53035);
#12186=PLANE('',#53037);
#12187=PLANE('',#53039);
#12188=PLANE('',#53041);
#12189=PLANE('',#53042);
#12190=PLANE('',#53044);
#12191=PLANE('',#53046);
#12192=PLANE('',#53048);
#12193=PLANE('',#53050);
#12194=PLANE('',#53052);
#12195=PLANE('',#53053);
#12196=PLANE('',#53067);
#12197=PLANE('',#53068);
#12198=PLANE('',#53069);
#12199=PLANE('',#53070);
#12200=PLANE('',#53071);
#12201=PLANE('',#53072);
#12202=PLANE('',#53073);
#12203=PLANE('',#53074);
#12204=PLANE('',#53075);
#12205=PLANE('',#53076);
#12206=PLANE('',#53077);
#12207=PLANE('',#53078);
#12208=PLANE('',#53079);
#12209=PLANE('',#53080);
#12210=PLANE('',#53081);
#12211=PLANE('',#53082);
#12212=PLANE('',#53084);
#12213=PLANE('',#53086);
#12214=PLANE('',#53088);
#12215=PLANE('',#53090);
#12216=PLANE('',#53092);
#12217=PLANE('',#53093);
#12218=PLANE('',#53095);
#12219=PLANE('',#53097);
#12220=PLANE('',#53099);
#12221=PLANE('',#53101);
#12222=PLANE('',#53103);
#12223=PLANE('',#53104);
#12224=PLANE('',#53118);
#12225=PLANE('',#53119);
#12226=PLANE('',#53120);
#12227=PLANE('',#53121);
#12228=PLANE('',#53122);
#12229=PLANE('',#53123);
#12230=PLANE('',#53124);
#12231=PLANE('',#53125);
#12232=PLANE('',#53126);
#12233=PLANE('',#53127);
#12234=PLANE('',#53128);
#12235=PLANE('',#53129);
#12236=PLANE('',#53130);
#12237=PLANE('',#53131);
#12238=PLANE('',#53132);
#12239=PLANE('',#53133);
#12240=PLANE('',#53135);
#12241=PLANE('',#53137);
#12242=PLANE('',#53139);
#12243=PLANE('',#53141);
#12244=PLANE('',#53143);
#12245=PLANE('',#53144);
#12246=PLANE('',#53146);
#12247=PLANE('',#53148);
#12248=PLANE('',#53150);
#12249=PLANE('',#53152);
#12250=PLANE('',#53154);
#12251=PLANE('',#53155);
#12252=PLANE('',#53169);
#12253=PLANE('',#53170);
#12254=PLANE('',#53171);
#12255=PLANE('',#53172);
#12256=PLANE('',#53173);
#12257=PLANE('',#53174);
#12258=PLANE('',#53175);
#12259=PLANE('',#53176);
#12260=PLANE('',#53177);
#12261=PLANE('',#53178);
#12262=PLANE('',#53179);
#12263=PLANE('',#53180);
#12264=PLANE('',#53181);
#12265=PLANE('',#53182);
#12266=PLANE('',#53183);
#12267=PLANE('',#53184);
#12268=PLANE('',#53186);
#12269=PLANE('',#53188);
#12270=PLANE('',#53190);
#12271=PLANE('',#53192);
#12272=PLANE('',#53194);
#12273=PLANE('',#53195);
#12274=PLANE('',#53197);
#12275=PLANE('',#53199);
#12276=PLANE('',#53201);
#12277=PLANE('',#53203);
#12278=PLANE('',#53205);
#12279=PLANE('',#53206);
#12280=PLANE('',#53220);
#12281=PLANE('',#53221);
#12282=PLANE('',#53222);
#12283=PLANE('',#53223);
#12284=PLANE('',#53224);
#12285=PLANE('',#53225);
#12286=PLANE('',#53226);
#12287=PLANE('',#53227);
#12288=PLANE('',#53228);
#12289=PLANE('',#53229);
#12290=PLANE('',#53230);
#12291=PLANE('',#53231);
#12292=PLANE('',#53232);
#12293=PLANE('',#53233);
#12294=PLANE('',#53234);
#12295=PLANE('',#53235);
#12296=PLANE('',#53237);
#12297=PLANE('',#53239);
#12298=PLANE('',#53241);
#12299=PLANE('',#53243);
#12300=PLANE('',#53245);
#12301=PLANE('',#53246);
#12302=PLANE('',#53248);
#12303=PLANE('',#53250);
#12304=PLANE('',#53252);
#12305=PLANE('',#53254);
#12306=PLANE('',#53256);
#12307=PLANE('',#53257);
#12308=PLANE('',#53271);
#12309=PLANE('',#53272);
#12310=PLANE('',#53273);
#12311=PLANE('',#53274);
#12312=PLANE('',#53275);
#12313=PLANE('',#53276);
#12314=PLANE('',#53277);
#12315=PLANE('',#53278);
#12316=PLANE('',#53279);
#12317=PLANE('',#53280);
#12318=PLANE('',#53281);
#12319=PLANE('',#53282);
#12320=PLANE('',#53283);
#12321=PLANE('',#53284);
#12322=PLANE('',#53285);
#12323=PLANE('',#53286);
#12324=PLANE('',#53288);
#12325=PLANE('',#53290);
#12326=PLANE('',#53292);
#12327=PLANE('',#53294);
#12328=PLANE('',#53296);
#12329=PLANE('',#53297);
#12330=PLANE('',#53299);
#12331=PLANE('',#53301);
#12332=PLANE('',#53303);
#12333=PLANE('',#53305);
#12334=PLANE('',#53307);
#12335=PLANE('',#53308);
#12336=PLANE('',#53322);
#12337=PLANE('',#53323);
#12338=PLANE('',#53324);
#12339=PLANE('',#53325);
#12340=PLANE('',#53326);
#12341=PLANE('',#53327);
#12342=PLANE('',#53328);
#12343=PLANE('',#53329);
#12344=PLANE('',#53330);
#12345=PLANE('',#53331);
#12346=PLANE('',#53332);
#12347=PLANE('',#53333);
#12348=PLANE('',#53334);
#12349=PLANE('',#53335);
#12350=PLANE('',#53336);
#12351=PLANE('',#53337);
#12352=PLANE('',#53339);
#12353=PLANE('',#53341);
#12354=PLANE('',#53343);
#12355=PLANE('',#53345);
#12356=PLANE('',#53347);
#12357=PLANE('',#53348);
#12358=PLANE('',#53350);
#12359=PLANE('',#53352);
#12360=PLANE('',#53354);
#12361=PLANE('',#53356);
#12362=PLANE('',#53358);
#12363=PLANE('',#53359);
#12364=PLANE('',#53373);
#12365=PLANE('',#53374);
#12366=PLANE('',#53375);
#12367=PLANE('',#53376);
#12368=PLANE('',#53377);
#12369=PLANE('',#53378);
#12370=PLANE('',#53379);
#12371=PLANE('',#53380);
#12372=PLANE('',#53381);
#12373=PLANE('',#53382);
#12374=PLANE('',#53383);
#12375=PLANE('',#53384);
#12376=PLANE('',#53385);
#12377=PLANE('',#53386);
#12378=PLANE('',#53387);
#12379=PLANE('',#53388);
#12380=PLANE('',#53390);
#12381=PLANE('',#53392);
#12382=PLANE('',#53394);
#12383=PLANE('',#53396);
#12384=PLANE('',#53398);
#12385=PLANE('',#53399);
#12386=PLANE('',#53401);
#12387=PLANE('',#53403);
#12388=PLANE('',#53405);
#12389=PLANE('',#53407);
#12390=PLANE('',#53409);
#12391=PLANE('',#53410);
#12392=PLANE('',#53424);
#12393=PLANE('',#53425);
#12394=PLANE('',#53426);
#12395=PLANE('',#53427);
#12396=PLANE('',#53428);
#12397=PLANE('',#53429);
#12398=PLANE('',#53430);
#12399=PLANE('',#53431);
#12400=PLANE('',#53432);
#12401=PLANE('',#53433);
#12402=PLANE('',#53434);
#12403=PLANE('',#53435);
#12404=PLANE('',#53436);
#12405=PLANE('',#53437);
#12406=PLANE('',#53438);
#12407=PLANE('',#53439);
#12408=PLANE('',#53441);
#12409=PLANE('',#53443);
#12410=PLANE('',#53445);
#12411=PLANE('',#53447);
#12412=PLANE('',#53449);
#12413=PLANE('',#53450);
#12414=PLANE('',#53452);
#12415=PLANE('',#53454);
#12416=PLANE('',#53456);
#12417=PLANE('',#53458);
#12418=PLANE('',#53460);
#12419=PLANE('',#53461);
#12420=PLANE('',#53475);
#12421=PLANE('',#53476);
#12422=PLANE('',#53477);
#12423=PLANE('',#53478);
#12424=PLANE('',#53479);
#12425=PLANE('',#53480);
#12426=PLANE('',#53481);
#12427=PLANE('',#53482);
#12428=PLANE('',#53483);
#12429=PLANE('',#53484);
#12430=PLANE('',#53485);
#12431=PLANE('',#53486);
#12432=PLANE('',#53487);
#12433=PLANE('',#53488);
#12434=PLANE('',#53489);
#12435=PLANE('',#53490);
#12436=PLANE('',#53492);
#12437=PLANE('',#53494);
#12438=PLANE('',#53496);
#12439=PLANE('',#53498);
#12440=PLANE('',#53500);
#12441=PLANE('',#53501);
#12442=PLANE('',#53503);
#12443=PLANE('',#53505);
#12444=PLANE('',#53507);
#12445=PLANE('',#53509);
#12446=PLANE('',#53511);
#12447=PLANE('',#53512);
#12448=PLANE('',#53526);
#12449=PLANE('',#53527);
#12450=PLANE('',#53529);
#12451=PLANE('',#53531);
#12452=PLANE('',#53533);
#12453=PLANE('',#53535);
#12454=PLANE('',#53537);
#12455=PLANE('',#53538);
#12456=PLANE('',#53540);
#12457=PLANE('',#53542);
#12458=PLANE('',#53544);
#12459=PLANE('',#53546);
#12460=PLANE('',#53548);
#12461=PLANE('',#53549);
#12462=PLANE('',#53551);
#12463=PLANE('',#53552);
#12464=PLANE('',#53553);
#12465=PLANE('',#53554);
#12466=PLANE('',#53555);
#12467=PLANE('',#53556);
#12468=PLANE('',#53557);
#12469=PLANE('',#53558);
#12470=PLANE('',#53559);
#12471=PLANE('',#53560);
#12472=PLANE('',#53561);
#12473=PLANE('',#53562);
#12474=PLANE('',#53563);
#12475=PLANE('',#53564);
#12476=PLANE('',#53575);
#12477=PLANE('',#53590);
#12478=PLANE('',#53595);
#12479=PLANE('',#53598);
#13249=FACE_OUTER_BOUND('',#15931,.T.);
#13250=FACE_OUTER_BOUND('',#15932,.T.);
#13251=FACE_OUTER_BOUND('',#15933,.T.);
#13252=FACE_OUTER_BOUND('',#15934,.T.);
#13253=FACE_OUTER_BOUND('',#15935,.T.);
#13254=FACE_OUTER_BOUND('',#15936,.T.);
#13255=FACE_OUTER_BOUND('',#15937,.T.);
#13256=FACE_OUTER_BOUND('',#15938,.T.);
#13257=FACE_OUTER_BOUND('',#15939,.T.);
#13258=FACE_OUTER_BOUND('',#15940,.T.);
#13259=FACE_OUTER_BOUND('',#15941,.T.);
#13260=FACE_OUTER_BOUND('',#15942,.T.);
#13261=FACE_OUTER_BOUND('',#15943,.T.);
#13262=FACE_OUTER_BOUND('',#15944,.T.);
#13263=FACE_OUTER_BOUND('',#15945,.T.);
#13264=FACE_OUTER_BOUND('',#15946,.T.);
#13265=FACE_OUTER_BOUND('',#15947,.T.);
#13266=FACE_OUTER_BOUND('',#15948,.T.);
#13267=FACE_OUTER_BOUND('',#15949,.T.);
#13268=FACE_OUTER_BOUND('',#15950,.T.);
#13269=FACE_OUTER_BOUND('',#15951,.T.);
#13270=FACE_OUTER_BOUND('',#15952,.T.);
#13271=FACE_OUTER_BOUND('',#15953,.T.);
#13272=FACE_OUTER_BOUND('',#15954,.T.);
#13273=FACE_OUTER_BOUND('',#15955,.T.);
#13274=FACE_OUTER_BOUND('',#15956,.T.);
#13275=FACE_OUTER_BOUND('',#15957,.T.);
#13276=FACE_OUTER_BOUND('',#15958,.T.);
#13277=FACE_OUTER_BOUND('',#15959,.T.);
#13278=FACE_OUTER_BOUND('',#15960,.T.);
#13279=FACE_OUTER_BOUND('',#15961,.T.);
#13280=FACE_OUTER_BOUND('',#15962,.T.);
#13281=FACE_OUTER_BOUND('',#15963,.T.);
#13282=FACE_OUTER_BOUND('',#15964,.T.);
#13283=FACE_OUTER_BOUND('',#15965,.T.);
#13284=FACE_OUTER_BOUND('',#15966,.T.);
#13285=FACE_OUTER_BOUND('',#15967,.T.);
#13286=FACE_OUTER_BOUND('',#15968,.T.);
#13287=FACE_OUTER_BOUND('',#15969,.T.);
#13288=FACE_OUTER_BOUND('',#15970,.T.);
#13289=FACE_OUTER_BOUND('',#15971,.T.);
#13290=FACE_OUTER_BOUND('',#15972,.T.);
#13291=FACE_OUTER_BOUND('',#15973,.T.);
#13292=FACE_OUTER_BOUND('',#15974,.T.);
#13293=FACE_OUTER_BOUND('',#15975,.T.);
#13294=FACE_OUTER_BOUND('',#15976,.T.);
#13295=FACE_OUTER_BOUND('',#15977,.T.);
#13296=FACE_OUTER_BOUND('',#15978,.T.);
#13297=FACE_OUTER_BOUND('',#15979,.T.);
#13298=FACE_OUTER_BOUND('',#15980,.T.);
#13299=FACE_OUTER_BOUND('',#15981,.T.);
#13300=FACE_OUTER_BOUND('',#15982,.T.);
#13301=FACE_OUTER_BOUND('',#15983,.T.);
#13302=FACE_OUTER_BOUND('',#15984,.T.);
#13303=FACE_OUTER_BOUND('',#15985,.T.);
#13304=FACE_OUTER_BOUND('',#15986,.T.);
#13305=FACE_OUTER_BOUND('',#15987,.T.);
#13306=FACE_OUTER_BOUND('',#15988,.T.);
#13307=FACE_OUTER_BOUND('',#15989,.T.);
#13308=FACE_OUTER_BOUND('',#15990,.T.);
#13309=FACE_OUTER_BOUND('',#15991,.T.);
#13310=FACE_OUTER_BOUND('',#15992,.T.);
#13311=FACE_OUTER_BOUND('',#15993,.T.);
#13312=FACE_OUTER_BOUND('',#15994,.T.);
#13313=FACE_OUTER_BOUND('',#15995,.T.);
#13314=FACE_OUTER_BOUND('',#15996,.T.);
#13315=FACE_OUTER_BOUND('',#15997,.T.);
#13316=FACE_OUTER_BOUND('',#15998,.T.);
#13317=FACE_OUTER_BOUND('',#15999,.T.);
#13318=FACE_OUTER_BOUND('',#16000,.T.);
#13319=FACE_OUTER_BOUND('',#16001,.T.);
#13320=FACE_OUTER_BOUND('',#16002,.T.);
#13321=FACE_OUTER_BOUND('',#16003,.T.);
#13322=FACE_OUTER_BOUND('',#16004,.T.);
#13323=FACE_OUTER_BOUND('',#16005,.T.);
#13324=FACE_OUTER_BOUND('',#16006,.T.);
#13325=FACE_OUTER_BOUND('',#16007,.T.);
#13326=FACE_OUTER_BOUND('',#16008,.T.);
#13327=FACE_OUTER_BOUND('',#16009,.T.);
#13328=FACE_OUTER_BOUND('',#16010,.T.);
#13329=FACE_OUTER_BOUND('',#16011,.T.);
#13330=FACE_OUTER_BOUND('',#16012,.T.);
#13331=FACE_OUTER_BOUND('',#16013,.T.);
#13332=FACE_OUTER_BOUND('',#16014,.T.);
#13333=FACE_OUTER_BOUND('',#16015,.T.);
#13334=FACE_OUTER_BOUND('',#16016,.T.);
#13335=FACE_OUTER_BOUND('',#16017,.T.);
#13336=FACE_OUTER_BOUND('',#16018,.T.);
#13337=FACE_OUTER_BOUND('',#16019,.T.);
#13338=FACE_OUTER_BOUND('',#16020,.T.);
#13339=FACE_OUTER_BOUND('',#16021,.T.);
#13340=FACE_OUTER_BOUND('',#16022,.T.);
#13341=FACE_OUTER_BOUND('',#16023,.T.);
#13342=FACE_OUTER_BOUND('',#16024,.T.);
#13343=FACE_OUTER_BOUND('',#16025,.T.);
#13344=FACE_OUTER_BOUND('',#16026,.T.);
#13345=FACE_OUTER_BOUND('',#16027,.T.);
#13346=FACE_OUTER_BOUND('',#16028,.T.);
#13347=FACE_OUTER_BOUND('',#16029,.T.);
#13348=FACE_OUTER_BOUND('',#16030,.T.);
#13349=FACE_OUTER_BOUND('',#16031,.T.);
#13350=FACE_OUTER_BOUND('',#16032,.T.);
#13351=FACE_OUTER_BOUND('',#16033,.T.);
#13352=FACE_OUTER_BOUND('',#16034,.T.);
#13353=FACE_OUTER_BOUND('',#16035,.T.);
#13354=FACE_OUTER_BOUND('',#16036,.T.);
#13355=FACE_OUTER_BOUND('',#16037,.T.);
#13356=FACE_OUTER_BOUND('',#16038,.T.);
#13357=FACE_OUTER_BOUND('',#16039,.T.);
#13358=FACE_OUTER_BOUND('',#16040,.T.);
#13359=FACE_OUTER_BOUND('',#16041,.T.);
#13360=FACE_OUTER_BOUND('',#16042,.T.);
#13361=FACE_OUTER_BOUND('',#16043,.T.);
#13362=FACE_OUTER_BOUND('',#16044,.T.);
#13363=FACE_OUTER_BOUND('',#16045,.T.);
#13364=FACE_OUTER_BOUND('',#16046,.T.);
#13365=FACE_OUTER_BOUND('',#16047,.T.);
#13366=FACE_OUTER_BOUND('',#16048,.T.);
#13367=FACE_OUTER_BOUND('',#16049,.T.);
#13368=FACE_OUTER_BOUND('',#16050,.T.);
#13369=FACE_OUTER_BOUND('',#16051,.T.);
#13370=FACE_OUTER_BOUND('',#16052,.T.);
#13371=FACE_OUTER_BOUND('',#16053,.T.);
#13372=FACE_OUTER_BOUND('',#16054,.T.);
#13373=FACE_OUTER_BOUND('',#16055,.T.);
#13374=FACE_OUTER_BOUND('',#16056,.T.);
#13375=FACE_OUTER_BOUND('',#16057,.T.);
#13376=FACE_OUTER_BOUND('',#16058,.T.);
#13377=FACE_OUTER_BOUND('',#16059,.T.);
#13378=FACE_OUTER_BOUND('',#16060,.T.);
#13379=FACE_OUTER_BOUND('',#16061,.T.);
#13380=FACE_OUTER_BOUND('',#16062,.T.);
#13381=FACE_OUTER_BOUND('',#16063,.T.);
#13382=FACE_OUTER_BOUND('',#16064,.T.);
#13383=FACE_OUTER_BOUND('',#16065,.T.);
#13384=FACE_OUTER_BOUND('',#16066,.T.);
#13385=FACE_OUTER_BOUND('',#16067,.T.);
#13386=FACE_OUTER_BOUND('',#16068,.T.);
#13387=FACE_OUTER_BOUND('',#16069,.T.);
#13388=FACE_OUTER_BOUND('',#16070,.T.);
#13389=FACE_OUTER_BOUND('',#16071,.T.);
#13390=FACE_OUTER_BOUND('',#16072,.T.);
#13391=FACE_OUTER_BOUND('',#16073,.T.);
#13392=FACE_OUTER_BOUND('',#16074,.T.);
#13393=FACE_OUTER_BOUND('',#16075,.T.);
#13394=FACE_OUTER_BOUND('',#16076,.T.);
#13395=FACE_OUTER_BOUND('',#16077,.T.);
#13396=FACE_OUTER_BOUND('',#16078,.T.);
#13397=FACE_OUTER_BOUND('',#16079,.T.);
#13398=FACE_OUTER_BOUND('',#16080,.T.);
#13399=FACE_OUTER_BOUND('',#16081,.T.);
#13400=FACE_OUTER_BOUND('',#16082,.T.);
#13401=FACE_OUTER_BOUND('',#16083,.T.);
#13402=FACE_OUTER_BOUND('',#16084,.T.);
#13403=FACE_OUTER_BOUND('',#16085,.T.);
#13404=FACE_OUTER_BOUND('',#16086,.T.);
#13405=FACE_OUTER_BOUND('',#16087,.T.);
#13406=FACE_OUTER_BOUND('',#16088,.T.);
#13407=FACE_OUTER_BOUND('',#16089,.T.);
#13408=FACE_OUTER_BOUND('',#16090,.T.);
#13409=FACE_OUTER_BOUND('',#16091,.T.);
#13410=FACE_OUTER_BOUND('',#16092,.T.);
#13411=FACE_OUTER_BOUND('',#16093,.T.);
#13412=FACE_OUTER_BOUND('',#16094,.T.);
#13413=FACE_OUTER_BOUND('',#16095,.T.);
#13414=FACE_OUTER_BOUND('',#16096,.T.);
#13415=FACE_OUTER_BOUND('',#16097,.T.);
#13416=FACE_OUTER_BOUND('',#16098,.T.);
#13417=FACE_OUTER_BOUND('',#16099,.T.);
#13418=FACE_OUTER_BOUND('',#16100,.T.);
#13419=FACE_OUTER_BOUND('',#16101,.T.);
#13420=FACE_OUTER_BOUND('',#16102,.T.);
#13421=FACE_OUTER_BOUND('',#16103,.T.);
#13422=FACE_OUTER_BOUND('',#16104,.T.);
#13423=FACE_OUTER_BOUND('',#16105,.T.);
#13424=FACE_OUTER_BOUND('',#16106,.T.);
#13425=FACE_OUTER_BOUND('',#16107,.T.);
#13426=FACE_OUTER_BOUND('',#16108,.T.);
#13427=FACE_OUTER_BOUND('',#16109,.T.);
#13428=FACE_OUTER_BOUND('',#16110,.T.);
#13429=FACE_OUTER_BOUND('',#16111,.T.);
#13430=FACE_OUTER_BOUND('',#16112,.T.);
#13431=FACE_OUTER_BOUND('',#16113,.T.);
#13432=FACE_OUTER_BOUND('',#16114,.T.);
#13433=FACE_OUTER_BOUND('',#16115,.T.);
#13434=FACE_OUTER_BOUND('',#16116,.T.);
#13435=FACE_OUTER_BOUND('',#16117,.T.);
#13436=FACE_OUTER_BOUND('',#16118,.T.);
#13437=FACE_OUTER_BOUND('',#16119,.T.);
#13438=FACE_OUTER_BOUND('',#16120,.T.);
#13439=FACE_OUTER_BOUND('',#16121,.T.);
#13440=FACE_OUTER_BOUND('',#16122,.T.);
#13441=FACE_OUTER_BOUND('',#16123,.T.);
#13442=FACE_OUTER_BOUND('',#16124,.T.);
#13443=FACE_OUTER_BOUND('',#16125,.T.);
#13444=FACE_OUTER_BOUND('',#16126,.T.);
#13445=FACE_OUTER_BOUND('',#16127,.T.);
#13446=FACE_OUTER_BOUND('',#16128,.T.);
#13447=FACE_OUTER_BOUND('',#16129,.T.);
#13448=FACE_OUTER_BOUND('',#16130,.T.);
#13449=FACE_OUTER_BOUND('',#16131,.T.);
#13450=FACE_OUTER_BOUND('',#16132,.T.);
#13451=FACE_OUTER_BOUND('',#16133,.T.);
#13452=FACE_OUTER_BOUND('',#16134,.T.);
#13453=FACE_OUTER_BOUND('',#16135,.T.);
#13454=FACE_OUTER_BOUND('',#16136,.T.);
#13455=FACE_OUTER_BOUND('',#16137,.T.);
#13456=FACE_OUTER_BOUND('',#16138,.T.);
#13457=FACE_OUTER_BOUND('',#16139,.T.);
#13458=FACE_OUTER_BOUND('',#16140,.T.);
#13459=FACE_OUTER_BOUND('',#16141,.T.);
#13460=FACE_OUTER_BOUND('',#16142,.T.);
#13461=FACE_OUTER_BOUND('',#16143,.T.);
#13462=FACE_OUTER_BOUND('',#16144,.T.);
#13463=FACE_OUTER_BOUND('',#16145,.T.);
#13464=FACE_OUTER_BOUND('',#16146,.T.);
#13465=FACE_OUTER_BOUND('',#16147,.T.);
#13466=FACE_OUTER_BOUND('',#16148,.T.);
#13467=FACE_OUTER_BOUND('',#16149,.T.);
#13468=FACE_OUTER_BOUND('',#16150,.T.);
#13469=FACE_OUTER_BOUND('',#16151,.T.);
#13470=FACE_OUTER_BOUND('',#16152,.T.);
#13471=FACE_OUTER_BOUND('',#16153,.T.);
#13472=FACE_OUTER_BOUND('',#16154,.T.);
#13473=FACE_OUTER_BOUND('',#16155,.T.);
#13474=FACE_OUTER_BOUND('',#16156,.T.);
#13475=FACE_OUTER_BOUND('',#16157,.T.);
#13476=FACE_OUTER_BOUND('',#16158,.T.);
#13477=FACE_OUTER_BOUND('',#16159,.T.);
#13478=FACE_OUTER_BOUND('',#16160,.T.);
#13479=FACE_OUTER_BOUND('',#16161,.T.);
#13480=FACE_OUTER_BOUND('',#16162,.T.);
#13481=FACE_OUTER_BOUND('',#16163,.T.);
#13482=FACE_OUTER_BOUND('',#16164,.T.);
#13483=FACE_OUTER_BOUND('',#16165,.T.);
#13484=FACE_OUTER_BOUND('',#16166,.T.);
#13485=FACE_OUTER_BOUND('',#16167,.T.);
#13486=FACE_OUTER_BOUND('',#16168,.T.);
#13487=FACE_OUTER_BOUND('',#16169,.T.);
#13488=FACE_OUTER_BOUND('',#16170,.T.);
#13489=FACE_OUTER_BOUND('',#16171,.T.);
#13490=FACE_OUTER_BOUND('',#16172,.T.);
#13491=FACE_OUTER_BOUND('',#16173,.T.);
#13492=FACE_OUTER_BOUND('',#16174,.T.);
#13493=FACE_OUTER_BOUND('',#16175,.T.);
#13494=FACE_OUTER_BOUND('',#16176,.T.);
#13495=FACE_OUTER_BOUND('',#16177,.T.);
#13496=FACE_OUTER_BOUND('',#16178,.T.);
#13497=FACE_OUTER_BOUND('',#16179,.T.);
#13498=FACE_OUTER_BOUND('',#16180,.T.);
#13499=FACE_OUTER_BOUND('',#16181,.T.);
#13500=FACE_OUTER_BOUND('',#16182,.T.);
#13501=FACE_OUTER_BOUND('',#16183,.T.);
#13502=FACE_OUTER_BOUND('',#16184,.T.);
#13503=FACE_OUTER_BOUND('',#16185,.T.);
#13504=FACE_OUTER_BOUND('',#16186,.T.);
#13505=FACE_OUTER_BOUND('',#16187,.T.);
#13506=FACE_OUTER_BOUND('',#16188,.T.);
#13507=FACE_OUTER_BOUND('',#16189,.T.);
#13508=FACE_OUTER_BOUND('',#16190,.T.);
#13509=FACE_OUTER_BOUND('',#16191,.T.);
#13510=FACE_OUTER_BOUND('',#16192,.T.);
#13511=FACE_OUTER_BOUND('',#16193,.T.);
#13512=FACE_OUTER_BOUND('',#16194,.T.);
#13513=FACE_OUTER_BOUND('',#16195,.T.);
#13514=FACE_OUTER_BOUND('',#16196,.T.);
#13515=FACE_OUTER_BOUND('',#16197,.T.);
#13516=FACE_OUTER_BOUND('',#16198,.T.);
#13517=FACE_OUTER_BOUND('',#16199,.T.);
#13518=FACE_OUTER_BOUND('',#16200,.T.);
#13519=FACE_OUTER_BOUND('',#16201,.T.);
#13520=FACE_OUTER_BOUND('',#16202,.T.);
#13521=FACE_OUTER_BOUND('',#16203,.T.);
#13522=FACE_OUTER_BOUND('',#16204,.T.);
#13523=FACE_OUTER_BOUND('',#16205,.T.);
#13524=FACE_OUTER_BOUND('',#16206,.T.);
#13525=FACE_OUTER_BOUND('',#16207,.T.);
#13526=FACE_OUTER_BOUND('',#16208,.T.);
#13527=FACE_OUTER_BOUND('',#16209,.T.);
#13528=FACE_OUTER_BOUND('',#16210,.T.);
#13529=FACE_OUTER_BOUND('',#16211,.T.);
#13530=FACE_OUTER_BOUND('',#16212,.T.);
#13531=FACE_OUTER_BOUND('',#16213,.T.);
#13532=FACE_OUTER_BOUND('',#16214,.T.);
#13533=FACE_OUTER_BOUND('',#16215,.T.);
#13534=FACE_OUTER_BOUND('',#16216,.T.);
#13535=FACE_OUTER_BOUND('',#16217,.T.);
#13536=FACE_OUTER_BOUND('',#16218,.T.);
#13537=FACE_OUTER_BOUND('',#16219,.T.);
#13538=FACE_OUTER_BOUND('',#16220,.T.);
#13539=FACE_OUTER_BOUND('',#16221,.T.);
#13540=FACE_OUTER_BOUND('',#16222,.T.);
#13541=FACE_OUTER_BOUND('',#16223,.T.);
#13542=FACE_OUTER_BOUND('',#16224,.T.);
#13543=FACE_OUTER_BOUND('',#16225,.T.);
#13544=FACE_OUTER_BOUND('',#16226,.T.);
#13545=FACE_OUTER_BOUND('',#16227,.T.);
#13546=FACE_OUTER_BOUND('',#16228,.T.);
#13547=FACE_OUTER_BOUND('',#16229,.T.);
#13548=FACE_OUTER_BOUND('',#16230,.T.);
#13549=FACE_OUTER_BOUND('',#16231,.T.);
#13550=FACE_OUTER_BOUND('',#16232,.T.);
#13551=FACE_OUTER_BOUND('',#16233,.T.);
#13552=FACE_OUTER_BOUND('',#16234,.T.);
#13553=FACE_OUTER_BOUND('',#16235,.T.);
#13554=FACE_OUTER_BOUND('',#16236,.T.);
#13555=FACE_OUTER_BOUND('',#16237,.T.);
#13556=FACE_OUTER_BOUND('',#16238,.T.);
#13557=FACE_OUTER_BOUND('',#16239,.T.);
#13558=FACE_OUTER_BOUND('',#16240,.T.);
#13559=FACE_OUTER_BOUND('',#16241,.T.);
#13560=FACE_OUTER_BOUND('',#16242,.T.);
#13561=FACE_OUTER_BOUND('',#16243,.T.);
#13562=FACE_OUTER_BOUND('',#16244,.T.);
#13563=FACE_OUTER_BOUND('',#16245,.T.);
#13564=FACE_OUTER_BOUND('',#16246,.T.);
#13565=FACE_OUTER_BOUND('',#16247,.T.);
#13566=FACE_OUTER_BOUND('',#16248,.T.);
#13567=FACE_OUTER_BOUND('',#16249,.T.);
#13568=FACE_OUTER_BOUND('',#16250,.T.);
#13569=FACE_OUTER_BOUND('',#16251,.T.);
#13570=FACE_OUTER_BOUND('',#16252,.T.);
#13571=FACE_OUTER_BOUND('',#16253,.T.);
#13572=FACE_OUTER_BOUND('',#16254,.T.);
#13573=FACE_OUTER_BOUND('',#16255,.T.);
#13574=FACE_OUTER_BOUND('',#16256,.T.);
#13575=FACE_OUTER_BOUND('',#16257,.T.);
#13576=FACE_OUTER_BOUND('',#16258,.T.);
#13577=FACE_OUTER_BOUND('',#16259,.T.);
#13578=FACE_OUTER_BOUND('',#16260,.T.);
#13579=FACE_OUTER_BOUND('',#16261,.T.);
#13580=FACE_OUTER_BOUND('',#16262,.T.);
#13581=FACE_OUTER_BOUND('',#16263,.T.);
#13582=FACE_OUTER_BOUND('',#16264,.T.);
#13583=FACE_OUTER_BOUND('',#16265,.T.);
#13584=FACE_OUTER_BOUND('',#16266,.T.);
#13585=FACE_OUTER_BOUND('',#16267,.T.);
#13586=FACE_OUTER_BOUND('',#16268,.T.);
#13587=FACE_OUTER_BOUND('',#16269,.T.);
#13588=FACE_OUTER_BOUND('',#16270,.T.);
#13589=FACE_OUTER_BOUND('',#16271,.T.);
#13590=FACE_OUTER_BOUND('',#16272,.T.);
#13591=FACE_OUTER_BOUND('',#16273,.T.);
#13592=FACE_OUTER_BOUND('',#16274,.T.);
#13593=FACE_OUTER_BOUND('',#16275,.T.);
#13594=FACE_OUTER_BOUND('',#16276,.T.);
#13595=FACE_OUTER_BOUND('',#16277,.T.);
#13596=FACE_OUTER_BOUND('',#16278,.T.);
#13597=FACE_OUTER_BOUND('',#16279,.T.);
#13598=FACE_OUTER_BOUND('',#16280,.T.);
#13599=FACE_OUTER_BOUND('',#16281,.T.);
#13600=FACE_OUTER_BOUND('',#16282,.T.);
#13601=FACE_OUTER_BOUND('',#16283,.T.);
#13602=FACE_OUTER_BOUND('',#16284,.T.);
#13603=FACE_OUTER_BOUND('',#16285,.T.);
#13604=FACE_OUTER_BOUND('',#16286,.T.);
#13605=FACE_OUTER_BOUND('',#16287,.T.);
#13606=FACE_OUTER_BOUND('',#16288,.T.);
#13607=FACE_OUTER_BOUND('',#16289,.T.);
#13608=FACE_OUTER_BOUND('',#16290,.T.);
#13609=FACE_OUTER_BOUND('',#16291,.T.);
#13610=FACE_OUTER_BOUND('',#16292,.T.);
#13611=FACE_OUTER_BOUND('',#16293,.T.);
#13612=FACE_OUTER_BOUND('',#16294,.T.);
#13613=FACE_OUTER_BOUND('',#16295,.T.);
#13614=FACE_OUTER_BOUND('',#16296,.T.);
#13615=FACE_OUTER_BOUND('',#16297,.T.);
#13616=FACE_OUTER_BOUND('',#16298,.T.);
#13617=FACE_OUTER_BOUND('',#16299,.T.);
#13618=FACE_OUTER_BOUND('',#16300,.T.);
#13619=FACE_OUTER_BOUND('',#16301,.T.);
#13620=FACE_OUTER_BOUND('',#16302,.T.);
#13621=FACE_OUTER_BOUND('',#16303,.T.);
#13622=FACE_OUTER_BOUND('',#16304,.T.);
#13623=FACE_OUTER_BOUND('',#16305,.T.);
#13624=FACE_OUTER_BOUND('',#16306,.T.);
#13625=FACE_OUTER_BOUND('',#16307,.T.);
#13626=FACE_OUTER_BOUND('',#16308,.T.);
#13627=FACE_OUTER_BOUND('',#16309,.T.);
#13628=FACE_OUTER_BOUND('',#16310,.T.);
#13629=FACE_OUTER_BOUND('',#16311,.T.);
#13630=FACE_OUTER_BOUND('',#16312,.T.);
#13631=FACE_OUTER_BOUND('',#16313,.T.);
#13632=FACE_OUTER_BOUND('',#16314,.T.);
#13633=FACE_OUTER_BOUND('',#16315,.T.);
#13634=FACE_OUTER_BOUND('',#16316,.T.);
#13635=FACE_OUTER_BOUND('',#16317,.T.);
#13636=FACE_OUTER_BOUND('',#16318,.T.);
#13637=FACE_OUTER_BOUND('',#16319,.T.);
#13638=FACE_OUTER_BOUND('',#16320,.T.);
#13639=FACE_OUTER_BOUND('',#16321,.T.);
#13640=FACE_OUTER_BOUND('',#16322,.T.);
#13641=FACE_OUTER_BOUND('',#16323,.T.);
#13642=FACE_OUTER_BOUND('',#16324,.T.);
#13643=FACE_OUTER_BOUND('',#16325,.T.);
#13644=FACE_OUTER_BOUND('',#16326,.T.);
#13645=FACE_OUTER_BOUND('',#16327,.T.);
#13646=FACE_OUTER_BOUND('',#16328,.T.);
#13647=FACE_OUTER_BOUND('',#16329,.T.);
#13648=FACE_OUTER_BOUND('',#16330,.T.);
#13649=FACE_OUTER_BOUND('',#16331,.T.);
#13650=FACE_OUTER_BOUND('',#16332,.T.);
#13651=FACE_OUTER_BOUND('',#16333,.T.);
#13652=FACE_OUTER_BOUND('',#16334,.T.);
#13653=FACE_OUTER_BOUND('',#16335,.T.);
#13654=FACE_OUTER_BOUND('',#16336,.T.);
#13655=FACE_OUTER_BOUND('',#16337,.T.);
#13656=FACE_OUTER_BOUND('',#16338,.T.);
#13657=FACE_OUTER_BOUND('',#16339,.T.);
#13658=FACE_OUTER_BOUND('',#16340,.T.);
#13659=FACE_OUTER_BOUND('',#16341,.T.);
#13660=FACE_OUTER_BOUND('',#16342,.T.);
#13661=FACE_OUTER_BOUND('',#16343,.T.);
#13662=FACE_OUTER_BOUND('',#16344,.T.);
#13663=FACE_OUTER_BOUND('',#16345,.T.);
#13664=FACE_OUTER_BOUND('',#16346,.T.);
#13665=FACE_OUTER_BOUND('',#16347,.T.);
#13666=FACE_OUTER_BOUND('',#16348,.T.);
#13667=FACE_OUTER_BOUND('',#16349,.T.);
#13668=FACE_OUTER_BOUND('',#16350,.T.);
#13669=FACE_OUTER_BOUND('',#16351,.T.);
#13670=FACE_OUTER_BOUND('',#16352,.T.);
#13671=FACE_OUTER_BOUND('',#16353,.T.);
#13672=FACE_OUTER_BOUND('',#16354,.T.);
#13673=FACE_OUTER_BOUND('',#16355,.T.);
#13674=FACE_OUTER_BOUND('',#16356,.T.);
#13675=FACE_OUTER_BOUND('',#16357,.T.);
#13676=FACE_OUTER_BOUND('',#16358,.T.);
#13677=FACE_OUTER_BOUND('',#16359,.T.);
#13678=FACE_OUTER_BOUND('',#16360,.T.);
#13679=FACE_OUTER_BOUND('',#16361,.T.);
#13680=FACE_OUTER_BOUND('',#16362,.T.);
#13681=FACE_OUTER_BOUND('',#16363,.T.);
#13682=FACE_OUTER_BOUND('',#16364,.T.);
#13683=FACE_OUTER_BOUND('',#16365,.T.);
#13684=FACE_OUTER_BOUND('',#16366,.T.);
#13685=FACE_OUTER_BOUND('',#16367,.T.);
#13686=FACE_OUTER_BOUND('',#16368,.T.);
#13687=FACE_OUTER_BOUND('',#16369,.T.);
#13688=FACE_OUTER_BOUND('',#16370,.T.);
#13689=FACE_OUTER_BOUND('',#16371,.T.);
#13690=FACE_OUTER_BOUND('',#16372,.T.);
#13691=FACE_OUTER_BOUND('',#16373,.T.);
#13692=FACE_OUTER_BOUND('',#16374,.T.);
#13693=FACE_OUTER_BOUND('',#16375,.T.);
#13694=FACE_OUTER_BOUND('',#16376,.T.);
#13695=FACE_OUTER_BOUND('',#16377,.T.);
#13696=FACE_OUTER_BOUND('',#16378,.T.);
#13697=FACE_OUTER_BOUND('',#16379,.T.);
#13698=FACE_OUTER_BOUND('',#16380,.T.);
#13699=FACE_OUTER_BOUND('',#16381,.T.);
#13700=FACE_OUTER_BOUND('',#16382,.T.);
#13701=FACE_OUTER_BOUND('',#16383,.T.);
#13702=FACE_OUTER_BOUND('',#16384,.T.);
#13703=FACE_OUTER_BOUND('',#16385,.T.);
#13704=FACE_OUTER_BOUND('',#16386,.T.);
#13705=FACE_OUTER_BOUND('',#16387,.T.);
#13706=FACE_OUTER_BOUND('',#16388,.T.);
#13707=FACE_OUTER_BOUND('',#16389,.T.);
#13708=FACE_OUTER_BOUND('',#16390,.T.);
#13709=FACE_OUTER_BOUND('',#16391,.T.);
#13710=FACE_OUTER_BOUND('',#16392,.T.);
#13711=FACE_OUTER_BOUND('',#16393,.T.);
#13712=FACE_OUTER_BOUND('',#16394,.T.);
#13713=FACE_OUTER_BOUND('',#16395,.T.);
#13714=FACE_OUTER_BOUND('',#16396,.T.);
#13715=FACE_OUTER_BOUND('',#16397,.T.);
#13716=FACE_OUTER_BOUND('',#16398,.T.);
#13717=FACE_OUTER_BOUND('',#16399,.T.);
#13718=FACE_OUTER_BOUND('',#16400,.T.);
#13719=FACE_OUTER_BOUND('',#16401,.T.);
#13720=FACE_OUTER_BOUND('',#16402,.T.);
#13721=FACE_OUTER_BOUND('',#16403,.T.);
#13722=FACE_OUTER_BOUND('',#16404,.T.);
#13723=FACE_OUTER_BOUND('',#16405,.T.);
#13724=FACE_OUTER_BOUND('',#16406,.T.);
#13725=FACE_OUTER_BOUND('',#16407,.T.);
#13726=FACE_OUTER_BOUND('',#16408,.T.);
#13727=FACE_OUTER_BOUND('',#16409,.T.);
#13728=FACE_OUTER_BOUND('',#16410,.T.);
#13729=FACE_OUTER_BOUND('',#16411,.T.);
#13730=FACE_OUTER_BOUND('',#16412,.T.);
#13731=FACE_OUTER_BOUND('',#16413,.T.);
#13732=FACE_OUTER_BOUND('',#16414,.T.);
#13733=FACE_OUTER_BOUND('',#16415,.T.);
#13734=FACE_OUTER_BOUND('',#16416,.T.);
#13735=FACE_OUTER_BOUND('',#16417,.T.);
#13736=FACE_OUTER_BOUND('',#16418,.T.);
#13737=FACE_OUTER_BOUND('',#16419,.T.);
#13738=FACE_OUTER_BOUND('',#16420,.T.);
#13739=FACE_OUTER_BOUND('',#16421,.T.);
#13740=FACE_OUTER_BOUND('',#16422,.T.);
#13741=FACE_OUTER_BOUND('',#16423,.T.);
#13742=FACE_OUTER_BOUND('',#16424,.T.);
#13743=FACE_OUTER_BOUND('',#16425,.T.);
#13744=FACE_OUTER_BOUND('',#16426,.T.);
#13745=FACE_OUTER_BOUND('',#16427,.T.);
#13746=FACE_OUTER_BOUND('',#16428,.T.);
#13747=FACE_OUTER_BOUND('',#16429,.T.);
#13748=FACE_OUTER_BOUND('',#16430,.T.);
#13749=FACE_OUTER_BOUND('',#16431,.T.);
#13750=FACE_OUTER_BOUND('',#16432,.T.);
#13751=FACE_OUTER_BOUND('',#16433,.T.);
#13752=FACE_OUTER_BOUND('',#16434,.T.);
#13753=FACE_OUTER_BOUND('',#16435,.T.);
#13754=FACE_OUTER_BOUND('',#16436,.T.);
#13755=FACE_OUTER_BOUND('',#16437,.T.);
#13756=FACE_OUTER_BOUND('',#16438,.T.);
#13757=FACE_OUTER_BOUND('',#16439,.T.);
#13758=FACE_OUTER_BOUND('',#16440,.T.);
#13759=FACE_OUTER_BOUND('',#16441,.T.);
#13760=FACE_OUTER_BOUND('',#16442,.T.);
#13761=FACE_OUTER_BOUND('',#16443,.T.);
#13762=FACE_OUTER_BOUND('',#16444,.T.);
#13763=FACE_OUTER_BOUND('',#16445,.T.);
#13764=FACE_OUTER_BOUND('',#16446,.T.);
#13765=FACE_OUTER_BOUND('',#16447,.T.);
#13766=FACE_OUTER_BOUND('',#16448,.T.);
#13767=FACE_OUTER_BOUND('',#16449,.T.);
#13768=FACE_OUTER_BOUND('',#16450,.T.);
#13769=FACE_OUTER_BOUND('',#16451,.T.);
#13770=FACE_OUTER_BOUND('',#16452,.T.);
#13771=FACE_OUTER_BOUND('',#16453,.T.);
#13772=FACE_OUTER_BOUND('',#16454,.T.);
#13773=FACE_OUTER_BOUND('',#16455,.T.);
#13774=FACE_OUTER_BOUND('',#16456,.T.);
#13775=FACE_OUTER_BOUND('',#16457,.T.);
#13776=FACE_OUTER_BOUND('',#16458,.T.);
#13777=FACE_OUTER_BOUND('',#16459,.T.);
#13778=FACE_OUTER_BOUND('',#16460,.T.);
#13779=FACE_OUTER_BOUND('',#16461,.T.);
#13780=FACE_OUTER_BOUND('',#16462,.T.);
#13781=FACE_OUTER_BOUND('',#16463,.T.);
#13782=FACE_OUTER_BOUND('',#16464,.T.);
#13783=FACE_OUTER_BOUND('',#16465,.T.);
#13784=FACE_OUTER_BOUND('',#16466,.T.);
#13785=FACE_OUTER_BOUND('',#16467,.T.);
#13786=FACE_OUTER_BOUND('',#16468,.T.);
#13787=FACE_OUTER_BOUND('',#16469,.T.);
#13788=FACE_OUTER_BOUND('',#16470,.T.);
#13789=FACE_OUTER_BOUND('',#16471,.T.);
#13790=FACE_OUTER_BOUND('',#16472,.T.);
#13791=FACE_OUTER_BOUND('',#16473,.T.);
#13792=FACE_OUTER_BOUND('',#16474,.T.);
#13793=FACE_OUTER_BOUND('',#16475,.T.);
#13794=FACE_OUTER_BOUND('',#16476,.T.);
#13795=FACE_OUTER_BOUND('',#16477,.T.);
#13796=FACE_OUTER_BOUND('',#16478,.T.);
#13797=FACE_OUTER_BOUND('',#16479,.T.);
#13798=FACE_OUTER_BOUND('',#16480,.T.);
#13799=FACE_OUTER_BOUND('',#16481,.T.);
#13800=FACE_OUTER_BOUND('',#16482,.T.);
#13801=FACE_OUTER_BOUND('',#16483,.T.);
#13802=FACE_OUTER_BOUND('',#16484,.T.);
#13803=FACE_OUTER_BOUND('',#16485,.T.);
#13804=FACE_OUTER_BOUND('',#16486,.T.);
#13805=FACE_OUTER_BOUND('',#16487,.T.);
#13806=FACE_OUTER_BOUND('',#16488,.T.);
#13807=FACE_OUTER_BOUND('',#16489,.T.);
#13808=FACE_OUTER_BOUND('',#16490,.T.);
#13809=FACE_OUTER_BOUND('',#16491,.T.);
#13810=FACE_OUTER_BOUND('',#16492,.T.);
#13811=FACE_OUTER_BOUND('',#16493,.T.);
#13812=FACE_OUTER_BOUND('',#16494,.T.);
#13813=FACE_OUTER_BOUND('',#16495,.T.);
#13814=FACE_OUTER_BOUND('',#16496,.T.);
#13815=FACE_OUTER_BOUND('',#16497,.T.);
#13816=FACE_OUTER_BOUND('',#16498,.T.);
#13817=FACE_OUTER_BOUND('',#16499,.T.);
#13818=FACE_OUTER_BOUND('',#16500,.T.);
#13819=FACE_OUTER_BOUND('',#16501,.T.);
#13820=FACE_OUTER_BOUND('',#16502,.T.);
#13821=FACE_OUTER_BOUND('',#16503,.T.);
#13822=FACE_OUTER_BOUND('',#16504,.T.);
#13823=FACE_OUTER_BOUND('',#16505,.T.);
#13824=FACE_OUTER_BOUND('',#16506,.T.);
#13825=FACE_OUTER_BOUND('',#16507,.T.);
#13826=FACE_OUTER_BOUND('',#16508,.T.);
#13827=FACE_OUTER_BOUND('',#16509,.T.);
#13828=FACE_OUTER_BOUND('',#16510,.T.);
#13829=FACE_OUTER_BOUND('',#16511,.T.);
#13830=FACE_OUTER_BOUND('',#16512,.T.);
#13831=FACE_OUTER_BOUND('',#16513,.T.);
#13832=FACE_OUTER_BOUND('',#16514,.T.);
#13833=FACE_OUTER_BOUND('',#16515,.T.);
#13834=FACE_OUTER_BOUND('',#16516,.T.);
#13835=FACE_OUTER_BOUND('',#16517,.T.);
#13836=FACE_OUTER_BOUND('',#16518,.T.);
#13837=FACE_OUTER_BOUND('',#16519,.T.);
#13838=FACE_OUTER_BOUND('',#16520,.T.);
#13839=FACE_OUTER_BOUND('',#16521,.T.);
#13840=FACE_OUTER_BOUND('',#16522,.T.);
#13841=FACE_OUTER_BOUND('',#16523,.T.);
#13842=FACE_OUTER_BOUND('',#16524,.T.);
#13843=FACE_OUTER_BOUND('',#16525,.T.);
#13844=FACE_OUTER_BOUND('',#16526,.T.);
#13845=FACE_OUTER_BOUND('',#16527,.T.);
#13846=FACE_OUTER_BOUND('',#16528,.T.);
#13847=FACE_OUTER_BOUND('',#16529,.T.);
#13848=FACE_OUTER_BOUND('',#16530,.T.);
#13849=FACE_OUTER_BOUND('',#16531,.T.);
#13850=FACE_OUTER_BOUND('',#16532,.T.);
#13851=FACE_OUTER_BOUND('',#16533,.T.);
#13852=FACE_OUTER_BOUND('',#16534,.T.);
#13853=FACE_OUTER_BOUND('',#16535,.T.);
#13854=FACE_OUTER_BOUND('',#16536,.T.);
#13855=FACE_OUTER_BOUND('',#16537,.T.);
#13856=FACE_OUTER_BOUND('',#16538,.T.);
#13857=FACE_OUTER_BOUND('',#16539,.T.);
#13858=FACE_OUTER_BOUND('',#16540,.T.);
#13859=FACE_OUTER_BOUND('',#16541,.T.);
#13860=FACE_OUTER_BOUND('',#16542,.T.);
#13861=FACE_OUTER_BOUND('',#16543,.T.);
#13862=FACE_OUTER_BOUND('',#16544,.T.);
#13863=FACE_OUTER_BOUND('',#16545,.T.);
#13864=FACE_OUTER_BOUND('',#16546,.T.);
#13865=FACE_OUTER_BOUND('',#16547,.T.);
#13866=FACE_OUTER_BOUND('',#16548,.T.);
#13867=FACE_OUTER_BOUND('',#16549,.T.);
#13868=FACE_OUTER_BOUND('',#16550,.T.);
#13869=FACE_OUTER_BOUND('',#16551,.T.);
#13870=FACE_OUTER_BOUND('',#16552,.T.);
#13871=FACE_OUTER_BOUND('',#16553,.T.);
#13872=FACE_OUTER_BOUND('',#16554,.T.);
#13873=FACE_OUTER_BOUND('',#16555,.T.);
#13874=FACE_OUTER_BOUND('',#16556,.T.);
#13875=FACE_OUTER_BOUND('',#16557,.T.);
#13876=FACE_OUTER_BOUND('',#16558,.T.);
#13877=FACE_OUTER_BOUND('',#16559,.T.);
#13878=FACE_OUTER_BOUND('',#16560,.T.);
#13879=FACE_OUTER_BOUND('',#16561,.T.);
#13880=FACE_OUTER_BOUND('',#16562,.T.);
#13881=FACE_OUTER_BOUND('',#16563,.T.);
#13882=FACE_OUTER_BOUND('',#16564,.T.);
#13883=FACE_OUTER_BOUND('',#16565,.T.);
#13884=FACE_OUTER_BOUND('',#16566,.T.);
#13885=FACE_OUTER_BOUND('',#16567,.T.);
#13886=FACE_OUTER_BOUND('',#16568,.T.);
#13887=FACE_OUTER_BOUND('',#16569,.T.);
#13888=FACE_OUTER_BOUND('',#16570,.T.);
#13889=FACE_OUTER_BOUND('',#16571,.T.);
#13890=FACE_OUTER_BOUND('',#16572,.T.);
#13891=FACE_OUTER_BOUND('',#16573,.T.);
#13892=FACE_OUTER_BOUND('',#16574,.T.);
#13893=FACE_OUTER_BOUND('',#16575,.T.);
#13894=FACE_OUTER_BOUND('',#16576,.T.);
#13895=FACE_OUTER_BOUND('',#16577,.T.);
#13896=FACE_OUTER_BOUND('',#16578,.T.);
#13897=FACE_OUTER_BOUND('',#16579,.T.);
#13898=FACE_OUTER_BOUND('',#16580,.T.);
#13899=FACE_OUTER_BOUND('',#16581,.T.);
#13900=FACE_OUTER_BOUND('',#16582,.T.);
#13901=FACE_OUTER_BOUND('',#16583,.T.);
#13902=FACE_OUTER_BOUND('',#16584,.T.);
#13903=FACE_OUTER_BOUND('',#16585,.T.);
#13904=FACE_OUTER_BOUND('',#16586,.T.);
#13905=FACE_OUTER_BOUND('',#16587,.T.);
#13906=FACE_OUTER_BOUND('',#16588,.T.);
#13907=FACE_OUTER_BOUND('',#16589,.T.);
#13908=FACE_OUTER_BOUND('',#16590,.T.);
#13909=FACE_OUTER_BOUND('',#16591,.T.);
#13910=FACE_OUTER_BOUND('',#16592,.T.);
#13911=FACE_OUTER_BOUND('',#16593,.T.);
#13912=FACE_OUTER_BOUND('',#16594,.T.);
#13913=FACE_OUTER_BOUND('',#16595,.T.);
#13914=FACE_OUTER_BOUND('',#16596,.T.);
#13915=FACE_OUTER_BOUND('',#16597,.T.);
#13916=FACE_OUTER_BOUND('',#16598,.T.);
#13917=FACE_OUTER_BOUND('',#16599,.T.);
#13918=FACE_OUTER_BOUND('',#16600,.T.);
#13919=FACE_OUTER_BOUND('',#16601,.T.);
#13920=FACE_OUTER_BOUND('',#16602,.T.);
#13921=FACE_OUTER_BOUND('',#16603,.T.);
#13922=FACE_OUTER_BOUND('',#16604,.T.);
#13923=FACE_OUTER_BOUND('',#16605,.T.);
#13924=FACE_OUTER_BOUND('',#16606,.T.);
#13925=FACE_OUTER_BOUND('',#16607,.T.);
#13926=FACE_OUTER_BOUND('',#16608,.T.);
#13927=FACE_OUTER_BOUND('',#16609,.T.);
#13928=FACE_OUTER_BOUND('',#16610,.T.);
#13929=FACE_OUTER_BOUND('',#16611,.T.);
#13930=FACE_OUTER_BOUND('',#16612,.T.);
#13931=FACE_OUTER_BOUND('',#16613,.T.);
#13932=FACE_OUTER_BOUND('',#16614,.T.);
#13933=FACE_OUTER_BOUND('',#16615,.T.);
#13934=FACE_OUTER_BOUND('',#16616,.T.);
#13935=FACE_OUTER_BOUND('',#16617,.T.);
#13936=FACE_OUTER_BOUND('',#16618,.T.);
#13937=FACE_OUTER_BOUND('',#16619,.T.);
#13938=FACE_OUTER_BOUND('',#16620,.T.);
#13939=FACE_OUTER_BOUND('',#16621,.T.);
#13940=FACE_OUTER_BOUND('',#16622,.T.);
#13941=FACE_OUTER_BOUND('',#16623,.T.);
#13942=FACE_OUTER_BOUND('',#16624,.T.);
#13943=FACE_OUTER_BOUND('',#16625,.T.);
#13944=FACE_OUTER_BOUND('',#16626,.T.);
#13945=FACE_OUTER_BOUND('',#16627,.T.);
#13946=FACE_OUTER_BOUND('',#16628,.T.);
#13947=FACE_OUTER_BOUND('',#16629,.T.);
#13948=FACE_OUTER_BOUND('',#16630,.T.);
#13949=FACE_OUTER_BOUND('',#16631,.T.);
#13950=FACE_OUTER_BOUND('',#16632,.T.);
#13951=FACE_OUTER_BOUND('',#16633,.T.);
#13952=FACE_OUTER_BOUND('',#16634,.T.);
#13953=FACE_OUTER_BOUND('',#16635,.T.);
#13954=FACE_OUTER_BOUND('',#16636,.T.);
#13955=FACE_OUTER_BOUND('',#16637,.T.);
#13956=FACE_OUTER_BOUND('',#16638,.T.);
#13957=FACE_OUTER_BOUND('',#16639,.T.);
#13958=FACE_OUTER_BOUND('',#16640,.T.);
#13959=FACE_OUTER_BOUND('',#16641,.T.);
#13960=FACE_OUTER_BOUND('',#16642,.T.);
#13961=FACE_OUTER_BOUND('',#16643,.T.);
#13962=FACE_OUTER_BOUND('',#16644,.T.);
#13963=FACE_OUTER_BOUND('',#16645,.T.);
#13964=FACE_OUTER_BOUND('',#16646,.T.);
#13965=FACE_OUTER_BOUND('',#16647,.T.);
#13966=FACE_OUTER_BOUND('',#16648,.T.);
#13967=FACE_OUTER_BOUND('',#16649,.T.);
#13968=FACE_OUTER_BOUND('',#16650,.T.);
#13969=FACE_OUTER_BOUND('',#16651,.T.);
#13970=FACE_OUTER_BOUND('',#16652,.T.);
#13971=FACE_OUTER_BOUND('',#16653,.T.);
#13972=FACE_OUTER_BOUND('',#16654,.T.);
#13973=FACE_OUTER_BOUND('',#16655,.T.);
#13974=FACE_OUTER_BOUND('',#16656,.T.);
#13975=FACE_OUTER_BOUND('',#16657,.T.);
#13976=FACE_OUTER_BOUND('',#16658,.T.);
#13977=FACE_OUTER_BOUND('',#16659,.T.);
#13978=FACE_OUTER_BOUND('',#16660,.T.);
#13979=FACE_OUTER_BOUND('',#16661,.T.);
#13980=FACE_OUTER_BOUND('',#16662,.T.);
#13981=FACE_OUTER_BOUND('',#16663,.T.);
#13982=FACE_OUTER_BOUND('',#16664,.T.);
#13983=FACE_OUTER_BOUND('',#16665,.T.);
#13984=FACE_OUTER_BOUND('',#16666,.T.);
#13985=FACE_OUTER_BOUND('',#16667,.T.);
#13986=FACE_OUTER_BOUND('',#16668,.T.);
#13987=FACE_OUTER_BOUND('',#16669,.T.);
#13988=FACE_OUTER_BOUND('',#16670,.T.);
#13989=FACE_OUTER_BOUND('',#16671,.T.);
#13990=FACE_OUTER_BOUND('',#16672,.T.);
#13991=FACE_OUTER_BOUND('',#16673,.T.);
#13992=FACE_OUTER_BOUND('',#16674,.T.);
#13993=FACE_OUTER_BOUND('',#16675,.T.);
#13994=FACE_OUTER_BOUND('',#16676,.T.);
#13995=FACE_OUTER_BOUND('',#16677,.T.);
#13996=FACE_OUTER_BOUND('',#16678,.T.);
#13997=FACE_OUTER_BOUND('',#16679,.T.);
#13998=FACE_OUTER_BOUND('',#16680,.T.);
#13999=FACE_OUTER_BOUND('',#16681,.T.);
#14000=FACE_OUTER_BOUND('',#16682,.T.);
#14001=FACE_OUTER_BOUND('',#16683,.T.);
#14002=FACE_OUTER_BOUND('',#16684,.T.);
#14003=FACE_OUTER_BOUND('',#16685,.T.);
#14004=FACE_OUTER_BOUND('',#16686,.T.);
#14005=FACE_OUTER_BOUND('',#16687,.T.);
#14006=FACE_OUTER_BOUND('',#16688,.T.);
#14007=FACE_OUTER_BOUND('',#16689,.T.);
#14008=FACE_OUTER_BOUND('',#16690,.T.);
#14009=FACE_OUTER_BOUND('',#16691,.T.);
#14010=FACE_OUTER_BOUND('',#16692,.T.);
#14011=FACE_OUTER_BOUND('',#16693,.T.);
#14012=FACE_OUTER_BOUND('',#16694,.T.);
#14013=FACE_OUTER_BOUND('',#16695,.T.);
#14014=FACE_OUTER_BOUND('',#16696,.T.);
#14015=FACE_OUTER_BOUND('',#16697,.T.);
#14016=FACE_OUTER_BOUND('',#16698,.T.);
#14017=FACE_OUTER_BOUND('',#16699,.T.);
#14018=FACE_OUTER_BOUND('',#16700,.T.);
#14019=FACE_OUTER_BOUND('',#16701,.T.);
#14020=FACE_OUTER_BOUND('',#16702,.T.);
#14021=FACE_OUTER_BOUND('',#16703,.T.);
#14022=FACE_OUTER_BOUND('',#16704,.T.);
#14023=FACE_OUTER_BOUND('',#16705,.T.);
#14024=FACE_OUTER_BOUND('',#16706,.T.);
#14025=FACE_OUTER_BOUND('',#16707,.T.);
#14026=FACE_OUTER_BOUND('',#16708,.T.);
#14027=FACE_OUTER_BOUND('',#16709,.T.);
#14028=FACE_OUTER_BOUND('',#16710,.T.);
#14029=FACE_OUTER_BOUND('',#16711,.T.);
#14030=FACE_OUTER_BOUND('',#16712,.T.);
#14031=FACE_OUTER_BOUND('',#16713,.T.);
#14032=FACE_OUTER_BOUND('',#16714,.T.);
#14033=FACE_OUTER_BOUND('',#16715,.T.);
#14034=FACE_OUTER_BOUND('',#16716,.T.);
#14035=FACE_OUTER_BOUND('',#16717,.T.);
#14036=FACE_OUTER_BOUND('',#16718,.T.);
#14037=FACE_OUTER_BOUND('',#16719,.T.);
#14038=FACE_OUTER_BOUND('',#16720,.T.);
#14039=FACE_OUTER_BOUND('',#16721,.T.);
#14040=FACE_OUTER_BOUND('',#16722,.T.);
#14041=FACE_OUTER_BOUND('',#16723,.T.);
#14042=FACE_OUTER_BOUND('',#16724,.T.);
#14043=FACE_OUTER_BOUND('',#16725,.T.);
#14044=FACE_OUTER_BOUND('',#16726,.T.);
#14045=FACE_OUTER_BOUND('',#16727,.T.);
#14046=FACE_OUTER_BOUND('',#16728,.T.);
#14047=FACE_OUTER_BOUND('',#16729,.T.);
#14048=FACE_OUTER_BOUND('',#16730,.T.);
#14049=FACE_OUTER_BOUND('',#16731,.T.);
#14050=FACE_OUTER_BOUND('',#16732,.T.);
#14051=FACE_OUTER_BOUND('',#16733,.T.);
#14052=FACE_OUTER_BOUND('',#16734,.T.);
#14053=FACE_OUTER_BOUND('',#16735,.T.);
#14054=FACE_OUTER_BOUND('',#16736,.T.);
#14055=FACE_OUTER_BOUND('',#16737,.T.);
#14056=FACE_OUTER_BOUND('',#16738,.T.);
#14057=FACE_OUTER_BOUND('',#16739,.T.);
#14058=FACE_OUTER_BOUND('',#16740,.T.);
#14059=FACE_OUTER_BOUND('',#16741,.T.);
#14060=FACE_OUTER_BOUND('',#16742,.T.);
#14061=FACE_OUTER_BOUND('',#16743,.T.);
#14062=FACE_OUTER_BOUND('',#16744,.T.);
#14063=FACE_OUTER_BOUND('',#16745,.T.);
#14064=FACE_OUTER_BOUND('',#16746,.T.);
#14065=FACE_OUTER_BOUND('',#16747,.T.);
#14066=FACE_OUTER_BOUND('',#16748,.T.);
#14067=FACE_OUTER_BOUND('',#16749,.T.);
#14068=FACE_OUTER_BOUND('',#16750,.T.);
#14069=FACE_OUTER_BOUND('',#16751,.T.);
#14070=FACE_OUTER_BOUND('',#16752,.T.);
#14071=FACE_OUTER_BOUND('',#16753,.T.);
#14072=FACE_OUTER_BOUND('',#16754,.T.);
#14073=FACE_OUTER_BOUND('',#16755,.T.);
#14074=FACE_OUTER_BOUND('',#16756,.T.);
#14075=FACE_OUTER_BOUND('',#16757,.T.);
#14076=FACE_OUTER_BOUND('',#16758,.T.);
#14077=FACE_OUTER_BOUND('',#16759,.T.);
#14078=FACE_OUTER_BOUND('',#16760,.T.);
#14079=FACE_OUTER_BOUND('',#16761,.T.);
#14080=FACE_OUTER_BOUND('',#16762,.T.);
#14081=FACE_OUTER_BOUND('',#16763,.T.);
#14082=FACE_OUTER_BOUND('',#16764,.T.);
#14083=FACE_OUTER_BOUND('',#16765,.T.);
#14084=FACE_OUTER_BOUND('',#16766,.T.);
#14085=FACE_OUTER_BOUND('',#16767,.T.);
#14086=FACE_OUTER_BOUND('',#16768,.T.);
#14087=FACE_OUTER_BOUND('',#16769,.T.);
#14088=FACE_OUTER_BOUND('',#16770,.T.);
#14089=FACE_OUTER_BOUND('',#16771,.T.);
#14090=FACE_OUTER_BOUND('',#16772,.T.);
#14091=FACE_OUTER_BOUND('',#16773,.T.);
#14092=FACE_OUTER_BOUND('',#16774,.T.);
#14093=FACE_OUTER_BOUND('',#16775,.T.);
#14094=FACE_OUTER_BOUND('',#16776,.T.);
#14095=FACE_OUTER_BOUND('',#16777,.T.);
#14096=FACE_OUTER_BOUND('',#16778,.T.);
#14097=FACE_OUTER_BOUND('',#16779,.T.);
#14098=FACE_OUTER_BOUND('',#16780,.T.);
#14099=FACE_OUTER_BOUND('',#16781,.T.);
#14100=FACE_OUTER_BOUND('',#16782,.T.);
#14101=FACE_OUTER_BOUND('',#16783,.T.);
#14102=FACE_OUTER_BOUND('',#16784,.T.);
#14103=FACE_OUTER_BOUND('',#16785,.T.);
#14104=FACE_OUTER_BOUND('',#16786,.T.);
#14105=FACE_OUTER_BOUND('',#16787,.T.);
#14106=FACE_OUTER_BOUND('',#16788,.T.);
#14107=FACE_OUTER_BOUND('',#16789,.T.);
#14108=FACE_OUTER_BOUND('',#16790,.T.);
#14109=FACE_OUTER_BOUND('',#16791,.T.);
#14110=FACE_OUTER_BOUND('',#16792,.T.);
#14111=FACE_OUTER_BOUND('',#16793,.T.);
#14112=FACE_OUTER_BOUND('',#16794,.T.);
#14113=FACE_OUTER_BOUND('',#16795,.T.);
#14114=FACE_OUTER_BOUND('',#16796,.T.);
#14115=FACE_OUTER_BOUND('',#16797,.T.);
#14116=FACE_OUTER_BOUND('',#16798,.T.);
#14117=FACE_OUTER_BOUND('',#16799,.T.);
#14118=FACE_OUTER_BOUND('',#16800,.T.);
#14119=FACE_OUTER_BOUND('',#16801,.T.);
#14120=FACE_OUTER_BOUND('',#16802,.T.);
#14121=FACE_OUTER_BOUND('',#16803,.T.);
#14122=FACE_OUTER_BOUND('',#16804,.T.);
#14123=FACE_OUTER_BOUND('',#16805,.T.);
#14124=FACE_OUTER_BOUND('',#16806,.T.);
#14125=FACE_OUTER_BOUND('',#16807,.T.);
#14126=FACE_OUTER_BOUND('',#16808,.T.);
#14127=FACE_OUTER_BOUND('',#16809,.T.);
#14128=FACE_OUTER_BOUND('',#16810,.T.);
#14129=FACE_OUTER_BOUND('',#16811,.T.);
#14130=FACE_OUTER_BOUND('',#16812,.T.);
#14131=FACE_OUTER_BOUND('',#16813,.T.);
#14132=FACE_OUTER_BOUND('',#16814,.T.);
#14133=FACE_OUTER_BOUND('',#16815,.T.);
#14134=FACE_OUTER_BOUND('',#16816,.T.);
#14135=FACE_OUTER_BOUND('',#16817,.T.);
#14136=FACE_OUTER_BOUND('',#16818,.T.);
#14137=FACE_OUTER_BOUND('',#16819,.T.);
#14138=FACE_OUTER_BOUND('',#16820,.T.);
#14139=FACE_OUTER_BOUND('',#16821,.T.);
#14140=FACE_OUTER_BOUND('',#16822,.T.);
#14141=FACE_OUTER_BOUND('',#16823,.T.);
#14142=FACE_OUTER_BOUND('',#16824,.T.);
#14143=FACE_OUTER_BOUND('',#16825,.T.);
#14144=FACE_OUTER_BOUND('',#16826,.T.);
#14145=FACE_OUTER_BOUND('',#16827,.T.);
#14146=FACE_OUTER_BOUND('',#16828,.T.);
#14147=FACE_OUTER_BOUND('',#16829,.T.);
#14148=FACE_OUTER_BOUND('',#16830,.T.);
#14149=FACE_OUTER_BOUND('',#16831,.T.);
#14150=FACE_OUTER_BOUND('',#16832,.T.);
#14151=FACE_OUTER_BOUND('',#16833,.T.);
#14152=FACE_OUTER_BOUND('',#16834,.T.);
#14153=FACE_OUTER_BOUND('',#16835,.T.);
#14154=FACE_OUTER_BOUND('',#16836,.T.);
#14155=FACE_OUTER_BOUND('',#16837,.T.);
#14156=FACE_OUTER_BOUND('',#16838,.T.);
#14157=FACE_OUTER_BOUND('',#16839,.T.);
#14158=FACE_OUTER_BOUND('',#16840,.T.);
#14159=FACE_OUTER_BOUND('',#16841,.T.);
#14160=FACE_OUTER_BOUND('',#16842,.T.);
#14161=FACE_OUTER_BOUND('',#16843,.T.);
#14162=FACE_OUTER_BOUND('',#16844,.T.);
#14163=FACE_OUTER_BOUND('',#16845,.T.);
#14164=FACE_OUTER_BOUND('',#16846,.T.);
#14165=FACE_OUTER_BOUND('',#16847,.T.);
#14166=FACE_OUTER_BOUND('',#16848,.T.);
#14167=FACE_OUTER_BOUND('',#16849,.T.);
#14168=FACE_OUTER_BOUND('',#16850,.T.);
#14169=FACE_OUTER_BOUND('',#16851,.T.);
#14170=FACE_OUTER_BOUND('',#16852,.T.);
#14171=FACE_OUTER_BOUND('',#16853,.T.);
#14172=FACE_OUTER_BOUND('',#16854,.T.);
#14173=FACE_OUTER_BOUND('',#16855,.T.);
#14174=FACE_OUTER_BOUND('',#16856,.T.);
#14175=FACE_OUTER_BOUND('',#16857,.T.);
#14176=FACE_OUTER_BOUND('',#16858,.T.);
#14177=FACE_OUTER_BOUND('',#16859,.T.);
#14178=FACE_OUTER_BOUND('',#16860,.T.);
#14179=FACE_OUTER_BOUND('',#16861,.T.);
#14180=FACE_OUTER_BOUND('',#16862,.T.);
#14181=FACE_OUTER_BOUND('',#16863,.T.);
#14182=FACE_OUTER_BOUND('',#16864,.T.);
#14183=FACE_OUTER_BOUND('',#16865,.T.);
#14184=FACE_OUTER_BOUND('',#16866,.T.);
#14185=FACE_OUTER_BOUND('',#16867,.T.);
#14186=FACE_OUTER_BOUND('',#16868,.T.);
#14187=FACE_OUTER_BOUND('',#16869,.T.);
#14188=FACE_OUTER_BOUND('',#16870,.T.);
#14189=FACE_OUTER_BOUND('',#16871,.T.);
#14190=FACE_OUTER_BOUND('',#16872,.T.);
#14191=FACE_OUTER_BOUND('',#16873,.T.);
#14192=FACE_OUTER_BOUND('',#16874,.T.);
#14193=FACE_OUTER_BOUND('',#16875,.T.);
#14194=FACE_OUTER_BOUND('',#16876,.T.);
#14195=FACE_OUTER_BOUND('',#16877,.T.);
#14196=FACE_OUTER_BOUND('',#16878,.T.);
#14197=FACE_OUTER_BOUND('',#16879,.T.);
#14198=FACE_OUTER_BOUND('',#16880,.T.);
#14199=FACE_OUTER_BOUND('',#16881,.T.);
#14200=FACE_OUTER_BOUND('',#16882,.T.);
#14201=FACE_OUTER_BOUND('',#16883,.T.);
#14202=FACE_OUTER_BOUND('',#16884,.T.);
#14203=FACE_OUTER_BOUND('',#16885,.T.);
#14204=FACE_OUTER_BOUND('',#16886,.T.);
#14205=FACE_OUTER_BOUND('',#16887,.T.);
#14206=FACE_OUTER_BOUND('',#16888,.T.);
#14207=FACE_OUTER_BOUND('',#16889,.T.);
#14208=FACE_OUTER_BOUND('',#16890,.T.);
#14209=FACE_OUTER_BOUND('',#16891,.T.);
#14210=FACE_OUTER_BOUND('',#16892,.T.);
#14211=FACE_OUTER_BOUND('',#16893,.T.);
#14212=FACE_OUTER_BOUND('',#16894,.T.);
#14213=FACE_OUTER_BOUND('',#16895,.T.);
#14214=FACE_OUTER_BOUND('',#16896,.T.);
#14215=FACE_OUTER_BOUND('',#16897,.T.);
#14216=FACE_OUTER_BOUND('',#16898,.T.);
#14217=FACE_OUTER_BOUND('',#16899,.T.);
#14218=FACE_OUTER_BOUND('',#16900,.T.);
#14219=FACE_OUTER_BOUND('',#16901,.T.);
#14220=FACE_OUTER_BOUND('',#16902,.T.);
#14221=FACE_OUTER_BOUND('',#16903,.T.);
#14222=FACE_OUTER_BOUND('',#16904,.T.);
#14223=FACE_OUTER_BOUND('',#16905,.T.);
#14224=FACE_OUTER_BOUND('',#16906,.T.);
#14225=FACE_OUTER_BOUND('',#16907,.T.);
#14226=FACE_OUTER_BOUND('',#16908,.T.);
#14227=FACE_OUTER_BOUND('',#16909,.T.);
#14228=FACE_OUTER_BOUND('',#16910,.T.);
#14229=FACE_OUTER_BOUND('',#16911,.T.);
#14230=FACE_OUTER_BOUND('',#16912,.T.);
#14231=FACE_OUTER_BOUND('',#16913,.T.);
#14232=FACE_OUTER_BOUND('',#16914,.T.);
#14233=FACE_OUTER_BOUND('',#16915,.T.);
#14234=FACE_OUTER_BOUND('',#16916,.T.);
#14235=FACE_OUTER_BOUND('',#16917,.T.);
#14236=FACE_OUTER_BOUND('',#16918,.T.);
#14237=FACE_OUTER_BOUND('',#16919,.T.);
#14238=FACE_OUTER_BOUND('',#16920,.T.);
#14239=FACE_OUTER_BOUND('',#16921,.T.);
#14240=FACE_OUTER_BOUND('',#16922,.T.);
#14241=FACE_OUTER_BOUND('',#16923,.T.);
#14242=FACE_OUTER_BOUND('',#16924,.T.);
#14243=FACE_OUTER_BOUND('',#16925,.T.);
#14244=FACE_OUTER_BOUND('',#16926,.T.);
#14245=FACE_OUTER_BOUND('',#16927,.T.);
#14246=FACE_OUTER_BOUND('',#16928,.T.);
#14247=FACE_OUTER_BOUND('',#16929,.T.);
#14248=FACE_OUTER_BOUND('',#16930,.T.);
#14249=FACE_OUTER_BOUND('',#16931,.T.);
#14250=FACE_OUTER_BOUND('',#16932,.T.);
#14251=FACE_OUTER_BOUND('',#16933,.T.);
#14252=FACE_OUTER_BOUND('',#16934,.T.);
#14253=FACE_OUTER_BOUND('',#16935,.T.);
#14254=FACE_OUTER_BOUND('',#16936,.T.);
#14255=FACE_OUTER_BOUND('',#16937,.T.);
#14256=FACE_OUTER_BOUND('',#16938,.T.);
#14257=FACE_OUTER_BOUND('',#16939,.T.);
#14258=FACE_OUTER_BOUND('',#16940,.T.);
#14259=FACE_OUTER_BOUND('',#16941,.T.);
#14260=FACE_OUTER_BOUND('',#16942,.T.);
#14261=FACE_OUTER_BOUND('',#16943,.T.);
#14262=FACE_OUTER_BOUND('',#16944,.T.);
#14263=FACE_OUTER_BOUND('',#16945,.T.);
#14264=FACE_OUTER_BOUND('',#16946,.T.);
#14265=FACE_OUTER_BOUND('',#16947,.T.);
#14266=FACE_OUTER_BOUND('',#16948,.T.);
#14267=FACE_OUTER_BOUND('',#16949,.T.);
#14268=FACE_OUTER_BOUND('',#16950,.T.);
#14269=FACE_OUTER_BOUND('',#16951,.T.);
#14270=FACE_OUTER_BOUND('',#16952,.T.);
#14271=FACE_OUTER_BOUND('',#16953,.T.);
#14272=FACE_OUTER_BOUND('',#16954,.T.);
#14273=FACE_OUTER_BOUND('',#16955,.T.);
#14274=FACE_OUTER_BOUND('',#16956,.T.);
#14275=FACE_OUTER_BOUND('',#16957,.T.);
#14276=FACE_OUTER_BOUND('',#16958,.T.);
#14277=FACE_OUTER_BOUND('',#16959,.T.);
#14278=FACE_OUTER_BOUND('',#16960,.T.);
#14279=FACE_OUTER_BOUND('',#16961,.T.);
#14280=FACE_OUTER_BOUND('',#16962,.T.);
#14281=FACE_OUTER_BOUND('',#16963,.T.);
#14282=FACE_OUTER_BOUND('',#16964,.T.);
#14283=FACE_OUTER_BOUND('',#16965,.T.);
#14284=FACE_OUTER_BOUND('',#16966,.T.);
#14285=FACE_OUTER_BOUND('',#16967,.T.);
#14286=FACE_OUTER_BOUND('',#16968,.T.);
#14287=FACE_OUTER_BOUND('',#16969,.T.);
#14288=FACE_OUTER_BOUND('',#16970,.T.);
#14289=FACE_OUTER_BOUND('',#16971,.T.);
#14290=FACE_OUTER_BOUND('',#16972,.T.);
#14291=FACE_OUTER_BOUND('',#16973,.T.);
#14292=FACE_OUTER_BOUND('',#16974,.T.);
#14293=FACE_OUTER_BOUND('',#16975,.T.);
#14294=FACE_OUTER_BOUND('',#16976,.T.);
#14295=FACE_OUTER_BOUND('',#16977,.T.);
#14296=FACE_OUTER_BOUND('',#16978,.T.);
#14297=FACE_OUTER_BOUND('',#16979,.T.);
#14298=FACE_OUTER_BOUND('',#16980,.T.);
#14299=FACE_OUTER_BOUND('',#16981,.T.);
#14300=FACE_OUTER_BOUND('',#16982,.T.);
#14301=FACE_OUTER_BOUND('',#16983,.T.);
#14302=FACE_OUTER_BOUND('',#16984,.T.);
#14303=FACE_OUTER_BOUND('',#16985,.T.);
#14304=FACE_OUTER_BOUND('',#16986,.T.);
#14305=FACE_OUTER_BOUND('',#16987,.T.);
#14306=FACE_OUTER_BOUND('',#16988,.T.);
#14307=FACE_OUTER_BOUND('',#16989,.T.);
#14308=FACE_OUTER_BOUND('',#16990,.T.);
#14309=FACE_OUTER_BOUND('',#16991,.T.);
#14310=FACE_OUTER_BOUND('',#16992,.T.);
#14311=FACE_OUTER_BOUND('',#16993,.T.);
#14312=FACE_OUTER_BOUND('',#16994,.T.);
#14313=FACE_OUTER_BOUND('',#16995,.T.);
#14314=FACE_OUTER_BOUND('',#16996,.T.);
#14315=FACE_OUTER_BOUND('',#16997,.T.);
#14316=FACE_OUTER_BOUND('',#16998,.T.);
#14317=FACE_OUTER_BOUND('',#16999,.T.);
#14318=FACE_OUTER_BOUND('',#17000,.T.);
#14319=FACE_OUTER_BOUND('',#17001,.T.);
#14320=FACE_OUTER_BOUND('',#17002,.T.);
#14321=FACE_OUTER_BOUND('',#17003,.T.);
#14322=FACE_OUTER_BOUND('',#17004,.T.);
#14323=FACE_OUTER_BOUND('',#17005,.T.);
#14324=FACE_OUTER_BOUND('',#17006,.T.);
#14325=FACE_OUTER_BOUND('',#17007,.T.);
#14326=FACE_OUTER_BOUND('',#17008,.T.);
#14327=FACE_OUTER_BOUND('',#17009,.T.);
#14328=FACE_OUTER_BOUND('',#17010,.T.);
#14329=FACE_OUTER_BOUND('',#17011,.T.);
#14330=FACE_OUTER_BOUND('',#17012,.T.);
#14331=FACE_OUTER_BOUND('',#17013,.T.);
#14332=FACE_OUTER_BOUND('',#17014,.T.);
#14333=FACE_OUTER_BOUND('',#17015,.T.);
#14334=FACE_OUTER_BOUND('',#17016,.T.);
#14335=FACE_OUTER_BOUND('',#17017,.T.);
#14336=FACE_OUTER_BOUND('',#17018,.T.);
#14337=FACE_OUTER_BOUND('',#17019,.T.);
#14338=FACE_OUTER_BOUND('',#17020,.T.);
#14339=FACE_OUTER_BOUND('',#17021,.T.);
#14340=FACE_OUTER_BOUND('',#17022,.T.);
#14341=FACE_OUTER_BOUND('',#17023,.T.);
#14342=FACE_OUTER_BOUND('',#17024,.T.);
#14343=FACE_OUTER_BOUND('',#17025,.T.);
#14344=FACE_OUTER_BOUND('',#17026,.T.);
#14345=FACE_OUTER_BOUND('',#17027,.T.);
#14346=FACE_OUTER_BOUND('',#17028,.T.);
#14347=FACE_OUTER_BOUND('',#17029,.T.);
#14348=FACE_OUTER_BOUND('',#17030,.T.);
#14349=FACE_OUTER_BOUND('',#17031,.T.);
#14350=FACE_OUTER_BOUND('',#17032,.T.);
#14351=FACE_OUTER_BOUND('',#17033,.T.);
#14352=FACE_OUTER_BOUND('',#17034,.T.);
#14353=FACE_OUTER_BOUND('',#17035,.T.);
#14354=FACE_OUTER_BOUND('',#17036,.T.);
#14355=FACE_OUTER_BOUND('',#17037,.T.);
#14356=FACE_OUTER_BOUND('',#17038,.T.);
#14357=FACE_OUTER_BOUND('',#17039,.T.);
#14358=FACE_OUTER_BOUND('',#17040,.T.);
#14359=FACE_OUTER_BOUND('',#17041,.T.);
#14360=FACE_OUTER_BOUND('',#17042,.T.);
#14361=FACE_OUTER_BOUND('',#17043,.T.);
#14362=FACE_OUTER_BOUND('',#17044,.T.);
#14363=FACE_OUTER_BOUND('',#17045,.T.);
#14364=FACE_OUTER_BOUND('',#17046,.T.);
#14365=FACE_OUTER_BOUND('',#17047,.T.);
#14366=FACE_OUTER_BOUND('',#17048,.T.);
#14367=FACE_OUTER_BOUND('',#17049,.T.);
#14368=FACE_OUTER_BOUND('',#17050,.T.);
#14369=FACE_OUTER_BOUND('',#17051,.T.);
#14370=FACE_OUTER_BOUND('',#17052,.T.);
#14371=FACE_OUTER_BOUND('',#17053,.T.);
#14372=FACE_OUTER_BOUND('',#17054,.T.);
#14373=FACE_OUTER_BOUND('',#17055,.T.);
#14374=FACE_OUTER_BOUND('',#17056,.T.);
#14375=FACE_OUTER_BOUND('',#17057,.T.);
#14376=FACE_OUTER_BOUND('',#17058,.T.);
#14377=FACE_OUTER_BOUND('',#17059,.T.);
#14378=FACE_OUTER_BOUND('',#17060,.T.);
#14379=FACE_OUTER_BOUND('',#17061,.T.);
#14380=FACE_OUTER_BOUND('',#17062,.T.);
#14381=FACE_OUTER_BOUND('',#17063,.T.);
#14382=FACE_OUTER_BOUND('',#17064,.T.);
#14383=FACE_OUTER_BOUND('',#17065,.T.);
#14384=FACE_OUTER_BOUND('',#17066,.T.);
#14385=FACE_OUTER_BOUND('',#17067,.T.);
#14386=FACE_OUTER_BOUND('',#17068,.T.);
#14387=FACE_OUTER_BOUND('',#17069,.T.);
#14388=FACE_OUTER_BOUND('',#17070,.T.);
#14389=FACE_OUTER_BOUND('',#17071,.T.);
#14390=FACE_OUTER_BOUND('',#17072,.T.);
#14391=FACE_OUTER_BOUND('',#17073,.T.);
#14392=FACE_OUTER_BOUND('',#17074,.T.);
#14393=FACE_OUTER_BOUND('',#17075,.T.);
#14394=FACE_OUTER_BOUND('',#17076,.T.);
#14395=FACE_OUTER_BOUND('',#17077,.T.);
#14396=FACE_OUTER_BOUND('',#17078,.T.);
#14397=FACE_OUTER_BOUND('',#17079,.T.);
#14398=FACE_OUTER_BOUND('',#17080,.T.);
#14399=FACE_OUTER_BOUND('',#17081,.T.);
#14400=FACE_OUTER_BOUND('',#17082,.T.);
#14401=FACE_OUTER_BOUND('',#17083,.T.);
#14402=FACE_OUTER_BOUND('',#17084,.T.);
#14403=FACE_OUTER_BOUND('',#17085,.T.);
#14404=FACE_OUTER_BOUND('',#17086,.T.);
#14405=FACE_OUTER_BOUND('',#17087,.T.);
#14406=FACE_OUTER_BOUND('',#17088,.T.);
#14407=FACE_OUTER_BOUND('',#17089,.T.);
#14408=FACE_OUTER_BOUND('',#17090,.T.);
#14409=FACE_OUTER_BOUND('',#17091,.T.);
#14410=FACE_OUTER_BOUND('',#17092,.T.);
#14411=FACE_OUTER_BOUND('',#17093,.T.);
#14412=FACE_OUTER_BOUND('',#17094,.T.);
#14413=FACE_OUTER_BOUND('',#17095,.T.);
#14414=FACE_OUTER_BOUND('',#17096,.T.);
#14415=FACE_OUTER_BOUND('',#17097,.T.);
#14416=FACE_OUTER_BOUND('',#17098,.T.);
#14417=FACE_OUTER_BOUND('',#17099,.T.);
#14418=FACE_OUTER_BOUND('',#17100,.T.);
#14419=FACE_OUTER_BOUND('',#17101,.T.);
#14420=FACE_OUTER_BOUND('',#17102,.T.);
#14421=FACE_OUTER_BOUND('',#17103,.T.);
#14422=FACE_OUTER_BOUND('',#17104,.T.);
#14423=FACE_OUTER_BOUND('',#17105,.T.);
#14424=FACE_OUTER_BOUND('',#17106,.T.);
#14425=FACE_OUTER_BOUND('',#17107,.T.);
#14426=FACE_OUTER_BOUND('',#17108,.T.);
#14427=FACE_OUTER_BOUND('',#17109,.T.);
#14428=FACE_OUTER_BOUND('',#17110,.T.);
#14429=FACE_OUTER_BOUND('',#17111,.T.);
#14430=FACE_OUTER_BOUND('',#17112,.T.);
#14431=FACE_OUTER_BOUND('',#17113,.T.);
#14432=FACE_OUTER_BOUND('',#17114,.T.);
#14433=FACE_OUTER_BOUND('',#17115,.T.);
#14434=FACE_OUTER_BOUND('',#17116,.T.);
#14435=FACE_OUTER_BOUND('',#17117,.T.);
#14436=FACE_OUTER_BOUND('',#17118,.T.);
#14437=FACE_OUTER_BOUND('',#17119,.T.);
#14438=FACE_OUTER_BOUND('',#17120,.T.);
#14439=FACE_OUTER_BOUND('',#17121,.T.);
#14440=FACE_OUTER_BOUND('',#17122,.T.);
#14441=FACE_OUTER_BOUND('',#17123,.T.);
#14442=FACE_OUTER_BOUND('',#17124,.T.);
#14443=FACE_OUTER_BOUND('',#17125,.T.);
#14444=FACE_OUTER_BOUND('',#17126,.T.);
#14445=FACE_OUTER_BOUND('',#17127,.T.);
#14446=FACE_OUTER_BOUND('',#17128,.T.);
#14447=FACE_OUTER_BOUND('',#17129,.T.);
#14448=FACE_OUTER_BOUND('',#17130,.T.);
#14449=FACE_OUTER_BOUND('',#17131,.T.);
#14450=FACE_OUTER_BOUND('',#17132,.T.);
#14451=FACE_OUTER_BOUND('',#17133,.T.);
#14452=FACE_OUTER_BOUND('',#17134,.T.);
#14453=FACE_OUTER_BOUND('',#17135,.T.);
#14454=FACE_OUTER_BOUND('',#17136,.T.);
#14455=FACE_OUTER_BOUND('',#17137,.T.);
#14456=FACE_OUTER_BOUND('',#17138,.T.);
#14457=FACE_OUTER_BOUND('',#17139,.T.);
#14458=FACE_OUTER_BOUND('',#17140,.T.);
#14459=FACE_OUTER_BOUND('',#17141,.T.);
#14460=FACE_OUTER_BOUND('',#17142,.T.);
#14461=FACE_OUTER_BOUND('',#17143,.T.);
#14462=FACE_OUTER_BOUND('',#17144,.T.);
#14463=FACE_OUTER_BOUND('',#17145,.T.);
#14464=FACE_OUTER_BOUND('',#17146,.T.);
#14465=FACE_OUTER_BOUND('',#17147,.T.);
#14466=FACE_OUTER_BOUND('',#17148,.T.);
#14467=FACE_OUTER_BOUND('',#17149,.T.);
#14468=FACE_OUTER_BOUND('',#17150,.T.);
#14469=FACE_OUTER_BOUND('',#17151,.T.);
#14470=FACE_OUTER_BOUND('',#17152,.T.);
#14471=FACE_OUTER_BOUND('',#17153,.T.);
#14472=FACE_OUTER_BOUND('',#17154,.T.);
#14473=FACE_OUTER_BOUND('',#17155,.T.);
#14474=FACE_OUTER_BOUND('',#17156,.T.);
#14475=FACE_OUTER_BOUND('',#17157,.T.);
#14476=FACE_OUTER_BOUND('',#17158,.T.);
#14477=FACE_OUTER_BOUND('',#17159,.T.);
#14478=FACE_OUTER_BOUND('',#17160,.T.);
#14479=FACE_OUTER_BOUND('',#17161,.T.);
#14480=FACE_OUTER_BOUND('',#17162,.T.);
#14481=FACE_OUTER_BOUND('',#17163,.T.);
#14482=FACE_OUTER_BOUND('',#17164,.T.);
#14483=FACE_OUTER_BOUND('',#17165,.T.);
#14484=FACE_OUTER_BOUND('',#17166,.T.);
#14485=FACE_OUTER_BOUND('',#17167,.T.);
#14486=FACE_OUTER_BOUND('',#17168,.T.);
#14487=FACE_OUTER_BOUND('',#17169,.T.);
#14488=FACE_OUTER_BOUND('',#17170,.T.);
#14489=FACE_OUTER_BOUND('',#17171,.T.);
#14490=FACE_OUTER_BOUND('',#17172,.T.);
#14491=FACE_OUTER_BOUND('',#17173,.T.);
#14492=FACE_OUTER_BOUND('',#17174,.T.);
#14493=FACE_OUTER_BOUND('',#17175,.T.);
#14494=FACE_OUTER_BOUND('',#17176,.T.);
#14495=FACE_OUTER_BOUND('',#17177,.T.);
#14496=FACE_OUTER_BOUND('',#17178,.T.);
#14497=FACE_OUTER_BOUND('',#17179,.T.);
#14498=FACE_OUTER_BOUND('',#17180,.T.);
#14499=FACE_OUTER_BOUND('',#17181,.T.);
#14500=FACE_OUTER_BOUND('',#17182,.T.);
#14501=FACE_OUTER_BOUND('',#17183,.T.);
#14502=FACE_OUTER_BOUND('',#17184,.T.);
#14503=FACE_OUTER_BOUND('',#17185,.T.);
#14504=FACE_OUTER_BOUND('',#17186,.T.);
#14505=FACE_OUTER_BOUND('',#17187,.T.);
#14506=FACE_OUTER_BOUND('',#17188,.T.);
#14507=FACE_OUTER_BOUND('',#17189,.T.);
#14508=FACE_OUTER_BOUND('',#17190,.T.);
#14509=FACE_OUTER_BOUND('',#17191,.T.);
#14510=FACE_OUTER_BOUND('',#17192,.T.);
#14511=FACE_OUTER_BOUND('',#17193,.T.);
#14512=FACE_OUTER_BOUND('',#17194,.T.);
#14513=FACE_OUTER_BOUND('',#17195,.T.);
#14514=FACE_OUTER_BOUND('',#17196,.T.);
#14515=FACE_OUTER_BOUND('',#17197,.T.);
#14516=FACE_OUTER_BOUND('',#17198,.T.);
#14517=FACE_OUTER_BOUND('',#17199,.T.);
#14518=FACE_OUTER_BOUND('',#17200,.T.);
#14519=FACE_OUTER_BOUND('',#17201,.T.);
#14520=FACE_OUTER_BOUND('',#17202,.T.);
#14521=FACE_OUTER_BOUND('',#17203,.T.);
#14522=FACE_OUTER_BOUND('',#17204,.T.);
#14523=FACE_OUTER_BOUND('',#17205,.T.);
#14524=FACE_OUTER_BOUND('',#17206,.T.);
#14525=FACE_OUTER_BOUND('',#17207,.T.);
#14526=FACE_OUTER_BOUND('',#17208,.T.);
#14527=FACE_OUTER_BOUND('',#17209,.T.);
#14528=FACE_OUTER_BOUND('',#17210,.T.);
#14529=FACE_OUTER_BOUND('',#17211,.T.);
#14530=FACE_OUTER_BOUND('',#17212,.T.);
#14531=FACE_OUTER_BOUND('',#17213,.T.);
#14532=FACE_OUTER_BOUND('',#17214,.T.);
#14533=FACE_OUTER_BOUND('',#17215,.T.);
#14534=FACE_OUTER_BOUND('',#17216,.T.);
#14535=FACE_OUTER_BOUND('',#17217,.T.);
#14536=FACE_OUTER_BOUND('',#17218,.T.);
#14537=FACE_OUTER_BOUND('',#17219,.T.);
#14538=FACE_OUTER_BOUND('',#17220,.T.);
#14539=FACE_OUTER_BOUND('',#17221,.T.);
#14540=FACE_OUTER_BOUND('',#17222,.T.);
#14541=FACE_OUTER_BOUND('',#17223,.T.);
#14542=FACE_OUTER_BOUND('',#17224,.T.);
#14543=FACE_OUTER_BOUND('',#17225,.T.);
#14544=FACE_OUTER_BOUND('',#17226,.T.);
#14545=FACE_OUTER_BOUND('',#17227,.T.);
#14546=FACE_OUTER_BOUND('',#17228,.T.);
#14547=FACE_OUTER_BOUND('',#17229,.T.);
#14548=FACE_OUTER_BOUND('',#17230,.T.);
#14549=FACE_OUTER_BOUND('',#17231,.T.);
#14550=FACE_OUTER_BOUND('',#17232,.T.);
#14551=FACE_OUTER_BOUND('',#17233,.T.);
#14552=FACE_OUTER_BOUND('',#17234,.T.);
#14553=FACE_OUTER_BOUND('',#17235,.T.);
#14554=FACE_OUTER_BOUND('',#17236,.T.);
#14555=FACE_OUTER_BOUND('',#17237,.T.);
#14556=FACE_OUTER_BOUND('',#17238,.T.);
#14557=FACE_OUTER_BOUND('',#17239,.T.);
#14558=FACE_OUTER_BOUND('',#17240,.T.);
#14559=FACE_OUTER_BOUND('',#17241,.T.);
#14560=FACE_OUTER_BOUND('',#17242,.T.);
#14561=FACE_OUTER_BOUND('',#17243,.T.);
#14562=FACE_OUTER_BOUND('',#17244,.T.);
#14563=FACE_OUTER_BOUND('',#17245,.T.);
#14564=FACE_OUTER_BOUND('',#17246,.T.);
#14565=FACE_OUTER_BOUND('',#17247,.T.);
#14566=FACE_OUTER_BOUND('',#17248,.T.);
#14567=FACE_OUTER_BOUND('',#17249,.T.);
#14568=FACE_OUTER_BOUND('',#17250,.T.);
#14569=FACE_OUTER_BOUND('',#17251,.T.);
#14570=FACE_OUTER_BOUND('',#17252,.T.);
#14571=FACE_OUTER_BOUND('',#17253,.T.);
#14572=FACE_OUTER_BOUND('',#17254,.T.);
#14573=FACE_OUTER_BOUND('',#17255,.T.);
#14574=FACE_OUTER_BOUND('',#17256,.T.);
#14575=FACE_OUTER_BOUND('',#17257,.T.);
#14576=FACE_OUTER_BOUND('',#17258,.T.);
#14577=FACE_OUTER_BOUND('',#17259,.T.);
#14578=FACE_OUTER_BOUND('',#17260,.T.);
#14579=FACE_OUTER_BOUND('',#17261,.T.);
#14580=FACE_OUTER_BOUND('',#17262,.T.);
#14581=FACE_OUTER_BOUND('',#17263,.T.);
#14582=FACE_OUTER_BOUND('',#17264,.T.);
#14583=FACE_OUTER_BOUND('',#17265,.T.);
#14584=FACE_OUTER_BOUND('',#17266,.T.);
#14585=FACE_OUTER_BOUND('',#17267,.T.);
#14586=FACE_OUTER_BOUND('',#17268,.T.);
#14587=FACE_OUTER_BOUND('',#17269,.T.);
#14588=FACE_OUTER_BOUND('',#17270,.T.);
#14589=FACE_OUTER_BOUND('',#17271,.T.);
#14590=FACE_OUTER_BOUND('',#17272,.T.);
#14591=FACE_OUTER_BOUND('',#17273,.T.);
#14592=FACE_OUTER_BOUND('',#17274,.T.);
#14593=FACE_OUTER_BOUND('',#17275,.T.);
#14594=FACE_OUTER_BOUND('',#17276,.T.);
#14595=FACE_OUTER_BOUND('',#17277,.T.);
#14596=FACE_OUTER_BOUND('',#17278,.T.);
#14597=FACE_OUTER_BOUND('',#17279,.T.);
#14598=FACE_OUTER_BOUND('',#17280,.T.);
#14599=FACE_OUTER_BOUND('',#17281,.T.);
#14600=FACE_OUTER_BOUND('',#17282,.T.);
#14601=FACE_OUTER_BOUND('',#17283,.T.);
#14602=FACE_OUTER_BOUND('',#17284,.T.);
#14603=FACE_OUTER_BOUND('',#17285,.T.);
#14604=FACE_OUTER_BOUND('',#17286,.T.);
#14605=FACE_OUTER_BOUND('',#17287,.T.);
#14606=FACE_OUTER_BOUND('',#17288,.T.);
#14607=FACE_OUTER_BOUND('',#17289,.T.);
#14608=FACE_OUTER_BOUND('',#17290,.T.);
#14609=FACE_OUTER_BOUND('',#17291,.T.);
#14610=FACE_OUTER_BOUND('',#17292,.T.);
#14611=FACE_OUTER_BOUND('',#17293,.T.);
#14612=FACE_OUTER_BOUND('',#17294,.T.);
#14613=FACE_OUTER_BOUND('',#17295,.T.);
#14614=FACE_OUTER_BOUND('',#17296,.T.);
#14615=FACE_OUTER_BOUND('',#17297,.T.);
#14616=FACE_OUTER_BOUND('',#17298,.T.);
#14617=FACE_OUTER_BOUND('',#17299,.T.);
#14618=FACE_OUTER_BOUND('',#17300,.T.);
#14619=FACE_OUTER_BOUND('',#17301,.T.);
#14620=FACE_OUTER_BOUND('',#17302,.T.);
#14621=FACE_OUTER_BOUND('',#17304,.T.);
#14622=FACE_OUTER_BOUND('',#17305,.T.);
#14623=FACE_OUTER_BOUND('',#17306,.T.);
#14624=FACE_OUTER_BOUND('',#17307,.T.);
#14625=FACE_OUTER_BOUND('',#17308,.T.);
#14626=FACE_OUTER_BOUND('',#17310,.T.);
#14627=FACE_OUTER_BOUND('',#17311,.T.);
#14628=FACE_OUTER_BOUND('',#17313,.T.);
#14629=FACE_OUTER_BOUND('',#17314,.T.);
#14630=FACE_OUTER_BOUND('',#17316,.T.);
#14631=FACE_OUTER_BOUND('',#17317,.T.);
#14632=FACE_OUTER_BOUND('',#17318,.T.);
#14633=FACE_OUTER_BOUND('',#17319,.T.);
#14634=FACE_OUTER_BOUND('',#17320,.T.);
#15931=EDGE_LOOP('',(#32919,#32920,#32921,#32922));
#15932=EDGE_LOOP('',(#32923,#32924,#32925,#32926));
#15933=EDGE_LOOP('',(#32927,#32928,#32929,#32930));
#15934=EDGE_LOOP('',(#32931,#32932,#32933,#32934));
#15935=EDGE_LOOP('',(#32935,#32936,#32937,#32938));
#15936=EDGE_LOOP('',(#32939,#32940,#32941,#32942));
#15937=EDGE_LOOP('',(#32943,#32944,#32945,#32946));
#15938=EDGE_LOOP('',(#32947,#32948,#32949,#32950));
#15939=EDGE_LOOP('',(#32951,#32952,#32953,#32954));
#15940=EDGE_LOOP('',(#32955,#32956,#32957,#32958));
#15941=EDGE_LOOP('',(#32959,#32960,#32961,#32962));
#15942=EDGE_LOOP('',(#32963,#32964,#32965,#32966));
#15943=EDGE_LOOP('',(#32967,#32968,#32969,#32970));
#15944=EDGE_LOOP('',(#32971,#32972,#32973,#32974));
#15945=EDGE_LOOP('',(#32975,#32976,#32977,#32978));
#15946=EDGE_LOOP('',(#32979,#32980,#32981,#32982));
#15947=EDGE_LOOP('',(#32983,#32984,#32985,#32986));
#15948=EDGE_LOOP('',(#32987,#32988,#32989,#32990));
#15949=EDGE_LOOP('',(#32991,#32992,#32993,#32994));
#15950=EDGE_LOOP('',(#32995,#32996,#32997,#32998));
#15951=EDGE_LOOP('',(#32999,#33000,#33001,#33002));
#15952=EDGE_LOOP('',(#33003,#33004,#33005,#33006));
#15953=EDGE_LOOP('',(#33007,#33008,#33009,#33010));
#15954=EDGE_LOOP('',(#33011,#33012,#33013,#33014));
#15955=EDGE_LOOP('',(#33015,#33016,#33017,#33018));
#15956=EDGE_LOOP('',(#33019,#33020,#33021,#33022));
#15957=EDGE_LOOP('',(#33023,#33024,#33025,#33026));
#15958=EDGE_LOOP('',(#33027,#33028,#33029,#33030));
#15959=EDGE_LOOP('',(#33031,#33032,#33033,#33034));
#15960=EDGE_LOOP('',(#33035,#33036,#33037,#33038));
#15961=EDGE_LOOP('',(#33039,#33040,#33041,#33042));
#15962=EDGE_LOOP('',(#33043,#33044,#33045,#33046));
#15963=EDGE_LOOP('',(#33047,#33048,#33049,#33050));
#15964=EDGE_LOOP('',(#33051,#33052,#33053,#33054));
#15965=EDGE_LOOP('',(#33055,#33056,#33057,#33058));
#15966=EDGE_LOOP('',(#33059,#33060,#33061,#33062));
#15967=EDGE_LOOP('',(#33063,#33064,#33065,#33066,#33067,#33068,#33069,#33070,
#33071,#33072,#33073,#33074,#33075,#33076,#33077,#33078,#33079,#33080,#33081,
#33082,#33083,#33084,#33085,#33086,#33087,#33088,#33089,#33090,#33091,#33092,
#33093,#33094));
#15968=EDGE_LOOP('',(#33095,#33096,#33097,#33098,#33099,#33100,#33101));
#15969=EDGE_LOOP('',(#33102,#33103,#33104,#33105,#33106,#33107,#33108,#33109,
#33110,#33111,#33112,#33113,#33114,#33115,#33116,#33117,#33118,#33119,#33120,
#33121,#33122,#33123,#33124,#33125,#33126,#33127,#33128,#33129,#33130,#33131,
#33132,#33133));
#15970=EDGE_LOOP('',(#33134,#33135,#33136,#33137,#33138,#33139,#33140));
#15971=EDGE_LOOP('',(#33141,#33142,#33143,#33144,#33145,#33146,#33147,#33148,
#33149,#33150,#33151,#33152,#33153,#33154,#33155,#33156,#33157,#33158,#33159,
#33160,#33161,#33162,#33163,#33164,#33165,#33166,#33167,#33168,#33169,#33170,
#33171,#33172));
#15972=EDGE_LOOP('',(#33173,#33174,#33175,#33176,#33177,#33178,#33179));
#15973=EDGE_LOOP('',(#33180,#33181,#33182,#33183,#33184,#33185,#33186,#33187,
#33188,#33189,#33190,#33191,#33192,#33193,#33194,#33195,#33196,#33197,#33198,
#33199,#33200,#33201,#33202,#33203,#33204,#33205,#33206,#33207,#33208,#33209,
#33210,#33211));
#15974=EDGE_LOOP('',(#33212,#33213,#33214,#33215,#33216,#33217,#33218));
#15975=EDGE_LOOP('',(#33219,#33220,#33221,#33222,#33223,#33224,#33225,#33226,
#33227,#33228,#33229,#33230,#33231,#33232,#33233,#33234,#33235,#33236,#33237,
#33238,#33239,#33240,#33241,#33242,#33243,#33244,#33245,#33246,#33247,#33248,
#33249,#33250));
#15976=EDGE_LOOP('',(#33251,#33252,#33253,#33254,#33255,#33256,#33257));
#15977=EDGE_LOOP('',(#33258,#33259,#33260,#33261,#33262,#33263,#33264,#33265,
#33266,#33267,#33268,#33269,#33270,#33271,#33272,#33273,#33274,#33275,#33276,
#33277,#33278,#33279,#33280,#33281,#33282,#33283,#33284,#33285,#33286,#33287,
#33288,#33289));
#15978=EDGE_LOOP('',(#33290,#33291,#33292,#33293,#33294,#33295,#33296));
#15979=EDGE_LOOP('',(#33297,#33298,#33299,#33300,#33301,#33302,#33303,#33304,
#33305,#33306,#33307,#33308,#33309,#33310,#33311,#33312,#33313,#33314,#33315,
#33316,#33317,#33318,#33319,#33320,#33321,#33322,#33323,#33324,#33325,#33326,
#33327,#33328));
#15980=EDGE_LOOP('',(#33329,#33330,#33331,#33332,#33333,#33334,#33335));
#15981=EDGE_LOOP('',(#33336,#33337,#33338,#33339,#33340,#33341,#33342,#33343,
#33344,#33345,#33346,#33347,#33348,#33349,#33350,#33351,#33352,#33353,#33354,
#33355,#33356,#33357,#33358,#33359,#33360,#33361,#33362,#33363,#33364,#33365,
#33366,#33367));
#15982=EDGE_LOOP('',(#33368,#33369,#33370,#33371,#33372,#33373,#33374));
#15983=EDGE_LOOP('',(#33375,#33376,#33377,#33378,#33379,#33380,#33381,#33382,
#33383,#33384,#33385,#33386,#33387,#33388,#33389,#33390,#33391,#33392,#33393,
#33394,#33395,#33396,#33397,#33398,#33399,#33400,#33401,#33402,#33403,#33404,
#33405,#33406));
#15984=EDGE_LOOP('',(#33407,#33408,#33409,#33410,#33411,#33412,#33413));
#15985=EDGE_LOOP('',(#33414,#33415,#33416,#33417,#33418,#33419,#33420,#33421,
#33422,#33423,#33424,#33425,#33426,#33427,#33428,#33429,#33430,#33431,#33432,
#33433,#33434,#33435,#33436,#33437,#33438,#33439,#33440,#33441,#33442,#33443,
#33444,#33445));
#15986=EDGE_LOOP('',(#33446,#33447,#33448,#33449,#33450,#33451,#33452));
#15987=EDGE_LOOP('',(#33453,#33454,#33455,#33456,#33457,#33458,#33459,#33460,
#33461,#33462,#33463,#33464,#33465,#33466,#33467,#33468,#33469,#33470,#33471,
#33472,#33473,#33474,#33475,#33476,#33477,#33478,#33479,#33480,#33481,#33482,
#33483,#33484));
#15988=EDGE_LOOP('',(#33485,#33486,#33487,#33488,#33489,#33490,#33491));
#15989=EDGE_LOOP('',(#33492,#33493,#33494,#33495,#33496,#33497,#33498,#33499,
#33500,#33501,#33502,#33503,#33504,#33505,#33506,#33507,#33508,#33509,#33510,
#33511,#33512,#33513,#33514,#33515,#33516,#33517,#33518,#33519,#33520,#33521,
#33522,#33523));
#15990=EDGE_LOOP('',(#33524,#33525,#33526,#33527,#33528,#33529,#33530));
#15991=EDGE_LOOP('',(#33531,#33532,#33533,#33534,#33535,#33536,#33537,#33538,
#33539,#33540,#33541,#33542,#33543,#33544,#33545,#33546,#33547,#33548,#33549,
#33550,#33551,#33552,#33553,#33554,#33555,#33556,#33557,#33558,#33559,#33560,
#33561,#33562));
#15992=EDGE_LOOP('',(#33563,#33564,#33565,#33566,#33567,#33568,#33569));
#15993=EDGE_LOOP('',(#33570,#33571,#33572,#33573,#33574,#33575,#33576,#33577,
#33578,#33579,#33580,#33581,#33582,#33583,#33584,#33585,#33586,#33587,#33588,
#33589,#33590,#33591,#33592,#33593,#33594,#33595,#33596,#33597,#33598,#33599,
#33600,#33601));
#15994=EDGE_LOOP('',(#33602,#33603,#33604,#33605,#33606,#33607,#33608));
#15995=EDGE_LOOP('',(#33609,#33610,#33611,#33612,#33613,#33614,#33615,#33616,
#33617,#33618,#33619,#33620,#33621,#33622,#33623,#33624,#33625,#33626,#33627,
#33628,#33629,#33630,#33631,#33632,#33633,#33634,#33635,#33636,#33637,#33638,
#33639,#33640));
#15996=EDGE_LOOP('',(#33641,#33642,#33643,#33644,#33645,#33646,#33647));
#15997=EDGE_LOOP('',(#33648,#33649,#33650,#33651,#33652,#33653,#33654,#33655,
#33656,#33657,#33658,#33659,#33660,#33661,#33662,#33663,#33664,#33665,#33666,
#33667,#33668,#33669,#33670,#33671,#33672,#33673,#33674,#33675,#33676,#33677,
#33678,#33679));
#15998=EDGE_LOOP('',(#33680,#33681,#33682,#33683,#33684,#33685,#33686));
#15999=EDGE_LOOP('',(#33687,#33688,#33689,#33690,#33691,#33692,#33693,#33694,
#33695,#33696,#33697,#33698,#33699,#33700,#33701,#33702,#33703,#33704,#33705,
#33706,#33707,#33708,#33709,#33710,#33711,#33712,#33713,#33714,#33715,#33716,
#33717,#33718));
#16000=EDGE_LOOP('',(#33719,#33720,#33721,#33722,#33723,#33724,#33725));
#16001=EDGE_LOOP('',(#33726,#33727,#33728,#33729,#33730,#33731,#33732,#33733,
#33734,#33735,#33736,#33737,#33738,#33739,#33740,#33741,#33742,#33743,#33744,
#33745,#33746,#33747,#33748,#33749,#33750,#33751,#33752,#33753,#33754,#33755,
#33756,#33757));
#16002=EDGE_LOOP('',(#33758,#33759,#33760,#33761,#33762,#33763,#33764));
#16003=EDGE_LOOP('',(#33765,#33766,#33767,#33768,#33769,#33770,#33771,#33772,
#33773,#33774,#33775,#33776,#33777,#33778,#33779,#33780,#33781,#33782,#33783,
#33784,#33785,#33786,#33787,#33788,#33789,#33790,#33791,#33792,#33793,#33794,
#33795,#33796));
#16004=EDGE_LOOP('',(#33797,#33798,#33799,#33800,#33801,#33802,#33803));
#16005=EDGE_LOOP('',(#33804,#33805,#33806,#33807,#33808,#33809,#33810,#33811,
#33812,#33813,#33814,#33815,#33816,#33817,#33818,#33819,#33820,#33821,#33822,
#33823,#33824,#33825,#33826,#33827,#33828,#33829,#33830,#33831,#33832,#33833,
#33834,#33835));
#16006=EDGE_LOOP('',(#33836,#33837,#33838,#33839,#33840,#33841,#33842));
#16007=EDGE_LOOP('',(#33843,#33844,#33845,#33846,#33847,#33848,#33849,#33850,
#33851,#33852,#33853,#33854,#33855,#33856,#33857,#33858,#33859,#33860,#33861,
#33862,#33863,#33864,#33865,#33866,#33867,#33868,#33869,#33870,#33871,#33872,
#33873,#33874));
#16008=EDGE_LOOP('',(#33875,#33876,#33877,#33878,#33879,#33880,#33881));
#16009=EDGE_LOOP('',(#33882,#33883,#33884,#33885,#33886,#33887,#33888,#33889,
#33890,#33891,#33892,#33893,#33894,#33895,#33896,#33897,#33898,#33899,#33900,
#33901,#33902,#33903,#33904,#33905,#33906,#33907,#33908,#33909,#33910,#33911,
#33912,#33913));
#16010=EDGE_LOOP('',(#33914,#33915,#33916,#33917,#33918,#33919,#33920));
#16011=EDGE_LOOP('',(#33921,#33922,#33923,#33924,#33925,#33926,#33927,#33928,
#33929,#33930,#33931,#33932,#33933,#33934,#33935,#33936,#33937,#33938,#33939,
#33940,#33941,#33942,#33943,#33944,#33945,#33946,#33947,#33948,#33949,#33950,
#33951,#33952));
#16012=EDGE_LOOP('',(#33953,#33954,#33955,#33956,#33957,#33958,#33959));
#16013=EDGE_LOOP('',(#33960,#33961,#33962,#33963,#33964,#33965,#33966,#33967,
#33968,#33969,#33970,#33971,#33972,#33973,#33974,#33975,#33976,#33977,#33978,
#33979,#33980,#33981,#33982,#33983,#33984,#33985,#33986,#33987,#33988,#33989,
#33990,#33991));
#16014=EDGE_LOOP('',(#33992,#33993,#33994,#33995,#33996,#33997,#33998));
#16015=EDGE_LOOP('',(#33999,#34000,#34001,#34002,#34003,#34004,#34005,#34006,
#34007,#34008,#34009,#34010,#34011,#34012,#34013,#34014,#34015,#34016,#34017,
#34018,#34019,#34020,#34021,#34022,#34023,#34024,#34025,#34026,#34027,#34028,
#34029,#34030));
#16016=EDGE_LOOP('',(#34031,#34032,#34033,#34034,#34035,#34036,#34037));
#16017=EDGE_LOOP('',(#34038,#34039,#34040,#34041,#34042,#34043,#34044,#34045,
#34046,#34047,#34048,#34049,#34050,#34051,#34052,#34053,#34054,#34055,#34056,
#34057,#34058,#34059,#34060,#34061,#34062,#34063,#34064,#34065,#34066,#34067,
#34068,#34069));
#16018=EDGE_LOOP('',(#34070,#34071,#34072,#34073,#34074,#34075,#34076));
#16019=EDGE_LOOP('',(#34077,#34078,#34079,#34080,#34081,#34082,#34083,#34084,
#34085,#34086,#34087,#34088,#34089,#34090,#34091,#34092,#34093,#34094,#34095,
#34096,#34097,#34098,#34099,#34100,#34101,#34102,#34103,#34104,#34105,#34106,
#34107,#34108));
#16020=EDGE_LOOP('',(#34109,#34110,#34111,#34112,#34113,#34114,#34115));
#16021=EDGE_LOOP('',(#34116,#34117,#34118,#34119,#34120,#34121,#34122,#34123,
#34124,#34125,#34126,#34127,#34128,#34129,#34130,#34131,#34132,#34133,#34134,
#34135,#34136,#34137,#34138,#34139,#34140,#34141,#34142,#34143,#34144,#34145,
#34146,#34147));
#16022=EDGE_LOOP('',(#34148,#34149,#34150,#34151,#34152,#34153,#34154));
#16023=EDGE_LOOP('',(#34155,#34156,#34157,#34158,#34159,#34160,#34161,#34162,
#34163,#34164,#34165,#34166,#34167,#34168,#34169,#34170,#34171,#34172,#34173,
#34174,#34175,#34176,#34177,#34178,#34179,#34180,#34181,#34182,#34183,#34184,
#34185,#34186));
#16024=EDGE_LOOP('',(#34187,#34188,#34189,#34190,#34191,#34192,#34193));
#16025=EDGE_LOOP('',(#34194,#34195,#34196,#34197,#34198,#34199,#34200,#34201,
#34202,#34203,#34204,#34205,#34206,#34207,#34208,#34209,#34210,#34211,#34212,
#34213,#34214,#34215,#34216,#34217,#34218,#34219,#34220,#34221,#34222,#34223,
#34224,#34225));
#16026=EDGE_LOOP('',(#34226,#34227,#34228,#34229,#34230,#34231,#34232));
#16027=EDGE_LOOP('',(#34233,#34234,#34235,#34236,#34237,#34238,#34239,#34240,
#34241,#34242,#34243,#34244,#34245,#34246,#34247,#34248,#34249,#34250,#34251,
#34252,#34253,#34254,#34255,#34256,#34257,#34258,#34259,#34260,#34261,#34262,
#34263,#34264));
#16028=EDGE_LOOP('',(#34265,#34266,#34267,#34268,#34269,#34270,#34271));
#16029=EDGE_LOOP('',(#34272,#34273,#34274,#34275,#34276,#34277,#34278,#34279,
#34280,#34281,#34282,#34283,#34284,#34285,#34286,#34287,#34288,#34289,#34290,
#34291,#34292,#34293,#34294,#34295,#34296,#34297,#34298,#34299,#34300,#34301,
#34302,#34303));
#16030=EDGE_LOOP('',(#34304,#34305,#34306,#34307,#34308,#34309,#34310));
#16031=EDGE_LOOP('',(#34311,#34312,#34313,#34314,#34315,#34316,#34317,#34318,
#34319,#34320,#34321,#34322,#34323,#34324,#34325,#34326,#34327,#34328,#34329,
#34330,#34331,#34332,#34333,#34334,#34335,#34336,#34337,#34338,#34339,#34340,
#34341,#34342));
#16032=EDGE_LOOP('',(#34343,#34344,#34345,#34346,#34347,#34348,#34349));
#16033=EDGE_LOOP('',(#34350,#34351,#34352,#34353,#34354,#34355,#34356,#34357,
#34358,#34359,#34360,#34361,#34362,#34363,#34364,#34365,#34366,#34367,#34368,
#34369,#34370,#34371,#34372,#34373,#34374,#34375,#34376,#34377,#34378,#34379,
#34380,#34381));
#16034=EDGE_LOOP('',(#34382,#34383,#34384,#34385,#34386,#34387,#34388));
#16035=EDGE_LOOP('',(#34389,#34390,#34391,#34392,#34393,#34394,#34395,#34396,
#34397,#34398,#34399,#34400,#34401,#34402,#34403,#34404,#34405,#34406,#34407,
#34408,#34409,#34410,#34411,#34412,#34413,#34414,#34415,#34416,#34417,#34418,
#34419,#34420));
#16036=EDGE_LOOP('',(#34421,#34422,#34423,#34424,#34425,#34426,#34427));
#16037=EDGE_LOOP('',(#34428,#34429,#34430,#34431,#34432,#34433,#34434,#34435,
#34436,#34437,#34438,#34439,#34440,#34441,#34442,#34443,#34444,#34445,#34446,
#34447,#34448,#34449,#34450,#34451,#34452,#34453,#34454,#34455,#34456,#34457,
#34458,#34459));
#16038=EDGE_LOOP('',(#34460,#34461,#34462,#34463,#34464,#34465,#34466));
#16039=EDGE_LOOP('',(#34467,#34468,#34469,#34470));
#16040=EDGE_LOOP('',(#34471,#34472,#34473,#34474));
#16041=EDGE_LOOP('',(#34475,#34476,#34477,#34478));
#16042=EDGE_LOOP('',(#34479,#34480,#34481,#34482));
#16043=EDGE_LOOP('',(#34483,#34484,#34485,#34486));
#16044=EDGE_LOOP('',(#34487,#34488,#34489,#34490));
#16045=EDGE_LOOP('',(#34491,#34492,#34493,#34494));
#16046=EDGE_LOOP('',(#34495,#34496,#34497,#34498));
#16047=EDGE_LOOP('',(#34499,#34500,#34501,#34502));
#16048=EDGE_LOOP('',(#34503,#34504,#34505,#34506));
#16049=EDGE_LOOP('',(#34507,#34508,#34509,#34510));
#16050=EDGE_LOOP('',(#34511,#34512,#34513,#34514));
#16051=EDGE_LOOP('',(#34515,#34516,#34517,#34518));
#16052=EDGE_LOOP('',(#34519,#34520,#34521,#34522));
#16053=EDGE_LOOP('',(#34523,#34524,#34525,#34526));
#16054=EDGE_LOOP('',(#34527,#34528,#34529,#34530));
#16055=EDGE_LOOP('',(#34531,#34532,#34533,#34534));
#16056=EDGE_LOOP('',(#34535,#34536,#34537,#34538));
#16057=EDGE_LOOP('',(#34539,#34540,#34541,#34542));
#16058=EDGE_LOOP('',(#34543,#34544,#34545,#34546));
#16059=EDGE_LOOP('',(#34547,#34548,#34549,#34550));
#16060=EDGE_LOOP('',(#34551,#34552,#34553,#34554));
#16061=EDGE_LOOP('',(#34555,#34556,#34557,#34558));
#16062=EDGE_LOOP('',(#34559,#34560,#34561,#34562));
#16063=EDGE_LOOP('',(#34563,#34564,#34565,#34566));
#16064=EDGE_LOOP('',(#34567,#34568,#34569,#34570));
#16065=EDGE_LOOP('',(#34571,#34572,#34573,#34574));
#16066=EDGE_LOOP('',(#34575,#34576,#34577,#34578));
#16067=EDGE_LOOP('',(#34579,#34580,#34581,#34582));
#16068=EDGE_LOOP('',(#34583,#34584,#34585,#34586));
#16069=EDGE_LOOP('',(#34587,#34588,#34589,#34590));
#16070=EDGE_LOOP('',(#34591,#34592,#34593,#34594));
#16071=EDGE_LOOP('',(#34595,#34596,#34597,#34598));
#16072=EDGE_LOOP('',(#34599,#34600,#34601,#34602));
#16073=EDGE_LOOP('',(#34603,#34604,#34605,#34606));
#16074=EDGE_LOOP('',(#34607,#34608,#34609,#34610));
#16075=EDGE_LOOP('',(#34611,#34612,#34613,#34614,#34615,#34616,#34617));
#16076=EDGE_LOOP('',(#34618,#34619,#34620,#34621,#34622,#34623,#34624));
#16077=EDGE_LOOP('',(#34625,#34626,#34627,#34628,#34629,#34630,#34631));
#16078=EDGE_LOOP('',(#34632,#34633,#34634,#34635,#34636,#34637,#34638));
#16079=EDGE_LOOP('',(#34639,#34640,#34641,#34642,#34643,#34644,#34645));
#16080=EDGE_LOOP('',(#34646,#34647,#34648,#34649,#34650,#34651,#34652));
#16081=EDGE_LOOP('',(#34653,#34654,#34655,#34656,#34657,#34658,#34659));
#16082=EDGE_LOOP('',(#34660,#34661,#34662,#34663,#34664,#34665,#34666));
#16083=EDGE_LOOP('',(#34667,#34668,#34669,#34670,#34671,#34672,#34673));
#16084=EDGE_LOOP('',(#34674,#34675,#34676,#34677,#34678,#34679,#34680));
#16085=EDGE_LOOP('',(#34681,#34682,#34683,#34684,#34685,#34686,#34687));
#16086=EDGE_LOOP('',(#34688,#34689,#34690,#34691,#34692,#34693,#34694));
#16087=EDGE_LOOP('',(#34695,#34696,#34697,#34698,#34699,#34700,#34701));
#16088=EDGE_LOOP('',(#34702,#34703,#34704,#34705,#34706,#34707,#34708));
#16089=EDGE_LOOP('',(#34709,#34710,#34711,#34712,#34713,#34714,#34715));
#16090=EDGE_LOOP('',(#34716,#34717,#34718,#34719,#34720,#34721,#34722));
#16091=EDGE_LOOP('',(#34723,#34724,#34725,#34726,#34727,#34728,#34729));
#16092=EDGE_LOOP('',(#34730,#34731,#34732,#34733,#34734,#34735,#34736));
#16093=EDGE_LOOP('',(#34737,#34738,#34739,#34740,#34741,#34742,#34743));
#16094=EDGE_LOOP('',(#34744,#34745,#34746,#34747,#34748,#34749,#34750));
#16095=EDGE_LOOP('',(#34751,#34752,#34753,#34754,#34755,#34756,#34757));
#16096=EDGE_LOOP('',(#34758,#34759,#34760,#34761,#34762,#34763,#34764));
#16097=EDGE_LOOP('',(#34765,#34766,#34767,#34768,#34769,#34770,#34771));
#16098=EDGE_LOOP('',(#34772,#34773,#34774,#34775,#34776,#34777,#34778));
#16099=EDGE_LOOP('',(#34779,#34780,#34781,#34782,#34783,#34784,#34785));
#16100=EDGE_LOOP('',(#34786,#34787,#34788,#34789,#34790,#34791,#34792));
#16101=EDGE_LOOP('',(#34793,#34794,#34795,#34796,#34797,#34798,#34799));
#16102=EDGE_LOOP('',(#34800,#34801,#34802,#34803,#34804,#34805,#34806));
#16103=EDGE_LOOP('',(#34807,#34808,#34809,#34810,#34811,#34812,#34813));
#16104=EDGE_LOOP('',(#34814,#34815,#34816,#34817,#34818,#34819,#34820));
#16105=EDGE_LOOP('',(#34821,#34822,#34823,#34824,#34825,#34826,#34827));
#16106=EDGE_LOOP('',(#34828,#34829,#34830,#34831,#34832,#34833,#34834));
#16107=EDGE_LOOP('',(#34835,#34836,#34837,#34838,#34839,#34840,#34841));
#16108=EDGE_LOOP('',(#34842,#34843,#34844,#34845,#34846,#34847,#34848));
#16109=EDGE_LOOP('',(#34849,#34850,#34851,#34852,#34853,#34854,#34855));
#16110=EDGE_LOOP('',(#34856,#34857,#34858,#34859,#34860,#34861,#34862));
#16111=EDGE_LOOP('',(#34863,#34864,#34865,#34866));
#16112=EDGE_LOOP('',(#34867,#34868,#34869,#34870));
#16113=EDGE_LOOP('',(#34871,#34872,#34873,#34874));
#16114=EDGE_LOOP('',(#34875,#34876,#34877,#34878));
#16115=EDGE_LOOP('',(#34879,#34880,#34881,#34882));
#16116=EDGE_LOOP('',(#34883,#34884,#34885,#34886));
#16117=EDGE_LOOP('',(#34887,#34888,#34889,#34890));
#16118=EDGE_LOOP('',(#34891,#34892,#34893,#34894));
#16119=EDGE_LOOP('',(#34895,#34896,#34897,#34898));
#16120=EDGE_LOOP('',(#34899,#34900,#34901,#34902));
#16121=EDGE_LOOP('',(#34903,#34904,#34905,#34906));
#16122=EDGE_LOOP('',(#34907,#34908,#34909,#34910));
#16123=EDGE_LOOP('',(#34911,#34912,#34913,#34914));
#16124=EDGE_LOOP('',(#34915,#34916,#34917,#34918));
#16125=EDGE_LOOP('',(#34919,#34920,#34921,#34922));
#16126=EDGE_LOOP('',(#34923,#34924,#34925,#34926));
#16127=EDGE_LOOP('',(#34927,#34928,#34929,#34930));
#16128=EDGE_LOOP('',(#34931,#34932,#34933,#34934));
#16129=EDGE_LOOP('',(#34935,#34936,#34937,#34938));
#16130=EDGE_LOOP('',(#34939,#34940,#34941,#34942));
#16131=EDGE_LOOP('',(#34943,#34944,#34945,#34946));
#16132=EDGE_LOOP('',(#34947,#34948,#34949,#34950));
#16133=EDGE_LOOP('',(#34951,#34952,#34953,#34954));
#16134=EDGE_LOOP('',(#34955,#34956,#34957,#34958));
#16135=EDGE_LOOP('',(#34959,#34960,#34961,#34962));
#16136=EDGE_LOOP('',(#34963,#34964,#34965,#34966));
#16137=EDGE_LOOP('',(#34967,#34968,#34969,#34970));
#16138=EDGE_LOOP('',(#34971,#34972,#34973,#34974));
#16139=EDGE_LOOP('',(#34975,#34976,#34977,#34978));
#16140=EDGE_LOOP('',(#34979,#34980,#34981,#34982));
#16141=EDGE_LOOP('',(#34983,#34984,#34985,#34986));
#16142=EDGE_LOOP('',(#34987,#34988,#34989,#34990));
#16143=EDGE_LOOP('',(#34991,#34992,#34993,#34994));
#16144=EDGE_LOOP('',(#34995,#34996,#34997,#34998));
#16145=EDGE_LOOP('',(#34999,#35000,#35001,#35002));
#16146=EDGE_LOOP('',(#35003,#35004,#35005,#35006));
#16147=EDGE_LOOP('',(#35007,#35008,#35009,#35010,#35011,#35012,#35013));
#16148=EDGE_LOOP('',(#35014,#35015,#35016,#35017,#35018,#35019,#35020));
#16149=EDGE_LOOP('',(#35021,#35022,#35023,#35024,#35025,#35026,#35027));
#16150=EDGE_LOOP('',(#35028,#35029,#35030,#35031,#35032,#35033,#35034));
#16151=EDGE_LOOP('',(#35035,#35036,#35037,#35038,#35039,#35040,#35041));
#16152=EDGE_LOOP('',(#35042,#35043,#35044,#35045,#35046,#35047,#35048));
#16153=EDGE_LOOP('',(#35049,#35050,#35051,#35052,#35053,#35054,#35055));
#16154=EDGE_LOOP('',(#35056,#35057,#35058,#35059,#35060,#35061,#35062));
#16155=EDGE_LOOP('',(#35063,#35064,#35065,#35066,#35067,#35068,#35069));
#16156=EDGE_LOOP('',(#35070,#35071,#35072,#35073,#35074,#35075,#35076));
#16157=EDGE_LOOP('',(#35077,#35078,#35079,#35080,#35081,#35082,#35083));
#16158=EDGE_LOOP('',(#35084,#35085,#35086,#35087,#35088,#35089,#35090));
#16159=EDGE_LOOP('',(#35091,#35092,#35093,#35094,#35095,#35096,#35097));
#16160=EDGE_LOOP('',(#35098,#35099,#35100,#35101,#35102,#35103,#35104));
#16161=EDGE_LOOP('',(#35105,#35106,#35107,#35108,#35109,#35110,#35111));
#16162=EDGE_LOOP('',(#35112,#35113,#35114,#35115,#35116,#35117,#35118));
#16163=EDGE_LOOP('',(#35119,#35120,#35121,#35122,#35123,#35124,#35125));
#16164=EDGE_LOOP('',(#35126,#35127,#35128,#35129,#35130,#35131,#35132));
#16165=EDGE_LOOP('',(#35133,#35134,#35135,#35136,#35137,#35138,#35139));
#16166=EDGE_LOOP('',(#35140,#35141,#35142,#35143,#35144,#35145,#35146));
#16167=EDGE_LOOP('',(#35147,#35148,#35149,#35150,#35151,#35152,#35153));
#16168=EDGE_LOOP('',(#35154,#35155,#35156,#35157,#35158,#35159,#35160));
#16169=EDGE_LOOP('',(#35161,#35162,#35163,#35164,#35165,#35166,#35167));
#16170=EDGE_LOOP('',(#35168,#35169,#35170,#35171,#35172,#35173,#35174));
#16171=EDGE_LOOP('',(#35175,#35176,#35177,#35178,#35179,#35180,#35181));
#16172=EDGE_LOOP('',(#35182,#35183,#35184,#35185,#35186,#35187,#35188));
#16173=EDGE_LOOP('',(#35189,#35190,#35191,#35192,#35193,#35194,#35195));
#16174=EDGE_LOOP('',(#35196,#35197,#35198,#35199,#35200,#35201,#35202));
#16175=EDGE_LOOP('',(#35203,#35204,#35205,#35206,#35207,#35208,#35209));
#16176=EDGE_LOOP('',(#35210,#35211,#35212,#35213,#35214,#35215,#35216));
#16177=EDGE_LOOP('',(#35217,#35218,#35219,#35220,#35221,#35222,#35223));
#16178=EDGE_LOOP('',(#35224,#35225,#35226,#35227,#35228,#35229,#35230));
#16179=EDGE_LOOP('',(#35231,#35232,#35233,#35234,#35235,#35236,#35237));
#16180=EDGE_LOOP('',(#35238,#35239,#35240,#35241,#35242,#35243,#35244));
#16181=EDGE_LOOP('',(#35245,#35246,#35247,#35248,#35249,#35250,#35251));
#16182=EDGE_LOOP('',(#35252,#35253,#35254,#35255));
#16183=EDGE_LOOP('',(#35256,#35257,#35258,#35259));
#16184=EDGE_LOOP('',(#35260,#35261,#35262,#35263));
#16185=EDGE_LOOP('',(#35264,#35265,#35266,#35267));
#16186=EDGE_LOOP('',(#35268,#35269,#35270,#35271));
#16187=EDGE_LOOP('',(#35272,#35273,#35274,#35275));
#16188=EDGE_LOOP('',(#35276,#35277,#35278,#35279));
#16189=EDGE_LOOP('',(#35280,#35281,#35282,#35283));
#16190=EDGE_LOOP('',(#35284,#35285,#35286,#35287));
#16191=EDGE_LOOP('',(#35288,#35289,#35290,#35291));
#16192=EDGE_LOOP('',(#35292,#35293,#35294,#35295));
#16193=EDGE_LOOP('',(#35296,#35297,#35298,#35299));
#16194=EDGE_LOOP('',(#35300,#35301,#35302,#35303));
#16195=EDGE_LOOP('',(#35304,#35305,#35306,#35307));
#16196=EDGE_LOOP('',(#35308,#35309,#35310,#35311));
#16197=EDGE_LOOP('',(#35312,#35313,#35314,#35315));
#16198=EDGE_LOOP('',(#35316,#35317,#35318,#35319));
#16199=EDGE_LOOP('',(#35320,#35321,#35322,#35323));
#16200=EDGE_LOOP('',(#35324,#35325,#35326,#35327));
#16201=EDGE_LOOP('',(#35328,#35329,#35330,#35331));
#16202=EDGE_LOOP('',(#35332,#35333,#35334,#35335));
#16203=EDGE_LOOP('',(#35336,#35337,#35338,#35339));
#16204=EDGE_LOOP('',(#35340,#35341,#35342,#35343));
#16205=EDGE_LOOP('',(#35344,#35345,#35346,#35347));
#16206=EDGE_LOOP('',(#35348,#35349,#35350,#35351));
#16207=EDGE_LOOP('',(#35352,#35353,#35354,#35355));
#16208=EDGE_LOOP('',(#35356,#35357,#35358,#35359));
#16209=EDGE_LOOP('',(#35360,#35361,#35362,#35363));
#16210=EDGE_LOOP('',(#35364,#35365,#35366,#35367));
#16211=EDGE_LOOP('',(#35368,#35369,#35370,#35371));
#16212=EDGE_LOOP('',(#35372,#35373,#35374,#35375));
#16213=EDGE_LOOP('',(#35376,#35377,#35378,#35379));
#16214=EDGE_LOOP('',(#35380,#35381,#35382,#35383));
#16215=EDGE_LOOP('',(#35384,#35385,#35386,#35387));
#16216=EDGE_LOOP('',(#35388,#35389,#35390,#35391));
#16217=EDGE_LOOP('',(#35392,#35393,#35394,#35395));
#16218=EDGE_LOOP('',(#35396,#35397,#35398,#35399));
#16219=EDGE_LOOP('',(#35400,#35401,#35402,#35403));
#16220=EDGE_LOOP('',(#35404,#35405,#35406,#35407));
#16221=EDGE_LOOP('',(#35408,#35409,#35410,#35411));
#16222=EDGE_LOOP('',(#35412,#35413,#35414,#35415));
#16223=EDGE_LOOP('',(#35416,#35417,#35418,#35419));
#16224=EDGE_LOOP('',(#35420,#35421,#35422,#35423));
#16225=EDGE_LOOP('',(#35424,#35425,#35426,#35427));
#16226=EDGE_LOOP('',(#35428,#35429,#35430,#35431));
#16227=EDGE_LOOP('',(#35432,#35433,#35434,#35435));
#16228=EDGE_LOOP('',(#35436,#35437,#35438,#35439));
#16229=EDGE_LOOP('',(#35440,#35441,#35442,#35443));
#16230=EDGE_LOOP('',(#35444,#35445,#35446,#35447));
#16231=EDGE_LOOP('',(#35448,#35449,#35450,#35451));
#16232=EDGE_LOOP('',(#35452,#35453,#35454,#35455));
#16233=EDGE_LOOP('',(#35456,#35457,#35458,#35459));
#16234=EDGE_LOOP('',(#35460,#35461,#35462,#35463));
#16235=EDGE_LOOP('',(#35464,#35465,#35466,#35467));
#16236=EDGE_LOOP('',(#35468,#35469,#35470,#35471,#35472));
#16237=EDGE_LOOP('',(#35473,#35474,#35475,#35476));
#16238=EDGE_LOOP('',(#35477,#35478,#35479,#35480));
#16239=EDGE_LOOP('',(#35481,#35482,#35483,#35484));
#16240=EDGE_LOOP('',(#35485,#35486,#35487,#35488));
#16241=EDGE_LOOP('',(#35489,#35490,#35491,#35492));
#16242=EDGE_LOOP('',(#35493,#35494,#35495,#35496));
#16243=EDGE_LOOP('',(#35497,#35498,#35499,#35500));
#16244=EDGE_LOOP('',(#35501,#35502,#35503,#35504));
#16245=EDGE_LOOP('',(#35505,#35506,#35507,#35508));
#16246=EDGE_LOOP('',(#35509,#35510,#35511,#35512));
#16247=EDGE_LOOP('',(#35513,#35514,#35515,#35516));
#16248=EDGE_LOOP('',(#35517,#35518,#35519,#35520));
#16249=EDGE_LOOP('',(#35521,#35522,#35523,#35524));
#16250=EDGE_LOOP('',(#35525,#35526,#35527,#35528));
#16251=EDGE_LOOP('',(#35529,#35530,#35531,#35532));
#16252=EDGE_LOOP('',(#35533,#35534,#35535,#35536));
#16253=EDGE_LOOP('',(#35537,#35538,#35539,#35540));
#16254=EDGE_LOOP('',(#35541,#35542,#35543,#35544));
#16255=EDGE_LOOP('',(#35545,#35546,#35547,#35548));
#16256=EDGE_LOOP('',(#35549,#35550,#35551,#35552));
#16257=EDGE_LOOP('',(#35553,#35554,#35555,#35556));
#16258=EDGE_LOOP('',(#35557,#35558,#35559,#35560));
#16259=EDGE_LOOP('',(#35561,#35562,#35563,#35564));
#16260=EDGE_LOOP('',(#35565,#35566,#35567,#35568));
#16261=EDGE_LOOP('',(#35569,#35570,#35571,#35572));
#16262=EDGE_LOOP('',(#35573,#35574,#35575,#35576));
#16263=EDGE_LOOP('',(#35577,#35578,#35579,#35580));
#16264=EDGE_LOOP('',(#35581,#35582,#35583,#35584));
#16265=EDGE_LOOP('',(#35585,#35586,#35587,#35588));
#16266=EDGE_LOOP('',(#35589,#35590,#35591,#35592));
#16267=EDGE_LOOP('',(#35593,#35594,#35595,#35596));
#16268=EDGE_LOOP('',(#35597,#35598,#35599,#35600,#35601,#35602,#35603));
#16269=EDGE_LOOP('',(#35604,#35605,#35606,#35607));
#16270=EDGE_LOOP('',(#35608,#35609,#35610,#35611));
#16271=EDGE_LOOP('',(#35612,#35613,#35614,#35615));
#16272=EDGE_LOOP('',(#35616,#35617,#35618,#35619));
#16273=EDGE_LOOP('',(#35620,#35621,#35622,#35623));
#16274=EDGE_LOOP('',(#35624,#35625,#35626,#35627));
#16275=EDGE_LOOP('',(#35628,#35629,#35630,#35631));
#16276=EDGE_LOOP('',(#35632,#35633,#35634,#35635));
#16277=EDGE_LOOP('',(#35636,#35637,#35638,#35639));
#16278=EDGE_LOOP('',(#35640,#35641,#35642,#35643));
#16279=EDGE_LOOP('',(#35644,#35645,#35646,#35647));
#16280=EDGE_LOOP('',(#35648,#35649,#35650,#35651));
#16281=EDGE_LOOP('',(#35652,#35653,#35654,#35655));
#16282=EDGE_LOOP('',(#35656,#35657,#35658,#35659));
#16283=EDGE_LOOP('',(#35660,#35661,#35662,#35663,#35664,#35665,#35666,#35667,
#35668,#35669,#35670,#35671,#35672,#35673,#35674,#35675,#35676,#35677,#35678,
#35679,#35680,#35681,#35682,#35683,#35684,#35685,#35686,#35687,#35688,#35689,
#35690,#35691,#35692,#35693,#35694,#35695,#35696,#35697,#35698,#35699,#35700,
#35701,#35702,#35703,#35704,#35705,#35706,#35707,#35708,#35709,#35710,#35711,
#35712,#35713,#35714,#35715,#35716,#35717,#35718,#35719,#35720,#35721,#35722,
#35723,#35724,#35725,#35726,#35727,#35728,#35729,#35730,#35731,#35732,#35733,
#35734,#35735,#35736,#35737,#35738,#35739,#35740,#35741,#35742,#35743,#35744,
#35745,#35746,#35747,#35748,#35749,#35750,#35751,#35752,#35753,#35754,#35755,
#35756,#35757,#35758,#35759,#35760,#35761,#35762,#35763,#35764,#35765,#35766,
#35767,#35768,#35769,#35770,#35771,#35772,#35773,#35774,#35775,#35776,#35777,
#35778,#35779,#35780,#35781,#35782,#35783,#35784,#35785,#35786,#35787,#35788,
#35789,#35790,#35791,#35792,#35793,#35794,#35795,#35796,#35797,#35798,#35799,
#35800,#35801,#35802,#35803,#35804,#35805,#35806,#35807));
#16284=EDGE_LOOP('',(#35808,#35809,#35810,#35811,#35812,#35813,#35814,#35815,
#35816,#35817,#35818,#35819,#35820,#35821,#35822,#35823,#35824,#35825,#35826,
#35827,#35828,#35829,#35830,#35831,#35832,#35833,#35834,#35835,#35836,#35837,
#35838,#35839));
#16285=EDGE_LOOP('',(#35840,#35841,#35842,#35843));
#16286=EDGE_LOOP('',(#35844,#35845,#35846,#35847));
#16287=EDGE_LOOP('',(#35848,#35849,#35850,#35851));
#16288=EDGE_LOOP('',(#35852,#35853,#35854,#35855));
#16289=EDGE_LOOP('',(#35856,#35857,#35858,#35859));
#16290=EDGE_LOOP('',(#35860,#35861,#35862,#35863));
#16291=EDGE_LOOP('',(#35864,#35865,#35866,#35867));
#16292=EDGE_LOOP('',(#35868,#35869,#35870,#35871));
#16293=EDGE_LOOP('',(#35872,#35873,#35874,#35875));
#16294=EDGE_LOOP('',(#35876,#35877,#35878,#35879));
#16295=EDGE_LOOP('',(#35880,#35881,#35882,#35883));
#16296=EDGE_LOOP('',(#35884,#35885,#35886,#35887));
#16297=EDGE_LOOP('',(#35888,#35889,#35890,#35891));
#16298=EDGE_LOOP('',(#35892,#35893,#35894,#35895,#35896,#35897,#35898));
#16299=EDGE_LOOP('',(#35899,#35900,#35901,#35902));
#16300=EDGE_LOOP('',(#35903,#35904,#35905,#35906));
#16301=EDGE_LOOP('',(#35907,#35908,#35909,#35910));
#16302=EDGE_LOOP('',(#35911,#35912,#35913,#35914));
#16303=EDGE_LOOP('',(#35915,#35916,#35917,#35918));
#16304=EDGE_LOOP('',(#35919,#35920,#35921,#35922));
#16305=EDGE_LOOP('',(#35923,#35924,#35925,#35926));
#16306=EDGE_LOOP('',(#35927,#35928,#35929,#35930));
#16307=EDGE_LOOP('',(#35931,#35932,#35933,#35934));
#16308=EDGE_LOOP('',(#35935,#35936,#35937,#35938));
#16309=EDGE_LOOP('',(#35939,#35940,#35941,#35942));
#16310=EDGE_LOOP('',(#35943,#35944,#35945,#35946));
#16311=EDGE_LOOP('',(#35947,#35948,#35949,#35950));
#16312=EDGE_LOOP('',(#35951,#35952,#35953,#35954));
#16313=EDGE_LOOP('',(#35955,#35956,#35957,#35958,#35959,#35960,#35961,#35962,
#35963,#35964,#35965,#35966,#35967,#35968,#35969,#35970,#35971,#35972,#35973,
#35974,#35975,#35976,#35977,#35978,#35979,#35980,#35981,#35982,#35983,#35984,
#35985,#35986));
#16314=EDGE_LOOP('',(#35987,#35988,#35989,#35990));
#16315=EDGE_LOOP('',(#35991,#35992,#35993,#35994));
#16316=EDGE_LOOP('',(#35995,#35996,#35997,#35998));
#16317=EDGE_LOOP('',(#35999,#36000,#36001,#36002));
#16318=EDGE_LOOP('',(#36003,#36004,#36005,#36006));
#16319=EDGE_LOOP('',(#36007,#36008,#36009,#36010));
#16320=EDGE_LOOP('',(#36011,#36012,#36013,#36014));
#16321=EDGE_LOOP('',(#36015,#36016,#36017,#36018));
#16322=EDGE_LOOP('',(#36019,#36020,#36021,#36022));
#16323=EDGE_LOOP('',(#36023,#36024,#36025,#36026));
#16324=EDGE_LOOP('',(#36027,#36028,#36029,#36030));
#16325=EDGE_LOOP('',(#36031,#36032,#36033,#36034));
#16326=EDGE_LOOP('',(#36035,#36036,#36037,#36038));
#16327=EDGE_LOOP('',(#36039,#36040,#36041,#36042,#36043,#36044,#36045));
#16328=EDGE_LOOP('',(#36046,#36047,#36048,#36049));
#16329=EDGE_LOOP('',(#36050,#36051,#36052,#36053));
#16330=EDGE_LOOP('',(#36054,#36055,#36056,#36057));
#16331=EDGE_LOOP('',(#36058,#36059,#36060,#36061));
#16332=EDGE_LOOP('',(#36062,#36063,#36064,#36065));
#16333=EDGE_LOOP('',(#36066,#36067,#36068,#36069));
#16334=EDGE_LOOP('',(#36070,#36071,#36072,#36073));
#16335=EDGE_LOOP('',(#36074,#36075,#36076,#36077));
#16336=EDGE_LOOP('',(#36078,#36079,#36080,#36081));
#16337=EDGE_LOOP('',(#36082,#36083,#36084,#36085));
#16338=EDGE_LOOP('',(#36086,#36087,#36088,#36089));
#16339=EDGE_LOOP('',(#36090,#36091,#36092,#36093));
#16340=EDGE_LOOP('',(#36094,#36095,#36096,#36097));
#16341=EDGE_LOOP('',(#36098,#36099,#36100,#36101));
#16342=EDGE_LOOP('',(#36102,#36103,#36104,#36105,#36106,#36107,#36108,#36109,
#36110,#36111,#36112,#36113,#36114,#36115,#36116,#36117,#36118,#36119,#36120,
#36121,#36122,#36123,#36124,#36125,#36126,#36127,#36128,#36129,#36130,#36131,
#36132,#36133));
#16343=EDGE_LOOP('',(#36134,#36135,#36136,#36137));
#16344=EDGE_LOOP('',(#36138,#36139,#36140,#36141));
#16345=EDGE_LOOP('',(#36142,#36143,#36144,#36145));
#16346=EDGE_LOOP('',(#36146,#36147,#36148,#36149));
#16347=EDGE_LOOP('',(#36150,#36151,#36152,#36153));
#16348=EDGE_LOOP('',(#36154,#36155,#36156,#36157));
#16349=EDGE_LOOP('',(#36158,#36159,#36160,#36161));
#16350=EDGE_LOOP('',(#36162,#36163,#36164,#36165));
#16351=EDGE_LOOP('',(#36166,#36167,#36168,#36169));
#16352=EDGE_LOOP('',(#36170,#36171,#36172,#36173));
#16353=EDGE_LOOP('',(#36174,#36175,#36176,#36177));
#16354=EDGE_LOOP('',(#36178,#36179,#36180,#36181));
#16355=EDGE_LOOP('',(#36182,#36183,#36184,#36185));
#16356=EDGE_LOOP('',(#36186,#36187,#36188,#36189,#36190,#36191,#36192));
#16357=EDGE_LOOP('',(#36193,#36194,#36195,#36196));
#16358=EDGE_LOOP('',(#36197,#36198,#36199,#36200));
#16359=EDGE_LOOP('',(#36201,#36202,#36203,#36204));
#16360=EDGE_LOOP('',(#36205,#36206,#36207,#36208));
#16361=EDGE_LOOP('',(#36209,#36210,#36211,#36212));
#16362=EDGE_LOOP('',(#36213,#36214,#36215,#36216));
#16363=EDGE_LOOP('',(#36217,#36218,#36219,#36220));
#16364=EDGE_LOOP('',(#36221,#36222,#36223,#36224));
#16365=EDGE_LOOP('',(#36225,#36226,#36227,#36228));
#16366=EDGE_LOOP('',(#36229,#36230,#36231,#36232));
#16367=EDGE_LOOP('',(#36233,#36234,#36235,#36236));
#16368=EDGE_LOOP('',(#36237,#36238,#36239,#36240));
#16369=EDGE_LOOP('',(#36241,#36242,#36243,#36244));
#16370=EDGE_LOOP('',(#36245,#36246,#36247,#36248));
#16371=EDGE_LOOP('',(#36249,#36250,#36251,#36252,#36253,#36254,#36255,#36256,
#36257,#36258,#36259,#36260,#36261,#36262,#36263,#36264,#36265,#36266,#36267,
#36268,#36269,#36270,#36271,#36272,#36273,#36274,#36275,#36276,#36277,#36278,
#36279,#36280));
#16372=EDGE_LOOP('',(#36281,#36282,#36283,#36284));
#16373=EDGE_LOOP('',(#36285,#36286,#36287,#36288));
#16374=EDGE_LOOP('',(#36289,#36290,#36291,#36292));
#16375=EDGE_LOOP('',(#36293,#36294,#36295,#36296));
#16376=EDGE_LOOP('',(#36297,#36298,#36299,#36300));
#16377=EDGE_LOOP('',(#36301,#36302,#36303,#36304));
#16378=EDGE_LOOP('',(#36305,#36306,#36307,#36308));
#16379=EDGE_LOOP('',(#36309,#36310,#36311,#36312));
#16380=EDGE_LOOP('',(#36313,#36314,#36315,#36316));
#16381=EDGE_LOOP('',(#36317,#36318,#36319,#36320));
#16382=EDGE_LOOP('',(#36321,#36322,#36323,#36324));
#16383=EDGE_LOOP('',(#36325,#36326,#36327,#36328));
#16384=EDGE_LOOP('',(#36329,#36330,#36331,#36332));
#16385=EDGE_LOOP('',(#36333,#36334,#36335,#36336,#36337,#36338,#36339));
#16386=EDGE_LOOP('',(#36340,#36341,#36342,#36343));
#16387=EDGE_LOOP('',(#36344,#36345,#36346,#36347));
#16388=EDGE_LOOP('',(#36348,#36349,#36350,#36351));
#16389=EDGE_LOOP('',(#36352,#36353,#36354,#36355));
#16390=EDGE_LOOP('',(#36356,#36357,#36358,#36359));
#16391=EDGE_LOOP('',(#36360,#36361,#36362,#36363));
#16392=EDGE_LOOP('',(#36364,#36365,#36366,#36367));
#16393=EDGE_LOOP('',(#36368,#36369,#36370,#36371));
#16394=EDGE_LOOP('',(#36372,#36373,#36374,#36375));
#16395=EDGE_LOOP('',(#36376,#36377,#36378,#36379));
#16396=EDGE_LOOP('',(#36380,#36381,#36382,#36383));
#16397=EDGE_LOOP('',(#36384,#36385,#36386,#36387));
#16398=EDGE_LOOP('',(#36388,#36389,#36390,#36391));
#16399=EDGE_LOOP('',(#36392,#36393,#36394,#36395));
#16400=EDGE_LOOP('',(#36396,#36397,#36398,#36399,#36400,#36401,#36402,#36403,
#36404,#36405,#36406,#36407,#36408,#36409,#36410,#36411,#36412,#36413,#36414,
#36415,#36416,#36417,#36418,#36419,#36420,#36421,#36422,#36423,#36424,#36425,
#36426,#36427));
#16401=EDGE_LOOP('',(#36428,#36429,#36430,#36431));
#16402=EDGE_LOOP('',(#36432,#36433,#36434,#36435));
#16403=EDGE_LOOP('',(#36436,#36437,#36438,#36439));
#16404=EDGE_LOOP('',(#36440,#36441,#36442,#36443));
#16405=EDGE_LOOP('',(#36444,#36445,#36446,#36447));
#16406=EDGE_LOOP('',(#36448,#36449,#36450,#36451));
#16407=EDGE_LOOP('',(#36452,#36453,#36454,#36455));
#16408=EDGE_LOOP('',(#36456,#36457,#36458,#36459));
#16409=EDGE_LOOP('',(#36460,#36461,#36462,#36463));
#16410=EDGE_LOOP('',(#36464,#36465,#36466,#36467));
#16411=EDGE_LOOP('',(#36468,#36469,#36470,#36471));
#16412=EDGE_LOOP('',(#36472,#36473,#36474,#36475));
#16413=EDGE_LOOP('',(#36476,#36477,#36478,#36479));
#16414=EDGE_LOOP('',(#36480,#36481,#36482,#36483,#36484,#36485,#36486));
#16415=EDGE_LOOP('',(#36487,#36488,#36489,#36490));
#16416=EDGE_LOOP('',(#36491,#36492,#36493,#36494));
#16417=EDGE_LOOP('',(#36495,#36496,#36497,#36498));
#16418=EDGE_LOOP('',(#36499,#36500,#36501,#36502));
#16419=EDGE_LOOP('',(#36503,#36504,#36505,#36506));
#16420=EDGE_LOOP('',(#36507,#36508,#36509,#36510));
#16421=EDGE_LOOP('',(#36511,#36512,#36513,#36514));
#16422=EDGE_LOOP('',(#36515,#36516,#36517,#36518));
#16423=EDGE_LOOP('',(#36519,#36520,#36521,#36522));
#16424=EDGE_LOOP('',(#36523,#36524,#36525,#36526));
#16425=EDGE_LOOP('',(#36527,#36528,#36529,#36530));
#16426=EDGE_LOOP('',(#36531,#36532,#36533,#36534));
#16427=EDGE_LOOP('',(#36535,#36536,#36537,#36538));
#16428=EDGE_LOOP('',(#36539,#36540,#36541,#36542));
#16429=EDGE_LOOP('',(#36543,#36544,#36545,#36546,#36547,#36548,#36549,#36550,
#36551,#36552,#36553,#36554,#36555,#36556,#36557,#36558,#36559,#36560,#36561,
#36562,#36563,#36564,#36565,#36566,#36567,#36568,#36569,#36570,#36571,#36572,
#36573,#36574));
#16430=EDGE_LOOP('',(#36575,#36576,#36577,#36578));
#16431=EDGE_LOOP('',(#36579,#36580,#36581,#36582));
#16432=EDGE_LOOP('',(#36583,#36584,#36585,#36586));
#16433=EDGE_LOOP('',(#36587,#36588,#36589,#36590));
#16434=EDGE_LOOP('',(#36591,#36592,#36593,#36594));
#16435=EDGE_LOOP('',(#36595,#36596,#36597,#36598));
#16436=EDGE_LOOP('',(#36599,#36600,#36601,#36602));
#16437=EDGE_LOOP('',(#36603,#36604,#36605,#36606));
#16438=EDGE_LOOP('',(#36607,#36608,#36609,#36610));
#16439=EDGE_LOOP('',(#36611,#36612,#36613,#36614));
#16440=EDGE_LOOP('',(#36615,#36616,#36617,#36618));
#16441=EDGE_LOOP('',(#36619,#36620,#36621,#36622));
#16442=EDGE_LOOP('',(#36623,#36624,#36625,#36626));
#16443=EDGE_LOOP('',(#36627,#36628,#36629,#36630,#36631,#36632,#36633));
#16444=EDGE_LOOP('',(#36634,#36635,#36636,#36637));
#16445=EDGE_LOOP('',(#36638,#36639,#36640,#36641));
#16446=EDGE_LOOP('',(#36642,#36643,#36644,#36645));
#16447=EDGE_LOOP('',(#36646,#36647,#36648,#36649));
#16448=EDGE_LOOP('',(#36650,#36651,#36652,#36653));
#16449=EDGE_LOOP('',(#36654,#36655,#36656,#36657));
#16450=EDGE_LOOP('',(#36658,#36659,#36660,#36661));
#16451=EDGE_LOOP('',(#36662,#36663,#36664,#36665));
#16452=EDGE_LOOP('',(#36666,#36667,#36668,#36669));
#16453=EDGE_LOOP('',(#36670,#36671,#36672,#36673));
#16454=EDGE_LOOP('',(#36674,#36675,#36676,#36677));
#16455=EDGE_LOOP('',(#36678,#36679,#36680,#36681));
#16456=EDGE_LOOP('',(#36682,#36683,#36684,#36685));
#16457=EDGE_LOOP('',(#36686,#36687,#36688,#36689));
#16458=EDGE_LOOP('',(#36690,#36691,#36692,#36693,#36694,#36695,#36696,#36697,
#36698,#36699,#36700,#36701,#36702,#36703,#36704,#36705,#36706,#36707,#36708,
#36709,#36710,#36711,#36712,#36713,#36714,#36715,#36716,#36717,#36718,#36719,
#36720,#36721));
#16459=EDGE_LOOP('',(#36722,#36723,#36724,#36725));
#16460=EDGE_LOOP('',(#36726,#36727,#36728,#36729));
#16461=EDGE_LOOP('',(#36730,#36731,#36732,#36733));
#16462=EDGE_LOOP('',(#36734,#36735,#36736,#36737));
#16463=EDGE_LOOP('',(#36738,#36739,#36740,#36741));
#16464=EDGE_LOOP('',(#36742,#36743,#36744,#36745));
#16465=EDGE_LOOP('',(#36746,#36747,#36748,#36749));
#16466=EDGE_LOOP('',(#36750,#36751,#36752,#36753));
#16467=EDGE_LOOP('',(#36754,#36755,#36756,#36757));
#16468=EDGE_LOOP('',(#36758,#36759,#36760,#36761));
#16469=EDGE_LOOP('',(#36762,#36763,#36764,#36765));
#16470=EDGE_LOOP('',(#36766,#36767,#36768,#36769));
#16471=EDGE_LOOP('',(#36770,#36771,#36772,#36773));
#16472=EDGE_LOOP('',(#36774,#36775,#36776,#36777,#36778,#36779,#36780));
#16473=EDGE_LOOP('',(#36781,#36782,#36783,#36784));
#16474=EDGE_LOOP('',(#36785,#36786,#36787,#36788));
#16475=EDGE_LOOP('',(#36789,#36790,#36791,#36792));
#16476=EDGE_LOOP('',(#36793,#36794,#36795,#36796));
#16477=EDGE_LOOP('',(#36797,#36798,#36799,#36800));
#16478=EDGE_LOOP('',(#36801,#36802,#36803,#36804));
#16479=EDGE_LOOP('',(#36805,#36806,#36807,#36808));
#16480=EDGE_LOOP('',(#36809,#36810,#36811,#36812));
#16481=EDGE_LOOP('',(#36813,#36814,#36815,#36816));
#16482=EDGE_LOOP('',(#36817,#36818,#36819,#36820));
#16483=EDGE_LOOP('',(#36821,#36822,#36823,#36824));
#16484=EDGE_LOOP('',(#36825,#36826,#36827,#36828));
#16485=EDGE_LOOP('',(#36829,#36830,#36831,#36832));
#16486=EDGE_LOOP('',(#36833,#36834,#36835,#36836));
#16487=EDGE_LOOP('',(#36837,#36838,#36839,#36840,#36841,#36842,#36843,#36844,
#36845,#36846,#36847,#36848,#36849,#36850,#36851,#36852,#36853,#36854,#36855,
#36856,#36857,#36858,#36859,#36860,#36861,#36862,#36863,#36864,#36865,#36866,
#36867,#36868));
#16488=EDGE_LOOP('',(#36869,#36870,#36871,#36872));
#16489=EDGE_LOOP('',(#36873,#36874,#36875,#36876));
#16490=EDGE_LOOP('',(#36877,#36878,#36879,#36880));
#16491=EDGE_LOOP('',(#36881,#36882,#36883,#36884));
#16492=EDGE_LOOP('',(#36885,#36886,#36887,#36888));
#16493=EDGE_LOOP('',(#36889,#36890,#36891,#36892));
#16494=EDGE_LOOP('',(#36893,#36894,#36895,#36896));
#16495=EDGE_LOOP('',(#36897,#36898,#36899,#36900));
#16496=EDGE_LOOP('',(#36901,#36902,#36903,#36904));
#16497=EDGE_LOOP('',(#36905,#36906,#36907,#36908));
#16498=EDGE_LOOP('',(#36909,#36910,#36911,#36912));
#16499=EDGE_LOOP('',(#36913,#36914,#36915,#36916));
#16500=EDGE_LOOP('',(#36917,#36918,#36919,#36920));
#16501=EDGE_LOOP('',(#36921,#36922,#36923,#36924,#36925,#36926,#36927));
#16502=EDGE_LOOP('',(#36928,#36929,#36930,#36931));
#16503=EDGE_LOOP('',(#36932,#36933,#36934,#36935));
#16504=EDGE_LOOP('',(#36936,#36937,#36938,#36939));
#16505=EDGE_LOOP('',(#36940,#36941,#36942,#36943));
#16506=EDGE_LOOP('',(#36944,#36945,#36946,#36947));
#16507=EDGE_LOOP('',(#36948,#36949,#36950,#36951));
#16508=EDGE_LOOP('',(#36952,#36953,#36954,#36955));
#16509=EDGE_LOOP('',(#36956,#36957,#36958,#36959));
#16510=EDGE_LOOP('',(#36960,#36961,#36962,#36963));
#16511=EDGE_LOOP('',(#36964,#36965,#36966,#36967));
#16512=EDGE_LOOP('',(#36968,#36969,#36970,#36971));
#16513=EDGE_LOOP('',(#36972,#36973,#36974,#36975));
#16514=EDGE_LOOP('',(#36976,#36977,#36978,#36979));
#16515=EDGE_LOOP('',(#36980,#36981,#36982,#36983));
#16516=EDGE_LOOP('',(#36984,#36985,#36986,#36987,#36988,#36989,#36990,#36991,
#36992,#36993,#36994,#36995,#36996,#36997,#36998,#36999,#37000,#37001,#37002,
#37003,#37004,#37005,#37006,#37007,#37008,#37009,#37010,#37011,#37012,#37013,
#37014,#37015));
#16517=EDGE_LOOP('',(#37016,#37017,#37018,#37019));
#16518=EDGE_LOOP('',(#37020,#37021,#37022,#37023));
#16519=EDGE_LOOP('',(#37024,#37025,#37026,#37027));
#16520=EDGE_LOOP('',(#37028,#37029,#37030,#37031));
#16521=EDGE_LOOP('',(#37032,#37033,#37034,#37035));
#16522=EDGE_LOOP('',(#37036,#37037,#37038,#37039));
#16523=EDGE_LOOP('',(#37040,#37041,#37042,#37043));
#16524=EDGE_LOOP('',(#37044,#37045,#37046,#37047));
#16525=EDGE_LOOP('',(#37048,#37049,#37050,#37051));
#16526=EDGE_LOOP('',(#37052,#37053,#37054,#37055));
#16527=EDGE_LOOP('',(#37056,#37057,#37058,#37059));
#16528=EDGE_LOOP('',(#37060,#37061,#37062,#37063));
#16529=EDGE_LOOP('',(#37064,#37065,#37066,#37067));
#16530=EDGE_LOOP('',(#37068,#37069,#37070,#37071,#37072,#37073,#37074));
#16531=EDGE_LOOP('',(#37075,#37076,#37077,#37078));
#16532=EDGE_LOOP('',(#37079,#37080,#37081,#37082));
#16533=EDGE_LOOP('',(#37083,#37084,#37085,#37086));
#16534=EDGE_LOOP('',(#37087,#37088,#37089,#37090));
#16535=EDGE_LOOP('',(#37091,#37092,#37093,#37094));
#16536=EDGE_LOOP('',(#37095,#37096,#37097,#37098));
#16537=EDGE_LOOP('',(#37099,#37100,#37101,#37102));
#16538=EDGE_LOOP('',(#37103,#37104,#37105,#37106));
#16539=EDGE_LOOP('',(#37107,#37108,#37109,#37110));
#16540=EDGE_LOOP('',(#37111,#37112,#37113,#37114));
#16541=EDGE_LOOP('',(#37115,#37116,#37117,#37118));
#16542=EDGE_LOOP('',(#37119,#37120,#37121,#37122));
#16543=EDGE_LOOP('',(#37123,#37124,#37125,#37126));
#16544=EDGE_LOOP('',(#37127,#37128,#37129,#37130));
#16545=EDGE_LOOP('',(#37131,#37132,#37133,#37134,#37135,#37136,#37137,#37138,
#37139,#37140,#37141,#37142,#37143,#37144,#37145,#37146,#37147,#37148,#37149,
#37150,#37151,#37152,#37153,#37154,#37155,#37156,#37157,#37158,#37159,#37160,
#37161,#37162));
#16546=EDGE_LOOP('',(#37163,#37164,#37165,#37166));
#16547=EDGE_LOOP('',(#37167,#37168,#37169,#37170));
#16548=EDGE_LOOP('',(#37171,#37172,#37173,#37174));
#16549=EDGE_LOOP('',(#37175,#37176,#37177,#37178));
#16550=EDGE_LOOP('',(#37179,#37180,#37181,#37182));
#16551=EDGE_LOOP('',(#37183,#37184,#37185,#37186));
#16552=EDGE_LOOP('',(#37187,#37188,#37189,#37190));
#16553=EDGE_LOOP('',(#37191,#37192,#37193,#37194));
#16554=EDGE_LOOP('',(#37195,#37196,#37197,#37198));
#16555=EDGE_LOOP('',(#37199,#37200,#37201,#37202));
#16556=EDGE_LOOP('',(#37203,#37204,#37205,#37206));
#16557=EDGE_LOOP('',(#37207,#37208,#37209,#37210));
#16558=EDGE_LOOP('',(#37211,#37212,#37213,#37214));
#16559=EDGE_LOOP('',(#37215,#37216,#37217,#37218,#37219,#37220,#37221));
#16560=EDGE_LOOP('',(#37222,#37223,#37224,#37225));
#16561=EDGE_LOOP('',(#37226,#37227,#37228,#37229));
#16562=EDGE_LOOP('',(#37230,#37231,#37232,#37233));
#16563=EDGE_LOOP('',(#37234,#37235,#37236,#37237));
#16564=EDGE_LOOP('',(#37238,#37239,#37240,#37241));
#16565=EDGE_LOOP('',(#37242,#37243,#37244,#37245));
#16566=EDGE_LOOP('',(#37246,#37247,#37248,#37249));
#16567=EDGE_LOOP('',(#37250,#37251,#37252,#37253));
#16568=EDGE_LOOP('',(#37254,#37255,#37256,#37257));
#16569=EDGE_LOOP('',(#37258,#37259,#37260,#37261));
#16570=EDGE_LOOP('',(#37262,#37263,#37264,#37265));
#16571=EDGE_LOOP('',(#37266,#37267,#37268,#37269));
#16572=EDGE_LOOP('',(#37270,#37271,#37272,#37273));
#16573=EDGE_LOOP('',(#37274,#37275,#37276,#37277));
#16574=EDGE_LOOP('',(#37278,#37279,#37280,#37281,#37282,#37283,#37284,#37285,
#37286,#37287,#37288,#37289,#37290,#37291,#37292,#37293,#37294,#37295,#37296,
#37297,#37298,#37299,#37300,#37301,#37302,#37303,#37304,#37305,#37306,#37307,
#37308,#37309));
#16575=EDGE_LOOP('',(#37310,#37311,#37312,#37313));
#16576=EDGE_LOOP('',(#37314,#37315,#37316,#37317));
#16577=EDGE_LOOP('',(#37318,#37319,#37320,#37321));
#16578=EDGE_LOOP('',(#37322,#37323,#37324,#37325));
#16579=EDGE_LOOP('',(#37326,#37327,#37328,#37329));
#16580=EDGE_LOOP('',(#37330,#37331,#37332,#37333));
#16581=EDGE_LOOP('',(#37334,#37335,#37336,#37337));
#16582=EDGE_LOOP('',(#37338,#37339,#37340,#37341));
#16583=EDGE_LOOP('',(#37342,#37343,#37344,#37345));
#16584=EDGE_LOOP('',(#37346,#37347,#37348,#37349));
#16585=EDGE_LOOP('',(#37350,#37351,#37352,#37353));
#16586=EDGE_LOOP('',(#37354,#37355,#37356,#37357));
#16587=EDGE_LOOP('',(#37358,#37359,#37360,#37361));
#16588=EDGE_LOOP('',(#37362,#37363,#37364,#37365,#37366,#37367,#37368));
#16589=EDGE_LOOP('',(#37369,#37370,#37371,#37372));
#16590=EDGE_LOOP('',(#37373,#37374,#37375,#37376));
#16591=EDGE_LOOP('',(#37377,#37378,#37379,#37380));
#16592=EDGE_LOOP('',(#37381,#37382,#37383,#37384));
#16593=EDGE_LOOP('',(#37385,#37386,#37387,#37388));
#16594=EDGE_LOOP('',(#37389,#37390,#37391,#37392));
#16595=EDGE_LOOP('',(#37393,#37394,#37395,#37396));
#16596=EDGE_LOOP('',(#37397,#37398,#37399,#37400));
#16597=EDGE_LOOP('',(#37401,#37402,#37403,#37404));
#16598=EDGE_LOOP('',(#37405,#37406,#37407,#37408));
#16599=EDGE_LOOP('',(#37409,#37410,#37411,#37412));
#16600=EDGE_LOOP('',(#37413,#37414,#37415,#37416));
#16601=EDGE_LOOP('',(#37417,#37418,#37419,#37420));
#16602=EDGE_LOOP('',(#37421,#37422,#37423,#37424));
#16603=EDGE_LOOP('',(#37425,#37426,#37427,#37428,#37429,#37430,#37431,#37432,
#37433,#37434,#37435,#37436,#37437,#37438,#37439,#37440,#37441,#37442,#37443,
#37444,#37445,#37446,#37447,#37448,#37449,#37450,#37451,#37452,#37453,#37454,
#37455,#37456));
#16604=EDGE_LOOP('',(#37457,#37458,#37459,#37460));
#16605=EDGE_LOOP('',(#37461,#37462,#37463,#37464));
#16606=EDGE_LOOP('',(#37465,#37466,#37467,#37468));
#16607=EDGE_LOOP('',(#37469,#37470,#37471,#37472));
#16608=EDGE_LOOP('',(#37473,#37474,#37475,#37476));
#16609=EDGE_LOOP('',(#37477,#37478,#37479,#37480));
#16610=EDGE_LOOP('',(#37481,#37482,#37483,#37484));
#16611=EDGE_LOOP('',(#37485,#37486,#37487,#37488));
#16612=EDGE_LOOP('',(#37489,#37490,#37491,#37492));
#16613=EDGE_LOOP('',(#37493,#37494,#37495,#37496));
#16614=EDGE_LOOP('',(#37497,#37498,#37499,#37500));
#16615=EDGE_LOOP('',(#37501,#37502,#37503,#37504));
#16616=EDGE_LOOP('',(#37505,#37506,#37507,#37508));
#16617=EDGE_LOOP('',(#37509,#37510,#37511,#37512,#37513,#37514,#37515));
#16618=EDGE_LOOP('',(#37516,#37517,#37518,#37519));
#16619=EDGE_LOOP('',(#37520,#37521,#37522,#37523));
#16620=EDGE_LOOP('',(#37524,#37525,#37526,#37527));
#16621=EDGE_LOOP('',(#37528,#37529,#37530,#37531));
#16622=EDGE_LOOP('',(#37532,#37533,#37534,#37535));
#16623=EDGE_LOOP('',(#37536,#37537,#37538,#37539));
#16624=EDGE_LOOP('',(#37540,#37541,#37542,#37543));
#16625=EDGE_LOOP('',(#37544,#37545,#37546,#37547));
#16626=EDGE_LOOP('',(#37548,#37549,#37550,#37551));
#16627=EDGE_LOOP('',(#37552,#37553,#37554,#37555));
#16628=EDGE_LOOP('',(#37556,#37557,#37558,#37559));
#16629=EDGE_LOOP('',(#37560,#37561,#37562,#37563));
#16630=EDGE_LOOP('',(#37564,#37565,#37566,#37567));
#16631=EDGE_LOOP('',(#37568,#37569,#37570,#37571));
#16632=EDGE_LOOP('',(#37572,#37573,#37574,#37575,#37576,#37577,#37578,#37579,
#37580,#37581,#37582,#37583,#37584,#37585,#37586,#37587,#37588,#37589,#37590,
#37591,#37592,#37593,#37594,#37595,#37596,#37597,#37598,#37599,#37600,#37601,
#37602,#37603));
#16633=EDGE_LOOP('',(#37604,#37605,#37606,#37607));
#16634=EDGE_LOOP('',(#37608,#37609,#37610,#37611));
#16635=EDGE_LOOP('',(#37612,#37613,#37614,#37615));
#16636=EDGE_LOOP('',(#37616,#37617,#37618,#37619));
#16637=EDGE_LOOP('',(#37620,#37621,#37622,#37623));
#16638=EDGE_LOOP('',(#37624,#37625,#37626,#37627));
#16639=EDGE_LOOP('',(#37628,#37629,#37630,#37631));
#16640=EDGE_LOOP('',(#37632,#37633,#37634,#37635));
#16641=EDGE_LOOP('',(#37636,#37637,#37638,#37639));
#16642=EDGE_LOOP('',(#37640,#37641,#37642,#37643));
#16643=EDGE_LOOP('',(#37644,#37645,#37646,#37647));
#16644=EDGE_LOOP('',(#37648,#37649,#37650,#37651));
#16645=EDGE_LOOP('',(#37652,#37653,#37654,#37655));
#16646=EDGE_LOOP('',(#37656,#37657,#37658,#37659,#37660,#37661,#37662));
#16647=EDGE_LOOP('',(#37663,#37664,#37665,#37666));
#16648=EDGE_LOOP('',(#37667,#37668,#37669,#37670));
#16649=EDGE_LOOP('',(#37671,#37672,#37673,#37674));
#16650=EDGE_LOOP('',(#37675,#37676,#37677,#37678));
#16651=EDGE_LOOP('',(#37679,#37680,#37681,#37682));
#16652=EDGE_LOOP('',(#37683,#37684,#37685,#37686));
#16653=EDGE_LOOP('',(#37687,#37688,#37689,#37690));
#16654=EDGE_LOOP('',(#37691,#37692,#37693,#37694));
#16655=EDGE_LOOP('',(#37695,#37696,#37697,#37698));
#16656=EDGE_LOOP('',(#37699,#37700,#37701,#37702));
#16657=EDGE_LOOP('',(#37703,#37704,#37705,#37706));
#16658=EDGE_LOOP('',(#37707,#37708,#37709,#37710));
#16659=EDGE_LOOP('',(#37711,#37712,#37713,#37714));
#16660=EDGE_LOOP('',(#37715,#37716,#37717,#37718));
#16661=EDGE_LOOP('',(#37719,#37720,#37721,#37722,#37723,#37724,#37725,#37726,
#37727,#37728,#37729,#37730,#37731,#37732,#37733,#37734,#37735,#37736,#37737,
#37738,#37739,#37740,#37741,#37742,#37743,#37744,#37745,#37746,#37747,#37748,
#37749,#37750));
#16662=EDGE_LOOP('',(#37751,#37752,#37753,#37754));
#16663=EDGE_LOOP('',(#37755,#37756,#37757,#37758));
#16664=EDGE_LOOP('',(#37759,#37760,#37761,#37762));
#16665=EDGE_LOOP('',(#37763,#37764,#37765,#37766));
#16666=EDGE_LOOP('',(#37767,#37768,#37769,#37770));
#16667=EDGE_LOOP('',(#37771,#37772,#37773,#37774));
#16668=EDGE_LOOP('',(#37775,#37776,#37777,#37778));
#16669=EDGE_LOOP('',(#37779,#37780,#37781,#37782));
#16670=EDGE_LOOP('',(#37783,#37784,#37785,#37786));
#16671=EDGE_LOOP('',(#37787,#37788,#37789,#37790));
#16672=EDGE_LOOP('',(#37791,#37792,#37793,#37794));
#16673=EDGE_LOOP('',(#37795,#37796,#37797,#37798));
#16674=EDGE_LOOP('',(#37799,#37800,#37801,#37802));
#16675=EDGE_LOOP('',(#37803,#37804,#37805,#37806,#37807,#37808,#37809));
#16676=EDGE_LOOP('',(#37810,#37811,#37812,#37813));
#16677=EDGE_LOOP('',(#37814,#37815,#37816,#37817));
#16678=EDGE_LOOP('',(#37818,#37819,#37820,#37821));
#16679=EDGE_LOOP('',(#37822,#37823,#37824,#37825));
#16680=EDGE_LOOP('',(#37826,#37827,#37828,#37829));
#16681=EDGE_LOOP('',(#37830,#37831,#37832,#37833));
#16682=EDGE_LOOP('',(#37834,#37835,#37836,#37837));
#16683=EDGE_LOOP('',(#37838,#37839,#37840,#37841));
#16684=EDGE_LOOP('',(#37842,#37843,#37844,#37845));
#16685=EDGE_LOOP('',(#37846,#37847,#37848,#37849));
#16686=EDGE_LOOP('',(#37850,#37851,#37852,#37853));
#16687=EDGE_LOOP('',(#37854,#37855,#37856,#37857));
#16688=EDGE_LOOP('',(#37858,#37859,#37860,#37861));
#16689=EDGE_LOOP('',(#37862,#37863,#37864,#37865));
#16690=EDGE_LOOP('',(#37866,#37867,#37868,#37869,#37870,#37871,#37872,#37873,
#37874,#37875,#37876,#37877,#37878,#37879,#37880,#37881,#37882,#37883,#37884,
#37885,#37886,#37887,#37888,#37889,#37890,#37891,#37892,#37893,#37894,#37895,
#37896,#37897));
#16691=EDGE_LOOP('',(#37898,#37899,#37900,#37901));
#16692=EDGE_LOOP('',(#37902,#37903,#37904,#37905));
#16693=EDGE_LOOP('',(#37906,#37907,#37908,#37909));
#16694=EDGE_LOOP('',(#37910,#37911,#37912,#37913));
#16695=EDGE_LOOP('',(#37914,#37915,#37916,#37917));
#16696=EDGE_LOOP('',(#37918,#37919,#37920,#37921));
#16697=EDGE_LOOP('',(#37922,#37923,#37924,#37925));
#16698=EDGE_LOOP('',(#37926,#37927,#37928,#37929));
#16699=EDGE_LOOP('',(#37930,#37931,#37932,#37933));
#16700=EDGE_LOOP('',(#37934,#37935,#37936,#37937));
#16701=EDGE_LOOP('',(#37938,#37939,#37940,#37941));
#16702=EDGE_LOOP('',(#37942,#37943,#37944,#37945));
#16703=EDGE_LOOP('',(#37946,#37947,#37948,#37949));
#16704=EDGE_LOOP('',(#37950,#37951,#37952,#37953,#37954,#37955,#37956));
#16705=EDGE_LOOP('',(#37957,#37958,#37959,#37960));
#16706=EDGE_LOOP('',(#37961,#37962,#37963,#37964));
#16707=EDGE_LOOP('',(#37965,#37966,#37967,#37968));
#16708=EDGE_LOOP('',(#37969,#37970,#37971,#37972));
#16709=EDGE_LOOP('',(#37973,#37974,#37975,#37976));
#16710=EDGE_LOOP('',(#37977,#37978,#37979,#37980));
#16711=EDGE_LOOP('',(#37981,#37982,#37983,#37984));
#16712=EDGE_LOOP('',(#37985,#37986,#37987,#37988));
#16713=EDGE_LOOP('',(#37989,#37990,#37991,#37992));
#16714=EDGE_LOOP('',(#37993,#37994,#37995,#37996));
#16715=EDGE_LOOP('',(#37997,#37998,#37999,#38000));
#16716=EDGE_LOOP('',(#38001,#38002,#38003,#38004));
#16717=EDGE_LOOP('',(#38005,#38006,#38007,#38008));
#16718=EDGE_LOOP('',(#38009,#38010,#38011,#38012));
#16719=EDGE_LOOP('',(#38013,#38014,#38015,#38016,#38017,#38018,#38019,#38020,
#38021,#38022,#38023,#38024,#38025,#38026,#38027,#38028,#38029,#38030,#38031,
#38032,#38033,#38034,#38035,#38036,#38037,#38038,#38039,#38040,#38041,#38042,
#38043,#38044));
#16720=EDGE_LOOP('',(#38045,#38046,#38047,#38048));
#16721=EDGE_LOOP('',(#38049,#38050,#38051,#38052));
#16722=EDGE_LOOP('',(#38053,#38054,#38055,#38056));
#16723=EDGE_LOOP('',(#38057,#38058,#38059,#38060));
#16724=EDGE_LOOP('',(#38061,#38062,#38063,#38064));
#16725=EDGE_LOOP('',(#38065,#38066,#38067,#38068));
#16726=EDGE_LOOP('',(#38069,#38070,#38071,#38072));
#16727=EDGE_LOOP('',(#38073,#38074,#38075,#38076));
#16728=EDGE_LOOP('',(#38077,#38078,#38079,#38080));
#16729=EDGE_LOOP('',(#38081,#38082,#38083,#38084));
#16730=EDGE_LOOP('',(#38085,#38086,#38087,#38088));
#16731=EDGE_LOOP('',(#38089,#38090,#38091,#38092));
#16732=EDGE_LOOP('',(#38093,#38094,#38095,#38096));
#16733=EDGE_LOOP('',(#38097,#38098,#38099,#38100,#38101,#38102,#38103));
#16734=EDGE_LOOP('',(#38104,#38105,#38106,#38107));
#16735=EDGE_LOOP('',(#38108,#38109,#38110,#38111));
#16736=EDGE_LOOP('',(#38112,#38113,#38114,#38115));
#16737=EDGE_LOOP('',(#38116,#38117,#38118,#38119));
#16738=EDGE_LOOP('',(#38120,#38121,#38122,#38123));
#16739=EDGE_LOOP('',(#38124,#38125,#38126,#38127));
#16740=EDGE_LOOP('',(#38128,#38129,#38130,#38131));
#16741=EDGE_LOOP('',(#38132,#38133,#38134,#38135));
#16742=EDGE_LOOP('',(#38136,#38137,#38138,#38139));
#16743=EDGE_LOOP('',(#38140,#38141,#38142,#38143));
#16744=EDGE_LOOP('',(#38144,#38145,#38146,#38147));
#16745=EDGE_LOOP('',(#38148,#38149,#38150,#38151));
#16746=EDGE_LOOP('',(#38152,#38153,#38154,#38155));
#16747=EDGE_LOOP('',(#38156,#38157,#38158,#38159));
#16748=EDGE_LOOP('',(#38160,#38161,#38162,#38163,#38164,#38165,#38166,#38167,
#38168,#38169,#38170,#38171,#38172,#38173,#38174,#38175,#38176,#38177,#38178,
#38179,#38180,#38181,#38182,#38183,#38184,#38185,#38186,#38187,#38188,#38189,
#38190,#38191));
#16749=EDGE_LOOP('',(#38192,#38193,#38194,#38195));
#16750=EDGE_LOOP('',(#38196,#38197,#38198,#38199));
#16751=EDGE_LOOP('',(#38200,#38201,#38202,#38203));
#16752=EDGE_LOOP('',(#38204,#38205,#38206,#38207));
#16753=EDGE_LOOP('',(#38208,#38209,#38210,#38211));
#16754=EDGE_LOOP('',(#38212,#38213,#38214,#38215));
#16755=EDGE_LOOP('',(#38216,#38217,#38218,#38219));
#16756=EDGE_LOOP('',(#38220,#38221,#38222,#38223));
#16757=EDGE_LOOP('',(#38224,#38225,#38226,#38227));
#16758=EDGE_LOOP('',(#38228,#38229,#38230,#38231));
#16759=EDGE_LOOP('',(#38232,#38233,#38234,#38235));
#16760=EDGE_LOOP('',(#38236,#38237,#38238,#38239));
#16761=EDGE_LOOP('',(#38240,#38241,#38242,#38243));
#16762=EDGE_LOOP('',(#38244,#38245,#38246,#38247,#38248,#38249,#38250));
#16763=EDGE_LOOP('',(#38251,#38252,#38253,#38254));
#16764=EDGE_LOOP('',(#38255,#38256,#38257,#38258));
#16765=EDGE_LOOP('',(#38259,#38260,#38261,#38262));
#16766=EDGE_LOOP('',(#38263,#38264,#38265,#38266));
#16767=EDGE_LOOP('',(#38267,#38268,#38269,#38270));
#16768=EDGE_LOOP('',(#38271,#38272,#38273,#38274));
#16769=EDGE_LOOP('',(#38275,#38276,#38277,#38278));
#16770=EDGE_LOOP('',(#38279,#38280,#38281,#38282));
#16771=EDGE_LOOP('',(#38283,#38284,#38285,#38286));
#16772=EDGE_LOOP('',(#38287,#38288,#38289,#38290));
#16773=EDGE_LOOP('',(#38291,#38292,#38293,#38294));
#16774=EDGE_LOOP('',(#38295,#38296,#38297,#38298));
#16775=EDGE_LOOP('',(#38299,#38300,#38301,#38302));
#16776=EDGE_LOOP('',(#38303,#38304,#38305,#38306,#38307));
#16777=EDGE_LOOP('',(#38308,#38309,#38310,#38311,#38312,#38313,#38314,#38315,
#38316,#38317,#38318,#38319,#38320,#38321,#38322,#38323,#38324,#38325,#38326,
#38327,#38328,#38329,#38330,#38331,#38332,#38333,#38334,#38335,#38336,#38337,
#38338,#38339));
#16778=EDGE_LOOP('',(#38340,#38341,#38342,#38343));
#16779=EDGE_LOOP('',(#38344,#38345,#38346,#38347));
#16780=EDGE_LOOP('',(#38348,#38349,#38350,#38351));
#16781=EDGE_LOOP('',(#38352,#38353,#38354,#38355));
#16782=EDGE_LOOP('',(#38356,#38357,#38358,#38359));
#16783=EDGE_LOOP('',(#38360,#38361,#38362,#38363));
#16784=EDGE_LOOP('',(#38364,#38365,#38366,#38367));
#16785=EDGE_LOOP('',(#38368,#38369,#38370,#38371));
#16786=EDGE_LOOP('',(#38372,#38373,#38374,#38375));
#16787=EDGE_LOOP('',(#38376,#38377,#38378,#38379));
#16788=EDGE_LOOP('',(#38380,#38381,#38382,#38383));
#16789=EDGE_LOOP('',(#38384,#38385,#38386,#38387));
#16790=EDGE_LOOP('',(#38388,#38389,#38390,#38391));
#16791=EDGE_LOOP('',(#38392,#38393,#38394,#38395,#38396,#38397,#38398));
#16792=EDGE_LOOP('',(#38399,#38400,#38401,#38402));
#16793=EDGE_LOOP('',(#38403,#38404,#38405,#38406));
#16794=EDGE_LOOP('',(#38407,#38408,#38409,#38410));
#16795=EDGE_LOOP('',(#38411,#38412,#38413,#38414));
#16796=EDGE_LOOP('',(#38415,#38416,#38417,#38418));
#16797=EDGE_LOOP('',(#38419,#38420,#38421,#38422));
#16798=EDGE_LOOP('',(#38423,#38424,#38425,#38426));
#16799=EDGE_LOOP('',(#38427,#38428,#38429,#38430));
#16800=EDGE_LOOP('',(#38431,#38432,#38433,#38434));
#16801=EDGE_LOOP('',(#38435,#38436,#38437,#38438));
#16802=EDGE_LOOP('',(#38439,#38440,#38441,#38442));
#16803=EDGE_LOOP('',(#38443,#38444,#38445,#38446));
#16804=EDGE_LOOP('',(#38447,#38448,#38449,#38450));
#16805=EDGE_LOOP('',(#38451,#38452,#38453,#38454));
#16806=EDGE_LOOP('',(#38455,#38456,#38457,#38458,#38459,#38460,#38461,#38462,
#38463,#38464,#38465,#38466,#38467,#38468,#38469,#38470,#38471,#38472,#38473,
#38474,#38475,#38476,#38477,#38478,#38479,#38480,#38481,#38482,#38483,#38484,
#38485,#38486));
#16807=EDGE_LOOP('',(#38487,#38488,#38489,#38490));
#16808=EDGE_LOOP('',(#38491,#38492,#38493,#38494));
#16809=EDGE_LOOP('',(#38495,#38496,#38497,#38498));
#16810=EDGE_LOOP('',(#38499,#38500,#38501,#38502));
#16811=EDGE_LOOP('',(#38503,#38504,#38505,#38506));
#16812=EDGE_LOOP('',(#38507,#38508,#38509,#38510));
#16813=EDGE_LOOP('',(#38511,#38512,#38513,#38514));
#16814=EDGE_LOOP('',(#38515,#38516,#38517,#38518));
#16815=EDGE_LOOP('',(#38519,#38520,#38521,#38522));
#16816=EDGE_LOOP('',(#38523,#38524,#38525,#38526));
#16817=EDGE_LOOP('',(#38527,#38528,#38529,#38530));
#16818=EDGE_LOOP('',(#38531,#38532,#38533,#38534));
#16819=EDGE_LOOP('',(#38535,#38536,#38537,#38538));
#16820=EDGE_LOOP('',(#38539,#38540,#38541,#38542,#38543,#38544,#38545));
#16821=EDGE_LOOP('',(#38546,#38547,#38548,#38549));
#16822=EDGE_LOOP('',(#38550,#38551,#38552,#38553));
#16823=EDGE_LOOP('',(#38554,#38555,#38556,#38557));
#16824=EDGE_LOOP('',(#38558,#38559,#38560,#38561));
#16825=EDGE_LOOP('',(#38562,#38563,#38564,#38565));
#16826=EDGE_LOOP('',(#38566,#38567,#38568,#38569));
#16827=EDGE_LOOP('',(#38570,#38571,#38572,#38573));
#16828=EDGE_LOOP('',(#38574,#38575,#38576,#38577));
#16829=EDGE_LOOP('',(#38578,#38579,#38580,#38581));
#16830=EDGE_LOOP('',(#38582,#38583,#38584,#38585));
#16831=EDGE_LOOP('',(#38586,#38587,#38588,#38589));
#16832=EDGE_LOOP('',(#38590,#38591,#38592,#38593));
#16833=EDGE_LOOP('',(#38594,#38595,#38596,#38597));
#16834=EDGE_LOOP('',(#38598,#38599,#38600,#38601));
#16835=EDGE_LOOP('',(#38602,#38603,#38604,#38605,#38606,#38607,#38608,#38609,
#38610,#38611,#38612,#38613,#38614,#38615,#38616,#38617,#38618,#38619,#38620,
#38621,#38622,#38623,#38624,#38625,#38626,#38627,#38628,#38629,#38630,#38631,
#38632,#38633));
#16836=EDGE_LOOP('',(#38634,#38635,#38636,#38637));
#16837=EDGE_LOOP('',(#38638,#38639,#38640,#38641));
#16838=EDGE_LOOP('',(#38642,#38643,#38644,#38645));
#16839=EDGE_LOOP('',(#38646,#38647,#38648,#38649));
#16840=EDGE_LOOP('',(#38650,#38651,#38652,#38653));
#16841=EDGE_LOOP('',(#38654,#38655,#38656,#38657));
#16842=EDGE_LOOP('',(#38658,#38659,#38660,#38661));
#16843=EDGE_LOOP('',(#38662,#38663,#38664,#38665));
#16844=EDGE_LOOP('',(#38666,#38667,#38668,#38669));
#16845=EDGE_LOOP('',(#38670,#38671,#38672,#38673));
#16846=EDGE_LOOP('',(#38674,#38675,#38676,#38677));
#16847=EDGE_LOOP('',(#38678,#38679,#38680,#38681));
#16848=EDGE_LOOP('',(#38682,#38683,#38684,#38685));
#16849=EDGE_LOOP('',(#38686,#38687,#38688,#38689,#38690,#38691,#38692));
#16850=EDGE_LOOP('',(#38693,#38694,#38695,#38696));
#16851=EDGE_LOOP('',(#38697,#38698,#38699,#38700));
#16852=EDGE_LOOP('',(#38701,#38702,#38703,#38704));
#16853=EDGE_LOOP('',(#38705,#38706,#38707,#38708));
#16854=EDGE_LOOP('',(#38709,#38710,#38711,#38712));
#16855=EDGE_LOOP('',(#38713,#38714,#38715,#38716));
#16856=EDGE_LOOP('',(#38717,#38718,#38719,#38720));
#16857=EDGE_LOOP('',(#38721,#38722,#38723,#38724));
#16858=EDGE_LOOP('',(#38725,#38726,#38727,#38728));
#16859=EDGE_LOOP('',(#38729,#38730,#38731,#38732));
#16860=EDGE_LOOP('',(#38733,#38734,#38735,#38736));
#16861=EDGE_LOOP('',(#38737,#38738,#38739,#38740));
#16862=EDGE_LOOP('',(#38741,#38742,#38743,#38744));
#16863=EDGE_LOOP('',(#38745,#38746,#38747,#38748));
#16864=EDGE_LOOP('',(#38749,#38750,#38751,#38752,#38753,#38754,#38755,#38756,
#38757,#38758,#38759,#38760,#38761,#38762,#38763,#38764,#38765,#38766,#38767,
#38768,#38769,#38770,#38771,#38772,#38773,#38774,#38775,#38776,#38777,#38778,
#38779,#38780));
#16865=EDGE_LOOP('',(#38781,#38782,#38783,#38784));
#16866=EDGE_LOOP('',(#38785,#38786,#38787,#38788));
#16867=EDGE_LOOP('',(#38789,#38790,#38791,#38792));
#16868=EDGE_LOOP('',(#38793,#38794,#38795,#38796));
#16869=EDGE_LOOP('',(#38797,#38798,#38799,#38800));
#16870=EDGE_LOOP('',(#38801,#38802,#38803,#38804));
#16871=EDGE_LOOP('',(#38805,#38806,#38807,#38808));
#16872=EDGE_LOOP('',(#38809,#38810,#38811,#38812));
#16873=EDGE_LOOP('',(#38813,#38814,#38815,#38816));
#16874=EDGE_LOOP('',(#38817,#38818,#38819,#38820));
#16875=EDGE_LOOP('',(#38821,#38822,#38823,#38824));
#16876=EDGE_LOOP('',(#38825,#38826,#38827,#38828));
#16877=EDGE_LOOP('',(#38829,#38830,#38831,#38832));
#16878=EDGE_LOOP('',(#38833,#38834,#38835,#38836,#38837,#38838,#38839));
#16879=EDGE_LOOP('',(#38840,#38841,#38842,#38843));
#16880=EDGE_LOOP('',(#38844,#38845,#38846,#38847));
#16881=EDGE_LOOP('',(#38848,#38849,#38850,#38851));
#16882=EDGE_LOOP('',(#38852,#38853,#38854,#38855));
#16883=EDGE_LOOP('',(#38856,#38857,#38858,#38859));
#16884=EDGE_LOOP('',(#38860,#38861,#38862,#38863));
#16885=EDGE_LOOP('',(#38864,#38865,#38866,#38867));
#16886=EDGE_LOOP('',(#38868,#38869,#38870,#38871));
#16887=EDGE_LOOP('',(#38872,#38873,#38874,#38875));
#16888=EDGE_LOOP('',(#38876,#38877,#38878,#38879));
#16889=EDGE_LOOP('',(#38880,#38881,#38882,#38883));
#16890=EDGE_LOOP('',(#38884,#38885,#38886,#38887));
#16891=EDGE_LOOP('',(#38888,#38889,#38890,#38891));
#16892=EDGE_LOOP('',(#38892,#38893,#38894,#38895));
#16893=EDGE_LOOP('',(#38896,#38897,#38898,#38899,#38900,#38901,#38902,#38903,
#38904,#38905,#38906,#38907,#38908,#38909,#38910,#38911,#38912,#38913,#38914,
#38915,#38916,#38917,#38918,#38919,#38920,#38921,#38922,#38923,#38924,#38925,
#38926,#38927));
#16894=EDGE_LOOP('',(#38928,#38929,#38930,#38931));
#16895=EDGE_LOOP('',(#38932,#38933,#38934,#38935));
#16896=EDGE_LOOP('',(#38936,#38937,#38938,#38939));
#16897=EDGE_LOOP('',(#38940,#38941,#38942,#38943));
#16898=EDGE_LOOP('',(#38944,#38945,#38946,#38947));
#16899=EDGE_LOOP('',(#38948,#38949,#38950,#38951));
#16900=EDGE_LOOP('',(#38952,#38953,#38954,#38955));
#16901=EDGE_LOOP('',(#38956,#38957,#38958,#38959));
#16902=EDGE_LOOP('',(#38960,#38961,#38962,#38963));
#16903=EDGE_LOOP('',(#38964,#38965,#38966,#38967));
#16904=EDGE_LOOP('',(#38968,#38969,#38970,#38971));
#16905=EDGE_LOOP('',(#38972,#38973,#38974,#38975));
#16906=EDGE_LOOP('',(#38976,#38977,#38978,#38979));
#16907=EDGE_LOOP('',(#38980,#38981,#38982,#38983,#38984,#38985,#38986));
#16908=EDGE_LOOP('',(#38987,#38988,#38989,#38990));
#16909=EDGE_LOOP('',(#38991,#38992,#38993,#38994));
#16910=EDGE_LOOP('',(#38995,#38996,#38997,#38998));
#16911=EDGE_LOOP('',(#38999,#39000,#39001,#39002));
#16912=EDGE_LOOP('',(#39003,#39004,#39005,#39006));
#16913=EDGE_LOOP('',(#39007,#39008,#39009,#39010));
#16914=EDGE_LOOP('',(#39011,#39012,#39013,#39014));
#16915=EDGE_LOOP('',(#39015,#39016,#39017,#39018));
#16916=EDGE_LOOP('',(#39019,#39020,#39021,#39022));
#16917=EDGE_LOOP('',(#39023,#39024,#39025,#39026));
#16918=EDGE_LOOP('',(#39027,#39028,#39029,#39030));
#16919=EDGE_LOOP('',(#39031,#39032,#39033,#39034));
#16920=EDGE_LOOP('',(#39035,#39036,#39037,#39038));
#16921=EDGE_LOOP('',(#39039,#39040,#39041,#39042));
#16922=EDGE_LOOP('',(#39043,#39044,#39045,#39046,#39047,#39048,#39049,#39050,
#39051,#39052,#39053,#39054,#39055,#39056,#39057,#39058,#39059,#39060,#39061,
#39062,#39063,#39064,#39065,#39066,#39067,#39068,#39069,#39070,#39071,#39072,
#39073,#39074));
#16923=EDGE_LOOP('',(#39075,#39076,#39077,#39078));
#16924=EDGE_LOOP('',(#39079,#39080,#39081,#39082));
#16925=EDGE_LOOP('',(#39083,#39084,#39085,#39086));
#16926=EDGE_LOOP('',(#39087,#39088,#39089,#39090));
#16927=EDGE_LOOP('',(#39091,#39092,#39093,#39094));
#16928=EDGE_LOOP('',(#39095,#39096,#39097,#39098));
#16929=EDGE_LOOP('',(#39099,#39100,#39101,#39102));
#16930=EDGE_LOOP('',(#39103,#39104,#39105,#39106));
#16931=EDGE_LOOP('',(#39107,#39108,#39109,#39110));
#16932=EDGE_LOOP('',(#39111,#39112,#39113,#39114));
#16933=EDGE_LOOP('',(#39115,#39116,#39117,#39118));
#16934=EDGE_LOOP('',(#39119,#39120,#39121,#39122));
#16935=EDGE_LOOP('',(#39123,#39124,#39125,#39126));
#16936=EDGE_LOOP('',(#39127,#39128,#39129,#39130,#39131,#39132,#39133));
#16937=EDGE_LOOP('',(#39134,#39135,#39136,#39137));
#16938=EDGE_LOOP('',(#39138,#39139,#39140,#39141));
#16939=EDGE_LOOP('',(#39142,#39143,#39144,#39145));
#16940=EDGE_LOOP('',(#39146,#39147,#39148,#39149));
#16941=EDGE_LOOP('',(#39150,#39151,#39152,#39153));
#16942=EDGE_LOOP('',(#39154,#39155,#39156,#39157));
#16943=EDGE_LOOP('',(#39158,#39159,#39160,#39161));
#16944=EDGE_LOOP('',(#39162,#39163,#39164,#39165));
#16945=EDGE_LOOP('',(#39166,#39167,#39168,#39169));
#16946=EDGE_LOOP('',(#39170,#39171,#39172,#39173));
#16947=EDGE_LOOP('',(#39174,#39175,#39176,#39177));
#16948=EDGE_LOOP('',(#39178,#39179,#39180,#39181));
#16949=EDGE_LOOP('',(#39182,#39183,#39184,#39185));
#16950=EDGE_LOOP('',(#39186,#39187,#39188,#39189));
#16951=EDGE_LOOP('',(#39190,#39191,#39192,#39193,#39194,#39195,#39196,#39197,
#39198,#39199,#39200,#39201,#39202,#39203,#39204,#39205,#39206,#39207,#39208,
#39209,#39210,#39211,#39212,#39213,#39214,#39215,#39216,#39217,#39218,#39219,
#39220,#39221));
#16952=EDGE_LOOP('',(#39222,#39223,#39224,#39225));
#16953=EDGE_LOOP('',(#39226,#39227,#39228,#39229));
#16954=EDGE_LOOP('',(#39230,#39231,#39232,#39233));
#16955=EDGE_LOOP('',(#39234,#39235,#39236,#39237));
#16956=EDGE_LOOP('',(#39238,#39239,#39240,#39241));
#16957=EDGE_LOOP('',(#39242,#39243,#39244,#39245));
#16958=EDGE_LOOP('',(#39246,#39247,#39248,#39249));
#16959=EDGE_LOOP('',(#39250,#39251,#39252,#39253));
#16960=EDGE_LOOP('',(#39254,#39255,#39256,#39257));
#16961=EDGE_LOOP('',(#39258,#39259,#39260,#39261));
#16962=EDGE_LOOP('',(#39262,#39263,#39264,#39265));
#16963=EDGE_LOOP('',(#39266,#39267,#39268,#39269));
#16964=EDGE_LOOP('',(#39270,#39271,#39272,#39273));
#16965=EDGE_LOOP('',(#39274,#39275,#39276,#39277,#39278,#39279,#39280));
#16966=EDGE_LOOP('',(#39281,#39282,#39283,#39284));
#16967=EDGE_LOOP('',(#39285,#39286,#39287,#39288));
#16968=EDGE_LOOP('',(#39289,#39290,#39291,#39292));
#16969=EDGE_LOOP('',(#39293,#39294,#39295,#39296));
#16970=EDGE_LOOP('',(#39297,#39298,#39299,#39300));
#16971=EDGE_LOOP('',(#39301,#39302,#39303,#39304));
#16972=EDGE_LOOP('',(#39305,#39306,#39307,#39308));
#16973=EDGE_LOOP('',(#39309,#39310,#39311,#39312));
#16974=EDGE_LOOP('',(#39313,#39314,#39315,#39316));
#16975=EDGE_LOOP('',(#39317,#39318,#39319,#39320));
#16976=EDGE_LOOP('',(#39321,#39322,#39323,#39324));
#16977=EDGE_LOOP('',(#39325,#39326,#39327,#39328));
#16978=EDGE_LOOP('',(#39329,#39330,#39331,#39332));
#16979=EDGE_LOOP('',(#39333,#39334,#39335,#39336));
#16980=EDGE_LOOP('',(#39337,#39338,#39339,#39340,#39341,#39342,#39343,#39344,
#39345,#39346,#39347,#39348,#39349,#39350,#39351,#39352,#39353,#39354,#39355,
#39356,#39357,#39358,#39359,#39360,#39361,#39362,#39363,#39364,#39365,#39366,
#39367,#39368));
#16981=EDGE_LOOP('',(#39369,#39370,#39371,#39372));
#16982=EDGE_LOOP('',(#39373,#39374,#39375,#39376));
#16983=EDGE_LOOP('',(#39377,#39378,#39379,#39380));
#16984=EDGE_LOOP('',(#39381,#39382,#39383,#39384));
#16985=EDGE_LOOP('',(#39385,#39386,#39387,#39388));
#16986=EDGE_LOOP('',(#39389,#39390,#39391,#39392));
#16987=EDGE_LOOP('',(#39393,#39394,#39395,#39396));
#16988=EDGE_LOOP('',(#39397,#39398,#39399,#39400));
#16989=EDGE_LOOP('',(#39401,#39402,#39403,#39404));
#16990=EDGE_LOOP('',(#39405,#39406,#39407,#39408));
#16991=EDGE_LOOP('',(#39409,#39410,#39411,#39412));
#16992=EDGE_LOOP('',(#39413,#39414,#39415,#39416));
#16993=EDGE_LOOP('',(#39417,#39418,#39419,#39420));
#16994=EDGE_LOOP('',(#39421,#39422,#39423,#39424,#39425,#39426,#39427));
#16995=EDGE_LOOP('',(#39428,#39429,#39430,#39431));
#16996=EDGE_LOOP('',(#39432,#39433,#39434,#39435));
#16997=EDGE_LOOP('',(#39436,#39437,#39438,#39439));
#16998=EDGE_LOOP('',(#39440,#39441,#39442,#39443));
#16999=EDGE_LOOP('',(#39444,#39445,#39446,#39447));
#17000=EDGE_LOOP('',(#39448,#39449,#39450,#39451));
#17001=EDGE_LOOP('',(#39452,#39453,#39454,#39455));
#17002=EDGE_LOOP('',(#39456,#39457,#39458,#39459));
#17003=EDGE_LOOP('',(#39460,#39461,#39462,#39463));
#17004=EDGE_LOOP('',(#39464,#39465,#39466,#39467));
#17005=EDGE_LOOP('',(#39468,#39469,#39470,#39471));
#17006=EDGE_LOOP('',(#39472,#39473,#39474,#39475));
#17007=EDGE_LOOP('',(#39476,#39477,#39478,#39479));
#17008=EDGE_LOOP('',(#39480,#39481,#39482,#39483));
#17009=EDGE_LOOP('',(#39484,#39485,#39486,#39487,#39488,#39489,#39490,#39491,
#39492,#39493,#39494,#39495,#39496,#39497,#39498,#39499,#39500,#39501,#39502,
#39503,#39504,#39505,#39506,#39507,#39508,#39509,#39510,#39511,#39512,#39513,
#39514,#39515));
#17010=EDGE_LOOP('',(#39516,#39517,#39518,#39519));
#17011=EDGE_LOOP('',(#39520,#39521,#39522,#39523));
#17012=EDGE_LOOP('',(#39524,#39525,#39526,#39527));
#17013=EDGE_LOOP('',(#39528,#39529,#39530,#39531));
#17014=EDGE_LOOP('',(#39532,#39533,#39534,#39535));
#17015=EDGE_LOOP('',(#39536,#39537,#39538,#39539));
#17016=EDGE_LOOP('',(#39540,#39541,#39542,#39543));
#17017=EDGE_LOOP('',(#39544,#39545,#39546,#39547));
#17018=EDGE_LOOP('',(#39548,#39549,#39550,#39551));
#17019=EDGE_LOOP('',(#39552,#39553,#39554,#39555));
#17020=EDGE_LOOP('',(#39556,#39557,#39558,#39559));
#17021=EDGE_LOOP('',(#39560,#39561,#39562,#39563));
#17022=EDGE_LOOP('',(#39564,#39565,#39566,#39567));
#17023=EDGE_LOOP('',(#39568,#39569,#39570,#39571,#39572,#39573,#39574));
#17024=EDGE_LOOP('',(#39575,#39576,#39577,#39578));
#17025=EDGE_LOOP('',(#39579,#39580,#39581,#39582));
#17026=EDGE_LOOP('',(#39583,#39584,#39585,#39586));
#17027=EDGE_LOOP('',(#39587,#39588,#39589,#39590));
#17028=EDGE_LOOP('',(#39591,#39592,#39593,#39594));
#17029=EDGE_LOOP('',(#39595,#39596,#39597,#39598));
#17030=EDGE_LOOP('',(#39599,#39600,#39601,#39602));
#17031=EDGE_LOOP('',(#39603,#39604,#39605,#39606));
#17032=EDGE_LOOP('',(#39607,#39608,#39609,#39610));
#17033=EDGE_LOOP('',(#39611,#39612,#39613,#39614));
#17034=EDGE_LOOP('',(#39615,#39616,#39617,#39618));
#17035=EDGE_LOOP('',(#39619,#39620,#39621,#39622));
#17036=EDGE_LOOP('',(#39623,#39624,#39625,#39626));
#17037=EDGE_LOOP('',(#39627,#39628,#39629,#39630));
#17038=EDGE_LOOP('',(#39631,#39632,#39633,#39634,#39635,#39636,#39637,#39638,
#39639,#39640,#39641,#39642,#39643,#39644,#39645,#39646,#39647,#39648,#39649,
#39650,#39651,#39652,#39653,#39654,#39655,#39656,#39657,#39658,#39659,#39660,
#39661,#39662));
#17039=EDGE_LOOP('',(#39663,#39664,#39665,#39666));
#17040=EDGE_LOOP('',(#39667,#39668,#39669,#39670));
#17041=EDGE_LOOP('',(#39671,#39672,#39673,#39674));
#17042=EDGE_LOOP('',(#39675,#39676,#39677,#39678));
#17043=EDGE_LOOP('',(#39679,#39680,#39681,#39682));
#17044=EDGE_LOOP('',(#39683,#39684,#39685,#39686));
#17045=EDGE_LOOP('',(#39687,#39688,#39689,#39690));
#17046=EDGE_LOOP('',(#39691,#39692,#39693,#39694));
#17047=EDGE_LOOP('',(#39695,#39696,#39697,#39698));
#17048=EDGE_LOOP('',(#39699,#39700,#39701,#39702));
#17049=EDGE_LOOP('',(#39703,#39704,#39705,#39706));
#17050=EDGE_LOOP('',(#39707,#39708,#39709,#39710));
#17051=EDGE_LOOP('',(#39711,#39712,#39713,#39714));
#17052=EDGE_LOOP('',(#39715,#39716,#39717,#39718,#39719,#39720,#39721));
#17053=EDGE_LOOP('',(#39722,#39723,#39724,#39725));
#17054=EDGE_LOOP('',(#39726,#39727,#39728,#39729));
#17055=EDGE_LOOP('',(#39730,#39731,#39732,#39733));
#17056=EDGE_LOOP('',(#39734,#39735,#39736,#39737));
#17057=EDGE_LOOP('',(#39738,#39739,#39740,#39741));
#17058=EDGE_LOOP('',(#39742,#39743,#39744,#39745));
#17059=EDGE_LOOP('',(#39746,#39747,#39748,#39749));
#17060=EDGE_LOOP('',(#39750,#39751,#39752,#39753));
#17061=EDGE_LOOP('',(#39754,#39755,#39756,#39757));
#17062=EDGE_LOOP('',(#39758,#39759,#39760,#39761));
#17063=EDGE_LOOP('',(#39762,#39763,#39764,#39765));
#17064=EDGE_LOOP('',(#39766,#39767,#39768,#39769));
#17065=EDGE_LOOP('',(#39770,#39771,#39772,#39773));
#17066=EDGE_LOOP('',(#39774,#39775,#39776,#39777));
#17067=EDGE_LOOP('',(#39778,#39779,#39780,#39781,#39782,#39783,#39784,#39785,
#39786,#39787,#39788,#39789,#39790,#39791,#39792,#39793,#39794,#39795,#39796,
#39797,#39798,#39799,#39800,#39801,#39802,#39803,#39804,#39805,#39806,#39807,
#39808,#39809));
#17068=EDGE_LOOP('',(#39810,#39811,#39812,#39813));
#17069=EDGE_LOOP('',(#39814,#39815,#39816,#39817));
#17070=EDGE_LOOP('',(#39818,#39819,#39820,#39821));
#17071=EDGE_LOOP('',(#39822,#39823,#39824,#39825));
#17072=EDGE_LOOP('',(#39826,#39827,#39828,#39829));
#17073=EDGE_LOOP('',(#39830,#39831,#39832,#39833));
#17074=EDGE_LOOP('',(#39834,#39835,#39836,#39837));
#17075=EDGE_LOOP('',(#39838,#39839,#39840,#39841));
#17076=EDGE_LOOP('',(#39842,#39843,#39844,#39845));
#17077=EDGE_LOOP('',(#39846,#39847,#39848,#39849));
#17078=EDGE_LOOP('',(#39850,#39851,#39852,#39853));
#17079=EDGE_LOOP('',(#39854,#39855,#39856,#39857));
#17080=EDGE_LOOP('',(#39858,#39859,#39860,#39861));
#17081=EDGE_LOOP('',(#39862,#39863,#39864,#39865,#39866,#39867,#39868));
#17082=EDGE_LOOP('',(#39869,#39870,#39871,#39872));
#17083=EDGE_LOOP('',(#39873,#39874,#39875,#39876));
#17084=EDGE_LOOP('',(#39877,#39878,#39879,#39880));
#17085=EDGE_LOOP('',(#39881,#39882,#39883,#39884));
#17086=EDGE_LOOP('',(#39885,#39886,#39887,#39888));
#17087=EDGE_LOOP('',(#39889,#39890,#39891,#39892));
#17088=EDGE_LOOP('',(#39893,#39894,#39895,#39896));
#17089=EDGE_LOOP('',(#39897,#39898,#39899,#39900));
#17090=EDGE_LOOP('',(#39901,#39902,#39903,#39904));
#17091=EDGE_LOOP('',(#39905,#39906,#39907,#39908));
#17092=EDGE_LOOP('',(#39909,#39910,#39911,#39912));
#17093=EDGE_LOOP('',(#39913,#39914,#39915,#39916));
#17094=EDGE_LOOP('',(#39917,#39918,#39919,#39920));
#17095=EDGE_LOOP('',(#39921,#39922,#39923,#39924));
#17096=EDGE_LOOP('',(#39925,#39926,#39927,#39928,#39929,#39930,#39931,#39932,
#39933,#39934,#39935,#39936,#39937,#39938,#39939,#39940,#39941,#39942,#39943,
#39944,#39945,#39946,#39947,#39948,#39949,#39950,#39951,#39952,#39953,#39954,
#39955,#39956));
#17097=EDGE_LOOP('',(#39957,#39958,#39959,#39960));
#17098=EDGE_LOOP('',(#39961,#39962,#39963,#39964));
#17099=EDGE_LOOP('',(#39965,#39966,#39967,#39968));
#17100=EDGE_LOOP('',(#39969,#39970,#39971,#39972));
#17101=EDGE_LOOP('',(#39973,#39974,#39975,#39976));
#17102=EDGE_LOOP('',(#39977,#39978,#39979,#39980));
#17103=EDGE_LOOP('',(#39981,#39982,#39983,#39984));
#17104=EDGE_LOOP('',(#39985,#39986,#39987,#39988));
#17105=EDGE_LOOP('',(#39989,#39990,#39991,#39992));
#17106=EDGE_LOOP('',(#39993,#39994,#39995,#39996));
#17107=EDGE_LOOP('',(#39997,#39998,#39999,#40000));
#17108=EDGE_LOOP('',(#40001,#40002,#40003,#40004));
#17109=EDGE_LOOP('',(#40005,#40006,#40007,#40008));
#17110=EDGE_LOOP('',(#40009,#40010,#40011,#40012,#40013,#40014,#40015));
#17111=EDGE_LOOP('',(#40016,#40017,#40018,#40019));
#17112=EDGE_LOOP('',(#40020,#40021,#40022,#40023));
#17113=EDGE_LOOP('',(#40024,#40025,#40026,#40027));
#17114=EDGE_LOOP('',(#40028,#40029,#40030,#40031));
#17115=EDGE_LOOP('',(#40032,#40033,#40034,#40035));
#17116=EDGE_LOOP('',(#40036,#40037,#40038,#40039));
#17117=EDGE_LOOP('',(#40040,#40041,#40042,#40043));
#17118=EDGE_LOOP('',(#40044,#40045,#40046,#40047));
#17119=EDGE_LOOP('',(#40048,#40049,#40050,#40051));
#17120=EDGE_LOOP('',(#40052,#40053,#40054,#40055));
#17121=EDGE_LOOP('',(#40056,#40057,#40058,#40059));
#17122=EDGE_LOOP('',(#40060,#40061,#40062,#40063));
#17123=EDGE_LOOP('',(#40064,#40065,#40066,#40067));
#17124=EDGE_LOOP('',(#40068,#40069,#40070,#40071));
#17125=EDGE_LOOP('',(#40072,#40073,#40074,#40075,#40076,#40077,#40078,#40079,
#40080,#40081,#40082,#40083,#40084,#40085,#40086,#40087,#40088,#40089,#40090,
#40091,#40092,#40093,#40094,#40095,#40096,#40097,#40098,#40099,#40100,#40101,
#40102,#40103));
#17126=EDGE_LOOP('',(#40104,#40105,#40106,#40107));
#17127=EDGE_LOOP('',(#40108,#40109,#40110,#40111));
#17128=EDGE_LOOP('',(#40112,#40113,#40114,#40115));
#17129=EDGE_LOOP('',(#40116,#40117,#40118,#40119));
#17130=EDGE_LOOP('',(#40120,#40121,#40122,#40123));
#17131=EDGE_LOOP('',(#40124,#40125,#40126,#40127));
#17132=EDGE_LOOP('',(#40128,#40129,#40130,#40131));
#17133=EDGE_LOOP('',(#40132,#40133,#40134,#40135));
#17134=EDGE_LOOP('',(#40136,#40137,#40138,#40139));
#17135=EDGE_LOOP('',(#40140,#40141,#40142,#40143));
#17136=EDGE_LOOP('',(#40144,#40145,#40146,#40147));
#17137=EDGE_LOOP('',(#40148,#40149,#40150,#40151));
#17138=EDGE_LOOP('',(#40152,#40153,#40154,#40155));
#17139=EDGE_LOOP('',(#40156,#40157,#40158,#40159,#40160,#40161,#40162));
#17140=EDGE_LOOP('',(#40163,#40164,#40165,#40166));
#17141=EDGE_LOOP('',(#40167,#40168,#40169,#40170));
#17142=EDGE_LOOP('',(#40171,#40172,#40173,#40174));
#17143=EDGE_LOOP('',(#40175,#40176,#40177,#40178));
#17144=EDGE_LOOP('',(#40179,#40180,#40181,#40182));
#17145=EDGE_LOOP('',(#40183,#40184,#40185,#40186));
#17146=EDGE_LOOP('',(#40187,#40188,#40189,#40190));
#17147=EDGE_LOOP('',(#40191,#40192,#40193,#40194));
#17148=EDGE_LOOP('',(#40195,#40196,#40197,#40198));
#17149=EDGE_LOOP('',(#40199,#40200,#40201,#40202));
#17150=EDGE_LOOP('',(#40203,#40204,#40205,#40206));
#17151=EDGE_LOOP('',(#40207,#40208,#40209,#40210));
#17152=EDGE_LOOP('',(#40211,#40212,#40213,#40214));
#17153=EDGE_LOOP('',(#40215,#40216,#40217,#40218));
#17154=EDGE_LOOP('',(#40219,#40220,#40221,#40222,#40223,#40224,#40225,#40226,
#40227,#40228,#40229,#40230,#40231,#40232,#40233,#40234,#40235,#40236,#40237,
#40238,#40239,#40240,#40241,#40242,#40243,#40244,#40245,#40246,#40247,#40248,
#40249,#40250));
#17155=EDGE_LOOP('',(#40251,#40252,#40253,#40254));
#17156=EDGE_LOOP('',(#40255,#40256,#40257,#40258));
#17157=EDGE_LOOP('',(#40259,#40260,#40261,#40262));
#17158=EDGE_LOOP('',(#40263,#40264,#40265,#40266));
#17159=EDGE_LOOP('',(#40267,#40268,#40269,#40270));
#17160=EDGE_LOOP('',(#40271,#40272,#40273,#40274));
#17161=EDGE_LOOP('',(#40275,#40276,#40277,#40278));
#17162=EDGE_LOOP('',(#40279,#40280,#40281,#40282));
#17163=EDGE_LOOP('',(#40283,#40284,#40285,#40286));
#17164=EDGE_LOOP('',(#40287,#40288,#40289,#40290));
#17165=EDGE_LOOP('',(#40291,#40292,#40293,#40294));
#17166=EDGE_LOOP('',(#40295,#40296,#40297,#40298));
#17167=EDGE_LOOP('',(#40299,#40300,#40301,#40302));
#17168=EDGE_LOOP('',(#40303,#40304,#40305,#40306,#40307,#40308,#40309));
#17169=EDGE_LOOP('',(#40310,#40311,#40312,#40313));
#17170=EDGE_LOOP('',(#40314,#40315,#40316,#40317));
#17171=EDGE_LOOP('',(#40318,#40319,#40320,#40321));
#17172=EDGE_LOOP('',(#40322,#40323,#40324,#40325));
#17173=EDGE_LOOP('',(#40326,#40327,#40328,#40329));
#17174=EDGE_LOOP('',(#40330,#40331,#40332,#40333));
#17175=EDGE_LOOP('',(#40334,#40335,#40336,#40337));
#17176=EDGE_LOOP('',(#40338,#40339,#40340,#40341));
#17177=EDGE_LOOP('',(#40342,#40343,#40344,#40345));
#17178=EDGE_LOOP('',(#40346,#40347,#40348,#40349));
#17179=EDGE_LOOP('',(#40350,#40351,#40352,#40353));
#17180=EDGE_LOOP('',(#40354,#40355,#40356,#40357));
#17181=EDGE_LOOP('',(#40358,#40359,#40360,#40361));
#17182=EDGE_LOOP('',(#40362,#40363,#40364,#40365));
#17183=EDGE_LOOP('',(#40366,#40367,#40368,#40369,#40370,#40371,#40372,#40373,
#40374,#40375,#40376,#40377,#40378,#40379,#40380,#40381,#40382,#40383,#40384,
#40385,#40386,#40387,#40388,#40389,#40390,#40391,#40392,#40393,#40394,#40395,
#40396,#40397));
#17184=EDGE_LOOP('',(#40398,#40399,#40400,#40401));
#17185=EDGE_LOOP('',(#40402,#40403,#40404,#40405));
#17186=EDGE_LOOP('',(#40406,#40407,#40408,#40409));
#17187=EDGE_LOOP('',(#40410,#40411,#40412,#40413));
#17188=EDGE_LOOP('',(#40414,#40415,#40416,#40417));
#17189=EDGE_LOOP('',(#40418,#40419,#40420,#40421));
#17190=EDGE_LOOP('',(#40422,#40423,#40424,#40425));
#17191=EDGE_LOOP('',(#40426,#40427,#40428,#40429));
#17192=EDGE_LOOP('',(#40430,#40431,#40432,#40433));
#17193=EDGE_LOOP('',(#40434,#40435,#40436,#40437));
#17194=EDGE_LOOP('',(#40438,#40439,#40440,#40441));
#17195=EDGE_LOOP('',(#40442,#40443,#40444,#40445));
#17196=EDGE_LOOP('',(#40446,#40447,#40448,#40449));
#17197=EDGE_LOOP('',(#40450,#40451,#40452,#40453,#40454,#40455,#40456));
#17198=EDGE_LOOP('',(#40457,#40458,#40459,#40460));
#17199=EDGE_LOOP('',(#40461,#40462,#40463,#40464));
#17200=EDGE_LOOP('',(#40465,#40466,#40467,#40468));
#17201=EDGE_LOOP('',(#40469,#40470,#40471,#40472));
#17202=EDGE_LOOP('',(#40473,#40474,#40475,#40476));
#17203=EDGE_LOOP('',(#40477,#40478,#40479,#40480));
#17204=EDGE_LOOP('',(#40481,#40482,#40483,#40484));
#17205=EDGE_LOOP('',(#40485,#40486,#40487,#40488));
#17206=EDGE_LOOP('',(#40489,#40490,#40491,#40492));
#17207=EDGE_LOOP('',(#40493,#40494,#40495,#40496));
#17208=EDGE_LOOP('',(#40497,#40498,#40499,#40500));
#17209=EDGE_LOOP('',(#40501,#40502,#40503,#40504));
#17210=EDGE_LOOP('',(#40505,#40506,#40507,#40508));
#17211=EDGE_LOOP('',(#40509,#40510,#40511,#40512));
#17212=EDGE_LOOP('',(#40513,#40514,#40515,#40516,#40517,#40518,#40519,#40520,
#40521,#40522,#40523,#40524,#40525,#40526,#40527,#40528,#40529,#40530,#40531,
#40532,#40533,#40534,#40535,#40536,#40537,#40538,#40539,#40540,#40541,#40542,
#40543,#40544));
#17213=EDGE_LOOP('',(#40545,#40546,#40547,#40548));
#17214=EDGE_LOOP('',(#40549,#40550,#40551,#40552));
#17215=EDGE_LOOP('',(#40553,#40554,#40555,#40556));
#17216=EDGE_LOOP('',(#40557,#40558,#40559,#40560));
#17217=EDGE_LOOP('',(#40561,#40562,#40563,#40564));
#17218=EDGE_LOOP('',(#40565,#40566,#40567,#40568));
#17219=EDGE_LOOP('',(#40569,#40570,#40571,#40572));
#17220=EDGE_LOOP('',(#40573,#40574,#40575,#40576));
#17221=EDGE_LOOP('',(#40577,#40578,#40579,#40580));
#17222=EDGE_LOOP('',(#40581,#40582,#40583,#40584));
#17223=EDGE_LOOP('',(#40585,#40586,#40587,#40588));
#17224=EDGE_LOOP('',(#40589,#40590,#40591,#40592));
#17225=EDGE_LOOP('',(#40593,#40594,#40595,#40596));
#17226=EDGE_LOOP('',(#40597,#40598,#40599,#40600,#40601,#40602,#40603));
#17227=EDGE_LOOP('',(#40604,#40605,#40606,#40607));
#17228=EDGE_LOOP('',(#40608,#40609,#40610,#40611));
#17229=EDGE_LOOP('',(#40612,#40613,#40614,#40615));
#17230=EDGE_LOOP('',(#40616,#40617,#40618,#40619));
#17231=EDGE_LOOP('',(#40620,#40621,#40622,#40623));
#17232=EDGE_LOOP('',(#40624,#40625,#40626,#40627));
#17233=EDGE_LOOP('',(#40628,#40629,#40630,#40631));
#17234=EDGE_LOOP('',(#40632,#40633,#40634,#40635));
#17235=EDGE_LOOP('',(#40636,#40637,#40638,#40639));
#17236=EDGE_LOOP('',(#40640,#40641,#40642,#40643));
#17237=EDGE_LOOP('',(#40644,#40645,#40646,#40647));
#17238=EDGE_LOOP('',(#40648,#40649,#40650,#40651));
#17239=EDGE_LOOP('',(#40652,#40653,#40654,#40655));
#17240=EDGE_LOOP('',(#40656,#40657,#40658,#40659));
#17241=EDGE_LOOP('',(#40660,#40661,#40662,#40663,#40664,#40665,#40666,#40667,
#40668,#40669,#40670,#40671,#40672,#40673,#40674,#40675,#40676,#40677,#40678,
#40679,#40680,#40681,#40682,#40683,#40684,#40685,#40686,#40687,#40688,#40689,
#40690,#40691));
#17242=EDGE_LOOP('',(#40692,#40693,#40694,#40695));
#17243=EDGE_LOOP('',(#40696,#40697,#40698,#40699));
#17244=EDGE_LOOP('',(#40700,#40701,#40702,#40703));
#17245=EDGE_LOOP('',(#40704,#40705,#40706,#40707));
#17246=EDGE_LOOP('',(#40708,#40709,#40710,#40711));
#17247=EDGE_LOOP('',(#40712,#40713,#40714,#40715));
#17248=EDGE_LOOP('',(#40716,#40717,#40718,#40719));
#17249=EDGE_LOOP('',(#40720,#40721,#40722,#40723));
#17250=EDGE_LOOP('',(#40724,#40725,#40726,#40727));
#17251=EDGE_LOOP('',(#40728,#40729,#40730,#40731));
#17252=EDGE_LOOP('',(#40732,#40733,#40734,#40735));
#17253=EDGE_LOOP('',(#40736,#40737,#40738,#40739));
#17254=EDGE_LOOP('',(#40740,#40741,#40742,#40743));
#17255=EDGE_LOOP('',(#40744,#40745,#40746,#40747,#40748,#40749,#40750));
#17256=EDGE_LOOP('',(#40751,#40752,#40753,#40754));
#17257=EDGE_LOOP('',(#40755,#40756,#40757,#40758));
#17258=EDGE_LOOP('',(#40759,#40760,#40761,#40762));
#17259=EDGE_LOOP('',(#40763,#40764,#40765,#40766));
#17260=EDGE_LOOP('',(#40767,#40768,#40769,#40770));
#17261=EDGE_LOOP('',(#40771,#40772,#40773,#40774));
#17262=EDGE_LOOP('',(#40775,#40776,#40777,#40778));
#17263=EDGE_LOOP('',(#40779,#40780,#40781,#40782));
#17264=EDGE_LOOP('',(#40783,#40784,#40785,#40786));
#17265=EDGE_LOOP('',(#40787,#40788,#40789,#40790));
#17266=EDGE_LOOP('',(#40791,#40792,#40793,#40794));
#17267=EDGE_LOOP('',(#40795,#40796,#40797,#40798));
#17268=EDGE_LOOP('',(#40799,#40800,#40801,#40802));
#17269=EDGE_LOOP('',(#40803,#40804,#40805,#40806));
#17270=EDGE_LOOP('',(#40807,#40808,#40809,#40810,#40811,#40812,#40813,#40814,
#40815,#40816,#40817,#40818,#40819,#40820,#40821,#40822,#40823,#40824,#40825,
#40826,#40827,#40828,#40829,#40830,#40831,#40832,#40833,#40834,#40835,#40836,
#40837,#40838));
#17271=EDGE_LOOP('',(#40839,#40840,#40841,#40842));
#17272=EDGE_LOOP('',(#40843,#40844,#40845,#40846));
#17273=EDGE_LOOP('',(#40847,#40848,#40849,#40850));
#17274=EDGE_LOOP('',(#40851,#40852,#40853,#40854));
#17275=EDGE_LOOP('',(#40855,#40856,#40857,#40858));
#17276=EDGE_LOOP('',(#40859,#40860,#40861,#40862));
#17277=EDGE_LOOP('',(#40863,#40864,#40865,#40866));
#17278=EDGE_LOOP('',(#40867,#40868,#40869,#40870));
#17279=EDGE_LOOP('',(#40871,#40872,#40873,#40874));
#17280=EDGE_LOOP('',(#40875,#40876,#40877,#40878));
#17281=EDGE_LOOP('',(#40879,#40880,#40881,#40882));
#17282=EDGE_LOOP('',(#40883,#40884,#40885,#40886));
#17283=EDGE_LOOP('',(#40887,#40888,#40889,#40890));
#17284=EDGE_LOOP('',(#40891,#40892,#40893,#40894,#40895,#40896,#40897));
#17285=EDGE_LOOP('',(#40898,#40899,#40900,#40901));
#17286=EDGE_LOOP('',(#40902,#40903,#40904,#40905));
#17287=EDGE_LOOP('',(#40906,#40907,#40908,#40909));
#17288=EDGE_LOOP('',(#40910,#40911,#40912,#40913));
#17289=EDGE_LOOP('',(#40914,#40915,#40916,#40917));
#17290=EDGE_LOOP('',(#40918,#40919,#40920,#40921));
#17291=EDGE_LOOP('',(#40922,#40923,#40924,#40925));
#17292=EDGE_LOOP('',(#40926,#40927,#40928,#40929));
#17293=EDGE_LOOP('',(#40930,#40931,#40932,#40933));
#17294=EDGE_LOOP('',(#40934,#40935,#40936,#40937));
#17295=EDGE_LOOP('',(#40938,#40939,#40940,#40941));
#17296=EDGE_LOOP('',(#40942,#40943,#40944,#40945));
#17297=EDGE_LOOP('',(#40946,#40947,#40948,#40949));
#17298=EDGE_LOOP('',(#40950,#40951,#40952,#40953,#40954,#40955,#40956));
#17299=EDGE_LOOP('',(#40957,#40958,#40959,#40960,#40961,#40962,#40963,#40964,
#40965,#40966,#40967,#40968,#40969,#40970,#40971,#40972,#40973,#40974,#40975,
#40976,#40977,#40978,#40979,#40980,#40981,#40982,#40983,#40984,#40985,#40986,
#40987,#40988,#40989,#40990,#40991,#40992,#40993,#40994,#40995,#40996,#40997,
#40998,#40999,#41000,#41001,#41002,#41003,#41004,#41005,#41006,#41007,#41008,
#41009,#41010,#41011,#41012,#41013,#41014,#41015,#41016,#41017,#41018,#41019,
#41020,#41021,#41022,#41023,#41024,#41025,#41026,#41027,#41028,#41029,#41030,
#41031,#41032,#41033,#41034,#41035,#41036,#41037,#41038,#41039,#41040,#41041,
#41042,#41043,#41044,#41045,#41046,#41047,#41048,#41049,#41050,#41051,#41052,
#41053,#41054,#41055,#41056,#41057,#41058,#41059,#41060,#41061,#41062,#41063,
#41064,#41065,#41066,#41067,#41068,#41069,#41070,#41071,#41072,#41073,#41074,
#41075,#41076,#41077,#41078,#41079,#41080,#41081,#41082,#41083,#41084,#41085,
#41086,#41087,#41088,#41089,#41090,#41091,#41092,#41093,#41094,#41095,#41096,
#41097,#41098,#41099,#41100,#41101,#41102,#41103,#41104));
#17300=EDGE_LOOP('',(#41105,#41106,#41107,#41108,#41109));
#17301=EDGE_LOOP('',(#41110,#41111,#41112,#41113,#41114,#41115));
#17302=EDGE_LOOP('',(#41116));
#17303=EDGE_LOOP('',(#41117));
#17304=EDGE_LOOP('',(#41118,#41119,#41120,#41121,#41122,#41123));
#17305=EDGE_LOOP('',(#41124,#41125,#41126,#41127,#41128));
#17306=EDGE_LOOP('',(#41129,#41130,#41131,#41132,#41133));
#17307=EDGE_LOOP('',(#41134,#41135,#41136,#41137,#41138,#41139));
#17308=EDGE_LOOP('',(#41140));
#17309=EDGE_LOOP('',(#41141));
#17310=EDGE_LOOP('',(#41142,#41143,#41144,#41145,#41146));
#17311=EDGE_LOOP('',(#41147));
#17312=EDGE_LOOP('',(#41148));
#17313=EDGE_LOOP('',(#41149,#41150,#41151,#41152,#41153,#41154,#41155,#41156,
#41157,#41158,#41159,#41160,#41161,#41162,#41163,#41164,#41165,#41166,#41167,
#41168,#41169,#41170,#41171,#41172,#41173,#41174,#41175,#41176,#41177,#41178,
#41179,#41180));
#17314=EDGE_LOOP('',(#41181));
#17315=EDGE_LOOP('',(#41182));
#17316=EDGE_LOOP('',(#41183,#41184,#41185,#41186));
#17317=EDGE_LOOP('',(#41187,#41188,#41189,#41190));
#17318=EDGE_LOOP('',(#41191,#41192,#41193,#41194));
#17319=EDGE_LOOP('',(#41195,#41196,#41197,#41198));
#17320=EDGE_LOOP('',(#41199,#41200,#41201,#41202));
#18698=(
BOUNDED_CURVE()
B_SPLINE_CURVE(2,(#68265,#68266,#68267),.UNSPECIFIED.,.F.,.F.)
B_SPLINE_CURVE_WITH_KNOTS((3,3),(0.0522192481407972,0.300149053231598),
 .UNSPECIFIED.)
CURVE()
GEOMETRIC_REPRESENTATION_ITEM()
RATIONAL_B_SPLINE_CURVE((1.00002415803342,1.00006942852605,1.))
REPRESENTATION_ITEM('')
);
#18699=(
BOUNDED_CURVE()
B_SPLINE_CURVE(2,(#68269,#68270,#68271),.UNSPECIFIED.,.F.,.F.)
B_SPLINE_CURVE_WITH_KNOTS((3,3),(0.98462316632217,1.26677639839307),
 .UNSPECIFIED.)
CURVE()
GEOMETRIC_REPRESENTATION_ITEM()
RATIONAL_B_SPLINE_CURVE((1.02072197947249,1.0213832836854,1.02072197947249))
REPRESENTATION_ITEM('')
);
#18700=(
BOUNDED_CURVE()
B_SPLINE_CURVE(2,(#68272,#68273,#68274),.UNSPECIFIED.,.F.,.F.)
B_SPLINE_CURVE_WITH_KNOTS((3,3),(0.,0.247929805090986),.UNSPECIFIED.)
CURVE()
GEOMETRIC_REPRESENTATION_ITEM()
RATIONAL_B_SPLINE_CURVE((1.,1.0000694285291,1.00002415803448))
REPRESENTATION_ITEM('')
);
#18701=(
BOUNDED_CURVE()
B_SPLINE_CURVE(2,(#68280,#68281,#68282),.UNSPECIFIED.,.F.,.F.)
B_SPLINE_CURVE_WITH_KNOTS((3,3),(0.0522192481407795,0.300149053231598),
 .UNSPECIFIED.)
CURVE()
GEOMETRIC_REPRESENTATION_ITEM()
RATIONAL_B_SPLINE_CURVE((1.00002415803391,1.00006942852745,1.))
REPRESENTATION_ITEM('')
);
#18702=(
BOUNDED_CURVE()
B_SPLINE_CURVE(2,(#68284,#68285,#68286),.UNSPECIFIED.,.F.,.F.)
B_SPLINE_CURVE_WITH_KNOTS((3,3),(0.984623166322172,1.26677639839308),
 .UNSPECIFIED.)
CURVE()
GEOMETRIC_REPRESENTATION_ITEM()
RATIONAL_B_SPLINE_CURVE((1.02072197947249,1.02138328368541,1.02072197947249))
REPRESENTATION_ITEM('')
);
#18703=(
BOUNDED_CURVE()
B_SPLINE_CURVE(2,(#68287,#68288,#68289),.UNSPECIFIED.,.F.,.F.)
B_SPLINE_CURVE_WITH_KNOTS((3,3),(0.,0.247929805090959),.UNSPECIFIED.)
CURVE()
GEOMETRIC_REPRESENTATION_ITEM()
RATIONAL_B_SPLINE_CURVE((1.,1.00006942853144,1.0000241580353))
REPRESENTATION_ITEM('')
);
#18704=(
BOUNDED_CURVE()
B_SPLINE_CURVE(2,(#68295,#68296,#68297),.UNSPECIFIED.,.F.,.F.)
B_SPLINE_CURVE_WITH_KNOTS((3,3),(0.0522192481406614,0.300149053231599),
 .UNSPECIFIED.)
CURVE()
GEOMETRIC_REPRESENTATION_ITEM()
RATIONAL_B_SPLINE_CURVE((1.00002415803474,1.00006942852983,1.))
REPRESENTATION_ITEM('')
);
#18705=(
BOUNDED_CURVE()
B_SPLINE_CURVE(2,(#68299,#68300,#68301),.UNSPECIFIED.,.F.,.F.)
B_SPLINE_CURVE_WITH_KNOTS((3,3),(0.984623166322172,1.26677639839307),
 .UNSPECIFIED.)
CURVE()
GEOMETRIC_REPRESENTATION_ITEM()
RATIONAL_B_SPLINE_CURVE((1.02072197947249,1.02138328368541,1.02072197947249))
REPRESENTATION_ITEM('')
);
#18706=(
BOUNDED_CURVE()
B_SPLINE_CURVE(2,(#68302,#68303,#68304),.UNSPECIFIED.,.F.,.F.)
B_SPLINE_CURVE_WITH_KNOTS((3,3),(0.,0.247929805090876),.UNSPECIFIED.)
CURVE()
GEOMETRIC_REPRESENTATION_ITEM()
RATIONAL_B_SPLINE_CURVE((1.,1.00006942852873,1.00002415803435))
REPRESENTATION_ITEM('')
);
#18707=(
BOUNDED_CURVE()
B_SPLINE_CURVE(2,(#68310,#68311,#68312),.UNSPECIFIED.,.F.,.F.)
B_SPLINE_CURVE_WITH_KNOTS((3,3),(0.0522192481406224,0.300149053231599),
 .UNSPECIFIED.)
CURVE()
GEOMETRIC_REPRESENTATION_ITEM()
RATIONAL_B_SPLINE_CURVE((1.00002415803453,1.00006942852923,1.))
REPRESENTATION_ITEM('')
);
#18708=(
BOUNDED_CURVE()
B_SPLINE_CURVE(2,(#68314,#68315,#68316),.UNSPECIFIED.,.F.,.F.)
B_SPLINE_CURVE_WITH_KNOTS((3,3),(0.984623166322173,1.26677639839308),
 .UNSPECIFIED.)
CURVE()
GEOMETRIC_REPRESENTATION_ITEM()
RATIONAL_B_SPLINE_CURVE((1.02072197947249,1.02138328368541,1.02072197947249))
REPRESENTATION_ITEM('')
);
#18709=(
BOUNDED_CURVE()
B_SPLINE_CURVE(2,(#68317,#68318,#68319),.UNSPECIFIED.,.F.,.F.)
B_SPLINE_CURVE_WITH_KNOTS((3,3),(0.,0.247929805090936),.UNSPECIFIED.)
CURVE()
GEOMETRIC_REPRESENTATION_ITEM()
RATIONAL_B_SPLINE_CURVE((1.,1.00006942853044,1.00002415803495))
REPRESENTATION_ITEM('')
);
#18710=(
BOUNDED_CURVE()
B_SPLINE_CURVE(2,(#68325,#68326,#68327),.UNSPECIFIED.,.F.,.F.)
B_SPLINE_CURVE_WITH_KNOTS((3,3),(0.0522192481406471,0.300149053231599),
 .UNSPECIFIED.)
CURVE()
GEOMETRIC_REPRESENTATION_ITEM()
RATIONAL_B_SPLINE_CURVE((1.00002415803429,1.00006942852855,1.))
REPRESENTATION_ITEM('')
);
#18711=(
BOUNDED_CURVE()
B_SPLINE_CURVE(2,(#68329,#68330,#68331),.UNSPECIFIED.,.F.,.F.)
B_SPLINE_CURVE_WITH_KNOTS((3,3),(0.98462316632217,1.26677639839307),
 .UNSPECIFIED.)
CURVE()
GEOMETRIC_REPRESENTATION_ITEM()
RATIONAL_B_SPLINE_CURVE((1.02072197947249,1.02138328368541,1.02072197947249))
REPRESENTATION_ITEM('')
);
#18712=(
BOUNDED_CURVE()
B_SPLINE_CURVE(2,(#68332,#68333,#68334),.UNSPECIFIED.,.F.,.F.)
B_SPLINE_CURVE_WITH_KNOTS((3,3),(0.,0.247929805090895),.UNSPECIFIED.)
CURVE()
GEOMETRIC_REPRESENTATION_ITEM()
RATIONAL_B_SPLINE_CURVE((1.,1.000069428528,1.0000241580341))
REPRESENTATION_ITEM('')
);
#18713=(
BOUNDED_CURVE()
B_SPLINE_CURVE(2,(#68340,#68341,#68342),.UNSPECIFIED.,.F.,.F.)
B_SPLINE_CURVE_WITH_KNOTS((3,3),(0.0522192481406872,0.300149053231598),
 .UNSPECIFIED.)
CURVE()
GEOMETRIC_REPRESENTATION_ITEM()
RATIONAL_B_SPLINE_CURVE((1.00002415803456,1.00006942852931,1.))
REPRESENTATION_ITEM('')
);
#18714=(
BOUNDED_CURVE()
B_SPLINE_CURVE(2,(#68344,#68345,#68346),.UNSPECIFIED.,.F.,.F.)
B_SPLINE_CURVE_WITH_KNOTS((3,3),(0.984623166322171,1.26677639839307),
 .UNSPECIFIED.)
CURVE()
GEOMETRIC_REPRESENTATION_ITEM()
RATIONAL_B_SPLINE_CURVE((1.02072197947249,1.02138328368541,1.02072197947249))
REPRESENTATION_ITEM('')
);
#18715=(
BOUNDED_CURVE()
B_SPLINE_CURVE(2,(#68347,#68348,#68349),.UNSPECIFIED.,.F.,.F.)
B_SPLINE_CURVE_WITH_KNOTS((3,3),(0.,0.247929805090952),.UNSPECIFIED.)
CURVE()
GEOMETRIC_REPRESENTATION_ITEM()
RATIONAL_B_SPLINE_CURVE((1.,1.00006942852864,1.00002415803432))
REPRESENTATION_ITEM('')
);
#18716=(
BOUNDED_CURVE()
B_SPLINE_CURVE(2,(#68355,#68356,#68357),.UNSPECIFIED.,.F.,.F.)
B_SPLINE_CURVE_WITH_KNOTS((3,3),(0.0522192481406724,0.300149053231598),
 .UNSPECIFIED.)
CURVE()
GEOMETRIC_REPRESENTATION_ITEM()
RATIONAL_B_SPLINE_CURVE((1.00002415803439,1.00006942852885,1.))
REPRESENTATION_ITEM('')
);
#18717=(
BOUNDED_CURVE()
B_SPLINE_CURVE(2,(#68359,#68360,#68361),.UNSPECIFIED.,.F.,.F.)
B_SPLINE_CURVE_WITH_KNOTS((3,3),(0.984623166322169,1.26677639839307),
 .UNSPECIFIED.)
CURVE()
GEOMETRIC_REPRESENTATION_ITEM()
RATIONAL_B_SPLINE_CURVE((1.02072197947249,1.02138328368541,1.02072197947249))
REPRESENTATION_ITEM('')
);
#18718=(
BOUNDED_CURVE()
B_SPLINE_CURVE(2,(#68362,#68363,#68364),.UNSPECIFIED.,.F.,.F.)
B_SPLINE_CURVE_WITH_KNOTS((3,3),(0.,0.24792980509092),.UNSPECIFIED.)
CURVE()
GEOMETRIC_REPRESENTATION_ITEM()
RATIONAL_B_SPLINE_CURVE((1.,1.0000694285281,1.00002415803414))
REPRESENTATION_ITEM('')
);
#18719=(
BOUNDED_CURVE()
B_SPLINE_CURVE(2,(#68370,#68371,#68372),.UNSPECIFIED.,.F.,.F.)
B_SPLINE_CURVE_WITH_KNOTS((3,3),(0.0522192481407194,0.300149053231599),
 .UNSPECIFIED.)
CURVE()
GEOMETRIC_REPRESENTATION_ITEM()
RATIONAL_B_SPLINE_CURVE((1.00002415803445,1.00006942852901,1.))
REPRESENTATION_ITEM('')
);
#18720=(
BOUNDED_CURVE()
B_SPLINE_CURVE(2,(#68374,#68375,#68376),.UNSPECIFIED.,.F.,.F.)
B_SPLINE_CURVE_WITH_KNOTS((3,3),(0.984623166322171,1.26677639839307),
 .UNSPECIFIED.)
CURVE()
GEOMETRIC_REPRESENTATION_ITEM()
RATIONAL_B_SPLINE_CURVE((1.02072197947249,1.02138328368541,1.02072197947249))
REPRESENTATION_ITEM('')
);
#18721=(
BOUNDED_CURVE()
B_SPLINE_CURVE(2,(#68377,#68378,#68379),.UNSPECIFIED.,.F.,.F.)
B_SPLINE_CURVE_WITH_KNOTS((3,3),(0.,0.247929805090845),.UNSPECIFIED.)
CURVE()
GEOMETRIC_REPRESENTATION_ITEM()
RATIONAL_B_SPLINE_CURVE((1.,1.00006942852734,1.00002415803387))
REPRESENTATION_ITEM('')
);
#18722=(
BOUNDED_CURVE()
B_SPLINE_CURVE(2,(#68385,#68386,#68387),.UNSPECIFIED.,.F.,.F.)
B_SPLINE_CURVE_WITH_KNOTS((3,3),(0.0522192481406634,0.300149053231598),
 .UNSPECIFIED.)
CURVE()
GEOMETRIC_REPRESENTATION_ITEM()
RATIONAL_B_SPLINE_CURVE((1.00002415803422,1.00006942852834,1.))
REPRESENTATION_ITEM('')
);
#18723=(
BOUNDED_CURVE()
B_SPLINE_CURVE(2,(#68389,#68390,#68391),.UNSPECIFIED.,.F.,.F.)
B_SPLINE_CURVE_WITH_KNOTS((3,3),(0.984623166322172,1.26677639839307),
 .UNSPECIFIED.)
CURVE()
GEOMETRIC_REPRESENTATION_ITEM()
RATIONAL_B_SPLINE_CURVE((1.02072197947249,1.02138328368541,1.02072197947249))
REPRESENTATION_ITEM('')
);
#18724=(
BOUNDED_CURVE()
B_SPLINE_CURVE(2,(#68392,#68393,#68394),.UNSPECIFIED.,.F.,.F.)
B_SPLINE_CURVE_WITH_KNOTS((3,3),(0.,0.247929805090971),.UNSPECIFIED.)
CURVE()
GEOMETRIC_REPRESENTATION_ITEM()
RATIONAL_B_SPLINE_CURVE((1.,1.0000694285305,1.00002415803497))
REPRESENTATION_ITEM('')
);
#18725=(
BOUNDED_CURVE()
B_SPLINE_CURVE(2,(#68400,#68401,#68402),.UNSPECIFIED.,.F.,.F.)
B_SPLINE_CURVE_WITH_KNOTS((3,3),(0.052219248140715,0.300149053231599),
 .UNSPECIFIED.)
CURVE()
GEOMETRIC_REPRESENTATION_ITEM()
RATIONAL_B_SPLINE_CURVE((1.00002415803427,1.00006942852848,1.))
REPRESENTATION_ITEM('')
);
#18726=(
BOUNDED_CURVE()
B_SPLINE_CURVE(2,(#68404,#68405,#68406),.UNSPECIFIED.,.F.,.F.)
B_SPLINE_CURVE_WITH_KNOTS((3,3),(0.98462316632217,1.26677639839307),
 .UNSPECIFIED.)
CURVE()
GEOMETRIC_REPRESENTATION_ITEM()
RATIONAL_B_SPLINE_CURVE((1.02072197947249,1.0213832836854,1.02072197947249))
REPRESENTATION_ITEM('')
);
#18727=(
BOUNDED_CURVE()
B_SPLINE_CURVE(2,(#68407,#68408,#68409),.UNSPECIFIED.,.F.,.F.)
B_SPLINE_CURVE_WITH_KNOTS((3,3),(0.,0.247929805090914),.UNSPECIFIED.)
CURVE()
GEOMETRIC_REPRESENTATION_ITEM()
RATIONAL_B_SPLINE_CURVE((1.,1.00006942852705,1.00002415803377))
REPRESENTATION_ITEM('')
);
#18728=(
BOUNDED_CURVE()
B_SPLINE_CURVE(2,(#68415,#68416,#68417),.UNSPECIFIED.,.F.,.F.)
B_SPLINE_CURVE_WITH_KNOTS((3,3),(0.0522192481406779,0.300149053231598),
 .UNSPECIFIED.)
CURVE()
GEOMETRIC_REPRESENTATION_ITEM()
RATIONAL_B_SPLINE_CURVE((1.00002415803406,1.0000694285279,1.))
REPRESENTATION_ITEM('')
);
#18729=(
BOUNDED_CURVE()
B_SPLINE_CURVE(2,(#68419,#68420,#68421),.UNSPECIFIED.,.F.,.F.)
B_SPLINE_CURVE_WITH_KNOTS((3,3),(0.984623166322172,1.26677639839307),
 .UNSPECIFIED.)
CURVE()
GEOMETRIC_REPRESENTATION_ITEM()
RATIONAL_B_SPLINE_CURVE((1.02072197947249,1.02138328368541,1.02072197947249))
REPRESENTATION_ITEM('')
);
#18730=(
BOUNDED_CURVE()
B_SPLINE_CURVE(2,(#68422,#68423,#68424),.UNSPECIFIED.,.F.,.F.)
B_SPLINE_CURVE_WITH_KNOTS((3,3),(0.,0.247929805090857),.UNSPECIFIED.)
CURVE()
GEOMETRIC_REPRESENTATION_ITEM()
RATIONAL_B_SPLINE_CURVE((1.,1.00006942852857,1.0000241580343))
REPRESENTATION_ITEM('')
);
#18731=(
BOUNDED_CURVE()
B_SPLINE_CURVE(2,(#68430,#68431,#68432),.UNSPECIFIED.,.F.,.F.)
B_SPLINE_CURVE_WITH_KNOTS((3,3),(0.0522192481406934,0.300149053231599),
 .UNSPECIFIED.)
CURVE()
GEOMETRIC_REPRESENTATION_ITEM()
RATIONAL_B_SPLINE_CURVE((1.00002415803403,1.00006942852779,1.))
REPRESENTATION_ITEM('')
);
#18732=(
BOUNDED_CURVE()
B_SPLINE_CURVE(2,(#68434,#68435,#68436),.UNSPECIFIED.,.F.,.F.)
B_SPLINE_CURVE_WITH_KNOTS((3,3),(0.984623166322171,1.26677639839307),
 .UNSPECIFIED.)
CURVE()
GEOMETRIC_REPRESENTATION_ITEM()
RATIONAL_B_SPLINE_CURVE((1.02072197947249,1.02138328368541,1.02072197947249))
REPRESENTATION_ITEM('')
);
#18733=(
BOUNDED_CURVE()
B_SPLINE_CURVE(2,(#68437,#68438,#68439),.UNSPECIFIED.,.F.,.F.)
B_SPLINE_CURVE_WITH_KNOTS((3,3),(0.,0.247929805090923),.UNSPECIFIED.)
CURVE()
GEOMETRIC_REPRESENTATION_ITEM()
RATIONAL_B_SPLINE_CURVE((1.,1.00006942853014,1.00002415803484))
REPRESENTATION_ITEM('')
);
#18734=(
BOUNDED_CURVE()
B_SPLINE_CURVE(2,(#68445,#68446,#68447),.UNSPECIFIED.,.F.,.F.)
B_SPLINE_CURVE_WITH_KNOTS((3,3),(0.0522192481406993,0.300149053231599),
 .UNSPECIFIED.)
CURVE()
GEOMETRIC_REPRESENTATION_ITEM()
RATIONAL_B_SPLINE_CURVE((1.0000241580339,1.00006942852741,1.))
REPRESENTATION_ITEM('')
);
#18735=(
BOUNDED_CURVE()
B_SPLINE_CURVE(2,(#68449,#68450,#68451),.UNSPECIFIED.,.F.,.F.)
B_SPLINE_CURVE_WITH_KNOTS((3,3),(0.984623166322172,1.26677639839308),
 .UNSPECIFIED.)
CURVE()
GEOMETRIC_REPRESENTATION_ITEM()
RATIONAL_B_SPLINE_CURVE((1.02072197947249,1.02138328368541,1.02072197947249))
REPRESENTATION_ITEM('')
);
#18736=(
BOUNDED_CURVE()
B_SPLINE_CURVE(2,(#68452,#68453,#68454),.UNSPECIFIED.,.F.,.F.)
B_SPLINE_CURVE_WITH_KNOTS((3,3),(0.,0.247929805090912),.UNSPECIFIED.)
CURVE()
GEOMETRIC_REPRESENTATION_ITEM()
RATIONAL_B_SPLINE_CURVE((1.,1.00006942852758,1.00002415803395))
REPRESENTATION_ITEM('')
);
#18737=(
BOUNDED_CURVE()
B_SPLINE_CURVE(2,(#68460,#68461,#68462),.UNSPECIFIED.,.F.,.F.)
B_SPLINE_CURVE_WITH_KNOTS((3,3),(0.0522192481406619,0.300149053231598),
 .UNSPECIFIED.)
CURVE()
GEOMETRIC_REPRESENTATION_ITEM()
RATIONAL_B_SPLINE_CURVE((1.00002415803529,1.00006942853141,1.))
REPRESENTATION_ITEM('')
);
#18738=(
BOUNDED_CURVE()
B_SPLINE_CURVE(2,(#68464,#68465,#68466),.UNSPECIFIED.,.F.,.F.)
B_SPLINE_CURVE_WITH_KNOTS((3,3),(0.984623166322169,1.26677639839307),
 .UNSPECIFIED.)
CURVE()
GEOMETRIC_REPRESENTATION_ITEM()
RATIONAL_B_SPLINE_CURVE((1.02072197947249,1.02138328368541,1.02072197947249))
REPRESENTATION_ITEM('')
);
#18739=(
BOUNDED_CURVE()
B_SPLINE_CURVE(2,(#68467,#68468,#68469),.UNSPECIFIED.,.F.,.F.)
B_SPLINE_CURVE_WITH_KNOTS((3,3),(0.,0.247929805090904),.UNSPECIFIED.)
CURVE()
GEOMETRIC_REPRESENTATION_ITEM()
RATIONAL_B_SPLINE_CURVE((1.,1.00006942852951,1.00002415803463))
REPRESENTATION_ITEM('')
);
#18740=(
BOUNDED_CURVE()
B_SPLINE_CURVE(2,(#68475,#68476,#68477),.UNSPECIFIED.,.F.,.F.)
B_SPLINE_CURVE_WITH_KNOTS((3,3),(0.0522192481406167,0.300149053231598),
 .UNSPECIFIED.)
CURVE()
GEOMETRIC_REPRESENTATION_ITEM()
RATIONAL_B_SPLINE_CURVE((1.0000241580343,1.00006942852858,1.))
REPRESENTATION_ITEM('')
);
#18741=(
BOUNDED_CURVE()
B_SPLINE_CURVE(2,(#68479,#68480,#68481),.UNSPECIFIED.,.F.,.F.)
B_SPLINE_CURVE_WITH_KNOTS((3,3),(0.984623166322174,1.26677639839308),
 .UNSPECIFIED.)
CURVE()
GEOMETRIC_REPRESENTATION_ITEM()
RATIONAL_B_SPLINE_CURVE((1.02072197947249,1.02138328368541,1.02072197947249))
REPRESENTATION_ITEM('')
);
#18742=(
BOUNDED_CURVE()
B_SPLINE_CURVE(2,(#68482,#68483,#68484),.UNSPECIFIED.,.F.,.F.)
B_SPLINE_CURVE_WITH_KNOTS((3,3),(0.,0.247929805090943),.UNSPECIFIED.)
CURVE()
GEOMETRIC_REPRESENTATION_ITEM()
RATIONAL_B_SPLINE_CURVE((1.,1.0000694285289,1.00002415803441))
REPRESENTATION_ITEM('')
);
#18743=(
BOUNDED_CURVE()
B_SPLINE_CURVE(2,(#68490,#68491,#68492),.UNSPECIFIED.,.F.,.F.)
B_SPLINE_CURVE_WITH_KNOTS((3,3),(0.0522192481406359,0.300149053231599),
 .UNSPECIFIED.)
CURVE()
GEOMETRIC_REPRESENTATION_ITEM()
RATIONAL_B_SPLINE_CURVE((1.00002415803477,1.00006942852992,1.))
REPRESENTATION_ITEM('')
);
#18744=(
BOUNDED_CURVE()
B_SPLINE_CURVE(2,(#68494,#68495,#68496),.UNSPECIFIED.,.F.,.F.)
B_SPLINE_CURVE_WITH_KNOTS((3,3),(0.984623166322174,1.26677639839308),
 .UNSPECIFIED.)
CURVE()
GEOMETRIC_REPRESENTATION_ITEM()
RATIONAL_B_SPLINE_CURVE((1.02072197947249,1.0213832836854,1.02072197947249))
REPRESENTATION_ITEM('')
);
#18745=(
BOUNDED_CURVE()
B_SPLINE_CURVE(2,(#68497,#68498,#68499),.UNSPECIFIED.,.F.,.F.)
B_SPLINE_CURVE_WITH_KNOTS((3,3),(0.,0.247929805090921),.UNSPECIFIED.)
CURVE()
GEOMETRIC_REPRESENTATION_ITEM()
RATIONAL_B_SPLINE_CURVE((1.,1.00006942852933,1.00002415803456))
REPRESENTATION_ITEM('')
);
#18746=(
BOUNDED_CURVE()
B_SPLINE_CURVE(2,(#68505,#68506,#68507),.UNSPECIFIED.,.F.,.F.)
B_SPLINE_CURVE_WITH_KNOTS((3,3),(0.052219248140584,0.300149053231599),
 .UNSPECIFIED.)
CURVE()
GEOMETRIC_REPRESENTATION_ITEM()
RATIONAL_B_SPLINE_CURVE((1.00002415803526,1.00006942853134,1.))
REPRESENTATION_ITEM('')
);
#18747=(
BOUNDED_CURVE()
B_SPLINE_CURVE(2,(#68509,#68510,#68511),.UNSPECIFIED.,.F.,.F.)
B_SPLINE_CURVE_WITH_KNOTS((3,3),(0.984623166322171,1.26677639839308),
 .UNSPECIFIED.)
CURVE()
GEOMETRIC_REPRESENTATION_ITEM()
RATIONAL_B_SPLINE_CURVE((1.02072197947249,1.02138328368541,1.02072197947249))
REPRESENTATION_ITEM('')
);
#18748=(
BOUNDED_CURVE()
B_SPLINE_CURVE(2,(#68512,#68513,#68514),.UNSPECIFIED.,.F.,.F.)
B_SPLINE_CURVE_WITH_KNOTS((3,3),(0.,0.247929805090749),.UNSPECIFIED.)
CURVE()
GEOMETRIC_REPRESENTATION_ITEM()
RATIONAL_B_SPLINE_CURVE((1.,1.0000694285275,1.00002415803393))
REPRESENTATION_ITEM('')
);
#18749=(
BOUNDED_CURVE()
B_SPLINE_CURVE(2,(#68520,#68521,#68522),.UNSPECIFIED.,.F.,.F.)
B_SPLINE_CURVE_WITH_KNOTS((3,3),(0.0522192481406365,0.300149053231598),
 .UNSPECIFIED.)
CURVE()
GEOMETRIC_REPRESENTATION_ITEM()
RATIONAL_B_SPLINE_CURVE((1.00002415803451,1.00006942852916,1.))
REPRESENTATION_ITEM('')
);
#18750=(
BOUNDED_CURVE()
B_SPLINE_CURVE(2,(#68524,#68525,#68526),.UNSPECIFIED.,.F.,.F.)
B_SPLINE_CURVE_WITH_KNOTS((3,3),(0.984623166322172,1.26677639839307),
 .UNSPECIFIED.)
CURVE()
GEOMETRIC_REPRESENTATION_ITEM()
RATIONAL_B_SPLINE_CURVE((1.02072197947249,1.02138328368541,1.02072197947249))
REPRESENTATION_ITEM('')
);
#18751=(
BOUNDED_CURVE()
B_SPLINE_CURVE(2,(#68527,#68528,#68529),.UNSPECIFIED.,.F.,.F.)
B_SPLINE_CURVE_WITH_KNOTS((3,3),(0.,0.247929805090921),.UNSPECIFIED.)
CURVE()
GEOMETRIC_REPRESENTATION_ITEM()
RATIONAL_B_SPLINE_CURVE((1.,1.00006942852834,1.00002415803422))
REPRESENTATION_ITEM('')
);
#18752=(
BOUNDED_CURVE()
B_SPLINE_CURVE(2,(#68535,#68536,#68537),.UNSPECIFIED.,.F.,.F.)
B_SPLINE_CURVE_WITH_KNOTS((3,3),(0.0522192481407573,0.300149053231598),
 .UNSPECIFIED.)
CURVE()
GEOMETRIC_REPRESENTATION_ITEM()
RATIONAL_B_SPLINE_CURVE((1.00002415803426,1.00006942852846,1.))
REPRESENTATION_ITEM('')
);
#18753=(
BOUNDED_CURVE()
B_SPLINE_CURVE(2,(#68539,#68540,#68541),.UNSPECIFIED.,.F.,.F.)
B_SPLINE_CURVE_WITH_KNOTS((3,3),(0.984623166322171,1.26677639839307),
 .UNSPECIFIED.)
CURVE()
GEOMETRIC_REPRESENTATION_ITEM()
RATIONAL_B_SPLINE_CURVE((1.02072197947249,1.0213832836854,1.02072197947249))
REPRESENTATION_ITEM('')
);
#18754=(
BOUNDED_CURVE()
B_SPLINE_CURVE(2,(#68542,#68543,#68544),.UNSPECIFIED.,.F.,.F.)
B_SPLINE_CURVE_WITH_KNOTS((3,3),(0.,0.247929805091041),.UNSPECIFIED.)
CURVE()
GEOMETRIC_REPRESENTATION_ITEM()
RATIONAL_B_SPLINE_CURVE((1.,1.0000694285297,1.00002415803469))
REPRESENTATION_ITEM('')
);
#18755=(
BOUNDED_CURVE()
B_SPLINE_CURVE(2,(#68550,#68551,#68552),.UNSPECIFIED.,.F.,.F.)
B_SPLINE_CURVE_WITH_KNOTS((3,3),(0.0522192481406059,0.300149053231598),
 .UNSPECIFIED.)
CURVE()
GEOMETRIC_REPRESENTATION_ITEM()
RATIONAL_B_SPLINE_CURVE((1.00002415803507,1.00006942853079,1.))
REPRESENTATION_ITEM('')
);
#18756=(
BOUNDED_CURVE()
B_SPLINE_CURVE(2,(#68554,#68555,#68556),.UNSPECIFIED.,.F.,.F.)
B_SPLINE_CURVE_WITH_KNOTS((3,3),(0.984623166322169,1.26677639839307),
 .UNSPECIFIED.)
CURVE()
GEOMETRIC_REPRESENTATION_ITEM()
RATIONAL_B_SPLINE_CURVE((1.02072197947249,1.02138328368541,1.02072197947249))
REPRESENTATION_ITEM('')
);
#18757=(
BOUNDED_CURVE()
B_SPLINE_CURVE(2,(#68557,#68558,#68559),.UNSPECIFIED.,.F.,.F.)
B_SPLINE_CURVE_WITH_KNOTS((3,3),(0.,0.247929805090961),.UNSPECIFIED.)
CURVE()
GEOMETRIC_REPRESENTATION_ITEM()
RATIONAL_B_SPLINE_CURVE((1.,1.00006942852846,1.00002415803426))
REPRESENTATION_ITEM('')
);
#18758=(
BOUNDED_CURVE()
B_SPLINE_CURVE(2,(#68565,#68566,#68567),.UNSPECIFIED.,.F.,.F.)
B_SPLINE_CURVE_WITH_KNOTS((3,3),(0.0522192481407161,0.300149053231599),
 .UNSPECIFIED.)
CURVE()
GEOMETRIC_REPRESENTATION_ITEM()
RATIONAL_B_SPLINE_CURVE((1.00002415803387,1.00006942852735,1.))
REPRESENTATION_ITEM('')
);
#18759=(
BOUNDED_CURVE()
B_SPLINE_CURVE(2,(#68569,#68570,#68571),.UNSPECIFIED.,.F.,.F.)
B_SPLINE_CURVE_WITH_KNOTS((3,3),(0.984623166322171,1.26677639839307),
 .UNSPECIFIED.)
CURVE()
GEOMETRIC_REPRESENTATION_ITEM()
RATIONAL_B_SPLINE_CURVE((1.02072197947249,1.02138328368541,1.02072197947249))
REPRESENTATION_ITEM('')
);
#18760=(
BOUNDED_CURVE()
B_SPLINE_CURVE(2,(#68572,#68573,#68574),.UNSPECIFIED.,.F.,.F.)
B_SPLINE_CURVE_WITH_KNOTS((3,3),(0.,0.247929805090882),.UNSPECIFIED.)
CURVE()
GEOMETRIC_REPRESENTATION_ITEM()
RATIONAL_B_SPLINE_CURVE((1.,1.00006942852857,1.0000241580343))
REPRESENTATION_ITEM('')
);
#18761=(
BOUNDED_CURVE()
B_SPLINE_CURVE(2,(#68580,#68581,#68582),.UNSPECIFIED.,.F.,.F.)
B_SPLINE_CURVE_WITH_KNOTS((3,3),(0.0522192481406709,0.300149053231599),
 .UNSPECIFIED.)
CURVE()
GEOMETRIC_REPRESENTATION_ITEM()
RATIONAL_B_SPLINE_CURVE((1.00002415803448,1.0000694285291,1.))
REPRESENTATION_ITEM('')
);
#18762=(
BOUNDED_CURVE()
B_SPLINE_CURVE(2,(#68584,#68585,#68586),.UNSPECIFIED.,.F.,.F.)
B_SPLINE_CURVE_WITH_KNOTS((3,3),(0.984623166322173,1.26677639839308),
 .UNSPECIFIED.)
CURVE()
GEOMETRIC_REPRESENTATION_ITEM()
RATIONAL_B_SPLINE_CURVE((1.02072197947249,1.02138328368541,1.02072197947249))
REPRESENTATION_ITEM('')
);
#18763=(
BOUNDED_CURVE()
B_SPLINE_CURVE(2,(#68587,#68588,#68589),.UNSPECIFIED.,.F.,.F.)
B_SPLINE_CURVE_WITH_KNOTS((3,3),(0.,0.247929805090867),.UNSPECIFIED.)
CURVE()
GEOMETRIC_REPRESENTATION_ITEM()
RATIONAL_B_SPLINE_CURVE((1.,1.00006942852627,1.0000241580335))
REPRESENTATION_ITEM('')
);
#18764=(
BOUNDED_CURVE()
B_SPLINE_CURVE(2,(#68595,#68596,#68597),.UNSPECIFIED.,.F.,.F.)
B_SPLINE_CURVE_WITH_KNOTS((3,3),(0.0522192481406783,0.300149053231598),
 .UNSPECIFIED.)
CURVE()
GEOMETRIC_REPRESENTATION_ITEM()
RATIONAL_B_SPLINE_CURVE((1.00002415803455,1.00006942852929,1.))
REPRESENTATION_ITEM('')
);
#18765=(
BOUNDED_CURVE()
B_SPLINE_CURVE(2,(#68599,#68600,#68601),.UNSPECIFIED.,.F.,.F.)
B_SPLINE_CURVE_WITH_KNOTS((3,3),(0.984623166322171,1.26677639839307),
 .UNSPECIFIED.)
CURVE()
GEOMETRIC_REPRESENTATION_ITEM()
RATIONAL_B_SPLINE_CURVE((1.02072197947249,1.02138328368541,1.02072197947249))
REPRESENTATION_ITEM('')
);
#18766=(
BOUNDED_CURVE()
B_SPLINE_CURVE(2,(#68602,#68603,#68604),.UNSPECIFIED.,.F.,.F.)
B_SPLINE_CURVE_WITH_KNOTS((3,3),(0.,0.247929805090952),.UNSPECIFIED.)
CURVE()
GEOMETRIC_REPRESENTATION_ITEM()
RATIONAL_B_SPLINE_CURVE((1.,1.00006942852834,1.00002415803422))
REPRESENTATION_ITEM('')
);
#18767=(
BOUNDED_CURVE()
B_SPLINE_CURVE(2,(#68610,#68611,#68612),.UNSPECIFIED.,.F.,.F.)
B_SPLINE_CURVE_WITH_KNOTS((3,3),(0.052219248140653,0.300149053231598),
 .UNSPECIFIED.)
CURVE()
GEOMETRIC_REPRESENTATION_ITEM()
RATIONAL_B_SPLINE_CURVE((1.00002415803398,1.00006942852765,1.))
REPRESENTATION_ITEM('')
);
#18768=(
BOUNDED_CURVE()
B_SPLINE_CURVE(2,(#68614,#68615,#68616),.UNSPECIFIED.,.F.,.F.)
B_SPLINE_CURVE_WITH_KNOTS((3,3),(0.984623166322171,1.26677639839307),
 .UNSPECIFIED.)
CURVE()
GEOMETRIC_REPRESENTATION_ITEM()
RATIONAL_B_SPLINE_CURVE((1.02072197947248,1.0213832836854,1.02072197947248))
REPRESENTATION_ITEM('')
);
#18769=(
BOUNDED_CURVE()
B_SPLINE_CURVE(2,(#68617,#68618,#68619),.UNSPECIFIED.,.F.,.F.)
B_SPLINE_CURVE_WITH_KNOTS((3,3),(0.,0.24792980509099),.UNSPECIFIED.)
CURVE()
GEOMETRIC_REPRESENTATION_ITEM()
RATIONAL_B_SPLINE_CURVE((1.,1.00006942852938,1.00002415803458))
REPRESENTATION_ITEM('')
);
#18770=(
BOUNDED_CURVE()
B_SPLINE_CURVE(2,(#68625,#68626,#68627),.UNSPECIFIED.,.F.,.F.)
B_SPLINE_CURVE_WITH_KNOTS((3,3),(0.0522192481406856,0.300149053231599),
 .UNSPECIFIED.)
CURVE()
GEOMETRIC_REPRESENTATION_ITEM()
RATIONAL_B_SPLINE_CURVE((1.00002415803379,1.00006942852711,1.))
REPRESENTATION_ITEM('')
);
#18771=(
BOUNDED_CURVE()
B_SPLINE_CURVE(2,(#68629,#68630,#68631),.UNSPECIFIED.,.F.,.F.)
B_SPLINE_CURVE_WITH_KNOTS((3,3),(0.984623166322173,1.26677639839307),
 .UNSPECIFIED.)
CURVE()
GEOMETRIC_REPRESENTATION_ITEM()
RATIONAL_B_SPLINE_CURVE((1.02072197947249,1.02138328368541,1.02072197947249))
REPRESENTATION_ITEM('')
);
#18772=(
BOUNDED_CURVE()
B_SPLINE_CURVE(2,(#68632,#68633,#68634),.UNSPECIFIED.,.F.,.F.)
B_SPLINE_CURVE_WITH_KNOTS((3,3),(0.,0.247929805090904),.UNSPECIFIED.)
CURVE()
GEOMETRIC_REPRESENTATION_ITEM()
RATIONAL_B_SPLINE_CURVE((1.,1.00006942852969,1.00002415803469))
REPRESENTATION_ITEM('')
);
#18773=(
BOUNDED_CURVE()
B_SPLINE_CURVE(2,(#68640,#68641,#68642),.UNSPECIFIED.,.F.,.F.)
B_SPLINE_CURVE_WITH_KNOTS((3,3),(0.0522192481406978,0.300149053231598),
 .UNSPECIFIED.)
CURVE()
GEOMETRIC_REPRESENTATION_ITEM()
RATIONAL_B_SPLINE_CURVE((1.00002415803478,1.00006942852994,1.))
REPRESENTATION_ITEM('')
);
#18774=(
BOUNDED_CURVE()
B_SPLINE_CURVE(2,(#68644,#68645,#68646),.UNSPECIFIED.,.F.,.F.)
B_SPLINE_CURVE_WITH_KNOTS((3,3),(0.984623166322171,1.26677639839307),
 .UNSPECIFIED.)
CURVE()
GEOMETRIC_REPRESENTATION_ITEM()
RATIONAL_B_SPLINE_CURVE((1.02072197947249,1.02138328368541,1.02072197947249))
REPRESENTATION_ITEM('')
);
#18775=(
BOUNDED_CURVE()
B_SPLINE_CURVE(2,(#68647,#68648,#68649),.UNSPECIFIED.,.F.,.F.)
B_SPLINE_CURVE_WITH_KNOTS((3,3),(0.,0.247929805090887),.UNSPECIFIED.)
CURVE()
GEOMETRIC_REPRESENTATION_ITEM()
RATIONAL_B_SPLINE_CURVE((1.,1.00006942852981,1.00002415803473))
REPRESENTATION_ITEM('')
);
#18776=(
BOUNDED_CURVE()
B_SPLINE_CURVE(2,(#68655,#68656,#68657),.UNSPECIFIED.,.F.,.F.)
B_SPLINE_CURVE_WITH_KNOTS((3,3),(0.0522192481406133,0.300149053231598),
 .UNSPECIFIED.)
CURVE()
GEOMETRIC_REPRESENTATION_ITEM()
RATIONAL_B_SPLINE_CURVE((1.00002415803473,1.00006942852981,1.))
REPRESENTATION_ITEM('')
);
#18777=(
BOUNDED_CURVE()
B_SPLINE_CURVE(2,(#68659,#68660,#68661),.UNSPECIFIED.,.F.,.F.)
B_SPLINE_CURVE_WITH_KNOTS((3,3),(0.984623166322172,1.26677639839307),
 .UNSPECIFIED.)
CURVE()
GEOMETRIC_REPRESENTATION_ITEM()
RATIONAL_B_SPLINE_CURVE((1.02072197947249,1.02138328368541,1.02072197947249))
REPRESENTATION_ITEM('')
);
#18778=(
BOUNDED_CURVE()
B_SPLINE_CURVE(2,(#68662,#68663,#68664),.UNSPECIFIED.,.F.,.F.)
B_SPLINE_CURVE_WITH_KNOTS((3,3),(0.,0.247929805090893),.UNSPECIFIED.)
CURVE()
GEOMETRIC_REPRESENTATION_ITEM()
RATIONAL_B_SPLINE_CURVE((1.,1.00006942852818,1.00002415803416))
REPRESENTATION_ITEM('')
);
#18779=(
BOUNDED_CURVE()
B_SPLINE_CURVE(2,(#68670,#68671,#68672),.UNSPECIFIED.,.F.,.F.)
B_SPLINE_CURVE_WITH_KNOTS((3,3),(0.0522192481407881,0.300149053231599),
 .UNSPECIFIED.)
CURVE()
GEOMETRIC_REPRESENTATION_ITEM()
RATIONAL_B_SPLINE_CURVE((1.0000241580339,1.00006942852742,1.))
REPRESENTATION_ITEM('')
);
#18780=(
BOUNDED_CURVE()
B_SPLINE_CURVE(2,(#68674,#68675,#68676),.UNSPECIFIED.,.F.,.F.)
B_SPLINE_CURVE_WITH_KNOTS((3,3),(0.984623166322172,1.26677639839307),
 .UNSPECIFIED.)
CURVE()
GEOMETRIC_REPRESENTATION_ITEM()
RATIONAL_B_SPLINE_CURVE((1.02072197947249,1.02138328368541,1.02072197947249))
REPRESENTATION_ITEM('')
);
#18781=(
BOUNDED_CURVE()
B_SPLINE_CURVE(2,(#68677,#68678,#68679),.UNSPECIFIED.,.F.,.F.)
B_SPLINE_CURVE_WITH_KNOTS((3,3),(0.,0.24792980509091),.UNSPECIFIED.)
CURVE()
GEOMETRIC_REPRESENTATION_ITEM()
RATIONAL_B_SPLINE_CURVE((1.,1.00006942852692,1.00002415803372))
REPRESENTATION_ITEM('')
);
#18782=(
BOUNDED_CURVE()
B_SPLINE_CURVE(2,(#68685,#68686,#68687),.UNSPECIFIED.,.F.,.F.)
B_SPLINE_CURVE_WITH_KNOTS((3,3),(0.0522192481406546,0.300149053231598),
 .UNSPECIFIED.)
CURVE()
GEOMETRIC_REPRESENTATION_ITEM()
RATIONAL_B_SPLINE_CURVE((1.00002415803456,1.00006942852932,1.))
REPRESENTATION_ITEM('')
);
#18783=(
BOUNDED_CURVE()
B_SPLINE_CURVE(2,(#68689,#68690,#68691),.UNSPECIFIED.,.F.,.F.)
B_SPLINE_CURVE_WITH_KNOTS((3,3),(0.984623166322169,1.26677639839307),
 .UNSPECIFIED.)
CURVE()
GEOMETRIC_REPRESENTATION_ITEM()
RATIONAL_B_SPLINE_CURVE((1.02072197947249,1.02138328368541,1.02072197947249))
REPRESENTATION_ITEM('')
);
#18784=(
BOUNDED_CURVE()
B_SPLINE_CURVE(2,(#68692,#68693,#68694),.UNSPECIFIED.,.F.,.F.)
B_SPLINE_CURVE_WITH_KNOTS((3,3),(0.,0.247929805090884),.UNSPECIFIED.)
CURVE()
GEOMETRIC_REPRESENTATION_ITEM()
RATIONAL_B_SPLINE_CURVE((1.,1.00006942852775,1.00002415803401))
REPRESENTATION_ITEM('')
);
#18785=(
BOUNDED_CURVE()
B_SPLINE_CURVE(2,(#68700,#68701,#68702),.UNSPECIFIED.,.F.,.F.)
B_SPLINE_CURVE_WITH_KNOTS((3,3),(0.0522192481406402,0.300149053231599),
 .UNSPECIFIED.)
CURVE()
GEOMETRIC_REPRESENTATION_ITEM()
RATIONAL_B_SPLINE_CURVE((1.00002415803407,1.0000694285279,1.))
REPRESENTATION_ITEM('')
);
#18786=(
BOUNDED_CURVE()
B_SPLINE_CURVE(2,(#68704,#68705,#68706),.UNSPECIFIED.,.F.,.F.)
B_SPLINE_CURVE_WITH_KNOTS((3,3),(0.984623166322172,1.26677639839307),
 .UNSPECIFIED.)
CURVE()
GEOMETRIC_REPRESENTATION_ITEM()
RATIONAL_B_SPLINE_CURVE((1.02072197947249,1.02138328368541,1.02072197947249))
REPRESENTATION_ITEM('')
);
#18787=(
BOUNDED_CURVE()
B_SPLINE_CURVE(2,(#68707,#68708,#68709),.UNSPECIFIED.,.F.,.F.)
B_SPLINE_CURVE_WITH_KNOTS((3,3),(0.,0.247929805090997),.UNSPECIFIED.)
CURVE()
GEOMETRIC_REPRESENTATION_ITEM()
RATIONAL_B_SPLINE_CURVE((1.,1.00006942852925,1.00002415803454))
REPRESENTATION_ITEM('')
);
#18788=(
BOUNDED_CURVE()
B_SPLINE_CURVE(2,(#68715,#68716,#68717),.UNSPECIFIED.,.F.,.F.)
B_SPLINE_CURVE_WITH_KNOTS((3,3),(0.0522192481407274,0.300149053231599),
 .UNSPECIFIED.)
CURVE()
GEOMETRIC_REPRESENTATION_ITEM()
RATIONAL_B_SPLINE_CURVE((1.00002415803356,1.00006942852645,1.))
REPRESENTATION_ITEM('')
);
#18789=(
BOUNDED_CURVE()
B_SPLINE_CURVE(2,(#68719,#68720,#68721),.UNSPECIFIED.,.F.,.F.)
B_SPLINE_CURVE_WITH_KNOTS((3,3),(0.984623166322171,1.26677639839307),
 .UNSPECIFIED.)
CURVE()
GEOMETRIC_REPRESENTATION_ITEM()
RATIONAL_B_SPLINE_CURVE((1.02072197947249,1.02138328368541,1.02072197947249))
REPRESENTATION_ITEM('')
);
#18790=(
BOUNDED_CURVE()
B_SPLINE_CURVE(2,(#68722,#68723,#68724),.UNSPECIFIED.,.F.,.F.)
B_SPLINE_CURVE_WITH_KNOTS((3,3),(0.,0.247929805090888),.UNSPECIFIED.)
CURVE()
GEOMETRIC_REPRESENTATION_ITEM()
RATIONAL_B_SPLINE_CURVE((1.,1.00006942852913,1.00002415803449))
REPRESENTATION_ITEM('')
);
#18791=(
BOUNDED_CURVE()
B_SPLINE_CURVE(2,(#68730,#68731,#68732),.UNSPECIFIED.,.F.,.F.)
B_SPLINE_CURVE_WITH_KNOTS((3,3),(0.0522192481406619,0.300149053231598),
 .UNSPECIFIED.)
CURVE()
GEOMETRIC_REPRESENTATION_ITEM()
RATIONAL_B_SPLINE_CURVE((1.00002415803529,1.00006942853141,1.))
REPRESENTATION_ITEM('')
);
#18792=(
BOUNDED_CURVE()
B_SPLINE_CURVE(2,(#68734,#68735,#68736),.UNSPECIFIED.,.F.,.F.)
B_SPLINE_CURVE_WITH_KNOTS((3,3),(0.984623166322169,1.26677639839307),
 .UNSPECIFIED.)
CURVE()
GEOMETRIC_REPRESENTATION_ITEM()
RATIONAL_B_SPLINE_CURVE((1.02072197947249,1.02138328368541,1.02072197947249))
REPRESENTATION_ITEM('')
);
#18793=(
BOUNDED_CURVE()
B_SPLINE_CURVE(2,(#68737,#68738,#68739),.UNSPECIFIED.,.F.,.F.)
B_SPLINE_CURVE_WITH_KNOTS((3,3),(0.,0.247929805090904),.UNSPECIFIED.)
CURVE()
GEOMETRIC_REPRESENTATION_ITEM()
RATIONAL_B_SPLINE_CURVE((1.,1.00006942852951,1.00002415803463))
REPRESENTATION_ITEM('')
);
#18794=(
BOUNDED_CURVE()
B_SPLINE_CURVE(2,(#68745,#68746,#68747),.UNSPECIFIED.,.F.,.F.)
B_SPLINE_CURVE_WITH_KNOTS((3,3),(0.0522192481407164,0.300149053231598),
 .UNSPECIFIED.)
CURVE()
GEOMETRIC_REPRESENTATION_ITEM()
RATIONAL_B_SPLINE_CURVE((1.00002415803377,1.00006942852705,1.))
REPRESENTATION_ITEM('')
);
#18795=(
BOUNDED_CURVE()
B_SPLINE_CURVE(2,(#68749,#68750,#68751),.UNSPECIFIED.,.F.,.F.)
B_SPLINE_CURVE_WITH_KNOTS((3,3),(0.984623166322171,1.26677639839307),
 .UNSPECIFIED.)
CURVE()
GEOMETRIC_REPRESENTATION_ITEM()
RATIONAL_B_SPLINE_CURVE((1.02072197947249,1.02138328368541,1.02072197947249))
REPRESENTATION_ITEM('')
);
#18796=(
BOUNDED_CURVE()
B_SPLINE_CURVE(2,(#68752,#68753,#68754),.UNSPECIFIED.,.F.,.F.)
B_SPLINE_CURVE_WITH_KNOTS((3,3),(0.,0.247929805090835),.UNSPECIFIED.)
CURVE()
GEOMETRIC_REPRESENTATION_ITEM()
RATIONAL_B_SPLINE_CURVE((1.,1.00006942852771,1.000024158034))
REPRESENTATION_ITEM('')
);
#18797=(
BOUNDED_CURVE()
B_SPLINE_CURVE(2,(#68760,#68761,#68762),.UNSPECIFIED.,.F.,.F.)
B_SPLINE_CURVE_WITH_KNOTS((3,3),(0.0522192481406349,0.300149053231599),
 .UNSPECIFIED.)
CURVE()
GEOMETRIC_REPRESENTATION_ITEM()
RATIONAL_B_SPLINE_CURVE((1.00002415803477,1.00006942852992,1.))
REPRESENTATION_ITEM('')
);
#18798=(
BOUNDED_CURVE()
B_SPLINE_CURVE(2,(#68764,#68765,#68766),.UNSPECIFIED.,.F.,.F.)
B_SPLINE_CURVE_WITH_KNOTS((3,3),(0.984623166322174,1.26677639839308),
 .UNSPECIFIED.)
CURVE()
GEOMETRIC_REPRESENTATION_ITEM()
RATIONAL_B_SPLINE_CURVE((1.02072197947248,1.0213832836854,1.02072197947248))
REPRESENTATION_ITEM('')
);
#18799=(
BOUNDED_CURVE()
B_SPLINE_CURVE(2,(#68767,#68768,#68769),.UNSPECIFIED.,.F.,.F.)
B_SPLINE_CURVE_WITH_KNOTS((3,3),(0.,0.247929805090929),.UNSPECIFIED.)
CURVE()
GEOMETRIC_REPRESENTATION_ITEM()
RATIONAL_B_SPLINE_CURVE((1.,1.00006942852897,1.00002415803444))
REPRESENTATION_ITEM('')
);
#18800=(
BOUNDED_CURVE()
B_SPLINE_CURVE(2,(#68775,#68776,#68777),.UNSPECIFIED.,.F.,.F.)
B_SPLINE_CURVE_WITH_KNOTS((3,3),(0.0522192481406456,0.300149053231598),
 .UNSPECIFIED.)
CURVE()
GEOMETRIC_REPRESENTATION_ITEM()
RATIONAL_B_SPLINE_CURVE((1.0000241580344,1.00006942852887,1.))
REPRESENTATION_ITEM('')
);
#18801=(
BOUNDED_CURVE()
B_SPLINE_CURVE(2,(#68779,#68780,#68781),.UNSPECIFIED.,.F.,.F.)
B_SPLINE_CURVE_WITH_KNOTS((3,3),(0.984623166322169,1.26677639839307),
 .UNSPECIFIED.)
CURVE()
GEOMETRIC_REPRESENTATION_ITEM()
RATIONAL_B_SPLINE_CURVE((1.02072197947249,1.0213832836854,1.02072197947249))
REPRESENTATION_ITEM('')
);
#18802=(
BOUNDED_CURVE()
B_SPLINE_CURVE(2,(#68782,#68783,#68784),.UNSPECIFIED.,.F.,.F.)
B_SPLINE_CURVE_WITH_KNOTS((3,3),(0.,0.247929805090801),.UNSPECIFIED.)
CURVE()
GEOMETRIC_REPRESENTATION_ITEM()
RATIONAL_B_SPLINE_CURVE((1.,1.00006942852834,1.00002415803422))
REPRESENTATION_ITEM('')
);
#18803=(
BOUNDED_CURVE()
B_SPLINE_CURVE(2,(#68790,#68791,#68792),.UNSPECIFIED.,.F.,.F.)
B_SPLINE_CURVE_WITH_KNOTS((3,3),(0.0522192481407089,0.300149053231598),
 .UNSPECIFIED.)
CURVE()
GEOMETRIC_REPRESENTATION_ITEM()
RATIONAL_B_SPLINE_CURVE((1.00002415803465,1.00006942852957,1.))
REPRESENTATION_ITEM('')
);
#18804=(
BOUNDED_CURVE()
B_SPLINE_CURVE(2,(#68794,#68795,#68796),.UNSPECIFIED.,.F.,.F.)
B_SPLINE_CURVE_WITH_KNOTS((3,3),(0.984623166322172,1.26677639839307),
 .UNSPECIFIED.)
CURVE()
GEOMETRIC_REPRESENTATION_ITEM()
RATIONAL_B_SPLINE_CURVE((1.02072197947249,1.02138328368541,1.02072197947249))
REPRESENTATION_ITEM('')
);
#18805=(
BOUNDED_CURVE()
B_SPLINE_CURVE(2,(#68797,#68798,#68799),.UNSPECIFIED.,.F.,.F.)
B_SPLINE_CURVE_WITH_KNOTS((3,3),(0.,0.247929805090902),.UNSPECIFIED.)
CURVE()
GEOMETRIC_REPRESENTATION_ITEM()
RATIONAL_B_SPLINE_CURVE((1.,1.0000694285288,1.00002415803438))
REPRESENTATION_ITEM('')
);
#18806=(
BOUNDED_CURVE()
B_SPLINE_CURVE(2,(#68832,#68833,#68834),.UNSPECIFIED.,.F.,.F.)
B_SPLINE_CURVE_WITH_KNOTS((3,3),(0.984623166322171,1.26677639839307),
 .UNSPECIFIED.)
CURVE()
GEOMETRIC_REPRESENTATION_ITEM()
RATIONAL_B_SPLINE_CURVE((1.02072197947249,1.02138328368541,1.02072197947249))
REPRESENTATION_ITEM('')
);
#18807=(
BOUNDED_CURVE()
B_SPLINE_CURVE(2,(#68870,#68871,#68872),.UNSPECIFIED.,.F.,.F.)
B_SPLINE_CURVE_WITH_KNOTS((3,3),(0.,0.0730837266078461),.UNSPECIFIED.)
CURVE()
GEOMETRIC_REPRESENTATION_ITEM()
RATIONAL_B_SPLINE_CURVE((1.,1.00000531281866,1.0000024358309))
REPRESENTATION_ITEM('')
);
#18808=(
BOUNDED_CURVE()
B_SPLINE_CURVE(2,(#68908,#68909,#68910),.UNSPECIFIED.,.F.,.F.)
B_SPLINE_CURVE_WITH_KNOTS((3,3),(0.98462316632217,1.26677639839307),
 .UNSPECIFIED.)
CURVE()
GEOMETRIC_REPRESENTATION_ITEM()
RATIONAL_B_SPLINE_CURVE((1.02072197947249,1.02138328368541,1.02072197947249))
REPRESENTATION_ITEM('')
);
#18809=(
BOUNDED_CURVE()
B_SPLINE_CURVE(2,(#68946,#68947,#68948),.UNSPECIFIED.,.F.,.F.)
B_SPLINE_CURVE_WITH_KNOTS((3,3),(0.,0.0730837266087433),.UNSPECIFIED.)
CURVE()
GEOMETRIC_REPRESENTATION_ITEM()
RATIONAL_B_SPLINE_CURVE((1.,1.00000531285818,1.00000243584903))
REPRESENTATION_ITEM('')
);
#18810=(
BOUNDED_CURVE()
B_SPLINE_CURVE(2,(#68984,#68985,#68986),.UNSPECIFIED.,.F.,.F.)
B_SPLINE_CURVE_WITH_KNOTS((3,3),(0.984623166322173,1.26677639839308),
 .UNSPECIFIED.)
CURVE()
GEOMETRIC_REPRESENTATION_ITEM()
RATIONAL_B_SPLINE_CURVE((1.02072197947249,1.02138328368541,1.02072197947249))
REPRESENTATION_ITEM('')
);
#18811=(
BOUNDED_CURVE()
B_SPLINE_CURVE(2,(#69022,#69023,#69024),.UNSPECIFIED.,.F.,.F.)
B_SPLINE_CURVE_WITH_KNOTS((3,3),(0.,0.0730837266085301),.UNSPECIFIED.)
CURVE()
GEOMETRIC_REPRESENTATION_ITEM()
RATIONAL_B_SPLINE_CURVE((1.,1.0000053128329,1.00000243583743))
REPRESENTATION_ITEM('')
);
#18812=(
BOUNDED_CURVE()
B_SPLINE_CURVE(2,(#69060,#69061,#69062),.UNSPECIFIED.,.F.,.F.)
B_SPLINE_CURVE_WITH_KNOTS((3,3),(0.984623166322171,1.26677639839307),
 .UNSPECIFIED.)
CURVE()
GEOMETRIC_REPRESENTATION_ITEM()
RATIONAL_B_SPLINE_CURVE((1.02072197947249,1.02138328368541,1.02072197947249))
REPRESENTATION_ITEM('')
);
#18813=(
BOUNDED_CURVE()
B_SPLINE_CURVE(2,(#69098,#69099,#69100),.UNSPECIFIED.,.F.,.F.)
B_SPLINE_CURVE_WITH_KNOTS((3,3),(0.,0.073083726608233),.UNSPECIFIED.)
CURVE()
GEOMETRIC_REPRESENTATION_ITEM()
RATIONAL_B_SPLINE_CURVE((1.,1.00000531282325,1.00000243583301))
REPRESENTATION_ITEM('')
);
#18814=(
BOUNDED_CURVE()
B_SPLINE_CURVE(2,(#69136,#69137,#69138),.UNSPECIFIED.,.F.,.F.)
B_SPLINE_CURVE_WITH_KNOTS((3,3),(0.98462316632217,1.26677639839307),
 .UNSPECIFIED.)
CURVE()
GEOMETRIC_REPRESENTATION_ITEM()
RATIONAL_B_SPLINE_CURVE((1.02072197947249,1.02138328368541,1.02072197947249))
REPRESENTATION_ITEM('')
);
#18815=(
BOUNDED_CURVE()
B_SPLINE_CURVE(2,(#69174,#69175,#69176),.UNSPECIFIED.,.F.,.F.)
B_SPLINE_CURVE_WITH_KNOTS((3,3),(0.,0.0730837266086981),.UNSPECIFIED.)
CURVE()
GEOMETRIC_REPRESENTATION_ITEM()
RATIONAL_B_SPLINE_CURVE((1.,1.000005312841,1.00000243584115))
REPRESENTATION_ITEM('')
);
#18816=(
BOUNDED_CURVE()
B_SPLINE_CURVE(2,(#69212,#69213,#69214),.UNSPECIFIED.,.F.,.F.)
B_SPLINE_CURVE_WITH_KNOTS((3,3),(0.984623166322174,1.26677639839308),
 .UNSPECIFIED.)
CURVE()
GEOMETRIC_REPRESENTATION_ITEM()
RATIONAL_B_SPLINE_CURVE((1.02072197947249,1.02138328368541,1.02072197947249))
REPRESENTATION_ITEM('')
);
#18817=(
BOUNDED_CURVE()
B_SPLINE_CURVE(2,(#69250,#69251,#69252),.UNSPECIFIED.,.F.,.F.)
B_SPLINE_CURVE_WITH_KNOTS((3,3),(0.,0.0730837266083448),.UNSPECIFIED.)
CURVE()
GEOMETRIC_REPRESENTATION_ITEM()
RATIONAL_B_SPLINE_CURVE((1.,1.00000531283336,1.00000243583764))
REPRESENTATION_ITEM('')
);
#18818=(
BOUNDED_CURVE()
B_SPLINE_CURVE(2,(#69288,#69289,#69290),.UNSPECIFIED.,.F.,.F.)
B_SPLINE_CURVE_WITH_KNOTS((3,3),(0.984623166322172,1.26677639839307),
 .UNSPECIFIED.)
CURVE()
GEOMETRIC_REPRESENTATION_ITEM()
RATIONAL_B_SPLINE_CURVE((1.02072197947249,1.02138328368541,1.02072197947249))
REPRESENTATION_ITEM('')
);
#18819=(
BOUNDED_CURVE()
B_SPLINE_CURVE(2,(#69326,#69327,#69328),.UNSPECIFIED.,.F.,.F.)
B_SPLINE_CURVE_WITH_KNOTS((3,3),(0.,0.0730837266085423),.UNSPECIFIED.)
CURVE()
GEOMETRIC_REPRESENTATION_ITEM()
RATIONAL_B_SPLINE_CURVE((1.,1.00000531284476,1.00000243584287))
REPRESENTATION_ITEM('')
);
#18820=(
BOUNDED_CURVE()
B_SPLINE_CURVE(2,(#69364,#69365,#69366),.UNSPECIFIED.,.F.,.F.)
B_SPLINE_CURVE_WITH_KNOTS((3,3),(0.98462316632217,1.26677639839307),
 .UNSPECIFIED.)
CURVE()
GEOMETRIC_REPRESENTATION_ITEM()
RATIONAL_B_SPLINE_CURVE((1.02072197947249,1.02138328368541,1.02072197947249))
REPRESENTATION_ITEM('')
);
#18821=(
BOUNDED_CURVE()
B_SPLINE_CURVE(2,(#69402,#69403,#69404),.UNSPECIFIED.,.F.,.F.)
B_SPLINE_CURVE_WITH_KNOTS((3,3),(0.,0.0730837266082547),.UNSPECIFIED.)
CURVE()
GEOMETRIC_REPRESENTATION_ITEM()
RATIONAL_B_SPLINE_CURVE((1.,1.0000053128325,1.00000243583725))
REPRESENTATION_ITEM('')
);
#18822=(
BOUNDED_CURVE()
B_SPLINE_CURVE(2,(#69440,#69441,#69442),.UNSPECIFIED.,.F.,.F.)
B_SPLINE_CURVE_WITH_KNOTS((3,3),(0.984623166322172,1.26677639839307),
 .UNSPECIFIED.)
CURVE()
GEOMETRIC_REPRESENTATION_ITEM()
RATIONAL_B_SPLINE_CURVE((1.02072197947249,1.02138328368541,1.02072197947249))
REPRESENTATION_ITEM('')
);
#18823=(
BOUNDED_CURVE()
B_SPLINE_CURVE(2,(#69478,#69479,#69480),.UNSPECIFIED.,.F.,.F.)
B_SPLINE_CURVE_WITH_KNOTS((3,3),(0.,0.0730837266088366),.UNSPECIFIED.)
CURVE()
GEOMETRIC_REPRESENTATION_ITEM()
RATIONAL_B_SPLINE_CURVE((1.,1.00000531284141,1.00000243584134))
REPRESENTATION_ITEM('')
);
#18824=(
BOUNDED_CURVE()
B_SPLINE_CURVE(2,(#69516,#69517,#69518),.UNSPECIFIED.,.F.,.F.)
B_SPLINE_CURVE_WITH_KNOTS((3,3),(0.984623166322171,1.26677639839307),
 .UNSPECIFIED.)
CURVE()
GEOMETRIC_REPRESENTATION_ITEM()
RATIONAL_B_SPLINE_CURVE((1.02072197947249,1.02138328368541,1.02072197947249))
REPRESENTATION_ITEM('')
);
#18825=(
BOUNDED_CURVE()
B_SPLINE_CURVE(2,(#69554,#69555,#69556),.UNSPECIFIED.,.F.,.F.)
B_SPLINE_CURVE_WITH_KNOTS((3,3),(0.,0.0730837266084984),.UNSPECIFIED.)
CURVE()
GEOMETRIC_REPRESENTATION_ITEM()
RATIONAL_B_SPLINE_CURVE((1.,1.00000531283258,1.00000243583729))
REPRESENTATION_ITEM('')
);
#18826=(
BOUNDED_CURVE()
B_SPLINE_CURVE(2,(#69592,#69593,#69594),.UNSPECIFIED.,.F.,.F.)
B_SPLINE_CURVE_WITH_KNOTS((3,3),(0.984623166322171,1.26677639839307),
 .UNSPECIFIED.)
CURVE()
GEOMETRIC_REPRESENTATION_ITEM()
RATIONAL_B_SPLINE_CURVE((1.02072197947249,1.02138328368541,1.02072197947249))
REPRESENTATION_ITEM('')
);
#18827=(
BOUNDED_CURVE()
B_SPLINE_CURVE(2,(#69630,#69631,#69632),.UNSPECIFIED.,.F.,.F.)
B_SPLINE_CURVE_WITH_KNOTS((3,3),(0.,0.07308372660832),.UNSPECIFIED.)
CURVE()
GEOMETRIC_REPRESENTATION_ITEM()
RATIONAL_B_SPLINE_CURVE((1.,1.00000531285587,1.00000243584797))
REPRESENTATION_ITEM('')
);
#18828=(
BOUNDED_CURVE()
B_SPLINE_CURVE(2,(#69668,#69669,#69670),.UNSPECIFIED.,.F.,.F.)
B_SPLINE_CURVE_WITH_KNOTS((3,3),(0.984623166322173,1.26677639839308),
 .UNSPECIFIED.)
CURVE()
GEOMETRIC_REPRESENTATION_ITEM()
RATIONAL_B_SPLINE_CURVE((1.02072197947249,1.02138328368541,1.02072197947249))
REPRESENTATION_ITEM('')
);
#18829=(
BOUNDED_CURVE()
B_SPLINE_CURVE(2,(#69706,#69707,#69708),.UNSPECIFIED.,.F.,.F.)
B_SPLINE_CURVE_WITH_KNOTS((3,3),(0.,0.0730837266084226),.UNSPECIFIED.)
CURVE()
GEOMETRIC_REPRESENTATION_ITEM()
RATIONAL_B_SPLINE_CURVE((1.,1.00000531284265,1.0000024358419))
REPRESENTATION_ITEM('')
);
#18830=(
BOUNDED_CURVE()
B_SPLINE_CURVE(2,(#69744,#69745,#69746),.UNSPECIFIED.,.F.,.F.)
B_SPLINE_CURVE_WITH_KNOTS((3,3),(0.984623166322167,1.26677639839307),
 .UNSPECIFIED.)
CURVE()
GEOMETRIC_REPRESENTATION_ITEM()
RATIONAL_B_SPLINE_CURVE((1.02072197947249,1.02138328368541,1.02072197947249))
REPRESENTATION_ITEM('')
);
#18831=(
BOUNDED_CURVE()
B_SPLINE_CURVE(2,(#69782,#69783,#69784),.UNSPECIFIED.,.F.,.F.)
B_SPLINE_CURVE_WITH_KNOTS((3,3),(0.,0.0730837266083765),.UNSPECIFIED.)
CURVE()
GEOMETRIC_REPRESENTATION_ITEM()
RATIONAL_B_SPLINE_CURVE((1.,1.00000531283331,1.00000243583762))
REPRESENTATION_ITEM('')
);
#18832=(
BOUNDED_CURVE()
B_SPLINE_CURVE(2,(#69820,#69821,#69822),.UNSPECIFIED.,.F.,.F.)
B_SPLINE_CURVE_WITH_KNOTS((3,3),(0.984623166322173,1.26677639839307),
 .UNSPECIFIED.)
CURVE()
GEOMETRIC_REPRESENTATION_ITEM()
RATIONAL_B_SPLINE_CURVE((1.02072197947249,1.02138328368541,1.02072197947249))
REPRESENTATION_ITEM('')
);
#18833=(
BOUNDED_CURVE()
B_SPLINE_CURVE(2,(#69858,#69859,#69860),.UNSPECIFIED.,.F.,.F.)
B_SPLINE_CURVE_WITH_KNOTS((3,3),(0.,0.0730837266082079),.UNSPECIFIED.)
CURVE()
GEOMETRIC_REPRESENTATION_ITEM()
RATIONAL_B_SPLINE_CURVE((1.,1.00000531281752,1.00000243583038))
REPRESENTATION_ITEM('')
);
#18834=(
BOUNDED_CURVE()
B_SPLINE_CURVE(2,(#69896,#69897,#69898),.UNSPECIFIED.,.F.,.F.)
B_SPLINE_CURVE_WITH_KNOTS((3,3),(0.984623166322173,1.26677639839308),
 .UNSPECIFIED.)
CURVE()
GEOMETRIC_REPRESENTATION_ITEM()
RATIONAL_B_SPLINE_CURVE((1.02072197947249,1.02138328368541,1.02072197947249))
REPRESENTATION_ITEM('')
);
#18835=(
BOUNDED_CURVE()
B_SPLINE_CURVE(2,(#69934,#69935,#69936),.UNSPECIFIED.,.F.,.F.)
B_SPLINE_CURVE_WITH_KNOTS((3,3),(0.,0.0730837266086429),.UNSPECIFIED.)
CURVE()
GEOMETRIC_REPRESENTATION_ITEM()
RATIONAL_B_SPLINE_CURVE((1.,1.00000531285462,1.00000243584739))
REPRESENTATION_ITEM('')
);
#18836=(
BOUNDED_CURVE()
B_SPLINE_CURVE(2,(#69972,#69973,#69974),.UNSPECIFIED.,.F.,.F.)
B_SPLINE_CURVE_WITH_KNOTS((3,3),(0.98462316632217,1.26677639839307),
 .UNSPECIFIED.)
CURVE()
GEOMETRIC_REPRESENTATION_ITEM()
RATIONAL_B_SPLINE_CURVE((1.02072197947249,1.02138328368541,1.02072197947249))
REPRESENTATION_ITEM('')
);
#18837=(
BOUNDED_CURVE()
B_SPLINE_CURVE(2,(#70010,#70011,#70012),.UNSPECIFIED.,.F.,.F.)
B_SPLINE_CURVE_WITH_KNOTS((3,3),(0.,0.0730837266083056),.UNSPECIFIED.)
CURVE()
GEOMETRIC_REPRESENTATION_ITEM()
RATIONAL_B_SPLINE_CURVE((1.,1.00000531283932,1.00000243584038))
REPRESENTATION_ITEM('')
);
#18838=(
BOUNDED_CURVE()
B_SPLINE_CURVE(2,(#70048,#70049,#70050),.UNSPECIFIED.,.F.,.F.)
B_SPLINE_CURVE_WITH_KNOTS((3,3),(0.98462316632217,1.26677639839307),
 .UNSPECIFIED.)
CURVE()
GEOMETRIC_REPRESENTATION_ITEM()
RATIONAL_B_SPLINE_CURVE((1.02072197947249,1.02138328368541,1.02072197947249))
REPRESENTATION_ITEM('')
);
#18839=(
BOUNDED_CURVE()
B_SPLINE_CURVE(2,(#70086,#70087,#70088),.UNSPECIFIED.,.F.,.F.)
B_SPLINE_CURVE_WITH_KNOTS((3,3),(0.,0.0730837266081987),.UNSPECIFIED.)
CURVE()
GEOMETRIC_REPRESENTATION_ITEM()
RATIONAL_B_SPLINE_CURVE((1.,1.00000531282782,1.00000243583511))
REPRESENTATION_ITEM('')
);
#18840=(
BOUNDED_CURVE()
B_SPLINE_CURVE(2,(#70124,#70125,#70126),.UNSPECIFIED.,.F.,.F.)
B_SPLINE_CURVE_WITH_KNOTS((3,3),(0.984623166322174,1.26677639839308),
 .UNSPECIFIED.)
CURVE()
GEOMETRIC_REPRESENTATION_ITEM()
RATIONAL_B_SPLINE_CURVE((1.02072197947248,1.0213832836854,1.02072197947248))
REPRESENTATION_ITEM('')
);
#18841=(
BOUNDED_CURVE()
B_SPLINE_CURVE(2,(#70162,#70163,#70164),.UNSPECIFIED.,.F.,.F.)
B_SPLINE_CURVE_WITH_KNOTS((3,3),(0.,0.0730837266084284),.UNSPECIFIED.)
CURVE()
GEOMETRIC_REPRESENTATION_ITEM()
RATIONAL_B_SPLINE_CURVE((1.,1.00000531283343,1.00000243583768))
REPRESENTATION_ITEM('')
);
#18842=(
BOUNDED_CURVE()
B_SPLINE_CURVE(2,(#70200,#70201,#70202),.UNSPECIFIED.,.F.,.F.)
B_SPLINE_CURVE_WITH_KNOTS((3,3),(0.984623166322172,1.26677639839307),
 .UNSPECIFIED.)
CURVE()
GEOMETRIC_REPRESENTATION_ITEM()
RATIONAL_B_SPLINE_CURVE((1.02072197947249,1.02138328368541,1.02072197947249))
REPRESENTATION_ITEM('')
);
#18843=(
BOUNDED_CURVE()
B_SPLINE_CURVE(2,(#70238,#70239,#70240),.UNSPECIFIED.,.F.,.F.)
B_SPLINE_CURVE_WITH_KNOTS((3,3),(0.,0.0730837266080622),.UNSPECIFIED.)
CURVE()
GEOMETRIC_REPRESENTATION_ITEM()
RATIONAL_B_SPLINE_CURVE((1.,1.00000531280049,1.00000243582258))
REPRESENTATION_ITEM('')
);
#18844=(
BOUNDED_CURVE()
B_SPLINE_CURVE(2,(#70276,#70277,#70278),.UNSPECIFIED.,.F.,.F.)
B_SPLINE_CURVE_WITH_KNOTS((3,3),(0.984623166322171,1.26677639839307),
 .UNSPECIFIED.)
CURVE()
GEOMETRIC_REPRESENTATION_ITEM()
RATIONAL_B_SPLINE_CURVE((1.02072197947249,1.02138328368541,1.02072197947249))
REPRESENTATION_ITEM('')
);
#18845=(
BOUNDED_CURVE()
B_SPLINE_CURVE(2,(#70314,#70315,#70316),.UNSPECIFIED.,.F.,.F.)
B_SPLINE_CURVE_WITH_KNOTS((3,3),(0.,0.0730837266082324),.UNSPECIFIED.)
CURVE()
GEOMETRIC_REPRESENTATION_ITEM()
RATIONAL_B_SPLINE_CURVE((1.,1.00000531281127,1.00000243582752))
REPRESENTATION_ITEM('')
);
#18846=(
BOUNDED_CURVE()
B_SPLINE_CURVE(2,(#70352,#70353,#70354),.UNSPECIFIED.,.F.,.F.)
B_SPLINE_CURVE_WITH_KNOTS((3,3),(0.984623166322172,1.26677639839308),
 .UNSPECIFIED.)
CURVE()
GEOMETRIC_REPRESENTATION_ITEM()
RATIONAL_B_SPLINE_CURVE((1.02072197947249,1.02138328368541,1.02072197947249))
REPRESENTATION_ITEM('')
);
#18847=(
BOUNDED_CURVE()
B_SPLINE_CURVE(2,(#70390,#70391,#70392),.UNSPECIFIED.,.F.,.F.)
B_SPLINE_CURVE_WITH_KNOTS((3,3),(0.,0.0730837266089022),.UNSPECIFIED.)
CURVE()
GEOMETRIC_REPRESENTATION_ITEM()
RATIONAL_B_SPLINE_CURVE((1.,1.00000531286309,1.00000243585128))
REPRESENTATION_ITEM('')
);
#18848=(
BOUNDED_CURVE()
B_SPLINE_CURVE(2,(#70428,#70429,#70430),.UNSPECIFIED.,.F.,.F.)
B_SPLINE_CURVE_WITH_KNOTS((3,3),(0.984623166322172,1.26677639839308),
 .UNSPECIFIED.)
CURVE()
GEOMETRIC_REPRESENTATION_ITEM()
RATIONAL_B_SPLINE_CURVE((1.02072197947249,1.02138328368541,1.02072197947249))
REPRESENTATION_ITEM('')
);
#18849=(
BOUNDED_CURVE()
B_SPLINE_CURVE(2,(#70466,#70467,#70468),.UNSPECIFIED.,.F.,.F.)
B_SPLINE_CURVE_WITH_KNOTS((3,3),(0.,0.0730837266085706),.UNSPECIFIED.)
CURVE()
GEOMETRIC_REPRESENTATION_ITEM()
RATIONAL_B_SPLINE_CURVE((1.,1.00000531283577,1.00000243583875))
REPRESENTATION_ITEM('')
);
#18850=(
BOUNDED_CURVE()
B_SPLINE_CURVE(2,(#70504,#70505,#70506),.UNSPECIFIED.,.F.,.F.)
B_SPLINE_CURVE_WITH_KNOTS((3,3),(0.98462316632217,1.26677639839307),
 .UNSPECIFIED.)
CURVE()
GEOMETRIC_REPRESENTATION_ITEM()
RATIONAL_B_SPLINE_CURVE((1.02072197947249,1.02138328368541,1.02072197947249))
REPRESENTATION_ITEM('')
);
#18851=(
BOUNDED_CURVE()
B_SPLINE_CURVE(2,(#70542,#70543,#70544),.UNSPECIFIED.,.F.,.F.)
B_SPLINE_CURVE_WITH_KNOTS((3,3),(0.,0.0730837266086981),.UNSPECIFIED.)
CURVE()
GEOMETRIC_REPRESENTATION_ITEM()
RATIONAL_B_SPLINE_CURVE((1.,1.000005312841,1.00000243584115))
REPRESENTATION_ITEM('')
);
#18852=(
BOUNDED_CURVE()
B_SPLINE_CURVE(2,(#70580,#70581,#70582),.UNSPECIFIED.,.F.,.F.)
B_SPLINE_CURVE_WITH_KNOTS((3,3),(0.984623166322173,1.26677639839308),
 .UNSPECIFIED.)
CURVE()
GEOMETRIC_REPRESENTATION_ITEM()
RATIONAL_B_SPLINE_CURVE((1.02072197947249,1.02138328368541,1.02072197947249))
REPRESENTATION_ITEM('')
);
#18853=(
BOUNDED_CURVE()
B_SPLINE_CURVE(2,(#70618,#70619,#70620),.UNSPECIFIED.,.F.,.F.)
B_SPLINE_CURVE_WITH_KNOTS((3,3),(0.,0.0730837266081137),.UNSPECIFIED.)
CURVE()
GEOMETRIC_REPRESENTATION_ITEM()
RATIONAL_B_SPLINE_CURVE((1.,1.0000053128201,1.00000243583157))
REPRESENTATION_ITEM('')
);
#18854=(
BOUNDED_CURVE()
B_SPLINE_CURVE(2,(#70656,#70657,#70658),.UNSPECIFIED.,.F.,.F.)
B_SPLINE_CURVE_WITH_KNOTS((3,3),(0.98462316632217,1.26677639839307),
 .UNSPECIFIED.)
CURVE()
GEOMETRIC_REPRESENTATION_ITEM()
RATIONAL_B_SPLINE_CURVE((1.02072197947249,1.02138328368541,1.02072197947249))
REPRESENTATION_ITEM('')
);
#18855=(
BOUNDED_CURVE()
B_SPLINE_CURVE(2,(#70694,#70695,#70696),.UNSPECIFIED.,.F.,.F.)
B_SPLINE_CURVE_WITH_KNOTS((3,3),(0.,0.0730837266081729),.UNSPECIFIED.)
CURVE()
GEOMETRIC_REPRESENTATION_ITEM()
RATIONAL_B_SPLINE_CURVE((1.,1.00000531281639,1.00000243582987))
REPRESENTATION_ITEM('')
);
#18856=(
BOUNDED_CURVE()
B_SPLINE_CURVE(2,(#70732,#70733,#70734),.UNSPECIFIED.,.F.,.F.)
B_SPLINE_CURVE_WITH_KNOTS((3,3),(0.984623166322172,1.26677639839307),
 .UNSPECIFIED.)
CURVE()
GEOMETRIC_REPRESENTATION_ITEM()
RATIONAL_B_SPLINE_CURVE((1.02072197947249,1.0213832836854,1.02072197947249))
REPRESENTATION_ITEM('')
);
#18857=(
BOUNDED_CURVE()
B_SPLINE_CURVE(2,(#70770,#70771,#70772),.UNSPECIFIED.,.F.,.F.)
B_SPLINE_CURVE_WITH_KNOTS((3,3),(0.,0.0730837266080691),.UNSPECIFIED.)
CURVE()
GEOMETRIC_REPRESENTATION_ITEM()
RATIONAL_B_SPLINE_CURVE((1.,1.00000531281001,1.00000243582694))
REPRESENTATION_ITEM('')
);
#18858=(
BOUNDED_CURVE()
B_SPLINE_CURVE(2,(#70808,#70809,#70810),.UNSPECIFIED.,.F.,.F.)
B_SPLINE_CURVE_WITH_KNOTS((3,3),(0.984623166322169,1.26677639839307),
 .UNSPECIFIED.)
CURVE()
GEOMETRIC_REPRESENTATION_ITEM()
RATIONAL_B_SPLINE_CURVE((1.02072197947249,1.02138328368541,1.02072197947249))
REPRESENTATION_ITEM('')
);
#18859=(
BOUNDED_CURVE()
B_SPLINE_CURVE(2,(#70846,#70847,#70848),.UNSPECIFIED.,.F.,.F.)
B_SPLINE_CURVE_WITH_KNOTS((3,3),(0.,0.0730837266082608),.UNSPECIFIED.)
CURVE()
GEOMETRIC_REPRESENTATION_ITEM()
RATIONAL_B_SPLINE_CURVE((1.,1.00000531281977,1.00000243583142))
REPRESENTATION_ITEM('')
);
#18860=(
BOUNDED_CURVE()
B_SPLINE_CURVE(2,(#70884,#70885,#70886),.UNSPECIFIED.,.F.,.F.)
B_SPLINE_CURVE_WITH_KNOTS((3,3),(0.984623166322172,1.26677639839307),
 .UNSPECIFIED.)
CURVE()
GEOMETRIC_REPRESENTATION_ITEM()
RATIONAL_B_SPLINE_CURVE((1.02072197947249,1.02138328368541,1.02072197947249))
REPRESENTATION_ITEM('')
);
#18861=(
BOUNDED_CURVE()
B_SPLINE_CURVE(2,(#70922,#70923,#70924),.UNSPECIFIED.,.F.,.F.)
B_SPLINE_CURVE_WITH_KNOTS((3,3),(0.,0.0730837266082887),.UNSPECIFIED.)
CURVE()
GEOMETRIC_REPRESENTATION_ITEM()
RATIONAL_B_SPLINE_CURVE((1.,1.00000531281023,1.00000243582704))
REPRESENTATION_ITEM('')
);
#18862=(
BOUNDED_CURVE()
B_SPLINE_CURVE(2,(#70960,#70961,#70962),.UNSPECIFIED.,.F.,.F.)
B_SPLINE_CURVE_WITH_KNOTS((3,3),(0.984623166322172,1.26677639839307),
 .UNSPECIFIED.)
CURVE()
GEOMETRIC_REPRESENTATION_ITEM()
RATIONAL_B_SPLINE_CURVE((1.02072197947249,1.02138328368541,1.02072197947249))
REPRESENTATION_ITEM('')
);
#18863=(
BOUNDED_CURVE()
B_SPLINE_CURVE(2,(#70998,#70999,#71000),.UNSPECIFIED.,.F.,.F.)
B_SPLINE_CURVE_WITH_KNOTS((3,3),(0.,0.0730837266079997),.UNSPECIFIED.)
CURVE()
GEOMETRIC_REPRESENTATION_ITEM()
RATIONAL_B_SPLINE_CURVE((1.,1.00000531280928,1.0000024358266))
REPRESENTATION_ITEM('')
);
#18864=(
BOUNDED_CURVE()
B_SPLINE_CURVE(2,(#71036,#71037,#71038),.UNSPECIFIED.,.F.,.F.)
B_SPLINE_CURVE_WITH_KNOTS((3,3),(0.984623166322169,1.26677639839307),
 .UNSPECIFIED.)
CURVE()
GEOMETRIC_REPRESENTATION_ITEM()
RATIONAL_B_SPLINE_CURVE((1.02072197947249,1.02138328368541,1.02072197947249))
REPRESENTATION_ITEM('')
);
#18865=(
BOUNDED_CURVE()
B_SPLINE_CURVE(2,(#71074,#71075,#71076),.UNSPECIFIED.,.F.,.F.)
B_SPLINE_CURVE_WITH_KNOTS((3,3),(0.,0.0730837266086672),.UNSPECIFIED.)
CURVE()
GEOMETRIC_REPRESENTATION_ITEM()
RATIONAL_B_SPLINE_CURVE((1.,1.00000531284996,1.00000243584525))
REPRESENTATION_ITEM('')
);
#18866=(
BOUNDED_CURVE()
B_SPLINE_CURVE(2,(#71112,#71113,#71114),.UNSPECIFIED.,.F.,.F.)
B_SPLINE_CURVE_WITH_KNOTS((3,3),(0.984623166322172,1.26677639839307),
 .UNSPECIFIED.)
CURVE()
GEOMETRIC_REPRESENTATION_ITEM()
RATIONAL_B_SPLINE_CURVE((1.02072197947249,1.02138328368541,1.02072197947249))
REPRESENTATION_ITEM('')
);
#18867=(
BOUNDED_CURVE()
B_SPLINE_CURVE(2,(#71150,#71151,#71152),.UNSPECIFIED.,.F.,.F.)
B_SPLINE_CURVE_WITH_KNOTS((3,3),(0.,0.0730837266084481),.UNSPECIFIED.)
CURVE()
GEOMETRIC_REPRESENTATION_ITEM()
RATIONAL_B_SPLINE_CURVE((1.,1.00000531284005,1.00000243584071))
REPRESENTATION_ITEM('')
);
#18868=(
BOUNDED_CURVE()
B_SPLINE_CURVE(2,(#71188,#71189,#71190),.UNSPECIFIED.,.F.,.F.)
B_SPLINE_CURVE_WITH_KNOTS((3,3),(0.984623166322169,1.26677639839307),
 .UNSPECIFIED.)
CURVE()
GEOMETRIC_REPRESENTATION_ITEM()
RATIONAL_B_SPLINE_CURVE((1.02072197947249,1.02138328368541,1.02072197947249))
REPRESENTATION_ITEM('')
);
#18869=(
BOUNDED_CURVE()
B_SPLINE_CURVE(2,(#71226,#71227,#71228),.UNSPECIFIED.,.F.,.F.)
B_SPLINE_CURVE_WITH_KNOTS((3,3),(0.,0.073083726608594),.UNSPECIFIED.)
CURVE()
GEOMETRIC_REPRESENTATION_ITEM()
RATIONAL_B_SPLINE_CURVE((1.,1.00000531283215,1.00000243583709))
REPRESENTATION_ITEM('')
);
#18870=(
BOUNDED_CURVE()
B_SPLINE_CURVE(2,(#71264,#71265,#71266),.UNSPECIFIED.,.F.,.F.)
B_SPLINE_CURVE_WITH_KNOTS((3,3),(0.984623166322171,1.26677639839307),
 .UNSPECIFIED.)
CURVE()
GEOMETRIC_REPRESENTATION_ITEM()
RATIONAL_B_SPLINE_CURVE((1.02072197947249,1.02138328368541,1.02072197947249))
REPRESENTATION_ITEM('')
);
#18871=(
BOUNDED_CURVE()
B_SPLINE_CURVE(2,(#71302,#71303,#71304),.UNSPECIFIED.,.F.,.F.)
B_SPLINE_CURVE_WITH_KNOTS((3,3),(0.,0.0730837266086082),.UNSPECIFIED.)
CURVE()
GEOMETRIC_REPRESENTATION_ITEM()
RATIONAL_B_SPLINE_CURVE((1.,1.00000531285031,1.00000243584542))
REPRESENTATION_ITEM('')
);
#18872=(
BOUNDED_CURVE()
B_SPLINE_CURVE(2,(#71340,#71341,#71342),.UNSPECIFIED.,.F.,.F.)
B_SPLINE_CURVE_WITH_KNOTS((3,3),(0.984623166322171,1.26677639839307),
 .UNSPECIFIED.)
CURVE()
GEOMETRIC_REPRESENTATION_ITEM()
RATIONAL_B_SPLINE_CURVE((1.02072197947249,1.02138328368541,1.02072197947249))
REPRESENTATION_ITEM('')
);
#18873=(
BOUNDED_CURVE()
B_SPLINE_CURVE(2,(#71378,#71379,#71380),.UNSPECIFIED.,.F.,.F.)
B_SPLINE_CURVE_WITH_KNOTS((3,3),(0.,0.0730837266081729),.UNSPECIFIED.)
CURVE()
GEOMETRIC_REPRESENTATION_ITEM()
RATIONAL_B_SPLINE_CURVE((1.,1.00000531281639,1.00000243582987))
REPRESENTATION_ITEM('')
);
#18874=(
BOUNDED_CURVE()
B_SPLINE_CURVE(2,(#71416,#71417,#71418),.UNSPECIFIED.,.F.,.F.)
B_SPLINE_CURVE_WITH_KNOTS((3,3),(0.984623166322171,1.26677639839308),
 .UNSPECIFIED.)
CURVE()
GEOMETRIC_REPRESENTATION_ITEM()
RATIONAL_B_SPLINE_CURVE((1.02072197947249,1.02138328368541,1.02072197947249))
REPRESENTATION_ITEM('')
);
#18875=(
BOUNDED_CURVE()
B_SPLINE_CURVE(2,(#71454,#71455,#71456),.UNSPECIFIED.,.F.,.F.)
B_SPLINE_CURVE_WITH_KNOTS((3,3),(0.,0.0730837266083873),.UNSPECIFIED.)
CURVE()
GEOMETRIC_REPRESENTATION_ITEM()
RATIONAL_B_SPLINE_CURVE((1.,1.00000531281801,1.00000243583061))
REPRESENTATION_ITEM('')
);
#18876=(
BOUNDED_CURVE()
B_SPLINE_CURVE(2,(#71492,#71493,#71494),.UNSPECIFIED.,.F.,.F.)
B_SPLINE_CURVE_WITH_KNOTS((3,3),(0.984623166322171,1.26677639839307),
 .UNSPECIFIED.)
CURVE()
GEOMETRIC_REPRESENTATION_ITEM()
RATIONAL_B_SPLINE_CURVE((1.02072197947249,1.02138328368541,1.02072197947249))
REPRESENTATION_ITEM('')
);
#18877=(
BOUNDED_CURVE()
B_SPLINE_CURVE(2,(#71530,#71531,#71532),.UNSPECIFIED.,.F.,.F.)
B_SPLINE_CURVE_WITH_KNOTS((3,3),(0.,0.0730837266086276),.UNSPECIFIED.)
CURVE()
GEOMETRIC_REPRESENTATION_ITEM()
RATIONAL_B_SPLINE_CURVE((1.,1.00000531283797,1.00000243583976))
REPRESENTATION_ITEM('')
);
#18878=(
BOUNDED_CURVE()
B_SPLINE_CURVE(2,(#71540,#71541,#71542),.UNSPECIFIED.,.F.,.F.)
B_SPLINE_CURVE_WITH_KNOTS((3,3),(0.0522192481407343,0.300149053231598),
 .UNSPECIFIED.)
CURVE()
GEOMETRIC_REPRESENTATION_ITEM()
RATIONAL_B_SPLINE_CURVE((1.00002415803369,1.00006942852683,1.))
REPRESENTATION_ITEM('')
);
#18879=(
BOUNDED_CURVE()
B_SPLINE_CURVE(2,(#71543,#71544,#71545),.UNSPECIFIED.,.F.,.F.)
B_SPLINE_CURVE_WITH_KNOTS((3,3),(0.,0.247929805090937),.UNSPECIFIED.)
CURVE()
GEOMETRIC_REPRESENTATION_ITEM()
RATIONAL_B_SPLINE_CURVE((1.,1.00006942853014,1.00002415803485))
REPRESENTATION_ITEM('')
);
#18880=(
BOUNDED_CURVE()
B_SPLINE_CURVE(2,(#71550,#71551,#71552),.UNSPECIFIED.,.F.,.F.)
B_SPLINE_CURVE_WITH_KNOTS((3,3),(0.0522192481406321,0.300149053231599),
 .UNSPECIFIED.)
CURVE()
GEOMETRIC_REPRESENTATION_ITEM()
RATIONAL_B_SPLINE_CURVE((1.00002415803476,1.00006942852989,1.))
REPRESENTATION_ITEM('')
);
#18881=(
BOUNDED_CURVE()
B_SPLINE_CURVE(2,(#71553,#71554,#71555),.UNSPECIFIED.,.F.,.F.)
B_SPLINE_CURVE_WITH_KNOTS((3,3),(0.,0.247929805090946),.UNSPECIFIED.)
CURVE()
GEOMETRIC_REPRESENTATION_ITEM()
RATIONAL_B_SPLINE_CURVE((1.,1.00006942853077,1.00002415803506))
REPRESENTATION_ITEM('')
);
#18882=(
BOUNDED_CURVE()
B_SPLINE_CURVE(2,(#71560,#71561,#71562),.UNSPECIFIED.,.F.,.F.)
B_SPLINE_CURVE_WITH_KNOTS((3,3),(0.0522192481406271,0.300149053231598),
 .UNSPECIFIED.)
CURVE()
GEOMETRIC_REPRESENTATION_ITEM()
RATIONAL_B_SPLINE_CURVE((1.00002415803463,1.00006942852952,1.))
REPRESENTATION_ITEM('')
);
#18883=(
BOUNDED_CURVE()
B_SPLINE_CURVE(2,(#71563,#71564,#71565),.UNSPECIFIED.,.F.,.F.)
B_SPLINE_CURVE_WITH_KNOTS((3,3),(0.,0.247929805090861),.UNSPECIFIED.)
CURVE()
GEOMETRIC_REPRESENTATION_ITEM()
RATIONAL_B_SPLINE_CURVE((1.,1.00006942852808,1.00002415803413))
REPRESENTATION_ITEM('')
);
#18884=(
BOUNDED_CURVE()
B_SPLINE_CURVE(2,(#71570,#71571,#71572),.UNSPECIFIED.,.F.,.F.)
B_SPLINE_CURVE_WITH_KNOTS((3,3),(0.0522192481407297,0.300149053231598),
 .UNSPECIFIED.)
CURVE()
GEOMETRIC_REPRESENTATION_ITEM()
RATIONAL_B_SPLINE_CURVE((1.00002415803409,1.00006942852797,1.))
REPRESENTATION_ITEM('')
);
#18885=(
BOUNDED_CURVE()
B_SPLINE_CURVE(2,(#71573,#71574,#71575),.UNSPECIFIED.,.F.,.F.)
B_SPLINE_CURVE_WITH_KNOTS((3,3),(0.,0.247929805090852),.UNSPECIFIED.)
CURVE()
GEOMETRIC_REPRESENTATION_ITEM()
RATIONAL_B_SPLINE_CURVE((1.,1.00006942852787,1.00002415803405))
REPRESENTATION_ITEM('')
);
#18886=(
BOUNDED_CURVE()
B_SPLINE_CURVE(2,(#71580,#71581,#71582),.UNSPECIFIED.,.F.,.F.)
B_SPLINE_CURVE_WITH_KNOTS((3,3),(0.0522192481407573,0.300149053231599),
 .UNSPECIFIED.)
CURVE()
GEOMETRIC_REPRESENTATION_ITEM()
RATIONAL_B_SPLINE_CURVE((1.00002415803393,1.00006942852751,1.))
REPRESENTATION_ITEM('')
);
#18887=(
BOUNDED_CURVE()
B_SPLINE_CURVE(2,(#71583,#71584,#71585),.UNSPECIFIED.,.F.,.F.)
B_SPLINE_CURVE_WITH_KNOTS((3,3),(0.,0.247929805090877),.UNSPECIFIED.)
CURVE()
GEOMETRIC_REPRESENTATION_ITEM()
RATIONAL_B_SPLINE_CURVE((1.,1.00006942852796,1.00002415803409))
REPRESENTATION_ITEM('')
);
#18888=(
BOUNDED_CURVE()
B_SPLINE_CURVE(2,(#71590,#71591,#71592),.UNSPECIFIED.,.F.,.F.)
B_SPLINE_CURVE_WITH_KNOTS((3,3),(0.0522192481406628,0.300149053231599),
 .UNSPECIFIED.)
CURVE()
GEOMETRIC_REPRESENTATION_ITEM()
RATIONAL_B_SPLINE_CURVE((1.00002415803503,1.00006942853066,1.))
REPRESENTATION_ITEM('')
);
#18889=(
BOUNDED_CURVE()
B_SPLINE_CURVE(2,(#71593,#71594,#71595),.UNSPECIFIED.,.F.,.F.)
B_SPLINE_CURVE_WITH_KNOTS((3,3),(0.,0.247929805090816),.UNSPECIFIED.)
CURVE()
GEOMETRIC_REPRESENTATION_ITEM()
RATIONAL_B_SPLINE_CURVE((1.,1.00006942852647,1.00002415803357))
REPRESENTATION_ITEM('')
);
#18890=(
BOUNDED_CURVE()
B_SPLINE_CURVE(2,(#71600,#71601,#71602),.UNSPECIFIED.,.F.,.F.)
B_SPLINE_CURVE_WITH_KNOTS((3,3),(0.0522192481406917,0.300149053231598),
 .UNSPECIFIED.)
CURVE()
GEOMETRIC_REPRESENTATION_ITEM()
RATIONAL_B_SPLINE_CURVE((1.0000241580342,1.00006942852828,1.))
REPRESENTATION_ITEM('')
);
#18891=(
BOUNDED_CURVE()
B_SPLINE_CURVE(2,(#71603,#71604,#71605),.UNSPECIFIED.,.F.,.F.)
B_SPLINE_CURVE_WITH_KNOTS((3,3),(0.,0.247929805090809),.UNSPECIFIED.)
CURVE()
GEOMETRIC_REPRESENTATION_ITEM()
RATIONAL_B_SPLINE_CURVE((1.,1.0000694285267,1.00002415803365))
REPRESENTATION_ITEM('')
);
#18892=(
BOUNDED_CURVE()
B_SPLINE_CURVE(2,(#71610,#71611,#71612),.UNSPECIFIED.,.F.,.F.)
B_SPLINE_CURVE_WITH_KNOTS((3,3),(0.0522192481406725,0.300149053231599),
 .UNSPECIFIED.)
CURVE()
GEOMETRIC_REPRESENTATION_ITEM()
RATIONAL_B_SPLINE_CURVE((1.00002415803451,1.00006942852917,1.))
REPRESENTATION_ITEM('')
);
#18893=(
BOUNDED_CURVE()
B_SPLINE_CURVE(2,(#71613,#71614,#71615),.UNSPECIFIED.,.F.,.F.)
B_SPLINE_CURVE_WITH_KNOTS((3,3),(0.,0.247929805090887),.UNSPECIFIED.)
CURVE()
GEOMETRIC_REPRESENTATION_ITEM()
RATIONAL_B_SPLINE_CURVE((1.,1.00006942852972,1.0000241580347))
REPRESENTATION_ITEM('')
);
#18894=(
BOUNDED_CURVE()
B_SPLINE_CURVE(2,(#71620,#71621,#71622),.UNSPECIFIED.,.F.,.F.)
B_SPLINE_CURVE_WITH_KNOTS((3,3),(0.0522192481407858,0.300149053231598),
 .UNSPECIFIED.)
CURVE()
GEOMETRIC_REPRESENTATION_ITEM()
RATIONAL_B_SPLINE_CURVE((1.00002415803371,1.00006942852687,1.))
REPRESENTATION_ITEM('')
);
#18895=(
BOUNDED_CURVE()
B_SPLINE_CURVE(2,(#71623,#71624,#71625),.UNSPECIFIED.,.F.,.F.)
B_SPLINE_CURVE_WITH_KNOTS((3,3),(0.,0.247929805090891),.UNSPECIFIED.)
CURVE()
GEOMETRIC_REPRESENTATION_ITEM()
RATIONAL_B_SPLINE_CURVE((1.,1.00006942852915,1.0000241580345))
REPRESENTATION_ITEM('')
);
#18896=(
BOUNDED_CURVE()
B_SPLINE_CURVE(2,(#71630,#71631,#71632),.UNSPECIFIED.,.F.,.F.)
B_SPLINE_CURVE_WITH_KNOTS((3,3),(0.0522192481406479,0.300149053231599),
 .UNSPECIFIED.)
CURVE()
GEOMETRIC_REPRESENTATION_ITEM()
RATIONAL_B_SPLINE_CURVE((1.0000241580347,1.00006942852973,1.))
REPRESENTATION_ITEM('')
);
#18897=(
BOUNDED_CURVE()
B_SPLINE_CURVE(2,(#71633,#71634,#71635),.UNSPECIFIED.,.F.,.F.)
B_SPLINE_CURVE_WITH_KNOTS((3,3),(0.,0.24792980509089),.UNSPECIFIED.)
CURVE()
GEOMETRIC_REPRESENTATION_ITEM()
RATIONAL_B_SPLINE_CURVE((1.,1.0000694285297,1.00002415803469))
REPRESENTATION_ITEM('')
);
#18898=(
BOUNDED_CURVE()
B_SPLINE_CURVE(2,(#71640,#71641,#71642),.UNSPECIFIED.,.F.,.F.)
B_SPLINE_CURVE_WITH_KNOTS((3,3),(0.0522192481407442,0.300149053231599),
 .UNSPECIFIED.)
CURVE()
GEOMETRIC_REPRESENTATION_ITEM()
RATIONAL_B_SPLINE_CURVE((1.00002415803411,1.00006942852801,1.))
REPRESENTATION_ITEM('')
);
#18899=(
BOUNDED_CURVE()
B_SPLINE_CURVE(2,(#71643,#71644,#71645),.UNSPECIFIED.,.F.,.F.)
B_SPLINE_CURVE_WITH_KNOTS((3,3),(0.,0.247929805090961),.UNSPECIFIED.)
CURVE()
GEOMETRIC_REPRESENTATION_ITEM()
RATIONAL_B_SPLINE_CURVE((1.,1.00006942852871,1.00002415803435))
REPRESENTATION_ITEM('')
);
#18900=(
BOUNDED_CURVE()
B_SPLINE_CURVE(2,(#71650,#71651,#71652),.UNSPECIFIED.,.F.,.F.)
B_SPLINE_CURVE_WITH_KNOTS((3,3),(0.0522192481406183,0.300149053231598),
 .UNSPECIFIED.)
CURVE()
GEOMETRIC_REPRESENTATION_ITEM()
RATIONAL_B_SPLINE_CURVE((1.0000241580348,1.00006942853,1.))
REPRESENTATION_ITEM('')
);
#18901=(
BOUNDED_CURVE()
B_SPLINE_CURVE(2,(#71653,#71654,#71655),.UNSPECIFIED.,.F.,.F.)
B_SPLINE_CURVE_WITH_KNOTS((3,3),(0.,0.247929805090888),.UNSPECIFIED.)
CURVE()
GEOMETRIC_REPRESENTATION_ITEM()
RATIONAL_B_SPLINE_CURVE((1.,1.00006942852642,1.00002415803355))
REPRESENTATION_ITEM('')
);
#18902=(
BOUNDED_CURVE()
B_SPLINE_CURVE(2,(#71660,#71661,#71662),.UNSPECIFIED.,.F.,.F.)
B_SPLINE_CURVE_WITH_KNOTS((3,3),(0.0522192481406737,0.300149053231598),
 .UNSPECIFIED.)
CURVE()
GEOMETRIC_REPRESENTATION_ITEM()
RATIONAL_B_SPLINE_CURVE((1.00002415803462,1.00006942852949,1.))
REPRESENTATION_ITEM('')
);
#18903=(
BOUNDED_CURVE()
B_SPLINE_CURVE(2,(#71663,#71664,#71665),.UNSPECIFIED.,.F.,.F.)
B_SPLINE_CURVE_WITH_KNOTS((3,3),(0.,0.247929805090943),.UNSPECIFIED.)
CURVE()
GEOMETRIC_REPRESENTATION_ITEM()
RATIONAL_B_SPLINE_CURVE((1.,1.00006942852869,1.00002415803434))
REPRESENTATION_ITEM('')
);
#18904=(
BOUNDED_CURVE()
B_SPLINE_CURVE(2,(#71670,#71671,#71672),.UNSPECIFIED.,.F.,.F.)
B_SPLINE_CURVE_WITH_KNOTS((3,3),(0.0522192481407655,0.300149053231599),
 .UNSPECIFIED.)
CURVE()
GEOMETRIC_REPRESENTATION_ITEM()
RATIONAL_B_SPLINE_CURVE((1.00002415803309,1.00006942852508,1.))
REPRESENTATION_ITEM('')
);
#18905=(
BOUNDED_CURVE()
B_SPLINE_CURVE(2,(#71673,#71674,#71675),.UNSPECIFIED.,.F.,.F.)
B_SPLINE_CURVE_WITH_KNOTS((3,3),(0.,0.247929805090823),.UNSPECIFIED.)
CURVE()
GEOMETRIC_REPRESENTATION_ITEM()
RATIONAL_B_SPLINE_CURVE((1.,1.00006942852759,1.00002415803396))
REPRESENTATION_ITEM('')
);
#18906=(
BOUNDED_CURVE()
B_SPLINE_CURVE(2,(#71680,#71681,#71682),.UNSPECIFIED.,.F.,.F.)
B_SPLINE_CURVE_WITH_KNOTS((3,3),(0.0522192481406535,0.300149053231599),
 .UNSPECIFIED.)
CURVE()
GEOMETRIC_REPRESENTATION_ITEM()
RATIONAL_B_SPLINE_CURVE((1.0000241580346,1.00006942852943,1.))
REPRESENTATION_ITEM('')
);
#18907=(
BOUNDED_CURVE()
B_SPLINE_CURVE(2,(#71683,#71684,#71685),.UNSPECIFIED.,.F.,.F.)
B_SPLINE_CURVE_WITH_KNOTS((3,3),(0.,0.247929805090934),.UNSPECIFIED.)
CURVE()
GEOMETRIC_REPRESENTATION_ITEM()
RATIONAL_B_SPLINE_CURVE((1.,1.00006942852716,1.00002415803381))
REPRESENTATION_ITEM('')
);
#18908=(
BOUNDED_CURVE()
B_SPLINE_CURVE(2,(#71690,#71691,#71692),.UNSPECIFIED.,.F.,.F.)
B_SPLINE_CURVE_WITH_KNOTS((3,3),(0.0522192481407335,0.300149053231598),
 .UNSPECIFIED.)
CURVE()
GEOMETRIC_REPRESENTATION_ITEM()
RATIONAL_B_SPLINE_CURVE((1.00002415803399,1.00006942852769,1.))
REPRESENTATION_ITEM('')
);
#18909=(
BOUNDED_CURVE()
B_SPLINE_CURVE(2,(#71693,#71694,#71695),.UNSPECIFIED.,.F.,.F.)
B_SPLINE_CURVE_WITH_KNOTS((3,3),(0.,0.247929805090796),.UNSPECIFIED.)
CURVE()
GEOMETRIC_REPRESENTATION_ITEM()
RATIONAL_B_SPLINE_CURVE((1.,1.00006942852549,1.00002415803323))
REPRESENTATION_ITEM('')
);
#18910=(
BOUNDED_CURVE()
B_SPLINE_CURVE(2,(#71700,#71701,#71702),.UNSPECIFIED.,.F.,.F.)
B_SPLINE_CURVE_WITH_KNOTS((3,3),(0.0522192481408277,0.300149053231598),
 .UNSPECIFIED.)
CURVE()
GEOMETRIC_REPRESENTATION_ITEM()
RATIONAL_B_SPLINE_CURVE((1.00002415803309,1.00006942852509,1.))
REPRESENTATION_ITEM('')
);
#18911=(
BOUNDED_CURVE()
B_SPLINE_CURVE(2,(#71703,#71704,#71705),.UNSPECIFIED.,.F.,.F.)
B_SPLINE_CURVE_WITH_KNOTS((3,3),(0.,0.247929805090907),.UNSPECIFIED.)
CURVE()
GEOMETRIC_REPRESENTATION_ITEM()
RATIONAL_B_SPLINE_CURVE((1.,1.00006942852842,1.00002415803425))
REPRESENTATION_ITEM('')
);
#18912=(
BOUNDED_CURVE()
B_SPLINE_CURVE(2,(#71710,#71711,#71712),.UNSPECIFIED.,.F.,.F.)
B_SPLINE_CURVE_WITH_KNOTS((3,3),(0.0522192481406971,0.300149053231598),
 .UNSPECIFIED.)
CURVE()
GEOMETRIC_REPRESENTATION_ITEM()
RATIONAL_B_SPLINE_CURVE((1.00002415803424,1.00006942852841,1.))
REPRESENTATION_ITEM('')
);
#18913=(
BOUNDED_CURVE()
B_SPLINE_CURVE(2,(#71713,#71714,#71715),.UNSPECIFIED.,.F.,.F.)
B_SPLINE_CURVE_WITH_KNOTS((3,3),(0.,0.247929805090908),.UNSPECIFIED.)
CURVE()
GEOMETRIC_REPRESENTATION_ITEM()
RATIONAL_B_SPLINE_CURVE((1.,1.00006942852784,1.00002415803404))
REPRESENTATION_ITEM('')
);
#18914=(
BOUNDED_CURVE()
B_SPLINE_CURVE(2,(#71720,#71721,#71722),.UNSPECIFIED.,.F.,.F.)
B_SPLINE_CURVE_WITH_KNOTS((3,3),(0.0522192481407081,0.300149053231599),
 .UNSPECIFIED.)
CURVE()
GEOMETRIC_REPRESENTATION_ITEM()
RATIONAL_B_SPLINE_CURVE((1.00002415803401,1.00006942852773,1.))
REPRESENTATION_ITEM('')
);
#18915=(
BOUNDED_CURVE()
B_SPLINE_CURVE(2,(#71723,#71724,#71725),.UNSPECIFIED.,.F.,.F.)
B_SPLINE_CURVE_WITH_KNOTS((3,3),(0.,0.247929805090776),.UNSPECIFIED.)
CURVE()
GEOMETRIC_REPRESENTATION_ITEM()
RATIONAL_B_SPLINE_CURVE((1.,1.00006942852821,1.00002415803417))
REPRESENTATION_ITEM('')
);
#18916=(
BOUNDED_CURVE()
B_SPLINE_CURVE(2,(#71730,#71731,#71732),.UNSPECIFIED.,.F.,.F.)
B_SPLINE_CURVE_WITH_KNOTS((3,3),(0.0522192481407325,0.300149053231599),
 .UNSPECIFIED.)
CURVE()
GEOMETRIC_REPRESENTATION_ITEM()
RATIONAL_B_SPLINE_CURVE((1.00002415803403,1.0000694285278,1.))
REPRESENTATION_ITEM('')
);
#18917=(
BOUNDED_CURVE()
B_SPLINE_CURVE(2,(#71733,#71734,#71735),.UNSPECIFIED.,.F.,.F.)
B_SPLINE_CURVE_WITH_KNOTS((3,3),(0.,0.24792980509088),.UNSPECIFIED.)
CURVE()
GEOMETRIC_REPRESENTATION_ITEM()
RATIONAL_B_SPLINE_CURVE((1.,1.00006942852859,1.00002415803431))
REPRESENTATION_ITEM('')
);
#18918=(
BOUNDED_CURVE()
B_SPLINE_CURVE(2,(#71740,#71741,#71742),.UNSPECIFIED.,.F.,.F.)
B_SPLINE_CURVE_WITH_KNOTS((3,3),(0.0522192481407089,0.300149053231599),
 .UNSPECIFIED.)
CURVE()
GEOMETRIC_REPRESENTATION_ITEM()
RATIONAL_B_SPLINE_CURVE((1.00002415803469,1.00006942852969,1.))
REPRESENTATION_ITEM('')
);
#18919=(
BOUNDED_CURVE()
B_SPLINE_CURVE(2,(#71743,#71744,#71745),.UNSPECIFIED.,.F.,.F.)
B_SPLINE_CURVE_WITH_KNOTS((3,3),(0.,0.24792980509083),.UNSPECIFIED.)
CURVE()
GEOMETRIC_REPRESENTATION_ITEM()
RATIONAL_B_SPLINE_CURVE((1.,1.00006942852682,1.00002415803369))
REPRESENTATION_ITEM('')
);
#18920=(
BOUNDED_CURVE()
B_SPLINE_CURVE(2,(#71750,#71751,#71752),.UNSPECIFIED.,.F.,.F.)
B_SPLINE_CURVE_WITH_KNOTS((3,3),(0.0522192481406734,0.300149053231598),
 .UNSPECIFIED.)
CURVE()
GEOMETRIC_REPRESENTATION_ITEM()
RATIONAL_B_SPLINE_CURVE((1.00002415803462,1.0000694285295,1.))
REPRESENTATION_ITEM('')
);
#18921=(
BOUNDED_CURVE()
B_SPLINE_CURVE(2,(#71753,#71754,#71755),.UNSPECIFIED.,.F.,.F.)
B_SPLINE_CURVE_WITH_KNOTS((3,3),(0.,0.247929805090843),.UNSPECIFIED.)
CURVE()
GEOMETRIC_REPRESENTATION_ITEM()
RATIONAL_B_SPLINE_CURVE((1.,1.00006942852709,1.00002415803378))
REPRESENTATION_ITEM('')
);
#18922=(
BOUNDED_CURVE()
B_SPLINE_CURVE(2,(#71760,#71761,#71762),.UNSPECIFIED.,.F.,.F.)
B_SPLINE_CURVE_WITH_KNOTS((3,3),(0.0522192481406847,0.300149053231599),
 .UNSPECIFIED.)
CURVE()
GEOMETRIC_REPRESENTATION_ITEM()
RATIONAL_B_SPLINE_CURVE((1.00002415803482,1.00006942853006,1.))
REPRESENTATION_ITEM('')
);
#18923=(
BOUNDED_CURVE()
B_SPLINE_CURVE(2,(#71763,#71764,#71765),.UNSPECIFIED.,.F.,.F.)
B_SPLINE_CURVE_WITH_KNOTS((3,3),(0.,0.247929805090743),.UNSPECIFIED.)
CURVE()
GEOMETRIC_REPRESENTATION_ITEM()
RATIONAL_B_SPLINE_CURVE((1.,1.00006942852572,1.00002415803331))
REPRESENTATION_ITEM('')
);
#18924=(
BOUNDED_CURVE()
B_SPLINE_CURVE(2,(#71770,#71771,#71772),.UNSPECIFIED.,.F.,.F.)
B_SPLINE_CURVE_WITH_KNOTS((3,3),(0.0522192481406775,0.300149053231598),
 .UNSPECIFIED.)
CURVE()
GEOMETRIC_REPRESENTATION_ITEM()
RATIONAL_B_SPLINE_CURVE((1.00002415803416,1.00006942852817,1.))
REPRESENTATION_ITEM('')
);
#18925=(
BOUNDED_CURVE()
B_SPLINE_CURVE(2,(#71773,#71774,#71775),.UNSPECIFIED.,.F.,.F.)
B_SPLINE_CURVE_WITH_KNOTS((3,3),(0.,0.247929805090921),.UNSPECIFIED.)
CURVE()
GEOMETRIC_REPRESENTATION_ITEM()
RATIONAL_B_SPLINE_CURVE((1.,1.00006942852804,1.00002415803411))
REPRESENTATION_ITEM('')
);
#18926=(
BOUNDED_CURVE()
B_SPLINE_CURVE(2,(#71780,#71781,#71782),.UNSPECIFIED.,.F.,.F.)
B_SPLINE_CURVE_WITH_KNOTS((3,3),(0.0522192481406454,0.300149053231599),
 .UNSPECIFIED.)
CURVE()
GEOMETRIC_REPRESENTATION_ITEM()
RATIONAL_B_SPLINE_CURVE((1.0000241580342,1.00006942852828,1.))
REPRESENTATION_ITEM('')
);
#18927=(
BOUNDED_CURVE()
B_SPLINE_CURVE(2,(#71783,#71784,#71785),.UNSPECIFIED.,.F.,.F.)
B_SPLINE_CURVE_WITH_KNOTS((3,3),(0.,0.247929805090911),.UNSPECIFIED.)
CURVE()
GEOMETRIC_REPRESENTATION_ITEM()
RATIONAL_B_SPLINE_CURVE((1.,1.00006942852954,1.00002415803464))
REPRESENTATION_ITEM('')
);
#18928=(
BOUNDED_CURVE()
B_SPLINE_CURVE(2,(#71790,#71791,#71792),.UNSPECIFIED.,.F.,.F.)
B_SPLINE_CURVE_WITH_KNOTS((3,3),(0.0522192481406103,0.300149053231599),
 .UNSPECIFIED.)
CURVE()
GEOMETRIC_REPRESENTATION_ITEM()
RATIONAL_B_SPLINE_CURVE((1.00002415803486,1.00006942853019,1.))
REPRESENTATION_ITEM('')
);
#18929=(
BOUNDED_CURVE()
B_SPLINE_CURVE(2,(#71793,#71794,#71795),.UNSPECIFIED.,.F.,.F.)
B_SPLINE_CURVE_WITH_KNOTS((3,3),(0.,0.247929805090893),.UNSPECIFIED.)
CURVE()
GEOMETRIC_REPRESENTATION_ITEM()
RATIONAL_B_SPLINE_CURVE((1.,1.00006942853005,1.00002415803481))
REPRESENTATION_ITEM('')
);
#18930=(
BOUNDED_CURVE()
B_SPLINE_CURVE(2,(#71800,#71801,#71802),.UNSPECIFIED.,.F.,.F.)
B_SPLINE_CURVE_WITH_KNOTS((3,3),(0.0522192481407398,0.300149053231598),
 .UNSPECIFIED.)
CURVE()
GEOMETRIC_REPRESENTATION_ITEM()
RATIONAL_B_SPLINE_CURVE((1.0000241580337,1.00006942852686,1.))
REPRESENTATION_ITEM('')
);
#18931=(
BOUNDED_CURVE()
B_SPLINE_CURVE(2,(#71803,#71804,#71805),.UNSPECIFIED.,.F.,.F.)
B_SPLINE_CURVE_WITH_KNOTS((3,3),(0.,0.247929805090968),.UNSPECIFIED.)
CURVE()
GEOMETRIC_REPRESENTATION_ITEM()
RATIONAL_B_SPLINE_CURVE((1.,1.00006942852967,1.00002415803468))
REPRESENTATION_ITEM('')
);
#18932=(
BOUNDED_CURVE()
B_SPLINE_CURVE(2,(#71810,#71811,#71812),.UNSPECIFIED.,.F.,.F.)
B_SPLINE_CURVE_WITH_KNOTS((3,3),(0.0522192481406895,0.300149053231599),
 .UNSPECIFIED.)
CURVE()
GEOMETRIC_REPRESENTATION_ITEM()
RATIONAL_B_SPLINE_CURVE((1.00002415803463,1.00006942852952,1.))
REPRESENTATION_ITEM('')
);
#18933=(
BOUNDED_CURVE()
B_SPLINE_CURVE(2,(#71813,#71814,#71815),.UNSPECIFIED.,.F.,.F.)
B_SPLINE_CURVE_WITH_KNOTS((3,3),(0.,0.247929805090878),.UNSPECIFIED.)
CURVE()
GEOMETRIC_REPRESENTATION_ITEM()
RATIONAL_B_SPLINE_CURVE((1.,1.00006942852936,1.00002415803458))
REPRESENTATION_ITEM('')
);
#18934=(
BOUNDED_CURVE()
B_SPLINE_CURVE(2,(#71820,#71821,#71822),.UNSPECIFIED.,.F.,.F.)
B_SPLINE_CURVE_WITH_KNOTS((3,3),(0.0522192481406974,0.300149053231598),
 .UNSPECIFIED.)
CURVE()
GEOMETRIC_REPRESENTATION_ITEM()
RATIONAL_B_SPLINE_CURVE((1.00002415803451,1.00006942852919,1.))
REPRESENTATION_ITEM('')
);
#18935=(
BOUNDED_CURVE()
B_SPLINE_CURVE(2,(#71823,#71824,#71825),.UNSPECIFIED.,.F.,.F.)
B_SPLINE_CURVE_WITH_KNOTS((3,3),(0.,0.247929805090898),.UNSPECIFIED.)
CURVE()
GEOMETRIC_REPRESENTATION_ITEM()
RATIONAL_B_SPLINE_CURVE((1.,1.00006942852895,1.00002415803443))
REPRESENTATION_ITEM('')
);
#18936=(
BOUNDED_CURVE()
B_SPLINE_CURVE(2,(#71830,#71831,#71832),.UNSPECIFIED.,.F.,.F.)
B_SPLINE_CURVE_WITH_KNOTS((3,3),(0.0522192481407298,0.300149053231598),
 .UNSPECIFIED.)
CURVE()
GEOMETRIC_REPRESENTATION_ITEM()
RATIONAL_B_SPLINE_CURVE((1.00002415803412,1.00006942852805,1.))
REPRESENTATION_ITEM('')
);
#18937=(
BOUNDED_CURVE()
B_SPLINE_CURVE(2,(#71833,#71834,#71835),.UNSPECIFIED.,.F.,.F.)
B_SPLINE_CURVE_WITH_KNOTS((3,3),(0.,0.247929805090915),.UNSPECIFIED.)
CURVE()
GEOMETRIC_REPRESENTATION_ITEM()
RATIONAL_B_SPLINE_CURVE((1.,1.00006942852918,1.00002415803451))
REPRESENTATION_ITEM('')
);
#18938=(
BOUNDED_CURVE()
B_SPLINE_CURVE(2,(#71840,#71841,#71842),.UNSPECIFIED.,.F.,.F.)
B_SPLINE_CURVE_WITH_KNOTS((3,3),(0.0522192481407133,0.300149053231598),
 .UNSPECIFIED.)
CURVE()
GEOMETRIC_REPRESENTATION_ITEM()
RATIONAL_B_SPLINE_CURVE((1.00002415803458,1.00006942852939,1.))
REPRESENTATION_ITEM('')
);
#18939=(
BOUNDED_CURVE()
B_SPLINE_CURVE(2,(#71843,#71844,#71845),.UNSPECIFIED.,.F.,.F.)
B_SPLINE_CURVE_WITH_KNOTS((3,3),(0.,0.247929805090875),.UNSPECIFIED.)
CURVE()
GEOMETRIC_REPRESENTATION_ITEM()
RATIONAL_B_SPLINE_CURVE((1.,1.00006942852786,1.00002415803405))
REPRESENTATION_ITEM('')
);
#18940=(
BOUNDED_CURVE()
B_SPLINE_CURVE(2,(#71850,#71851,#71852),.UNSPECIFIED.,.F.,.F.)
B_SPLINE_CURVE_WITH_KNOTS((3,3),(0.0522192481407655,0.300149053231599),
 .UNSPECIFIED.)
CURVE()
GEOMETRIC_REPRESENTATION_ITEM()
RATIONAL_B_SPLINE_CURVE((1.00002415803309,1.00006942852508,1.))
REPRESENTATION_ITEM('')
);
#18941=(
BOUNDED_CURVE()
B_SPLINE_CURVE(2,(#71853,#71854,#71855),.UNSPECIFIED.,.F.,.F.)
B_SPLINE_CURVE_WITH_KNOTS((3,3),(0.,0.247929805090823),.UNSPECIFIED.)
CURVE()
GEOMETRIC_REPRESENTATION_ITEM()
RATIONAL_B_SPLINE_CURVE((1.,1.00006942852759,1.00002415803396))
REPRESENTATION_ITEM('')
);
#18942=(
BOUNDED_CURVE()
B_SPLINE_CURVE(2,(#71860,#71861,#71862),.UNSPECIFIED.,.F.,.F.)
B_SPLINE_CURVE_WITH_KNOTS((3,3),(0.0522192481406882,0.300149053231598),
 .UNSPECIFIED.)
CURVE()
GEOMETRIC_REPRESENTATION_ITEM()
RATIONAL_B_SPLINE_CURVE((1.00002415803415,1.00006942852814,1.))
REPRESENTATION_ITEM('')
);
#18943=(
BOUNDED_CURVE()
B_SPLINE_CURVE(2,(#71863,#71864,#71865),.UNSPECIFIED.,.F.,.F.)
B_SPLINE_CURVE_WITH_KNOTS((3,3),(0.,0.247929805090945),.UNSPECIFIED.)
CURVE()
GEOMETRIC_REPRESENTATION_ITEM()
RATIONAL_B_SPLINE_CURVE((1.,1.00006942852919,1.00002415803451))
REPRESENTATION_ITEM('')
);
#18944=(
BOUNDED_CURVE()
B_SPLINE_CURVE(2,(#71870,#71871,#71872),.UNSPECIFIED.,.F.,.F.)
B_SPLINE_CURVE_WITH_KNOTS((3,3),(0.0522192481406479,0.300149053231598),
 .UNSPECIFIED.)
CURVE()
GEOMETRIC_REPRESENTATION_ITEM()
RATIONAL_B_SPLINE_CURVE((1.00002415803429,1.00006942852855,1.))
REPRESENTATION_ITEM('')
);
#18945=(
BOUNDED_CURVE()
B_SPLINE_CURVE(2,(#71873,#71874,#71875),.UNSPECIFIED.,.F.,.F.)
B_SPLINE_CURVE_WITH_KNOTS((3,3),(0.,0.2479298050909),.UNSPECIFIED.)
CURVE()
GEOMETRIC_REPRESENTATION_ITEM()
RATIONAL_B_SPLINE_CURVE((1.,1.00006942852908,1.00002415803448))
REPRESENTATION_ITEM('')
);
#18946=(
BOUNDED_CURVE()
B_SPLINE_CURVE(2,(#71880,#71881,#71882),.UNSPECIFIED.,.F.,.F.)
B_SPLINE_CURVE_WITH_KNOTS((3,3),(0.052219248140666,0.300149053231598),
 .UNSPECIFIED.)
CURVE()
GEOMETRIC_REPRESENTATION_ITEM()
RATIONAL_B_SPLINE_CURVE((1.0000241580347,1.00006942852973,1.))
REPRESENTATION_ITEM('')
);
#18947=(
BOUNDED_CURVE()
B_SPLINE_CURVE(2,(#71883,#71884,#71885),.UNSPECIFIED.,.F.,.F.)
B_SPLINE_CURVE_WITH_KNOTS((3,3),(0.,0.247929805090926),.UNSPECIFIED.)
CURVE()
GEOMETRIC_REPRESENTATION_ITEM()
RATIONAL_B_SPLINE_CURVE((1.,1.00006942852844,1.00002415803425))
REPRESENTATION_ITEM('')
);
#18948=(
BOUNDED_CURVE()
B_SPLINE_CURVE(2,(#71890,#71891,#71892),.UNSPECIFIED.,.F.,.F.)
B_SPLINE_CURVE_WITH_KNOTS((3,3),(0.05221924814067,0.300149053231598),
 .UNSPECIFIED.)
CURVE()
GEOMETRIC_REPRESENTATION_ITEM()
RATIONAL_B_SPLINE_CURVE((1.0000241580343,1.00006942852856,1.))
REPRESENTATION_ITEM('')
);
#18949=(
BOUNDED_CURVE()
B_SPLINE_CURVE(2,(#71893,#71894,#71895),.UNSPECIFIED.,.F.,.F.)
B_SPLINE_CURVE_WITH_KNOTS((3,3),(0.,0.247929805090796),.UNSPECIFIED.)
CURVE()
GEOMETRIC_REPRESENTATION_ITEM()
RATIONAL_B_SPLINE_CURVE((1.,1.0000694285271,1.00002415803379))
REPRESENTATION_ITEM('')
);
#18950=(
BOUNDED_CURVE()
B_SPLINE_CURVE(2,(#71902,#71903,#71904),.UNSPECIFIED.,.F.,.F.)
B_SPLINE_CURVE_WITH_KNOTS((3,3),(0.,0.0730837266077788),.UNSPECIFIED.)
CURVE()
GEOMETRIC_REPRESENTATION_ITEM()
RATIONAL_B_SPLINE_CURVE((1.,1.00000531280199,1.00000243582326))
REPRESENTATION_ITEM('')
);
#18951=(
BOUNDED_CURVE()
B_SPLINE_CURVE(2,(#71914,#71915,#71916),.UNSPECIFIED.,.F.,.F.)
B_SPLINE_CURVE_WITH_KNOTS((3,3),(0.,0.0730837266081571),.UNSPECIFIED.)
CURVE()
GEOMETRIC_REPRESENTATION_ITEM()
RATIONAL_B_SPLINE_CURVE((1.,1.00000531282708,1.00000243583477))
REPRESENTATION_ITEM('')
);
#18952=(
BOUNDED_CURVE()
B_SPLINE_CURVE(2,(#71926,#71927,#71928),.UNSPECIFIED.,.F.,.F.)
B_SPLINE_CURVE_WITH_KNOTS((3,3),(0.,0.0730837266086552),.UNSPECIFIED.)
CURVE()
GEOMETRIC_REPRESENTATION_ITEM()
RATIONAL_B_SPLINE_CURVE((1.,1.00000531285702,1.0000024358485))
REPRESENTATION_ITEM('')
);
#18953=(
BOUNDED_CURVE()
B_SPLINE_CURVE(2,(#71938,#71939,#71940),.UNSPECIFIED.,.F.,.F.)
B_SPLINE_CURVE_WITH_KNOTS((3,3),(0.,0.0730837266083511),.UNSPECIFIED.)
CURVE()
GEOMETRIC_REPRESENTATION_ITEM()
RATIONAL_B_SPLINE_CURVE((1.,1.00000531283583,1.00000243583878))
REPRESENTATION_ITEM('')
);
#18954=(
BOUNDED_CURVE()
B_SPLINE_CURVE(2,(#71950,#71951,#71952),.UNSPECIFIED.,.F.,.F.)
B_SPLINE_CURVE_WITH_KNOTS((3,3),(0.,0.0730837266086366),.UNSPECIFIED.)
CURVE()
GEOMETRIC_REPRESENTATION_ITEM()
RATIONAL_B_SPLINE_CURVE((1.,1.00000531282378,1.00000243583325))
REPRESENTATION_ITEM('')
);
#18955=(
BOUNDED_CURVE()
B_SPLINE_CURVE(2,(#71962,#71963,#71964),.UNSPECIFIED.,.F.,.F.)
B_SPLINE_CURVE_WITH_KNOTS((3,3),(0.,0.0730837266082308),.UNSPECIFIED.)
CURVE()
GEOMETRIC_REPRESENTATION_ITEM()
RATIONAL_B_SPLINE_CURVE((1.,1.00000531281989,1.00000243583147))
REPRESENTATION_ITEM('')
);
#18956=(
BOUNDED_CURVE()
B_SPLINE_CURVE(2,(#71974,#71975,#71976),.UNSPECIFIED.,.F.,.F.)
B_SPLINE_CURVE_WITH_KNOTS((3,3),(0.,0.0730837266084392),.UNSPECIFIED.)
CURVE()
GEOMETRIC_REPRESENTATION_ITEM()
RATIONAL_B_SPLINE_CURVE((1.,1.00000531283989,1.00000243584064))
REPRESENTATION_ITEM('')
);
#18957=(
BOUNDED_CURVE()
B_SPLINE_CURVE(2,(#71986,#71987,#71988),.UNSPECIFIED.,.F.,.F.)
B_SPLINE_CURVE_WITH_KNOTS((3,3),(0.,0.0730837266081689),.UNSPECIFIED.)
CURVE()
GEOMETRIC_REPRESENTATION_ITEM()
RATIONAL_B_SPLINE_CURVE((1.,1.00000531283784,1.0000024358397))
REPRESENTATION_ITEM('')
);
#18958=(
BOUNDED_CURVE()
B_SPLINE_CURVE(2,(#71998,#71999,#72000),.UNSPECIFIED.,.F.,.F.)
B_SPLINE_CURVE_WITH_KNOTS((3,3),(0.,0.0730837266082052),.UNSPECIFIED.)
CURVE()
GEOMETRIC_REPRESENTATION_ITEM()
RATIONAL_B_SPLINE_CURVE((1.,1.00000531284527,1.00000243584311))
REPRESENTATION_ITEM('')
);
#18959=(
BOUNDED_CURVE()
B_SPLINE_CURVE(2,(#72010,#72011,#72012),.UNSPECIFIED.,.F.,.F.)
B_SPLINE_CURVE_WITH_KNOTS((3,3),(0.,0.0730837266083936),.UNSPECIFIED.)
CURVE()
GEOMETRIC_REPRESENTATION_ITEM()
RATIONAL_B_SPLINE_CURVE((1.,1.00000531284332,1.00000243584221))
REPRESENTATION_ITEM('')
);
#18960=(
BOUNDED_CURVE()
B_SPLINE_CURVE(2,(#72022,#72023,#72024),.UNSPECIFIED.,.F.,.F.)
B_SPLINE_CURVE_WITH_KNOTS((3,3),(0.,0.073083726608569),.UNSPECIFIED.)
CURVE()
GEOMETRIC_REPRESENTATION_ITEM()
RATIONAL_B_SPLINE_CURVE((1.,1.00000531285339,1.00000243584683))
REPRESENTATION_ITEM('')
);
#18961=(
BOUNDED_CURVE()
B_SPLINE_CURVE(2,(#72034,#72035,#72036),.UNSPECIFIED.,.F.,.F.)
B_SPLINE_CURVE_WITH_KNOTS((3,3),(0.,0.0730837266082845),.UNSPECIFIED.)
CURVE()
GEOMETRIC_REPRESENTATION_ITEM()
RATIONAL_B_SPLINE_CURVE((1.,1.00000531285795,1.00000243584892))
REPRESENTATION_ITEM('')
);
#18962=(
BOUNDED_CURVE()
B_SPLINE_CURVE(2,(#72046,#72047,#72048),.UNSPECIFIED.,.F.,.F.)
B_SPLINE_CURVE_WITH_KNOTS((3,3),(0.,0.0730837266087279),.UNSPECIFIED.)
CURVE()
GEOMETRIC_REPRESENTATION_ITEM()
RATIONAL_B_SPLINE_CURVE((1.,1.00000531284088,1.00000243584109))
REPRESENTATION_ITEM('')
);
#18963=(
BOUNDED_CURVE()
B_SPLINE_CURVE(2,(#72058,#72059,#72060),.UNSPECIFIED.,.F.,.F.)
B_SPLINE_CURVE_WITH_KNOTS((3,3),(0.,0.07308372660842),.UNSPECIFIED.)
CURVE()
GEOMETRIC_REPRESENTATION_ITEM()
RATIONAL_B_SPLINE_CURVE((1.,1.0000053128307,1.00000243583643))
REPRESENTATION_ITEM('')
);
#18964=(
BOUNDED_CURVE()
B_SPLINE_CURVE(2,(#72070,#72071,#72072),.UNSPECIFIED.,.F.,.F.)
B_SPLINE_CURVE_WITH_KNOTS((3,3),(0.,0.0730837266082381),.UNSPECIFIED.)
CURVE()
GEOMETRIC_REPRESENTATION_ITEM()
RATIONAL_B_SPLINE_CURVE((1.,1.00000531281961,1.00000243583134))
REPRESENTATION_ITEM('')
);
#18965=(
BOUNDED_CURVE()
B_SPLINE_CURVE(2,(#72082,#72083,#72084),.UNSPECIFIED.,.F.,.F.)
B_SPLINE_CURVE_WITH_KNOTS((3,3),(0.,0.0730837266082899),.UNSPECIFIED.)
CURVE()
GEOMETRIC_REPRESENTATION_ITEM()
RATIONAL_B_SPLINE_CURVE((1.,1.00000531282543,1.00000243583401))
REPRESENTATION_ITEM('')
);
#18966=(
BOUNDED_CURVE()
B_SPLINE_CURVE(2,(#72094,#72095,#72096),.UNSPECIFIED.,.F.,.F.)
B_SPLINE_CURVE_WITH_KNOTS((3,3),(0.,0.07308372660794),.UNSPECIFIED.)
CURVE()
GEOMETRIC_REPRESENTATION_ITEM()
RATIONAL_B_SPLINE_CURVE((1.,1.0000053128172,1.00000243583024))
REPRESENTATION_ITEM('')
);
#18967=(
BOUNDED_CURVE()
B_SPLINE_CURVE(2,(#72106,#72107,#72108),.UNSPECIFIED.,.F.,.F.)
B_SPLINE_CURVE_WITH_KNOTS((3,3),(0.,0.0730837266081521),.UNSPECIFIED.)
CURVE()
GEOMETRIC_REPRESENTATION_ITEM()
RATIONAL_B_SPLINE_CURVE((1.,1.00000531282239,1.00000243583262))
REPRESENTATION_ITEM('')
);
#18968=(
BOUNDED_CURVE()
B_SPLINE_CURVE(2,(#72118,#72119,#72120),.UNSPECIFIED.,.F.,.F.)
B_SPLINE_CURVE_WITH_KNOTS((3,3),(0.,0.0730837266086474),.UNSPECIFIED.)
CURVE()
GEOMETRIC_REPRESENTATION_ITEM()
RATIONAL_B_SPLINE_CURVE((1.,1.00000531283521,1.0000024358385))
REPRESENTATION_ITEM('')
);
#18969=(
BOUNDED_CURVE()
B_SPLINE_CURVE(2,(#72130,#72131,#72132),.UNSPECIFIED.,.F.,.F.)
B_SPLINE_CURVE_WITH_KNOTS((3,3),(0.,0.0730837266084578),.UNSPECIFIED.)
CURVE()
GEOMETRIC_REPRESENTATION_ITEM()
RATIONAL_B_SPLINE_CURVE((1.,1.00000531285618,1.00000243584811))
REPRESENTATION_ITEM('')
);
#18970=(
BOUNDED_CURVE()
B_SPLINE_CURVE(2,(#72142,#72143,#72144),.UNSPECIFIED.,.F.,.F.)
B_SPLINE_CURVE_WITH_KNOTS((3,3),(0.,0.0730837266085192),.UNSPECIFIED.)
CURVE()
GEOMETRIC_REPRESENTATION_ITEM()
RATIONAL_B_SPLINE_CURVE((1.,1.0000053128433,1.0000024358422))
REPRESENTATION_ITEM('')
);
#18971=(
BOUNDED_CURVE()
B_SPLINE_CURVE(2,(#72154,#72155,#72156),.UNSPECIFIED.,.F.,.F.)
B_SPLINE_CURVE_WITH_KNOTS((3,3),(0.,0.0730837266085013),.UNSPECIFIED.)
CURVE()
GEOMETRIC_REPRESENTATION_ITEM()
RATIONAL_B_SPLINE_CURVE((1.,1.00000531284403,1.00000243584254))
REPRESENTATION_ITEM('')
);
#18972=(
BOUNDED_CURVE()
B_SPLINE_CURVE(2,(#72166,#72167,#72168),.UNSPECIFIED.,.F.,.F.)
B_SPLINE_CURVE_WITH_KNOTS((3,3),(0.,0.0730837266088684),.UNSPECIFIED.)
CURVE()
GEOMETRIC_REPRESENTATION_ITEM()
RATIONAL_B_SPLINE_CURVE((1.,1.00000531283876,1.00000243584012))
REPRESENTATION_ITEM('')
);
#18973=(
BOUNDED_CURVE()
B_SPLINE_CURVE(2,(#72178,#72179,#72180),.UNSPECIFIED.,.F.,.F.)
B_SPLINE_CURVE_WITH_KNOTS((3,3),(0.,0.0730837266083975),.UNSPECIFIED.)
CURVE()
GEOMETRIC_REPRESENTATION_ITEM()
RATIONAL_B_SPLINE_CURVE((1.,1.00000531281974,1.0000024358314))
REPRESENTATION_ITEM('')
);
#18974=(
BOUNDED_CURVE()
B_SPLINE_CURVE(2,(#72190,#72191,#72192),.UNSPECIFIED.,.F.,.F.)
B_SPLINE_CURVE_WITH_KNOTS((3,3),(0.,0.0730837266088218),.UNSPECIFIED.)
CURVE()
GEOMETRIC_REPRESENTATION_ITEM()
RATIONAL_B_SPLINE_CURVE((1.,1.00000531283784,1.0000024358397))
REPRESENTATION_ITEM('')
);
#18975=(
BOUNDED_CURVE()
B_SPLINE_CURVE(2,(#72202,#72203,#72204),.UNSPECIFIED.,.F.,.F.)
B_SPLINE_CURVE_WITH_KNOTS((3,3),(0.,0.0730837266083783),.UNSPECIFIED.)
CURVE()
GEOMETRIC_REPRESENTATION_ITEM()
RATIONAL_B_SPLINE_CURVE((1.,1.00000531283749,1.00000243583954))
REPRESENTATION_ITEM('')
);
#18976=(
BOUNDED_CURVE()
B_SPLINE_CURVE(2,(#72214,#72215,#72216),.UNSPECIFIED.,.F.,.F.)
B_SPLINE_CURVE_WITH_KNOTS((3,3),(0.,0.0730837266082154),.UNSPECIFIED.)
CURVE()
GEOMETRIC_REPRESENTATION_ITEM()
RATIONAL_B_SPLINE_CURVE((1.,1.00000531284379,1.00000243584243))
REPRESENTATION_ITEM('')
);
#18977=(
BOUNDED_CURVE()
B_SPLINE_CURVE(2,(#72226,#72227,#72228),.UNSPECIFIED.,.F.,.F.)
B_SPLINE_CURVE_WITH_KNOTS((3,3),(0.,0.0730837266084736),.UNSPECIFIED.)
CURVE()
GEOMETRIC_REPRESENTATION_ITEM()
RATIONAL_B_SPLINE_CURVE((1.,1.00000531282395,1.00000243583333))
REPRESENTATION_ITEM('')
);
#18978=(
BOUNDED_CURVE()
B_SPLINE_CURVE(2,(#72238,#72239,#72240),.UNSPECIFIED.,.F.,.F.)
B_SPLINE_CURVE_WITH_KNOTS((3,3),(0.,0.0730837266084901),.UNSPECIFIED.)
CURVE()
GEOMETRIC_REPRESENTATION_ITEM()
RATIONAL_B_SPLINE_CURVE((1.,1.00000531285787,1.00000243584888))
REPRESENTATION_ITEM('')
);
#18979=(
BOUNDED_CURVE()
B_SPLINE_CURVE(2,(#72250,#72251,#72252),.UNSPECIFIED.,.F.,.F.)
B_SPLINE_CURVE_WITH_KNOTS((3,3),(0.,0.0730837266088617),.UNSPECIFIED.)
CURVE()
GEOMETRIC_REPRESENTATION_ITEM()
RATIONAL_B_SPLINE_CURVE((1.,1.00000531286035,1.00000243585002))
REPRESENTATION_ITEM('')
);
#18980=(
BOUNDED_CURVE()
B_SPLINE_CURVE(2,(#72262,#72263,#72264),.UNSPECIFIED.,.F.,.F.)
B_SPLINE_CURVE_WITH_KNOTS((3,3),(0.,0.0730837266085078),.UNSPECIFIED.)
CURVE()
GEOMETRIC_REPRESENTATION_ITEM()
RATIONAL_B_SPLINE_CURVE((1.,1.00000531283572,1.00000243583873))
REPRESENTATION_ITEM('')
);
#18981=(
BOUNDED_CURVE()
B_SPLINE_CURVE(2,(#72274,#72275,#72276),.UNSPECIFIED.,.F.,.F.)
B_SPLINE_CURVE_WITH_KNOTS((3,3),(0.,0.0730837266082782),.UNSPECIFIED.)
CURVE()
GEOMETRIC_REPRESENTATION_ITEM()
RATIONAL_B_SPLINE_CURVE((1.,1.00000531280434,1.00000243582434))
REPRESENTATION_ITEM('')
);
#18982=(
BOUNDED_CURVE()
B_SPLINE_CURVE(2,(#72286,#72287,#72288),.UNSPECIFIED.,.F.,.F.)
B_SPLINE_CURVE_WITH_KNOTS((3,3),(0.,0.0730837266084148),.UNSPECIFIED.)
CURVE()
GEOMETRIC_REPRESENTATION_ITEM()
RATIONAL_B_SPLINE_CURVE((1.,1.00000531285132,1.00000243584588))
REPRESENTATION_ITEM('')
);
#18983=(
BOUNDED_CURVE()
B_SPLINE_CURVE(2,(#72298,#72299,#72300),.UNSPECIFIED.,.F.,.F.)
B_SPLINE_CURVE_WITH_KNOTS((3,3),(0.,0.0730837266088265),.UNSPECIFIED.)
CURVE()
GEOMETRIC_REPRESENTATION_ITEM()
RATIONAL_B_SPLINE_CURVE((1.,1.00000531285575,1.00000243584791))
REPRESENTATION_ITEM('')
);
#18984=(
BOUNDED_CURVE()
B_SPLINE_CURVE(2,(#72310,#72311,#72312),.UNSPECIFIED.,.F.,.F.)
B_SPLINE_CURVE_WITH_KNOTS((3,3),(0.,0.0730837266080522),.UNSPECIFIED.)
CURVE()
GEOMETRIC_REPRESENTATION_ITEM()
RATIONAL_B_SPLINE_CURVE((1.,1.00000531282666,1.00000243583457))
REPRESENTATION_ITEM('')
);
#18985=(
BOUNDED_CURVE()
B_SPLINE_CURVE(2,(#72322,#72323,#72324),.UNSPECIFIED.,.F.,.F.)
B_SPLINE_CURVE_WITH_KNOTS((3,3),(0.,0.0730837266080658),.UNSPECIFIED.)
CURVE()
GEOMETRIC_REPRESENTATION_ITEM()
RATIONAL_B_SPLINE_CURVE((1.,1.00000531283637,1.00000243583903))
REPRESENTATION_ITEM('')
);
#18986=(
BOUNDED_CURVE()
B_SPLINE_CURVE(2,(#72478,#72479,#72480),.UNSPECIFIED.,.F.,.F.)
B_SPLINE_CURVE_WITH_KNOTS((3,3),(0.021736728690041,0.0948204552983262),
 .UNSPECIFIED.)
CURVE()
GEOMETRIC_REPRESENTATION_ITEM()
RATIONAL_B_SPLINE_CURVE((1.00000243583482,1.00000531282719,1.))
REPRESENTATION_ITEM('')
);
#18987=(
BOUNDED_CURVE()
B_SPLINE_CURVE(2,(#72488,#72489,#72490),.UNSPECIFIED.,.F.,.F.)
B_SPLINE_CURVE_WITH_KNOTS((3,3),(0.0217367286900403,0.0948204552983261),
 .UNSPECIFIED.)
CURVE()
GEOMETRIC_REPRESENTATION_ITEM()
RATIONAL_B_SPLINE_CURVE((1.00000243584436,1.000005312848,1.))
REPRESENTATION_ITEM('')
);
#18988=(
BOUNDED_CURVE()
B_SPLINE_CURVE(2,(#72498,#72499,#72500),.UNSPECIFIED.,.F.,.F.)
B_SPLINE_CURVE_WITH_KNOTS((3,3),(0.0217367286900503,0.0948204552983257),
 .UNSPECIFIED.)
CURVE()
GEOMETRIC_REPRESENTATION_ITEM()
RATIONAL_B_SPLINE_CURVE((1.00000243583393,1.00000531282525,1.))
REPRESENTATION_ITEM('')
);
#18989=(
BOUNDED_CURVE()
B_SPLINE_CURVE(2,(#72508,#72509,#72510),.UNSPECIFIED.,.F.,.F.)
B_SPLINE_CURVE_WITH_KNOTS((3,3),(0.0217367286899,0.0948204552983259),
 .UNSPECIFIED.)
CURVE()
GEOMETRIC_REPRESENTATION_ITEM()
RATIONAL_B_SPLINE_CURVE((1.00000243583775,1.00000531283359,1.))
REPRESENTATION_ITEM('')
);
#18990=(
BOUNDED_CURVE()
B_SPLINE_CURVE(2,(#72518,#72519,#72520),.UNSPECIFIED.,.F.,.F.)
B_SPLINE_CURVE_WITH_KNOTS((3,3),(0.0217367286894302,0.0948204552983252),
 .UNSPECIFIED.)
CURVE()
GEOMETRIC_REPRESENTATION_ITEM()
RATIONAL_B_SPLINE_CURVE((1.00000243585063,1.00000531286168,1.))
REPRESENTATION_ITEM('')
);
#18991=(
BOUNDED_CURVE()
B_SPLINE_CURVE(2,(#72528,#72529,#72530),.UNSPECIFIED.,.F.,.F.)
B_SPLINE_CURVE_WITH_KNOTS((3,3),(0.0217367286902311,0.0948204552983257),
 .UNSPECIFIED.)
CURVE()
GEOMETRIC_REPRESENTATION_ITEM()
RATIONAL_B_SPLINE_CURVE((1.00000243584031,1.00000531283916,1.))
REPRESENTATION_ITEM('')
);
#18992=(
BOUNDED_CURVE()
B_SPLINE_CURVE(2,(#72538,#72539,#72540),.UNSPECIFIED.,.F.,.F.)
B_SPLINE_CURVE_WITH_KNOTS((3,3),(0.0217367286900553,0.0948204552983258),
 .UNSPECIFIED.)
CURVE()
GEOMETRIC_REPRESENTATION_ITEM()
RATIONAL_B_SPLINE_CURVE((1.00000243583602,1.00000531282982,1.))
REPRESENTATION_ITEM('')
);
#18993=(
BOUNDED_CURVE()
B_SPLINE_CURVE(2,(#72548,#72549,#72550),.UNSPECIFIED.,.F.,.F.)
B_SPLINE_CURVE_WITH_KNOTS((3,3),(0.0217367286900607,0.0948204552983253),
 .UNSPECIFIED.)
CURVE()
GEOMETRIC_REPRESENTATION_ITEM()
RATIONAL_B_SPLINE_CURVE((1.0000024358435,1.00000531284613,1.))
REPRESENTATION_ITEM('')
);
#18994=(
BOUNDED_CURVE()
B_SPLINE_CURVE(2,(#72558,#72559,#72560),.UNSPECIFIED.,.F.,.F.)
B_SPLINE_CURVE_WITH_KNOTS((3,3),(0.0217367286901279,0.0948204552983257),
 .UNSPECIFIED.)
CURVE()
GEOMETRIC_REPRESENTATION_ITEM()
RATIONAL_B_SPLINE_CURVE((1.00000243583628,1.00000531283037,1.))
REPRESENTATION_ITEM('')
);
#18995=(
BOUNDED_CURVE()
B_SPLINE_CURVE(2,(#72568,#72569,#72570),.UNSPECIFIED.,.F.,.F.)
B_SPLINE_CURVE_WITH_KNOTS((3,3),(0.0217367286900851,0.0948204552983262),
 .UNSPECIFIED.)
CURVE()
GEOMETRIC_REPRESENTATION_ITEM()
RATIONAL_B_SPLINE_CURVE((1.00000243583421,1.00000531282587,1.))
REPRESENTATION_ITEM('')
);
#18996=(
BOUNDED_CURVE()
B_SPLINE_CURVE(2,(#72578,#72579,#72580),.UNSPECIFIED.,.F.,.F.)
B_SPLINE_CURVE_WITH_KNOTS((3,3),(0.0217367286893238,0.0948204552983258),
 .UNSPECIFIED.)
CURVE()
GEOMETRIC_REPRESENTATION_ITEM()
RATIONAL_B_SPLINE_CURVE((1.000002435848,1.00000531285594,1.))
REPRESENTATION_ITEM('')
);
#18997=(
BOUNDED_CURVE()
B_SPLINE_CURVE(2,(#72588,#72589,#72590),.UNSPECIFIED.,.F.,.F.)
B_SPLINE_CURVE_WITH_KNOTS((3,3),(0.0217367286896447,0.0948204552983257),
 .UNSPECIFIED.)
CURVE()
GEOMETRIC_REPRESENTATION_ITEM()
RATIONAL_B_SPLINE_CURVE((1.00000243584317,1.00000531284541,1.))
REPRESENTATION_ITEM('')
);
#18998=(
BOUNDED_CURVE()
B_SPLINE_CURVE(2,(#72598,#72599,#72600),.UNSPECIFIED.,.F.,.F.)
B_SPLINE_CURVE_WITH_KNOTS((3,3),(0.0217367286897485,0.0948204552983259),
 .UNSPECIFIED.)
CURVE()
GEOMETRIC_REPRESENTATION_ITEM()
RATIONAL_B_SPLINE_CURVE((1.0000024358422,1.0000053128433,1.))
REPRESENTATION_ITEM('')
);
#18999=(
BOUNDED_CURVE()
B_SPLINE_CURVE(2,(#72608,#72609,#72610),.UNSPECIFIED.,.F.,.F.)
B_SPLINE_CURVE_WITH_KNOTS((3,3),(0.0217367286893197,0.0948204552983255),
 .UNSPECIFIED.)
CURVE()
GEOMETRIC_REPRESENTATION_ITEM()
RATIONAL_B_SPLINE_CURVE((1.00000243584811,1.00000531285618,1.))
REPRESENTATION_ITEM('')
);
#19000=(
BOUNDED_CURVE()
B_SPLINE_CURVE(2,(#72618,#72619,#72620),.UNSPECIFIED.,.F.,.F.)
B_SPLINE_CURVE_WITH_KNOTS((3,3),(0.0217367286898305,0.0948204552983257),
 .UNSPECIFIED.)
CURVE()
GEOMETRIC_REPRESENTATION_ITEM()
RATIONAL_B_SPLINE_CURVE((1.00000243584037,1.00000531283929,1.))
REPRESENTATION_ITEM('')
);
#19001=(
BOUNDED_CURVE()
B_SPLINE_CURVE(2,(#72628,#72629,#72630),.UNSPECIFIED.,.F.,.F.)
B_SPLINE_CURVE_WITH_KNOTS((3,3),(0.0217367286898262,0.0948204552983256),
 .UNSPECIFIED.)
CURVE()
GEOMETRIC_REPRESENTATION_ITEM()
RATIONAL_B_SPLINE_CURVE((1.00000243583868,1.00000531283562,1.))
REPRESENTATION_ITEM('')
);
#19002=(
BOUNDED_CURVE()
B_SPLINE_CURVE(2,(#72638,#72639,#72640),.UNSPECIFIED.,.F.,.F.)
B_SPLINE_CURVE_WITH_KNOTS((3,3),(0.0217367286902262,0.0948204552983252),
 .UNSPECIFIED.)
CURVE()
GEOMETRIC_REPRESENTATION_ITEM()
RATIONAL_B_SPLINE_CURVE((1.00000243583729,1.00000531283259,1.))
REPRESENTATION_ITEM('')
);
#19003=(
BOUNDED_CURVE()
B_SPLINE_CURVE(2,(#72648,#72649,#72650),.UNSPECIFIED.,.F.,.F.)
B_SPLINE_CURVE_WITH_KNOTS((3,3),(0.0217367286902091,0.0948204552983257),
 .UNSPECIFIED.)
CURVE()
GEOMETRIC_REPRESENTATION_ITEM()
RATIONAL_B_SPLINE_CURVE((1.00000243583305,1.00000531282334,1.))
REPRESENTATION_ITEM('')
);
#19004=(
BOUNDED_CURVE()
B_SPLINE_CURVE(2,(#72658,#72659,#72660),.UNSPECIFIED.,.F.,.F.)
B_SPLINE_CURVE_WITH_KNOTS((3,3),(0.0217367286892795,0.0948204552983256),
 .UNSPECIFIED.)
CURVE()
GEOMETRIC_REPRESENTATION_ITEM()
RATIONAL_B_SPLINE_CURVE((1.00000243584826,1.00000531285652,1.))
REPRESENTATION_ITEM('')
);
#19005=(
BOUNDED_CURVE()
B_SPLINE_CURVE(2,(#72668,#72669,#72670),.UNSPECIFIED.,.F.,.F.)
B_SPLINE_CURVE_WITH_KNOTS((3,3),(0.0217367286900581,0.0948204552983268),
 .UNSPECIFIED.)
CURVE()
GEOMETRIC_REPRESENTATION_ITEM()
RATIONAL_B_SPLINE_CURVE((1.00000243583706,1.00000531283209,1.))
REPRESENTATION_ITEM('')
);
#19006=(
BOUNDED_CURVE()
B_SPLINE_CURVE(2,(#72678,#72679,#72680),.UNSPECIFIED.,.F.,.F.)
B_SPLINE_CURVE_WITH_KNOTS((3,3),(0.0217367286899271,0.0948204552983257),
 .UNSPECIFIED.)
CURVE()
GEOMETRIC_REPRESENTATION_ITEM()
RATIONAL_B_SPLINE_CURVE((1.00000243583793,1.00000531283399,1.))
REPRESENTATION_ITEM('')
);
#19007=(
BOUNDED_CURVE()
B_SPLINE_CURVE(2,(#72688,#72689,#72690),.UNSPECIFIED.,.F.,.F.)
B_SPLINE_CURVE_WITH_KNOTS((3,3),(0.0217367286897488,0.0948204552983259),
 .UNSPECIFIED.)
CURVE()
GEOMETRIC_REPRESENTATION_ITEM()
RATIONAL_B_SPLINE_CURVE((1.0000024358422,1.0000053128433,1.))
REPRESENTATION_ITEM('')
);
#19008=(
BOUNDED_CURVE()
B_SPLINE_CURVE(2,(#72698,#72699,#72700),.UNSPECIFIED.,.F.,.F.)
B_SPLINE_CURVE_WITH_KNOTS((3,3),(0.0217367286894558,0.0948204552983258),
 .UNSPECIFIED.)
CURVE()
GEOMETRIC_REPRESENTATION_ITEM()
RATIONAL_B_SPLINE_CURVE((1.00000243584193,1.00000531284271,1.))
REPRESENTATION_ITEM('')
);
#19009=(
BOUNDED_CURVE()
B_SPLINE_CURVE(2,(#72708,#72709,#72710),.UNSPECIFIED.,.F.,.F.)
B_SPLINE_CURVE_WITH_KNOTS((3,3),(0.0217367286898531,0.0948204552983254),
 .UNSPECIFIED.)
CURVE()
GEOMETRIC_REPRESENTATION_ITEM()
RATIONAL_B_SPLINE_CURVE((1.00000243584379,1.00000531284676,1.))
REPRESENTATION_ITEM('')
);
#19010=(
BOUNDED_CURVE()
B_SPLINE_CURVE(2,(#72718,#72719,#72720),.UNSPECIFIED.,.F.,.F.)
B_SPLINE_CURVE_WITH_KNOTS((3,3),(0.0217367286900914,0.0948204552983258),
 .UNSPECIFIED.)
CURVE()
GEOMETRIC_REPRESENTATION_ITEM()
RATIONAL_B_SPLINE_CURVE((1.00000243582673,1.00000531280955,1.))
REPRESENTATION_ITEM('')
);
#19011=(
BOUNDED_CURVE()
B_SPLINE_CURVE(2,(#72728,#72729,#72730),.UNSPECIFIED.,.F.,.F.)
B_SPLINE_CURVE_WITH_KNOTS((3,3),(0.0217367286896848,0.0948204552983253),
 .UNSPECIFIED.)
CURVE()
GEOMETRIC_REPRESENTATION_ITEM()
RATIONAL_B_SPLINE_CURVE((1.00000243584611,1.00000531285181,1.))
REPRESENTATION_ITEM('')
);
#19012=(
BOUNDED_CURVE()
B_SPLINE_CURVE(2,(#72738,#72739,#72740),.UNSPECIFIED.,.F.,.F.)
B_SPLINE_CURVE_WITH_KNOTS((3,3),(0.0217367286896856,0.0948204552983257),
 .UNSPECIFIED.)
CURVE()
GEOMETRIC_REPRESENTATION_ITEM()
RATIONAL_B_SPLINE_CURVE((1.00000243583825,1.00000531283468,1.))
REPRESENTATION_ITEM('')
);
#19013=(
BOUNDED_CURVE()
B_SPLINE_CURVE(2,(#72748,#72749,#72750),.UNSPECIFIED.,.F.,.F.)
B_SPLINE_CURVE_WITH_KNOTS((3,3),(0.0217367286899301,0.0948204552983263),
 .UNSPECIFIED.)
CURVE()
GEOMETRIC_REPRESENTATION_ITEM()
RATIONAL_B_SPLINE_CURVE((1.00000243583883,1.00000531283595,1.))
REPRESENTATION_ITEM('')
);
#19014=(
BOUNDED_CURVE()
B_SPLINE_CURVE(2,(#72758,#72759,#72760),.UNSPECIFIED.,.F.,.F.)
B_SPLINE_CURVE_WITH_KNOTS((3,3),(0.0217367286899796,0.0948204552983267),
 .UNSPECIFIED.)
CURVE()
GEOMETRIC_REPRESENTATION_ITEM()
RATIONAL_B_SPLINE_CURVE((1.00000243584071,1.00000531284005,1.))
REPRESENTATION_ITEM('')
);
#19015=(
BOUNDED_CURVE()
B_SPLINE_CURVE(2,(#72768,#72769,#72770),.UNSPECIFIED.,.F.,.F.)
B_SPLINE_CURVE_WITH_KNOTS((3,3),(0.0217367286899505,0.0948204552983261),
 .UNSPECIFIED.)
CURVE()
GEOMETRIC_REPRESENTATION_ITEM()
RATIONAL_B_SPLINE_CURVE((1.00000243583762,1.00000531283331,1.))
REPRESENTATION_ITEM('')
);
#19016=(
BOUNDED_CURVE()
B_SPLINE_CURVE(2,(#72778,#72779,#72780),.UNSPECIFIED.,.F.,.F.)
B_SPLINE_CURVE_WITH_KNOTS((3,3),(0.0217367286898014,0.0948204552983259),
 .UNSPECIFIED.)
CURVE()
GEOMETRIC_REPRESENTATION_ITEM()
RATIONAL_B_SPLINE_CURVE((1.00000243585023,1.0000053128608,1.))
REPRESENTATION_ITEM('')
);
#19017=(
BOUNDED_CURVE()
B_SPLINE_CURVE(2,(#72788,#72789,#72790),.UNSPECIFIED.,.F.,.F.)
B_SPLINE_CURVE_WITH_KNOTS((3,3),(0.0217367286893197,0.0948204552983255),
 .UNSPECIFIED.)
CURVE()
GEOMETRIC_REPRESENTATION_ITEM()
RATIONAL_B_SPLINE_CURVE((1.00000243584811,1.00000531285618,1.))
REPRESENTATION_ITEM('')
);
#19018=(
BOUNDED_CURVE()
B_SPLINE_CURVE(2,(#72798,#72799,#72800),.UNSPECIFIED.,.F.,.F.)
B_SPLINE_CURVE_WITH_KNOTS((3,3),(0.0217367286898152,0.0948204552983257),
 .UNSPECIFIED.)
CURVE()
GEOMETRIC_REPRESENTATION_ITEM()
RATIONAL_B_SPLINE_CURVE((1.0000024358428,1.00000531284459,1.))
REPRESENTATION_ITEM('')
);
#19019=(
BOUNDED_CURVE()
B_SPLINE_CURVE(2,(#72808,#72809,#72810),.UNSPECIFIED.,.F.,.F.)
B_SPLINE_CURVE_WITH_KNOTS((3,3),(0.0217367286898778,0.0948204552983258),
 .UNSPECIFIED.)
CURVE()
GEOMETRIC_REPRESENTATION_ITEM()
RATIONAL_B_SPLINE_CURVE((1.000002435835,1.00000531282759,1.))
REPRESENTATION_ITEM('')
);
#19020=(
BOUNDED_CURVE()
B_SPLINE_CURVE(2,(#72818,#72819,#72820),.UNSPECIFIED.,.F.,.F.)
B_SPLINE_CURVE_WITH_KNOTS((3,3),(0.0217367286899082,0.0948204552983253),
 .UNSPECIFIED.)
CURVE()
GEOMETRIC_REPRESENTATION_ITEM()
RATIONAL_B_SPLINE_CURVE((1.00000243584336,1.00000531284581,1.))
REPRESENTATION_ITEM('')
);
#19021=(
BOUNDED_CURVE()
B_SPLINE_CURVE(2,(#72825,#72826,#72827),.UNSPECIFIED.,.F.,.F.)
B_SPLINE_CURVE_WITH_KNOTS((3,3),(0.258079386101496,0.459416258484591),
 .UNSPECIFIED.)
CURVE()
GEOMETRIC_REPRESENTATION_ITEM()
RATIONAL_B_SPLINE_CURVE((1.00161624157847,1.00189253035136,1.00161624157847))
REPRESENTATION_ITEM('')
);
#19022=(
BOUNDED_CURVE()
B_SPLINE_CURVE(2,(#72975,#72976,#72977),.UNSPECIFIED.,.F.,.F.)
B_SPLINE_CURVE_WITH_KNOTS((3,3),(0.258079386101492,0.459416258484576),
 .UNSPECIFIED.)
CURVE()
GEOMETRIC_REPRESENTATION_ITEM()
RATIONAL_B_SPLINE_CURVE((1.00161624157842,1.00189253035131,1.00161624157842))
REPRESENTATION_ITEM('')
);
#19023=(
BOUNDED_CURVE()
B_SPLINE_CURVE(2,(#72981,#72982,#72983),.UNSPECIFIED.,.F.,.F.)
B_SPLINE_CURVE_WITH_KNOTS((3,3),(0.258079386101496,0.459416258484592),
 .UNSPECIFIED.)
CURVE()
GEOMETRIC_REPRESENTATION_ITEM()
RATIONAL_B_SPLINE_CURVE((1.00161624157848,1.00189253035137,1.00161624157848))
REPRESENTATION_ITEM('')
);
#19024=(
BOUNDED_CURVE()
B_SPLINE_CURVE(2,(#72987,#72988,#72989),.UNSPECIFIED.,.F.,.F.)
B_SPLINE_CURVE_WITH_KNOTS((3,3),(0.258079386101498,0.459416258484592),
 .UNSPECIFIED.)
CURVE()
GEOMETRIC_REPRESENTATION_ITEM()
RATIONAL_B_SPLINE_CURVE((1.00161624157846,1.00189253035135,1.00161624157846))
REPRESENTATION_ITEM('')
);
#19025=(
BOUNDED_CURVE()
B_SPLINE_CURVE(2,(#72993,#72994,#72995),.UNSPECIFIED.,.F.,.F.)
B_SPLINE_CURVE_WITH_KNOTS((3,3),(0.258079386101496,0.45941625848459),
 .UNSPECIFIED.)
CURVE()
GEOMETRIC_REPRESENTATION_ITEM()
RATIONAL_B_SPLINE_CURVE((1.00161624157846,1.00189253035135,1.00161624157846))
REPRESENTATION_ITEM('')
);
#19026=(
BOUNDED_CURVE()
B_SPLINE_CURVE(2,(#72999,#73000,#73001),.UNSPECIFIED.,.F.,.F.)
B_SPLINE_CURVE_WITH_KNOTS((3,3),(0.258079386101498,0.45941625848459),
 .UNSPECIFIED.)
CURVE()
GEOMETRIC_REPRESENTATION_ITEM()
RATIONAL_B_SPLINE_CURVE((1.00161624157846,1.00189253035135,1.00161624157846))
REPRESENTATION_ITEM('')
);
#19027=(
BOUNDED_CURVE()
B_SPLINE_CURVE(2,(#73005,#73006,#73007),.UNSPECIFIED.,.F.,.F.)
B_SPLINE_CURVE_WITH_KNOTS((3,3),(0.258079386101502,0.459416258484588),
 .UNSPECIFIED.)
CURVE()
GEOMETRIC_REPRESENTATION_ITEM()
RATIONAL_B_SPLINE_CURVE((1.00161624157843,1.00189253035131,1.00161624157843))
REPRESENTATION_ITEM('')
);
#19028=(
BOUNDED_CURVE()
B_SPLINE_CURVE(2,(#73011,#73012,#73013),.UNSPECIFIED.,.F.,.F.)
B_SPLINE_CURVE_WITH_KNOTS((3,3),(0.258079386101497,0.459416258484587),
 .UNSPECIFIED.)
CURVE()
GEOMETRIC_REPRESENTATION_ITEM()
RATIONAL_B_SPLINE_CURVE((1.00161624157845,1.00189253035134,1.00161624157845))
REPRESENTATION_ITEM('')
);
#19029=(
BOUNDED_CURVE()
B_SPLINE_CURVE(2,(#73017,#73018,#73019),.UNSPECIFIED.,.F.,.F.)
B_SPLINE_CURVE_WITH_KNOTS((3,3),(0.258079386101498,0.459416258484589),
 .UNSPECIFIED.)
CURVE()
GEOMETRIC_REPRESENTATION_ITEM()
RATIONAL_B_SPLINE_CURVE((1.00161624157846,1.00189253035135,1.00161624157846))
REPRESENTATION_ITEM('')
);
#19030=(
BOUNDED_CURVE()
B_SPLINE_CURVE(2,(#73023,#73024,#73025),.UNSPECIFIED.,.F.,.F.)
B_SPLINE_CURVE_WITH_KNOTS((3,3),(0.258079386101496,0.459416258484592),
 .UNSPECIFIED.)
CURVE()
GEOMETRIC_REPRESENTATION_ITEM()
RATIONAL_B_SPLINE_CURVE((1.00161624157848,1.00189253035137,1.00161624157848))
REPRESENTATION_ITEM('')
);
#19031=(
BOUNDED_CURVE()
B_SPLINE_CURVE(2,(#73029,#73030,#73031),.UNSPECIFIED.,.F.,.F.)
B_SPLINE_CURVE_WITH_KNOTS((3,3),(0.258079386101487,0.459416258484582),
 .UNSPECIFIED.)
CURVE()
GEOMETRIC_REPRESENTATION_ITEM()
RATIONAL_B_SPLINE_CURVE((1.00161624157848,1.00189253035137,1.00161624157848))
REPRESENTATION_ITEM('')
);
#19032=(
BOUNDED_CURVE()
B_SPLINE_CURVE(2,(#73035,#73036,#73037),.UNSPECIFIED.,.F.,.F.)
B_SPLINE_CURVE_WITH_KNOTS((3,3),(0.258079386101498,0.459416258484594),
 .UNSPECIFIED.)
CURVE()
GEOMETRIC_REPRESENTATION_ITEM()
RATIONAL_B_SPLINE_CURVE((1.00161624157848,1.00189253035137,1.00161624157848))
REPRESENTATION_ITEM('')
);
#19033=(
BOUNDED_CURVE()
B_SPLINE_CURVE(2,(#73041,#73042,#73043),.UNSPECIFIED.,.F.,.F.)
B_SPLINE_CURVE_WITH_KNOTS((3,3),(0.258079386101494,0.459416258484593),
 .UNSPECIFIED.)
CURVE()
GEOMETRIC_REPRESENTATION_ITEM()
RATIONAL_B_SPLINE_CURVE((1.00161624157849,1.00189253035139,1.00161624157849))
REPRESENTATION_ITEM('')
);
#19034=(
BOUNDED_CURVE()
B_SPLINE_CURVE(2,(#73047,#73048,#73049),.UNSPECIFIED.,.F.,.F.)
B_SPLINE_CURVE_WITH_KNOTS((3,3),(0.258079386101507,0.459416258484601),
 .UNSPECIFIED.)
CURVE()
GEOMETRIC_REPRESENTATION_ITEM()
RATIONAL_B_SPLINE_CURVE((1.00161624157847,1.00189253035136,1.00161624157847))
REPRESENTATION_ITEM('')
);
#19035=(
BOUNDED_CURVE()
B_SPLINE_CURVE(2,(#73053,#73054,#73055),.UNSPECIFIED.,.F.,.F.)
B_SPLINE_CURVE_WITH_KNOTS((3,3),(0.258079386101498,0.459416258484589),
 .UNSPECIFIED.)
CURVE()
GEOMETRIC_REPRESENTATION_ITEM()
RATIONAL_B_SPLINE_CURVE((1.00161624157845,1.00189253035134,1.00161624157845))
REPRESENTATION_ITEM('')
);
#19036=(
BOUNDED_CURVE()
B_SPLINE_CURVE(2,(#73059,#73060,#73061),.UNSPECIFIED.,.F.,.F.)
B_SPLINE_CURVE_WITH_KNOTS((3,3),(0.258079386101491,0.45941625848459),
 .UNSPECIFIED.)
CURVE()
GEOMETRIC_REPRESENTATION_ITEM()
RATIONAL_B_SPLINE_CURVE((1.00161624157849,1.00189253035139,1.00161624157849))
REPRESENTATION_ITEM('')
);
#19037=(
BOUNDED_CURVE()
B_SPLINE_CURVE(2,(#73065,#73066,#73067),.UNSPECIFIED.,.F.,.F.)
B_SPLINE_CURVE_WITH_KNOTS((3,3),(0.258079386101511,0.459416258484598),
 .UNSPECIFIED.)
CURVE()
GEOMETRIC_REPRESENTATION_ITEM()
RATIONAL_B_SPLINE_CURVE((1.00161624157843,1.00189253035132,1.00161624157843))
REPRESENTATION_ITEM('')
);
#19038=(
BOUNDED_CURVE()
B_SPLINE_CURVE(2,(#73071,#73072,#73073),.UNSPECIFIED.,.F.,.F.)
B_SPLINE_CURVE_WITH_KNOTS((3,3),(0.258079386101497,0.459416258484589),
 .UNSPECIFIED.)
CURVE()
GEOMETRIC_REPRESENTATION_ITEM()
RATIONAL_B_SPLINE_CURVE((1.00161624157846,1.00189253035135,1.00161624157846))
REPRESENTATION_ITEM('')
);
#19039=(
BOUNDED_CURVE()
B_SPLINE_CURVE(2,(#73078,#73079,#73080),.UNSPECIFIED.,.F.,.F.)
B_SPLINE_CURVE_WITH_KNOTS((3,3),(0.358747822293045,0.459416258484592),
 .UNSPECIFIED.)
CURVE()
GEOMETRIC_REPRESENTATION_ITEM()
RATIONAL_B_SPLINE_CURVE((1.00175438596492,1.00175438596492,1.00161624157848))
REPRESENTATION_ITEM('')
);
#19040=(
BOUNDED_CURVE()
B_SPLINE_CURVE(2,(#73081,#73082,#73083),.UNSPECIFIED.,.F.,.F.)
B_SPLINE_CURVE_WITH_KNOTS((3,3),(0.258079386101496,0.358747822293045),
 .UNSPECIFIED.)
CURVE()
GEOMETRIC_REPRESENTATION_ITEM()
RATIONAL_B_SPLINE_CURVE((1.00161624157848,1.00175438596492,1.00175438596492))
REPRESENTATION_ITEM('')
);
#19041=(
BOUNDED_CURVE()
B_SPLINE_CURVE(2,(#73087,#73088,#73089),.UNSPECIFIED.,.F.,.F.)
B_SPLINE_CURVE_WITH_KNOTS((3,3),(0.258079386101499,0.459416258484591),
 .UNSPECIFIED.)
CURVE()
GEOMETRIC_REPRESENTATION_ITEM()
RATIONAL_B_SPLINE_CURVE((1.00161624157846,1.00189253035135,1.00161624157846))
REPRESENTATION_ITEM('')
);
#19042=(
BOUNDED_CURVE()
B_SPLINE_CURVE(2,(#73093,#73094,#73095),.UNSPECIFIED.,.F.,.F.)
B_SPLINE_CURVE_WITH_KNOTS((3,3),(0.258079386101487,0.459416258484581),
 .UNSPECIFIED.)
CURVE()
GEOMETRIC_REPRESENTATION_ITEM()
RATIONAL_B_SPLINE_CURVE((1.00161624157848,1.00189253035137,1.00161624157848))
REPRESENTATION_ITEM('')
);
#19043=(
BOUNDED_CURVE()
B_SPLINE_CURVE(2,(#73099,#73100,#73101),.UNSPECIFIED.,.F.,.F.)
B_SPLINE_CURVE_WITH_KNOTS((3,3),(0.258079386101499,0.459416258484585),
 .UNSPECIFIED.)
CURVE()
GEOMETRIC_REPRESENTATION_ITEM()
RATIONAL_B_SPLINE_CURVE((1.00161624157843,1.00189253035131,1.00161624157843))
REPRESENTATION_ITEM('')
);
#19044=(
BOUNDED_CURVE()
B_SPLINE_CURVE(2,(#73105,#73106,#73107),.UNSPECIFIED.,.F.,.F.)
B_SPLINE_CURVE_WITH_KNOTS((3,3),(0.258079386101507,0.459416258484601),
 .UNSPECIFIED.)
CURVE()
GEOMETRIC_REPRESENTATION_ITEM()
RATIONAL_B_SPLINE_CURVE((1.00161624157847,1.00189253035136,1.00161624157847))
REPRESENTATION_ITEM('')
);
#19045=(
BOUNDED_CURVE()
B_SPLINE_CURVE(2,(#73111,#73112,#73113),.UNSPECIFIED.,.F.,.F.)
B_SPLINE_CURVE_WITH_KNOTS((3,3),(0.258079386101492,0.459416258484594),
 .UNSPECIFIED.)
CURVE()
GEOMETRIC_REPRESENTATION_ITEM()
RATIONAL_B_SPLINE_CURVE((1.0016162415785,1.0018925303514,1.0016162415785))
REPRESENTATION_ITEM('')
);
#19046=(
BOUNDED_CURVE()
B_SPLINE_CURVE(2,(#73117,#73118,#73119),.UNSPECIFIED.,.F.,.F.)
B_SPLINE_CURVE_WITH_KNOTS((3,3),(0.258079386101498,0.459416258484587),
 .UNSPECIFIED.)
CURVE()
GEOMETRIC_REPRESENTATION_ITEM()
RATIONAL_B_SPLINE_CURVE((1.00161624157845,1.00189253035133,1.00161624157845))
REPRESENTATION_ITEM('')
);
#19047=(
BOUNDED_CURVE()
B_SPLINE_CURVE(2,(#73123,#73124,#73125),.UNSPECIFIED.,.F.,.F.)
B_SPLINE_CURVE_WITH_KNOTS((3,3),(0.258079386101511,0.459416258484597),
 .UNSPECIFIED.)
CURVE()
GEOMETRIC_REPRESENTATION_ITEM()
RATIONAL_B_SPLINE_CURVE((1.00161624157843,1.00189253035131,1.00161624157843))
REPRESENTATION_ITEM('')
);
#19048=(
BOUNDED_CURVE()
B_SPLINE_CURVE(2,(#73129,#73130,#73131),.UNSPECIFIED.,.F.,.F.)
B_SPLINE_CURVE_WITH_KNOTS((3,3),(0.258079386101486,0.459416258484581),
 .UNSPECIFIED.)
CURVE()
GEOMETRIC_REPRESENTATION_ITEM()
RATIONAL_B_SPLINE_CURVE((1.00161624157848,1.00189253035137,1.00161624157848))
REPRESENTATION_ITEM('')
);
#19049=(
BOUNDED_CURVE()
B_SPLINE_CURVE(2,(#73135,#73136,#73137),.UNSPECIFIED.,.F.,.F.)
B_SPLINE_CURVE_WITH_KNOTS((3,3),(0.258079386101496,0.459416258484591),
 .UNSPECIFIED.)
CURVE()
GEOMETRIC_REPRESENTATION_ITEM()
RATIONAL_B_SPLINE_CURVE((1.00161624157848,1.00189253035137,1.00161624157848))
REPRESENTATION_ITEM('')
);
#19050=(
BOUNDED_CURVE()
B_SPLINE_CURVE(2,(#73141,#73142,#73143),.UNSPECIFIED.,.F.,.F.)
B_SPLINE_CURVE_WITH_KNOTS((3,3),(0.258079386101487,0.459416258484582),
 .UNSPECIFIED.)
CURVE()
GEOMETRIC_REPRESENTATION_ITEM()
RATIONAL_B_SPLINE_CURVE((1.00161624157848,1.00189253035137,1.00161624157848))
REPRESENTATION_ITEM('')
);
#19051=(
BOUNDED_CURVE()
B_SPLINE_CURVE(2,(#73147,#73148,#73149),.UNSPECIFIED.,.F.,.F.)
B_SPLINE_CURVE_WITH_KNOTS((3,3),(0.258079386101486,0.459416258484582),
 .UNSPECIFIED.)
CURVE()
GEOMETRIC_REPRESENTATION_ITEM()
RATIONAL_B_SPLINE_CURVE((1.00161624157848,1.00189253035137,1.00161624157848))
REPRESENTATION_ITEM('')
);
#19052=(
BOUNDED_CURVE()
B_SPLINE_CURVE(2,(#73153,#73154,#73155),.UNSPECIFIED.,.F.,.F.)
B_SPLINE_CURVE_WITH_KNOTS((3,3),(0.258079386101501,0.459416258484586),
 .UNSPECIFIED.)
CURVE()
GEOMETRIC_REPRESENTATION_ITEM()
RATIONAL_B_SPLINE_CURVE((1.00161624157843,1.00189253035131,1.00161624157843))
REPRESENTATION_ITEM('')
);
#19053=(
BOUNDED_CURVE()
B_SPLINE_CURVE(2,(#73159,#73160,#73161),.UNSPECIFIED.,.F.,.F.)
B_SPLINE_CURVE_WITH_KNOTS((3,3),(0.258079386101494,0.459416258484595),
 .UNSPECIFIED.)
CURVE()
GEOMETRIC_REPRESENTATION_ITEM()
RATIONAL_B_SPLINE_CURVE((1.0016162415785,1.0018925303514,1.0016162415785))
REPRESENTATION_ITEM('')
);
#19054=(
BOUNDED_CURVE()
B_SPLINE_CURVE(2,(#73165,#73166,#73167),.UNSPECIFIED.,.F.,.F.)
B_SPLINE_CURVE_WITH_KNOTS((3,3),(0.258079386101498,0.459416258484589),
 .UNSPECIFIED.)
CURVE()
GEOMETRIC_REPRESENTATION_ITEM()
RATIONAL_B_SPLINE_CURVE((1.00161624157845,1.00189253035134,1.00161624157845))
REPRESENTATION_ITEM('')
);
#19055=(
BOUNDED_CURVE()
B_SPLINE_CURVE(2,(#73171,#73172,#73173),.UNSPECIFIED.,.F.,.F.)
B_SPLINE_CURVE_WITH_KNOTS((3,3),(0.258079386101503,0.459416258484589),
 .UNSPECIFIED.)
CURVE()
GEOMETRIC_REPRESENTATION_ITEM()
RATIONAL_B_SPLINE_CURVE((1.00161624157843,1.00189253035131,1.00161624157843))
REPRESENTATION_ITEM('')
);
#19056=(
BOUNDED_CURVE()
B_SPLINE_CURVE(2,(#73177,#73178,#73179),.UNSPECIFIED.,.F.,.F.)
B_SPLINE_CURVE_WITH_KNOTS((3,3),(0.258079386101511,0.459416258484597),
 .UNSPECIFIED.)
CURVE()
GEOMETRIC_REPRESENTATION_ITEM()
RATIONAL_B_SPLINE_CURVE((1.00161624157843,1.00189253035131,1.00161624157843))
REPRESENTATION_ITEM('')
);
#19057=(
BOUNDED_CURVE()
B_SPLINE_CURVE(2,(#73183,#73184,#73185),.UNSPECIFIED.,.F.,.F.)
B_SPLINE_CURVE_WITH_KNOTS((3,3),(0.258079386101485,0.45941625848458),
 .UNSPECIFIED.)
CURVE()
GEOMETRIC_REPRESENTATION_ITEM()
RATIONAL_B_SPLINE_CURVE((1.00161624157848,1.00189253035137,1.00161624157848))
REPRESENTATION_ITEM('')
);
#19058=(
BOUNDED_CURVE()
B_SPLINE_CURVE(2,(#73189,#73190,#73191),.UNSPECIFIED.,.F.,.F.)
B_SPLINE_CURVE_WITH_KNOTS((3,3),(0.258079386101495,0.459416258484592),
 .UNSPECIFIED.)
CURVE()
GEOMETRIC_REPRESENTATION_ITEM()
RATIONAL_B_SPLINE_CURVE((1.00161624157848,1.00189253035137,1.00161624157848))
REPRESENTATION_ITEM('')
);
#19059=(
BOUNDED_CURVE()
B_SPLINE_CURVE(2,(#73247,#73248,#73249),.UNSPECIFIED.,.F.,.F.)
B_SPLINE_CURVE_WITH_KNOTS((3,3),(0.0217367286895466,0.0948204552983258),
 .UNSPECIFIED.)
CURVE()
GEOMETRIC_REPRESENTATION_ITEM()
RATIONAL_B_SPLINE_CURVE((1.0000024358556,1.00000531287251,1.))
REPRESENTATION_ITEM('')
);
#19060=(
BOUNDED_CURVE()
B_SPLINE_CURVE(2,(#73301,#73302,#73303),.UNSPECIFIED.,.F.,.F.)
B_SPLINE_CURVE_WITH_KNOTS((3,3),(0.258079386101485,0.459416258484579),
 .UNSPECIFIED.)
CURVE()
GEOMETRIC_REPRESENTATION_ITEM()
RATIONAL_B_SPLINE_CURVE((1.00161624157847,1.00189253035136,1.00161624157847))
REPRESENTATION_ITEM('')
);
#19061=(
BOUNDED_CURVE()
B_SPLINE_CURVE(2,(#73309,#73310,#73311),.UNSPECIFIED.,.F.,.F.)
B_SPLINE_CURVE_WITH_KNOTS((3,3),(0.358747822293043,0.459416258484592),
 .UNSPECIFIED.)
CURVE()
GEOMETRIC_REPRESENTATION_ITEM()
RATIONAL_B_SPLINE_CURVE((1.00175438596492,1.00175438596492,1.00161624157847))
REPRESENTATION_ITEM('')
);
#19062=(
BOUNDED_CURVE()
B_SPLINE_CURVE(2,(#73313,#73314,#73315),.UNSPECIFIED.,.F.,.F.)
B_SPLINE_CURVE_WITH_KNOTS((3,3),(0.258079386101507,0.459416258484599),
 .UNSPECIFIED.)
CURVE()
GEOMETRIC_REPRESENTATION_ITEM()
RATIONAL_B_SPLINE_CURVE((1.00161624157844,1.00189253035133,1.00161624157844))
REPRESENTATION_ITEM('')
);
#19063=(
BOUNDED_CURVE()
B_SPLINE_CURVE(2,(#73317,#73318,#73319),.UNSPECIFIED.,.F.,.F.)
B_SPLINE_CURVE_WITH_KNOTS((3,3),(0.258079386101484,0.459416258484585),
 .UNSPECIFIED.)
CURVE()
GEOMETRIC_REPRESENTATION_ITEM()
RATIONAL_B_SPLINE_CURVE((1.0016162415785,1.0018925303514,1.0016162415785))
REPRESENTATION_ITEM('')
);
#19064=(
BOUNDED_CURVE()
B_SPLINE_CURVE(2,(#73321,#73322,#73323),.UNSPECIFIED.,.F.,.F.)
B_SPLINE_CURVE_WITH_KNOTS((3,3),(0.258079386101501,0.459416258484591),
 .UNSPECIFIED.)
CURVE()
GEOMETRIC_REPRESENTATION_ITEM()
RATIONAL_B_SPLINE_CURVE((1.00161624157844,1.00189253035133,1.00161624157844))
REPRESENTATION_ITEM('')
);
#19065=(
BOUNDED_CURVE()
B_SPLINE_CURVE(2,(#73325,#73326,#73327),.UNSPECIFIED.,.F.,.F.)
B_SPLINE_CURVE_WITH_KNOTS((3,3),(0.258079386101505,0.459416258484602),
 .UNSPECIFIED.)
CURVE()
GEOMETRIC_REPRESENTATION_ITEM()
RATIONAL_B_SPLINE_CURVE((1.00161624157847,1.00189253035136,1.00161624157847))
REPRESENTATION_ITEM('')
);
#19066=(
BOUNDED_CURVE()
B_SPLINE_CURVE(2,(#73329,#73330,#73331),.UNSPECIFIED.,.F.,.F.)
B_SPLINE_CURVE_WITH_KNOTS((3,3),(0.258079386101503,0.459416258484604),
 .UNSPECIFIED.)
CURVE()
GEOMETRIC_REPRESENTATION_ITEM()
RATIONAL_B_SPLINE_CURVE((1.0016162415785,1.0018925303514,1.0016162415785))
REPRESENTATION_ITEM('')
);
#19067=(
BOUNDED_CURVE()
B_SPLINE_CURVE(2,(#73333,#73334,#73335),.UNSPECIFIED.,.F.,.F.)
B_SPLINE_CURVE_WITH_KNOTS((3,3),(0.258079386101503,0.459416258484592),
 .UNSPECIFIED.)
CURVE()
GEOMETRIC_REPRESENTATION_ITEM()
RATIONAL_B_SPLINE_CURVE((1.00161624157844,1.00189253035133,1.00161624157844))
REPRESENTATION_ITEM('')
);
#19068=(
BOUNDED_CURVE()
B_SPLINE_CURVE(2,(#73337,#73338,#73339),.UNSPECIFIED.,.F.,.F.)
B_SPLINE_CURVE_WITH_KNOTS((3,3),(0.258079386101509,0.459416258484598),
 .UNSPECIFIED.)
CURVE()
GEOMETRIC_REPRESENTATION_ITEM()
RATIONAL_B_SPLINE_CURVE((1.00161624157844,1.00189253035133,1.00161624157844))
REPRESENTATION_ITEM('')
);
#19069=(
BOUNDED_CURVE()
B_SPLINE_CURVE(2,(#73341,#73342,#73343),.UNSPECIFIED.,.F.,.F.)
B_SPLINE_CURVE_WITH_KNOTS((3,3),(0.258079386101488,0.459416258484583),
 .UNSPECIFIED.)
CURVE()
GEOMETRIC_REPRESENTATION_ITEM()
RATIONAL_B_SPLINE_CURVE((1.00161624157847,1.00189253035136,1.00161624157847))
REPRESENTATION_ITEM('')
);
#19070=(
BOUNDED_CURVE()
B_SPLINE_CURVE(2,(#73345,#73346,#73347),.UNSPECIFIED.,.F.,.F.)
B_SPLINE_CURVE_WITH_KNOTS((3,3),(0.258079386101497,0.459416258484591),
 .UNSPECIFIED.)
CURVE()
GEOMETRIC_REPRESENTATION_ITEM()
RATIONAL_B_SPLINE_CURVE((1.00161624157847,1.00189253035136,1.00161624157847))
REPRESENTATION_ITEM('')
);
#19071=(
BOUNDED_CURVE()
B_SPLINE_CURVE(2,(#73349,#73350,#73351),.UNSPECIFIED.,.F.,.F.)
B_SPLINE_CURVE_WITH_KNOTS((3,3),(0.258079386101488,0.459416258484577),
 .UNSPECIFIED.)
CURVE()
GEOMETRIC_REPRESENTATION_ITEM()
RATIONAL_B_SPLINE_CURVE((1.00161624157844,1.00189253035133,1.00161624157844))
REPRESENTATION_ITEM('')
);
#19072=(
BOUNDED_CURVE()
B_SPLINE_CURVE(2,(#73353,#73354,#73355),.UNSPECIFIED.,.F.,.F.)
B_SPLINE_CURVE_WITH_KNOTS((3,3),(0.258079386101483,0.459416258484584),
 .UNSPECIFIED.)
CURVE()
GEOMETRIC_REPRESENTATION_ITEM()
RATIONAL_B_SPLINE_CURVE((1.0016162415785,1.0018925303514,1.0016162415785))
REPRESENTATION_ITEM('')
);
#19073=(
BOUNDED_CURVE()
B_SPLINE_CURVE(2,(#73357,#73358,#73359),.UNSPECIFIED.,.F.,.F.)
B_SPLINE_CURVE_WITH_KNOTS((3,3),(0.258079386101508,0.459416258484598),
 .UNSPECIFIED.)
CURVE()
GEOMETRIC_REPRESENTATION_ITEM()
RATIONAL_B_SPLINE_CURVE((1.00161624157844,1.00189253035133,1.00161624157844))
REPRESENTATION_ITEM('')
);
#19074=(
BOUNDED_CURVE()
B_SPLINE_CURVE(2,(#73361,#73362,#73363),.UNSPECIFIED.,.F.,.F.)
B_SPLINE_CURVE_WITH_KNOTS((3,3),(0.258079386101503,0.459416258484604),
 .UNSPECIFIED.)
CURVE()
GEOMETRIC_REPRESENTATION_ITEM()
RATIONAL_B_SPLINE_CURVE((1.0016162415785,1.0018925303514,1.0016162415785))
REPRESENTATION_ITEM('')
);
#19075=(
BOUNDED_CURVE()
B_SPLINE_CURVE(2,(#73365,#73366,#73367),.UNSPECIFIED.,.F.,.F.)
B_SPLINE_CURVE_WITH_KNOTS((3,3),(0.258079386101498,0.459416258484587),
 .UNSPECIFIED.)
CURVE()
GEOMETRIC_REPRESENTATION_ITEM()
RATIONAL_B_SPLINE_CURVE((1.00161624157844,1.00189253035133,1.00161624157844))
REPRESENTATION_ITEM('')
);
#19076=(
BOUNDED_CURVE()
B_SPLINE_CURVE(2,(#73369,#73370,#73371),.UNSPECIFIED.,.F.,.F.)
B_SPLINE_CURVE_WITH_KNOTS((3,3),(0.258079386101498,0.459416258484587),
 .UNSPECIFIED.)
CURVE()
GEOMETRIC_REPRESENTATION_ITEM()
RATIONAL_B_SPLINE_CURVE((1.00161624157844,1.00189253035133,1.00161624157844))
REPRESENTATION_ITEM('')
);
#19077=(
BOUNDED_CURVE()
B_SPLINE_CURVE(2,(#73373,#73374,#73375),.UNSPECIFIED.,.F.,.F.)
B_SPLINE_CURVE_WITH_KNOTS((3,3),(0.258079386101507,0.459416258484602),
 .UNSPECIFIED.)
CURVE()
GEOMETRIC_REPRESENTATION_ITEM()
RATIONAL_B_SPLINE_CURVE((1.00161624157847,1.00189253035136,1.00161624157847))
REPRESENTATION_ITEM('')
);
#19078=(
BOUNDED_CURVE()
B_SPLINE_CURVE(2,(#73377,#73378,#73379),.UNSPECIFIED.,.F.,.F.)
B_SPLINE_CURVE_WITH_KNOTS((3,3),(0.258079386101488,0.459416258484583),
 .UNSPECIFIED.)
CURVE()
GEOMETRIC_REPRESENTATION_ITEM()
RATIONAL_B_SPLINE_CURVE((1.00161624157847,1.00189253035136,1.00161624157847))
REPRESENTATION_ITEM('')
);
#19079=(
BOUNDED_CURVE()
B_SPLINE_CURVE(2,(#73382,#73383,#73384),.UNSPECIFIED.,.F.,.F.)
B_SPLINE_CURVE_WITH_KNOTS((3,3),(0.0217367286897871,0.0948204552983253),
 .UNSPECIFIED.)
CURVE()
GEOMETRIC_REPRESENTATION_ITEM()
RATIONAL_B_SPLINE_CURVE((1.00000243583551,1.00000531282869,1.))
REPRESENTATION_ITEM('')
);
#19080=(
BOUNDED_CURVE()
B_SPLINE_CURVE(2,(#73387,#73388,#73389),.UNSPECIFIED.,.F.,.F.)
B_SPLINE_CURVE_WITH_KNOTS((3,3),(0.258079386101499,0.459416258484588),
 .UNSPECIFIED.)
CURVE()
GEOMETRIC_REPRESENTATION_ITEM()
RATIONAL_B_SPLINE_CURVE((1.00161624157844,1.00189253035133,1.00161624157844))
REPRESENTATION_ITEM('')
);
#19081=(
BOUNDED_CURVE()
B_SPLINE_CURVE(2,(#73391,#73392,#73393),.UNSPECIFIED.,.F.,.F.)
B_SPLINE_CURVE_WITH_KNOTS((3,3),(0.258079386101495,0.459416258484591),
 .UNSPECIFIED.)
CURVE()
GEOMETRIC_REPRESENTATION_ITEM()
RATIONAL_B_SPLINE_CURVE((1.00161624157847,1.00189253035136,1.00161624157847))
REPRESENTATION_ITEM('')
);
#19082=(
BOUNDED_CURVE()
B_SPLINE_CURVE(2,(#73395,#73396,#73397),.UNSPECIFIED.,.F.,.F.)
B_SPLINE_CURVE_WITH_KNOTS((3,3),(0.258079386101508,0.459416258484599),
 .UNSPECIFIED.)
CURVE()
GEOMETRIC_REPRESENTATION_ITEM()
RATIONAL_B_SPLINE_CURVE((1.00161624157844,1.00189253035133,1.00161624157844))
REPRESENTATION_ITEM('')
);
#19083=(
BOUNDED_CURVE()
B_SPLINE_CURVE(2,(#73399,#73400,#73401),.UNSPECIFIED.,.F.,.F.)
B_SPLINE_CURVE_WITH_KNOTS((3,3),(0.258079386101511,0.459416258484596),
 .UNSPECIFIED.)
CURVE()
GEOMETRIC_REPRESENTATION_ITEM()
RATIONAL_B_SPLINE_CURVE((1.00161624157842,1.0018925303513,1.00161624157842))
REPRESENTATION_ITEM('')
);
#19084=(
BOUNDED_CURVE()
B_SPLINE_CURVE(2,(#73403,#73404,#73405),.UNSPECIFIED.,.F.,.F.)
B_SPLINE_CURVE_WITH_KNOTS((3,3),(0.25807938610151,0.459416258484599),
 .UNSPECIFIED.)
CURVE()
GEOMETRIC_REPRESENTATION_ITEM()
RATIONAL_B_SPLINE_CURVE((1.00161624157844,1.00189253035133,1.00161624157844))
REPRESENTATION_ITEM('')
);
#19085=(
BOUNDED_CURVE()
B_SPLINE_CURVE(2,(#73407,#73408,#73409),.UNSPECIFIED.,.F.,.F.)
B_SPLINE_CURVE_WITH_KNOTS((3,3),(0.258079386101508,0.459416258484599),
 .UNSPECIFIED.)
CURVE()
GEOMETRIC_REPRESENTATION_ITEM()
RATIONAL_B_SPLINE_CURVE((1.00161624157844,1.00189253035133,1.00161624157844))
REPRESENTATION_ITEM('')
);
#19086=(
BOUNDED_CURVE()
B_SPLINE_CURVE(2,(#73411,#73412,#73413),.UNSPECIFIED.,.F.,.F.)
B_SPLINE_CURVE_WITH_KNOTS((3,3),(0.258079386101509,0.459416258484598),
 .UNSPECIFIED.)
CURVE()
GEOMETRIC_REPRESENTATION_ITEM()
RATIONAL_B_SPLINE_CURVE((1.00161624157844,1.00189253035133,1.00161624157844))
REPRESENTATION_ITEM('')
);
#19087=(
BOUNDED_CURVE()
B_SPLINE_CURVE(2,(#73415,#73416,#73417),.UNSPECIFIED.,.F.,.F.)
B_SPLINE_CURVE_WITH_KNOTS((3,3),(0.258079386101496,0.459416258484592),
 .UNSPECIFIED.)
CURVE()
GEOMETRIC_REPRESENTATION_ITEM()
RATIONAL_B_SPLINE_CURVE((1.00161624157847,1.00189253035136,1.00161624157847))
REPRESENTATION_ITEM('')
);
#19088=(
BOUNDED_CURVE()
B_SPLINE_CURVE(2,(#73419,#73420,#73421),.UNSPECIFIED.,.F.,.F.)
B_SPLINE_CURVE_WITH_KNOTS((3,3),(0.258079386101486,0.45941625848458),
 .UNSPECIFIED.)
CURVE()
GEOMETRIC_REPRESENTATION_ITEM()
RATIONAL_B_SPLINE_CURVE((1.00161624157847,1.00189253035136,1.00161624157847))
REPRESENTATION_ITEM('')
);
#19089=(
BOUNDED_CURVE()
B_SPLINE_CURVE(2,(#73423,#73424,#73425),.UNSPECIFIED.,.F.,.F.)
B_SPLINE_CURVE_WITH_KNOTS((3,3),(0.258079386101509,0.459416258484599),
 .UNSPECIFIED.)
CURVE()
GEOMETRIC_REPRESENTATION_ITEM()
RATIONAL_B_SPLINE_CURVE((1.00161624157844,1.00189253035133,1.00161624157844))
REPRESENTATION_ITEM('')
);
#19090=(
BOUNDED_CURVE()
B_SPLINE_CURVE(2,(#73427,#73428,#73429),.UNSPECIFIED.,.F.,.F.)
B_SPLINE_CURVE_WITH_KNOTS((3,3),(0.258079386101495,0.45941625848459),
 .UNSPECIFIED.)
CURVE()
GEOMETRIC_REPRESENTATION_ITEM()
RATIONAL_B_SPLINE_CURVE((1.00161624157847,1.00189253035136,1.00161624157847))
REPRESENTATION_ITEM('')
);
#19091=(
BOUNDED_CURVE()
B_SPLINE_CURVE(2,(#73431,#73432,#73433),.UNSPECIFIED.,.F.,.F.)
B_SPLINE_CURVE_WITH_KNOTS((3,3),(0.258079386101507,0.459416258484603),
 .UNSPECIFIED.)
CURVE()
GEOMETRIC_REPRESENTATION_ITEM()
RATIONAL_B_SPLINE_CURVE((1.00161624157847,1.00189253035136,1.00161624157847))
REPRESENTATION_ITEM('')
);
#19092=(
BOUNDED_CURVE()
B_SPLINE_CURVE(2,(#73435,#73436,#73437),.UNSPECIFIED.,.F.,.F.)
B_SPLINE_CURVE_WITH_KNOTS((3,3),(0.258079386101498,0.459416258484587),
 .UNSPECIFIED.)
CURVE()
GEOMETRIC_REPRESENTATION_ITEM()
RATIONAL_B_SPLINE_CURVE((1.00161624157844,1.00189253035133,1.00161624157844))
REPRESENTATION_ITEM('')
);
#19093=(
BOUNDED_CURVE()
B_SPLINE_CURVE(2,(#73439,#73440,#73441),.UNSPECIFIED.,.F.,.F.)
B_SPLINE_CURVE_WITH_KNOTS((3,3),(0.258079386101511,0.4594162584846),
 .UNSPECIFIED.)
CURVE()
GEOMETRIC_REPRESENTATION_ITEM()
RATIONAL_B_SPLINE_CURVE((1.00161624157844,1.00189253035133,1.00161624157844))
REPRESENTATION_ITEM('')
);
#19094=(
BOUNDED_CURVE()
B_SPLINE_CURVE(2,(#73443,#73444,#73445),.UNSPECIFIED.,.F.,.F.)
B_SPLINE_CURVE_WITH_KNOTS((3,3),(0.258079386101507,0.459416258484602),
 .UNSPECIFIED.)
CURVE()
GEOMETRIC_REPRESENTATION_ITEM()
RATIONAL_B_SPLINE_CURVE((1.00161624157847,1.00189253035136,1.00161624157847))
REPRESENTATION_ITEM('')
);
#19095=(
BOUNDED_CURVE()
B_SPLINE_CURVE(2,(#73447,#73448,#73449),.UNSPECIFIED.,.F.,.F.)
B_SPLINE_CURVE_WITH_KNOTS((3,3),(0.258079386101496,0.459416258484591),
 .UNSPECIFIED.)
CURVE()
GEOMETRIC_REPRESENTATION_ITEM()
RATIONAL_B_SPLINE_CURVE((1.00161624157847,1.00189253035136,1.00161624157847))
REPRESENTATION_ITEM('')
);
#19096=(
BOUNDED_CURVE()
B_SPLINE_CURVE(2,(#73451,#73452,#73453),.UNSPECIFIED.,.F.,.F.)
B_SPLINE_CURVE_WITH_KNOTS((3,3),(0.258079386101497,0.358747822293043),
 .UNSPECIFIED.)
CURVE()
GEOMETRIC_REPRESENTATION_ITEM()
RATIONAL_B_SPLINE_CURVE((1.00161624157847,1.00175438596492,1.00175438596492))
REPRESENTATION_ITEM('')
);
#19097=(
BOUNDED_CURVE()
B_SPLINE_CURVE(2,(#73511,#73512,#73513),.UNSPECIFIED.,.F.,.F.)
B_SPLINE_CURVE_WITH_KNOTS((3,3),(0.0217367286898259,0.0948204552983258),
 .UNSPECIFIED.)
CURVE()
GEOMETRIC_REPRESENTATION_ITEM()
RATIONAL_B_SPLINE_CURVE((1.00000243584041,1.00000531283939,1.))
REPRESENTATION_ITEM('')
);
#19098=(
BOUNDED_CURVE()
B_SPLINE_CURVE(2,(#73622,#73623,#73624),.UNSPECIFIED.,.F.,.F.)
B_SPLINE_CURVE_WITH_KNOTS((3,3),(0.0217367286902918,0.0948204552983266),
 .UNSPECIFIED.)
CURVE()
GEOMETRIC_REPRESENTATION_ITEM()
RATIONAL_B_SPLINE_CURVE((1.00000243583421,1.00000531282586,1.))
REPRESENTATION_ITEM('')
);
#19099=(
BOUNDED_CURVE()
B_SPLINE_CURVE(2,(#73733,#73734,#73735),.UNSPECIFIED.,.F.,.F.)
B_SPLINE_CURVE_WITH_KNOTS((3,3),(0.0217367286900204,0.0948204552983262),
 .UNSPECIFIED.)
CURVE()
GEOMETRIC_REPRESENTATION_ITEM()
RATIONAL_B_SPLINE_CURVE((1.0000024358438,1.00000531284678,1.))
REPRESENTATION_ITEM('')
);
#19100=(
BOUNDED_CURVE()
B_SPLINE_CURVE(2,(#73844,#73845,#73846),.UNSPECIFIED.,.F.,.F.)
B_SPLINE_CURVE_WITH_KNOTS((3,3),(0.021736728689681,0.0948204552983264),
 .UNSPECIFIED.)
CURVE()
GEOMETRIC_REPRESENTATION_ITEM()
RATIONAL_B_SPLINE_CURVE((1.0000024358479,1.00000531285573,1.))
REPRESENTATION_ITEM('')
);
#19101=(
BOUNDED_CURVE()
B_SPLINE_CURVE(2,(#73955,#73956,#73957),.UNSPECIFIED.,.F.,.F.)
B_SPLINE_CURVE_WITH_KNOTS((3,3),(0.0217367286903269,0.0948204552983259),
 .UNSPECIFIED.)
CURVE()
GEOMETRIC_REPRESENTATION_ITEM()
RATIONAL_B_SPLINE_CURVE((1.00000243583057,1.00000531281792,1.))
REPRESENTATION_ITEM('')
);
#19102=(
BOUNDED_CURVE()
B_SPLINE_CURVE(2,(#74066,#74067,#74068),.UNSPECIFIED.,.F.,.F.)
B_SPLINE_CURVE_WITH_KNOTS((3,3),(0.0217367286899795,0.0948204552983258),
 .UNSPECIFIED.)
CURVE()
GEOMETRIC_REPRESENTATION_ITEM()
RATIONAL_B_SPLINE_CURVE((1.0000024358404,1.00000531283936,1.))
REPRESENTATION_ITEM('')
);
#19103=(
BOUNDED_CURVE()
B_SPLINE_CURVE(2,(#74177,#74178,#74179),.UNSPECIFIED.,.F.,.F.)
B_SPLINE_CURVE_WITH_KNOTS((3,3),(0.021736728689809,0.0948204552983252),
 .UNSPECIFIED.)
CURVE()
GEOMETRIC_REPRESENTATION_ITEM()
RATIONAL_B_SPLINE_CURVE((1.00000243583744,1.00000531283292,1.))
REPRESENTATION_ITEM('')
);
#19104=(
BOUNDED_CURVE()
B_SPLINE_CURVE(2,(#74288,#74289,#74290),.UNSPECIFIED.,.F.,.F.)
B_SPLINE_CURVE_WITH_KNOTS((3,3),(0.0217367286899008,0.0948204552983264),
 .UNSPECIFIED.)
CURVE()
GEOMETRIC_REPRESENTATION_ITEM()
RATIONAL_B_SPLINE_CURVE((1.00000243583837,1.00000531283495,1.))
REPRESENTATION_ITEM('')
);
#19105=(
BOUNDED_CURVE()
B_SPLINE_CURVE(2,(#74399,#74400,#74401),.UNSPECIFIED.,.F.,.F.)
B_SPLINE_CURVE_WITH_KNOTS((3,3),(0.0217367286899683,0.0948204552983256),
 .UNSPECIFIED.)
CURVE()
GEOMETRIC_REPRESENTATION_ITEM()
RATIONAL_B_SPLINE_CURVE((1.00000243584639,1.00000531285242,1.))
REPRESENTATION_ITEM('')
);
#19106=(
BOUNDED_CURVE()
B_SPLINE_CURVE(2,(#74510,#74511,#74512),.UNSPECIFIED.,.F.,.F.)
B_SPLINE_CURVE_WITH_KNOTS((3,3),(0.0217367286898393,0.0948204552983254),
 .UNSPECIFIED.)
CURVE()
GEOMETRIC_REPRESENTATION_ITEM()
RATIONAL_B_SPLINE_CURVE((1.00000243584073,1.00000531284008,1.))
REPRESENTATION_ITEM('')
);
#19107=(
BOUNDED_CURVE()
B_SPLINE_CURVE(2,(#74621,#74622,#74623),.UNSPECIFIED.,.F.,.F.)
B_SPLINE_CURVE_WITH_KNOTS((3,3),(0.0217367286899436,0.0948204552983261),
 .UNSPECIFIED.)
CURVE()
GEOMETRIC_REPRESENTATION_ITEM()
RATIONAL_B_SPLINE_CURVE((1.0000024358327,1.00000531282257,1.))
REPRESENTATION_ITEM('')
);
#19108=(
BOUNDED_CURVE()
B_SPLINE_CURVE(2,(#74732,#74733,#74734),.UNSPECIFIED.,.F.,.F.)
B_SPLINE_CURVE_WITH_KNOTS((3,3),(0.0217367286899227,0.094820455298326),
 .UNSPECIFIED.)
CURVE()
GEOMETRIC_REPRESENTATION_ITEM()
RATIONAL_B_SPLINE_CURVE((1.00000243583775,1.00000531283358,1.))
REPRESENTATION_ITEM('')
);
#19109=(
BOUNDED_CURVE()
B_SPLINE_CURVE(2,(#74843,#74844,#74845),.UNSPECIFIED.,.F.,.F.)
B_SPLINE_CURVE_WITH_KNOTS((3,3),(0.0217367286898759,0.0948204552983263),
 .UNSPECIFIED.)
CURVE()
GEOMETRIC_REPRESENTATION_ITEM()
RATIONAL_B_SPLINE_CURVE((1.00000243584141,1.00000531284156,1.))
REPRESENTATION_ITEM('')
);
#19110=(
BOUNDED_CURVE()
B_SPLINE_CURVE(2,(#74954,#74955,#74956),.UNSPECIFIED.,.F.,.F.)
B_SPLINE_CURVE_WITH_KNOTS((3,3),(0.0217367286898064,0.0948204552983261),
 .UNSPECIFIED.)
CURVE()
GEOMETRIC_REPRESENTATION_ITEM()
RATIONAL_B_SPLINE_CURVE((1.00000243584332,1.00000531284573,1.))
REPRESENTATION_ITEM('')
);
#19111=(
BOUNDED_CURVE()
B_SPLINE_CURVE(2,(#75065,#75066,#75067),.UNSPECIFIED.,.F.,.F.)
B_SPLINE_CURVE_WITH_KNOTS((3,3),(0.0217367286899321,0.0948204552983259),
 .UNSPECIFIED.)
CURVE()
GEOMETRIC_REPRESENTATION_ITEM()
RATIONAL_B_SPLINE_CURVE((1.00000243584617,1.00000531285196,1.))
REPRESENTATION_ITEM('')
);
#19112=(
BOUNDED_CURVE()
B_SPLINE_CURVE(2,(#75176,#75177,#75178),.UNSPECIFIED.,.F.,.F.)
B_SPLINE_CURVE_WITH_KNOTS((3,3),(0.0217367286900994,0.094820455298325),
 .UNSPECIFIED.)
CURVE()
GEOMETRIC_REPRESENTATION_ITEM()
RATIONAL_B_SPLINE_CURVE((1.0000024358338,1.00000531282496,1.))
REPRESENTATION_ITEM('')
);
#19113=(
BOUNDED_CURVE()
B_SPLINE_CURVE(2,(#75287,#75288,#75289),.UNSPECIFIED.,.F.,.F.)
B_SPLINE_CURVE_WITH_KNOTS((3,3),(0.0217367286897137,0.0948204552983262),
 .UNSPECIFIED.)
CURVE()
GEOMETRIC_REPRESENTATION_ITEM()
RATIONAL_B_SPLINE_CURVE((1.00000243584632,1.00000531285229,1.))
REPRESENTATION_ITEM('')
);
#19114=(
BOUNDED_CURVE()
B_SPLINE_CURVE(2,(#75398,#75399,#75400),.UNSPECIFIED.,.F.,.F.)
B_SPLINE_CURVE_WITH_KNOTS((3,3),(0.0217367286899984,0.0948204552983254),
 .UNSPECIFIED.)
CURVE()
GEOMETRIC_REPRESENTATION_ITEM()
RATIONAL_B_SPLINE_CURVE((1.00000243584651,1.0000053128527,1.))
REPRESENTATION_ITEM('')
);
#19115=(
BOUNDED_CURVE()
B_SPLINE_CURVE(2,(#75509,#75510,#75511),.UNSPECIFIED.,.F.,.F.)
B_SPLINE_CURVE_WITH_KNOTS((3,3),(0.0217367286897552,0.0948204552983258),
 .UNSPECIFIED.)
CURVE()
GEOMETRIC_REPRESENTATION_ITEM()
RATIONAL_B_SPLINE_CURVE((1.00000243584045,1.00000531283947,1.))
REPRESENTATION_ITEM('')
);
#19116=(
BOUNDED_CURVE()
B_SPLINE_CURVE(2,(#75620,#75621,#75622),.UNSPECIFIED.,.F.,.F.)
B_SPLINE_CURVE_WITH_KNOTS((3,3),(0.021736728689794,0.0948204552983258),
 .UNSPECIFIED.)
CURVE()
GEOMETRIC_REPRESENTATION_ITEM()
RATIONAL_B_SPLINE_CURVE((1.00000243584253,1.00000531284402,1.))
REPRESENTATION_ITEM('')
);
#19117=(
BOUNDED_CURVE()
B_SPLINE_CURVE(2,(#75731,#75732,#75733),.UNSPECIFIED.,.F.,.F.)
B_SPLINE_CURVE_WITH_KNOTS((3,3),(0.0217367286900131,0.0948204552983256),
 .UNSPECIFIED.)
CURVE()
GEOMETRIC_REPRESENTATION_ITEM()
RATIONAL_B_SPLINE_CURVE((1.00000243583569,1.00000531282909,1.))
REPRESENTATION_ITEM('')
);
#19118=(
BOUNDED_CURVE()
B_SPLINE_CURVE(2,(#75842,#75843,#75844),.UNSPECIFIED.,.F.,.F.)
B_SPLINE_CURVE_WITH_KNOTS((3,3),(0.0217367286898347,0.0948204552983258),
 .UNSPECIFIED.)
CURVE()
GEOMETRIC_REPRESENTATION_ITEM()
RATIONAL_B_SPLINE_CURVE((1.00000243583206,1.00000531282119,1.))
REPRESENTATION_ITEM('')
);
#19119=(
BOUNDED_CURVE()
B_SPLINE_CURVE(2,(#75953,#75954,#75955),.UNSPECIFIED.,.F.,.F.)
B_SPLINE_CURVE_WITH_KNOTS((3,3),(0.021736728689975,0.0948204552983256),
 .UNSPECIFIED.)
CURVE()
GEOMETRIC_REPRESENTATION_ITEM()
RATIONAL_B_SPLINE_CURVE((1.00000243583644,1.00000531283073,1.))
REPRESENTATION_ITEM('')
);
#19120=(
BOUNDED_CURVE()
B_SPLINE_CURVE(2,(#76064,#76065,#76066),.UNSPECIFIED.,.F.,.F.)
B_SPLINE_CURVE_WITH_KNOTS((3,3),(0.0217367286899247,0.0948204552983257),
 .UNSPECIFIED.)
CURVE()
GEOMETRIC_REPRESENTATION_ITEM()
RATIONAL_B_SPLINE_CURVE((1.00000243584565,1.00000531285082,1.))
REPRESENTATION_ITEM('')
);
#19121=(
BOUNDED_CURVE()
B_SPLINE_CURVE(2,(#76175,#76176,#76177),.UNSPECIFIED.,.F.,.F.)
B_SPLINE_CURVE_WITH_KNOTS((3,3),(0.0217367286899464,0.0948204552983249),
 .UNSPECIFIED.)
CURVE()
GEOMETRIC_REPRESENTATION_ITEM()
RATIONAL_B_SPLINE_CURVE((1.0000024358387,1.00000531283565,1.))
REPRESENTATION_ITEM('')
);
#19122=(
BOUNDED_CURVE()
B_SPLINE_CURVE(2,(#76286,#76287,#76288),.UNSPECIFIED.,.F.,.F.)
B_SPLINE_CURVE_WITH_KNOTS((3,3),(0.0217367286898777,0.0948204552983262),
 .UNSPECIFIED.)
CURVE()
GEOMETRIC_REPRESENTATION_ITEM()
RATIONAL_B_SPLINE_CURVE((1.00000243584005,1.00000531283861,1.))
REPRESENTATION_ITEM('')
);
#19123=(
BOUNDED_CURVE()
B_SPLINE_CURVE(2,(#76397,#76398,#76399),.UNSPECIFIED.,.F.,.F.)
B_SPLINE_CURVE_WITH_KNOTS((3,3),(0.0217367286897134,0.0948204552983253),
 .UNSPECIFIED.)
CURVE()
GEOMETRIC_REPRESENTATION_ITEM()
RATIONAL_B_SPLINE_CURVE((1.00000243584478,1.00000531284892,1.))
REPRESENTATION_ITEM('')
);
#19124=(
BOUNDED_CURVE()
B_SPLINE_CURVE(2,(#76508,#76509,#76510),.UNSPECIFIED.,.F.,.F.)
B_SPLINE_CURVE_WITH_KNOTS((3,3),(0.0217367286895846,0.0948204552983254),
 .UNSPECIFIED.)
CURVE()
GEOMETRIC_REPRESENTATION_ITEM()
RATIONAL_B_SPLINE_CURVE((1.0000024358477,1.00000531285529,1.))
REPRESENTATION_ITEM('')
);
#19125=(
BOUNDED_CURVE()
B_SPLINE_CURVE(2,(#76619,#76620,#76621),.UNSPECIFIED.,.F.,.F.)
B_SPLINE_CURVE_WITH_KNOTS((3,3),(0.0217367286901915,0.0948204552983254),
 .UNSPECIFIED.)
CURVE()
GEOMETRIC_REPRESENTATION_ITEM()
RATIONAL_B_SPLINE_CURVE((1.00000243582364,1.00000531280281,1.))
REPRESENTATION_ITEM('')
);
#19126=(
BOUNDED_CURVE()
B_SPLINE_CURVE(2,(#76730,#76731,#76732),.UNSPECIFIED.,.F.,.F.)
B_SPLINE_CURVE_WITH_KNOTS((3,3),(0.0217367286904276,0.0948204552983253),
 .UNSPECIFIED.)
CURVE()
GEOMETRIC_REPRESENTATION_ITEM()
RATIONAL_B_SPLINE_CURVE((1.00000243583521,1.00000531282805,1.))
REPRESENTATION_ITEM('')
);
#19127=(
BOUNDED_CURVE()
B_SPLINE_CURVE(2,(#76841,#76842,#76843),.UNSPECIFIED.,.F.,.F.)
B_SPLINE_CURVE_WITH_KNOTS((3,3),(0.0217367286899727,0.0948204552983254),
 .UNSPECIFIED.)
CURVE()
GEOMETRIC_REPRESENTATION_ITEM()
RATIONAL_B_SPLINE_CURVE((1.00000243583722,1.00000531283242,1.))
REPRESENTATION_ITEM('')
);
#19128=(
BOUNDED_CURVE()
B_SPLINE_CURVE(2,(#76952,#76953,#76954),.UNSPECIFIED.,.F.,.F.)
B_SPLINE_CURVE_WITH_KNOTS((3,3),(0.0217367286895435,0.0948204552983251),
 .UNSPECIFIED.)
CURVE()
GEOMETRIC_REPRESENTATION_ITEM()
RATIONAL_B_SPLINE_CURVE((1.00000243584605,1.0000053128517,1.))
REPRESENTATION_ITEM('')
);
#19129=(
BOUNDED_CURVE()
B_SPLINE_CURVE(2,(#77063,#77064,#77065),.UNSPECIFIED.,.F.,.F.)
B_SPLINE_CURVE_WITH_KNOTS((3,3),(0.021736728689847,0.0948204552983251),
 .UNSPECIFIED.)
CURVE()
GEOMETRIC_REPRESENTATION_ITEM()
RATIONAL_B_SPLINE_CURVE((1.00000243585107,1.00000531286265,1.))
REPRESENTATION_ITEM('')
);
#19130=(
BOUNDED_CURVE()
B_SPLINE_CURVE(2,(#77174,#77175,#77176),.UNSPECIFIED.,.F.,.F.)
B_SPLINE_CURVE_WITH_KNOTS((3,3),(0.0217367286902175,0.0948204552983246),
 .UNSPECIFIED.)
CURVE()
GEOMETRIC_REPRESENTATION_ITEM()
RATIONAL_B_SPLINE_CURVE((1.00000243582944,1.00000531281547,1.))
REPRESENTATION_ITEM('')
);
#19131=(
BOUNDED_CURVE()
B_SPLINE_CURVE(2,(#77339,#77340,#77341),.UNSPECIFIED.,.F.,.F.)
B_SPLINE_CURVE_WITH_KNOTS((3,3),(0.0217367286901568,0.0948204552983253),
 .UNSPECIFIED.)
CURVE()
GEOMETRIC_REPRESENTATION_ITEM()
RATIONAL_B_SPLINE_CURVE((1.00000243582781,1.00000531281191,1.))
REPRESENTATION_ITEM('')
);
#19574=CIRCLE('',#51190,39.6);
#19575=CIRCLE('',#51192,39.6);
#19576=CIRCLE('',#51194,39.6);
#19577=CIRCLE('',#51196,39.6);
#19578=CIRCLE('',#51198,39.6);
#19579=CIRCLE('',#51200,39.6);
#19580=CIRCLE('',#51202,39.6);
#19581=CIRCLE('',#51204,39.6);
#19582=CIRCLE('',#51206,39.6);
#19583=CIRCLE('',#51208,39.6);
#19584=CIRCLE('',#51210,39.6);
#19585=CIRCLE('',#51212,39.6);
#19586=CIRCLE('',#51214,39.6);
#19587=CIRCLE('',#51216,39.6);
#19588=CIRCLE('',#51218,39.6);
#19589=CIRCLE('',#51220,39.6);
#19590=CIRCLE('',#51222,39.6);
#19591=CIRCLE('',#51224,39.6);
#19592=CIRCLE('',#51226,39.6);
#19593=CIRCLE('',#51228,39.6);
#19594=CIRCLE('',#51230,39.6);
#19595=CIRCLE('',#51232,39.6);
#19596=CIRCLE('',#51234,39.6);
#19597=CIRCLE('',#51236,39.6);
#19598=CIRCLE('',#51238,39.6);
#19599=CIRCLE('',#51240,39.6);
#19600=CIRCLE('',#51242,39.6);
#19601=CIRCLE('',#51244,39.6);
#19602=CIRCLE('',#51246,39.6);
#19603=CIRCLE('',#51248,39.6);
#19604=CIRCLE('',#51250,39.6);
#19605=CIRCLE('',#51252,39.6);
#19606=CIRCLE('',#51254,39.6);
#19607=CIRCLE('',#51256,39.6);
#19608=CIRCLE('',#51258,39.6);
#19609=CIRCLE('',#51260,39.6);
#19610=CIRCLE('',#51370,39.6);
#19611=CIRCLE('',#51372,39.6);
#19612=CIRCLE('',#51374,39.6);
#19613=CIRCLE('',#51376,39.6);
#19614=CIRCLE('',#51378,39.6);
#19615=CIRCLE('',#51380,39.6);
#19616=CIRCLE('',#51382,39.6);
#19617=CIRCLE('',#51384,39.6);
#19618=CIRCLE('',#51386,39.6);
#19619=CIRCLE('',#51388,39.6);
#19620=CIRCLE('',#51390,39.6);
#19621=CIRCLE('',#51392,39.6);
#19622=CIRCLE('',#51394,39.6);
#19623=CIRCLE('',#51396,39.6);
#19624=CIRCLE('',#51398,39.6);
#19625=CIRCLE('',#51400,39.6);
#19626=CIRCLE('',#51402,39.6);
#19627=CIRCLE('',#51404,39.6);
#19628=CIRCLE('',#51406,39.6);
#19629=CIRCLE('',#51408,39.6);
#19630=CIRCLE('',#51410,39.6);
#19631=CIRCLE('',#51412,39.6);
#19632=CIRCLE('',#51414,39.6);
#19633=CIRCLE('',#51416,39.6);
#19634=CIRCLE('',#51418,39.6);
#19635=CIRCLE('',#51420,39.6);
#19636=CIRCLE('',#51422,39.6);
#19637=CIRCLE('',#51424,39.6);
#19638=CIRCLE('',#51426,39.6);
#19639=CIRCLE('',#51428,39.6);
#19640=CIRCLE('',#51430,39.6);
#19641=CIRCLE('',#51432,39.6);
#19642=CIRCLE('',#51434,39.6);
#19643=CIRCLE('',#51436,39.6);
#19644=CIRCLE('',#51438,39.6);
#19645=CIRCLE('',#51440,39.6);
#19646=CIRCLE('',#51742,42.9);
#19647=CIRCLE('',#51743,42.3);
#19648=CIRCLE('',#51744,42.3);
#19649=CIRCLE('',#51745,42.3);
#19650=CIRCLE('',#51746,42.3);
#19651=CIRCLE('',#51747,42.3);
#19652=CIRCLE('',#51748,42.3);
#19653=CIRCLE('',#51749,42.3);
#19654=CIRCLE('',#51750,42.3);
#19655=CIRCLE('',#51751,42.3);
#19656=CIRCLE('',#51752,42.3);
#19657=CIRCLE('',#51753,42.3);
#19658=CIRCLE('',#51754,42.3);
#19659=CIRCLE('',#51755,42.3);
#19660=CIRCLE('',#51756,42.3);
#19661=CIRCLE('',#51757,42.3);
#19662=CIRCLE('',#51758,42.3);
#19663=CIRCLE('',#51759,42.3);
#19664=CIRCLE('',#51760,42.3);
#19665=CIRCLE('',#51761,42.3);
#19666=CIRCLE('',#51762,42.3);
#19667=CIRCLE('',#51763,42.3);
#19668=CIRCLE('',#51764,42.3);
#19669=CIRCLE('',#51765,42.3);
#19670=CIRCLE('',#51766,42.3);
#19671=CIRCLE('',#51767,42.3);
#19672=CIRCLE('',#51768,42.3);
#19673=CIRCLE('',#51769,42.3);
#19674=CIRCLE('',#51770,42.3);
#19675=CIRCLE('',#51771,42.3);
#19676=CIRCLE('',#51772,42.3);
#19677=CIRCLE('',#51773,42.3);
#19678=CIRCLE('',#51774,42.3);
#19679=CIRCLE('',#51775,42.3);
#19680=CIRCLE('',#51776,42.3);
#19681=CIRCLE('',#51777,42.3);
#19682=CIRCLE('',#51778,42.3);
#19683=CIRCLE('',#51780,42.3);
#19684=CIRCLE('',#51831,42.3);
#19685=CIRCLE('',#51882,42.3);
#19686=CIRCLE('',#51933,42.3);
#19687=CIRCLE('',#51984,42.3);
#19688=CIRCLE('',#52035,42.3);
#19689=CIRCLE('',#52086,42.3);
#19690=CIRCLE('',#52137,42.3);
#19691=CIRCLE('',#52188,42.3);
#19692=CIRCLE('',#52239,42.3);
#19693=CIRCLE('',#52290,42.3);
#19694=CIRCLE('',#52341,42.3);
#19695=CIRCLE('',#52392,42.3);
#19696=CIRCLE('',#52443,42.3);
#19697=CIRCLE('',#52494,42.3);
#19698=CIRCLE('',#52545,42.3);
#19699=CIRCLE('',#52596,42.3);
#19700=CIRCLE('',#52647,42.3);
#19701=CIRCLE('',#52698,42.3);
#19702=CIRCLE('',#52749,42.3);
#19703=CIRCLE('',#52800,42.3);
#19704=CIRCLE('',#52851,42.3);
#19705=CIRCLE('',#52902,42.3);
#19706=CIRCLE('',#52953,42.3);
#19707=CIRCLE('',#53004,42.3);
#19708=CIRCLE('',#53055,42.3);
#19709=CIRCLE('',#53106,42.3);
#19710=CIRCLE('',#53157,42.3);
#19711=CIRCLE('',#53208,42.3);
#19712=CIRCLE('',#53259,42.3);
#19713=CIRCLE('',#53310,42.3);
#19714=CIRCLE('',#53361,42.3);
#19715=CIRCLE('',#53412,42.3);
#19716=CIRCLE('',#53463,42.3);
#19717=CIRCLE('',#53514,42.3);
#19718=CIRCLE('',#53566,42.3);
#19719=CIRCLE('',#53567,42.9);
#19720=CIRCLE('',#53569,47.1);
#19721=CIRCLE('',#53570,47.6321401698912);
#19722=CIRCLE('',#53571,47.6321401698912);
#19723=CIRCLE('',#53573,50.6631501381961);
#19724=CIRCLE('',#53574,50.6631501381961);
#19725=CIRCLE('',#53577,6.);
#19726=CIRCLE('',#53578,51.);
#19727=CIRCLE('',#53579,51.);
#19728=CIRCLE('',#53581,51.);
#19729=CIRCLE('',#53583,46.5);
#19730=CIRCLE('',#53584,0.4);
#19731=CIRCLE('',#53585,46.9);
#19732=CIRCLE('',#53586,46.5);
#19733=CIRCLE('',#53588,46.5);
#19734=CIRCLE('',#53589,46.5);
#19735=CIRCLE('',#53591,50.4);
#19736=CIRCLE('',#53593,46.9);
#19737=CIRCLE('',#53594,0.4);
#19738=CIRCLE('',#53596,50.);
#19739=CIRCLE('',#53599,49.7);
#19740=CIRCLE('',#53601,50.5);
#19741=CIRCLE('',#53603,50.5);
#19742=CIRCLE('',#53606,50.4);
#20324=VERTEX_POINT('',#68261);
#20325=VERTEX_POINT('',#68262);
#20326=VERTEX_POINT('',#68264);
#20327=VERTEX_POINT('',#68268);
#20328=VERTEX_POINT('',#68276);
#20329=VERTEX_POINT('',#68277);
#20330=VERTEX_POINT('',#68279);
#20331=VERTEX_POINT('',#68283);
#20332=VERTEX_POINT('',#68291);
#20333=VERTEX_POINT('',#68292);
#20334=VERTEX_POINT('',#68294);
#20335=VERTEX_POINT('',#68298);
#20336=VERTEX_POINT('',#68306);
#20337=VERTEX_POINT('',#68307);
#20338=VERTEX_POINT('',#68309);
#20339=VERTEX_POINT('',#68313);
#20340=VERTEX_POINT('',#68321);
#20341=VERTEX_POINT('',#68322);
#20342=VERTEX_POINT('',#68324);
#20343=VERTEX_POINT('',#68328);
#20344=VERTEX_POINT('',#68336);
#20345=VERTEX_POINT('',#68337);
#20346=VERTEX_POINT('',#68339);
#20347=VERTEX_POINT('',#68343);
#20348=VERTEX_POINT('',#68351);
#20349=VERTEX_POINT('',#68352);
#20350=VERTEX_POINT('',#68354);
#20351=VERTEX_POINT('',#68358);
#20352=VERTEX_POINT('',#68366);
#20353=VERTEX_POINT('',#68367);
#20354=VERTEX_POINT('',#68369);
#20355=VERTEX_POINT('',#68373);
#20356=VERTEX_POINT('',#68381);
#20357=VERTEX_POINT('',#68382);
#20358=VERTEX_POINT('',#68384);
#20359=VERTEX_POINT('',#68388);
#20360=VERTEX_POINT('',#68396);
#20361=VERTEX_POINT('',#68397);
#20362=VERTEX_POINT('',#68399);
#20363=VERTEX_POINT('',#68403);
#20364=VERTEX_POINT('',#68411);
#20365=VERTEX_POINT('',#68412);
#20366=VERTEX_POINT('',#68414);
#20367=VERTEX_POINT('',#68418);
#20368=VERTEX_POINT('',#68426);
#20369=VERTEX_POINT('',#68427);
#20370=VERTEX_POINT('',#68429);
#20371=VERTEX_POINT('',#68433);
#20372=VERTEX_POINT('',#68441);
#20373=VERTEX_POINT('',#68442);
#20374=VERTEX_POINT('',#68444);
#20375=VERTEX_POINT('',#68448);
#20376=VERTEX_POINT('',#68456);
#20377=VERTEX_POINT('',#68457);
#20378=VERTEX_POINT('',#68459);
#20379=VERTEX_POINT('',#68463);
#20380=VERTEX_POINT('',#68471);
#20381=VERTEX_POINT('',#68472);
#20382=VERTEX_POINT('',#68474);
#20383=VERTEX_POINT('',#68478);
#20384=VERTEX_POINT('',#68486);
#20385=VERTEX_POINT('',#68487);
#20386=VERTEX_POINT('',#68489);
#20387=VERTEX_POINT('',#68493);
#20388=VERTEX_POINT('',#68501);
#20389=VERTEX_POINT('',#68502);
#20390=VERTEX_POINT('',#68504);
#20391=VERTEX_POINT('',#68508);
#20392=VERTEX_POINT('',#68516);
#20393=VERTEX_POINT('',#68517);
#20394=VERTEX_POINT('',#68519);
#20395=VERTEX_POINT('',#68523);
#20396=VERTEX_POINT('',#68531);
#20397=VERTEX_POINT('',#68532);
#20398=VERTEX_POINT('',#68534);
#20399=VERTEX_POINT('',#68538);
#20400=VERTEX_POINT('',#68546);
#20401=VERTEX_POINT('',#68547);
#20402=VERTEX_POINT('',#68549);
#20403=VERTEX_POINT('',#68553);
#20404=VERTEX_POINT('',#68561);
#20405=VERTEX_POINT('',#68562);
#20406=VERTEX_POINT('',#68564);
#20407=VERTEX_POINT('',#68568);
#20408=VERTEX_POINT('',#68576);
#20409=VERTEX_POINT('',#68577);
#20410=VERTEX_POINT('',#68579);
#20411=VERTEX_POINT('',#68583);
#20412=VERTEX_POINT('',#68591);
#20413=VERTEX_POINT('',#68592);
#20414=VERTEX_POINT('',#68594);
#20415=VERTEX_POINT('',#68598);
#20416=VERTEX_POINT('',#68606);
#20417=VERTEX_POINT('',#68607);
#20418=VERTEX_POINT('',#68609);
#20419=VERTEX_POINT('',#68613);
#20420=VERTEX_POINT('',#68621);
#20421=VERTEX_POINT('',#68622);
#20422=VERTEX_POINT('',#68624);
#20423=VERTEX_POINT('',#68628);
#20424=VERTEX_POINT('',#68636);
#20425=VERTEX_POINT('',#68637);
#20426=VERTEX_POINT('',#68639);
#20427=VERTEX_POINT('',#68643);
#20428=VERTEX_POINT('',#68651);
#20429=VERTEX_POINT('',#68652);
#20430=VERTEX_POINT('',#68654);
#20431=VERTEX_POINT('',#68658);
#20432=VERTEX_POINT('',#68666);
#20433=VERTEX_POINT('',#68667);
#20434=VERTEX_POINT('',#68669);
#20435=VERTEX_POINT('',#68673);
#20436=VERTEX_POINT('',#68681);
#20437=VERTEX_POINT('',#68682);
#20438=VERTEX_POINT('',#68684);
#20439=VERTEX_POINT('',#68688);
#20440=VERTEX_POINT('',#68696);
#20441=VERTEX_POINT('',#68697);
#20442=VERTEX_POINT('',#68699);
#20443=VERTEX_POINT('',#68703);
#20444=VERTEX_POINT('',#68711);
#20445=VERTEX_POINT('',#68712);
#20446=VERTEX_POINT('',#68714);
#20447=VERTEX_POINT('',#68718);
#20448=VERTEX_POINT('',#68726);
#20449=VERTEX_POINT('',#68727);
#20450=VERTEX_POINT('',#68729);
#20451=VERTEX_POINT('',#68733);
#20452=VERTEX_POINT('',#68741);
#20453=VERTEX_POINT('',#68742);
#20454=VERTEX_POINT('',#68744);
#20455=VERTEX_POINT('',#68748);
#20456=VERTEX_POINT('',#68756);
#20457=VERTEX_POINT('',#68757);
#20458=VERTEX_POINT('',#68759);
#20459=VERTEX_POINT('',#68763);
#20460=VERTEX_POINT('',#68771);
#20461=VERTEX_POINT('',#68772);
#20462=VERTEX_POINT('',#68774);
#20463=VERTEX_POINT('',#68778);
#20464=VERTEX_POINT('',#68786);
#20465=VERTEX_POINT('',#68787);
#20466=VERTEX_POINT('',#68789);
#20467=VERTEX_POINT('',#68793);
#20468=VERTEX_POINT('',#68801);
#20469=VERTEX_POINT('',#68803);
#20470=VERTEX_POINT('',#68805);
#20471=VERTEX_POINT('',#68807);
#20472=VERTEX_POINT('',#68809);
#20473=VERTEX_POINT('',#68811);
#20474=VERTEX_POINT('',#68813);
#20475=VERTEX_POINT('',#68815);
#20476=VERTEX_POINT('',#68817);
#20477=VERTEX_POINT('',#68819);
#20478=VERTEX_POINT('',#68821);
#20479=VERTEX_POINT('',#68823);
#20480=VERTEX_POINT('',#68825);
#20481=VERTEX_POINT('',#68827);
#20482=VERTEX_POINT('',#68829);
#20483=VERTEX_POINT('',#68831);
#20484=VERTEX_POINT('',#68835);
#20485=VERTEX_POINT('',#68837);
#20486=VERTEX_POINT('',#68839);
#20487=VERTEX_POINT('',#68841);
#20488=VERTEX_POINT('',#68843);
#20489=VERTEX_POINT('',#68845);
#20490=VERTEX_POINT('',#68847);
#20491=VERTEX_POINT('',#68849);
#20492=VERTEX_POINT('',#68851);
#20493=VERTEX_POINT('',#68853);
#20494=VERTEX_POINT('',#68855);
#20495=VERTEX_POINT('',#68857);
#20496=VERTEX_POINT('',#68859);
#20497=VERTEX_POINT('',#68861);
#20498=VERTEX_POINT('',#68865);
#20499=VERTEX_POINT('',#68867);
#20500=VERTEX_POINT('',#68869);
#20501=VERTEX_POINT('',#68873);
#20502=VERTEX_POINT('',#68877);
#20503=VERTEX_POINT('',#68879);
#20504=VERTEX_POINT('',#68881);
#20505=VERTEX_POINT('',#68883);
#20506=VERTEX_POINT('',#68885);
#20507=VERTEX_POINT('',#68887);
#20508=VERTEX_POINT('',#68889);
#20509=VERTEX_POINT('',#68891);
#20510=VERTEX_POINT('',#68893);
#20511=VERTEX_POINT('',#68895);
#20512=VERTEX_POINT('',#68897);
#20513=VERTEX_POINT('',#68899);
#20514=VERTEX_POINT('',#68901);
#20515=VERTEX_POINT('',#68903);
#20516=VERTEX_POINT('',#68905);
#20517=VERTEX_POINT('',#68907);
#20518=VERTEX_POINT('',#68911);
#20519=VERTEX_POINT('',#68913);
#20520=VERTEX_POINT('',#68915);
#20521=VERTEX_POINT('',#68917);
#20522=VERTEX_POINT('',#68919);
#20523=VERTEX_POINT('',#68921);
#20524=VERTEX_POINT('',#68923);
#20525=VERTEX_POINT('',#68925);
#20526=VERTEX_POINT('',#68927);
#20527=VERTEX_POINT('',#68929);
#20528=VERTEX_POINT('',#68931);
#20529=VERTEX_POINT('',#68933);
#20530=VERTEX_POINT('',#68935);
#20531=VERTEX_POINT('',#68937);
#20532=VERTEX_POINT('',#68941);
#20533=VERTEX_POINT('',#68943);
#20534=VERTEX_POINT('',#68945);
#20535=VERTEX_POINT('',#68949);
#20536=VERTEX_POINT('',#68953);
#20537=VERTEX_POINT('',#68955);
#20538=VERTEX_POINT('',#68957);
#20539=VERTEX_POINT('',#68959);
#20540=VERTEX_POINT('',#68961);
#20541=VERTEX_POINT('',#68963);
#20542=VERTEX_POINT('',#68965);
#20543=VERTEX_POINT('',#68967);
#20544=VERTEX_POINT('',#68969);
#20545=VERTEX_POINT('',#68971);
#20546=VERTEX_POINT('',#68973);
#20547=VERTEX_POINT('',#68975);
#20548=VERTEX_POINT('',#68977);
#20549=VERTEX_POINT('',#68979);
#20550=VERTEX_POINT('',#68981);
#20551=VERTEX_POINT('',#68983);
#20552=VERTEX_POINT('',#68987);
#20553=VERTEX_POINT('',#68989);
#20554=VERTEX_POINT('',#68991);
#20555=VERTEX_POINT('',#68993);
#20556=VERTEX_POINT('',#68995);
#20557=VERTEX_POINT('',#68997);
#20558=VERTEX_POINT('',#68999);
#20559=VERTEX_POINT('',#69001);
#20560=VERTEX_POINT('',#69003);
#20561=VERTEX_POINT('',#69005);
#20562=VERTEX_POINT('',#69007);
#20563=VERTEX_POINT('',#69009);
#20564=VERTEX_POINT('',#69011);
#20565=VERTEX_POINT('',#69013);
#20566=VERTEX_POINT('',#69017);
#20567=VERTEX_POINT('',#69019);
#20568=VERTEX_POINT('',#69021);
#20569=VERTEX_POINT('',#69025);
#20570=VERTEX_POINT('',#69029);
#20571=VERTEX_POINT('',#69031);
#20572=VERTEX_POINT('',#69033);
#20573=VERTEX_POINT('',#69035);
#20574=VERTEX_POINT('',#69037);
#20575=VERTEX_POINT('',#69039);
#20576=VERTEX_POINT('',#69041);
#20577=VERTEX_POINT('',#69043);
#20578=VERTEX_POINT('',#69045);
#20579=VERTEX_POINT('',#69047);
#20580=VERTEX_POINT('',#69049);
#20581=VERTEX_POINT('',#69051);
#20582=VERTEX_POINT('',#69053);
#20583=VERTEX_POINT('',#69055);
#20584=VERTEX_POINT('',#69057);
#20585=VERTEX_POINT('',#69059);
#20586=VERTEX_POINT('',#69063);
#20587=VERTEX_POINT('',#69065);
#20588=VERTEX_POINT('',#69067);
#20589=VERTEX_POINT('',#69069);
#20590=VERTEX_POINT('',#69071);
#20591=VERTEX_POINT('',#69073);
#20592=VERTEX_POINT('',#69075);
#20593=VERTEX_POINT('',#69077);
#20594=VERTEX_POINT('',#69079);
#20595=VERTEX_POINT('',#69081);
#20596=VERTEX_POINT('',#69083);
#20597=VERTEX_POINT('',#69085);
#20598=VERTEX_POINT('',#69087);
#20599=VERTEX_POINT('',#69089);
#20600=VERTEX_POINT('',#69093);
#20601=VERTEX_POINT('',#69095);
#20602=VERTEX_POINT('',#69097);
#20603=VERTEX_POINT('',#69101);
#20604=VERTEX_POINT('',#69105);
#20605=VERTEX_POINT('',#69107);
#20606=VERTEX_POINT('',#69109);
#20607=VERTEX_POINT('',#69111);
#20608=VERTEX_POINT('',#69113);
#20609=VERTEX_POINT('',#69115);
#20610=VERTEX_POINT('',#69117);
#20611=VERTEX_POINT('',#69119);
#20612=VERTEX_POINT('',#69121);
#20613=VERTEX_POINT('',#69123);
#20614=VERTEX_POINT('',#69125);
#20615=VERTEX_POINT('',#69127);
#20616=VERTEX_POINT('',#69129);
#20617=VERTEX_POINT('',#69131);
#20618=VERTEX_POINT('',#69133);
#20619=VERTEX_POINT('',#69135);
#20620=VERTEX_POINT('',#69139);
#20621=VERTEX_POINT('',#69141);
#20622=VERTEX_POINT('',#69143);
#20623=VERTEX_POINT('',#69145);
#20624=VERTEX_POINT('',#69147);
#20625=VERTEX_POINT('',#69149);
#20626=VERTEX_POINT('',#69151);
#20627=VERTEX_POINT('',#69153);
#20628=VERTEX_POINT('',#69155);
#20629=VERTEX_POINT('',#69157);
#20630=VERTEX_POINT('',#69159);
#20631=VERTEX_POINT('',#69161);
#20632=VERTEX_POINT('',#69163);
#20633=VERTEX_POINT('',#69165);
#20634=VERTEX_POINT('',#69169);
#20635=VERTEX_POINT('',#69171);
#20636=VERTEX_POINT('',#69173);
#20637=VERTEX_POINT('',#69177);
#20638=VERTEX_POINT('',#69181);
#20639=VERTEX_POINT('',#69183);
#20640=VERTEX_POINT('',#69185);
#20641=VERTEX_POINT('',#69187);
#20642=VERTEX_POINT('',#69189);
#20643=VERTEX_POINT('',#69191);
#20644=VERTEX_POINT('',#69193);
#20645=VERTEX_POINT('',#69195);
#20646=VERTEX_POINT('',#69197);
#20647=VERTEX_POINT('',#69199);
#20648=VERTEX_POINT('',#69201);
#20649=VERTEX_POINT('',#69203);
#20650=VERTEX_POINT('',#69205);
#20651=VERTEX_POINT('',#69207);
#20652=VERTEX_POINT('',#69209);
#20653=VERTEX_POINT('',#69211);
#20654=VERTEX_POINT('',#69215);
#20655=VERTEX_POINT('',#69217);
#20656=VERTEX_POINT('',#69219);
#20657=VERTEX_POINT('',#69221);
#20658=VERTEX_POINT('',#69223);
#20659=VERTEX_POINT('',#69225);
#20660=VERTEX_POINT('',#69227);
#20661=VERTEX_POINT('',#69229);
#20662=VERTEX_POINT('',#69231);
#20663=VERTEX_POINT('',#69233);
#20664=VERTEX_POINT('',#69235);
#20665=VERTEX_POINT('',#69237);
#20666=VERTEX_POINT('',#69239);
#20667=VERTEX_POINT('',#69241);
#20668=VERTEX_POINT('',#69245);
#20669=VERTEX_POINT('',#69247);
#20670=VERTEX_POINT('',#69249);
#20671=VERTEX_POINT('',#69253);
#20672=VERTEX_POINT('',#69257);
#20673=VERTEX_POINT('',#69259);
#20674=VERTEX_POINT('',#69261);
#20675=VERTEX_POINT('',#69263);
#20676=VERTEX_POINT('',#69265);
#20677=VERTEX_POINT('',#69267);
#20678=VERTEX_POINT('',#69269);
#20679=VERTEX_POINT('',#69271);
#20680=VERTEX_POINT('',#69273);
#20681=VERTEX_POINT('',#69275);
#20682=VERTEX_POINT('',#69277);
#20683=VERTEX_POINT('',#69279);
#20684=VERTEX_POINT('',#69281);
#20685=VERTEX_POINT('',#69283);
#20686=VERTEX_POINT('',#69285);
#20687=VERTEX_POINT('',#69287);
#20688=VERTEX_POINT('',#69291);
#20689=VERTEX_POINT('',#69293);
#20690=VERTEX_POINT('',#69295);
#20691=VERTEX_POINT('',#69297);
#20692=VERTEX_POINT('',#69299);
#20693=VERTEX_POINT('',#69301);
#20694=VERTEX_POINT('',#69303);
#20695=VERTEX_POINT('',#69305);
#20696=VERTEX_POINT('',#69307);
#20697=VERTEX_POINT('',#69309);
#20698=VERTEX_POINT('',#69311);
#20699=VERTEX_POINT('',#69313);
#20700=VERTEX_POINT('',#69315);
#20701=VERTEX_POINT('',#69317);
#20702=VERTEX_POINT('',#69321);
#20703=VERTEX_POINT('',#69323);
#20704=VERTEX_POINT('',#69325);
#20705=VERTEX_POINT('',#69329);
#20706=VERTEX_POINT('',#69333);
#20707=VERTEX_POINT('',#69335);
#20708=VERTEX_POINT('',#69337);
#20709=VERTEX_POINT('',#69339);
#20710=VERTEX_POINT('',#69341);
#20711=VERTEX_POINT('',#69343);
#20712=VERTEX_POINT('',#69345);
#20713=VERTEX_POINT('',#69347);
#20714=VERTEX_POINT('',#69349);
#20715=VERTEX_POINT('',#69351);
#20716=VERTEX_POINT('',#69353);
#20717=VERTEX_POINT('',#69355);
#20718=VERTEX_POINT('',#69357);
#20719=VERTEX_POINT('',#69359);
#20720=VERTEX_POINT('',#69361);
#20721=VERTEX_POINT('',#69363);
#20722=VERTEX_POINT('',#69367);
#20723=VERTEX_POINT('',#69369);
#20724=VERTEX_POINT('',#69371);
#20725=VERTEX_POINT('',#69373);
#20726=VERTEX_POINT('',#69375);
#20727=VERTEX_POINT('',#69377);
#20728=VERTEX_POINT('',#69379);
#20729=VERTEX_POINT('',#69381);
#20730=VERTEX_POINT('',#69383);
#20731=VERTEX_POINT('',#69385);
#20732=VERTEX_POINT('',#69387);
#20733=VERTEX_POINT('',#69389);
#20734=VERTEX_POINT('',#69391);
#20735=VERTEX_POINT('',#69393);
#20736=VERTEX_POINT('',#69397);
#20737=VERTEX_POINT('',#69399);
#20738=VERTEX_POINT('',#69401);
#20739=VERTEX_POINT('',#69405);
#20740=VERTEX_POINT('',#69409);
#20741=VERTEX_POINT('',#69411);
#20742=VERTEX_POINT('',#69413);
#20743=VERTEX_POINT('',#69415);
#20744=VERTEX_POINT('',#69417);
#20745=VERTEX_POINT('',#69419);
#20746=VERTEX_POINT('',#69421);
#20747=VERTEX_POINT('',#69423);
#20748=VERTEX_POINT('',#69425);
#20749=VERTEX_POINT('',#69427);
#20750=VERTEX_POINT('',#69429);
#20751=VERTEX_POINT('',#69431);
#20752=VERTEX_POINT('',#69433);
#20753=VERTEX_POINT('',#69435);
#20754=VERTEX_POINT('',#69437);
#20755=VERTEX_POINT('',#69439);
#20756=VERTEX_POINT('',#69443);
#20757=VERTEX_POINT('',#69445);
#20758=VERTEX_POINT('',#69447);
#20759=VERTEX_POINT('',#69449);
#20760=VERTEX_POINT('',#69451);
#20761=VERTEX_POINT('',#69453);
#20762=VERTEX_POINT('',#69455);
#20763=VERTEX_POINT('',#69457);
#20764=VERTEX_POINT('',#69459);
#20765=VERTEX_POINT('',#69461);
#20766=VERTEX_POINT('',#69463);
#20767=VERTEX_POINT('',#69465);
#20768=VERTEX_POINT('',#69467);
#20769=VERTEX_POINT('',#69469);
#20770=VERTEX_POINT('',#69473);
#20771=VERTEX_POINT('',#69475);
#20772=VERTEX_POINT('',#69477);
#20773=VERTEX_POINT('',#69481);
#20774=VERTEX_POINT('',#69485);
#20775=VERTEX_POINT('',#69487);
#20776=VERTEX_POINT('',#69489);
#20777=VERTEX_POINT('',#69491);
#20778=VERTEX_POINT('',#69493);
#20779=VERTEX_POINT('',#69495);
#20780=VERTEX_POINT('',#69497);
#20781=VERTEX_POINT('',#69499);
#20782=VERTEX_POINT('',#69501);
#20783=VERTEX_POINT('',#69503);
#20784=VERTEX_POINT('',#69505);
#20785=VERTEX_POINT('',#69507);
#20786=VERTEX_POINT('',#69509);
#20787=VERTEX_POINT('',#69511);
#20788=VERTEX_POINT('',#69513);
#20789=VERTEX_POINT('',#69515);
#20790=VERTEX_POINT('',#69519);
#20791=VERTEX_POINT('',#69521);
#20792=VERTEX_POINT('',#69523);
#20793=VERTEX_POINT('',#69525);
#20794=VERTEX_POINT('',#69527);
#20795=VERTEX_POINT('',#69529);
#20796=VERTEX_POINT('',#69531);
#20797=VERTEX_POINT('',#69533);
#20798=VERTEX_POINT('',#69535);
#20799=VERTEX_POINT('',#69537);
#20800=VERTEX_POINT('',#69539);
#20801=VERTEX_POINT('',#69541);
#20802=VERTEX_POINT('',#69543);
#20803=VERTEX_POINT('',#69545);
#20804=VERTEX_POINT('',#69549);
#20805=VERTEX_POINT('',#69551);
#20806=VERTEX_POINT('',#69553);
#20807=VERTEX_POINT('',#69557);
#20808=VERTEX_POINT('',#69561);
#20809=VERTEX_POINT('',#69563);
#20810=VERTEX_POINT('',#69565);
#20811=VERTEX_POINT('',#69567);
#20812=VERTEX_POINT('',#69569);
#20813=VERTEX_POINT('',#69571);
#20814=VERTEX_POINT('',#69573);
#20815=VERTEX_POINT('',#69575);
#20816=VERTEX_POINT('',#69577);
#20817=VERTEX_POINT('',#69579);
#20818=VERTEX_POINT('',#69581);
#20819=VERTEX_POINT('',#69583);
#20820=VERTEX_POINT('',#69585);
#20821=VERTEX_POINT('',#69587);
#20822=VERTEX_POINT('',#69589);
#20823=VERTEX_POINT('',#69591);
#20824=VERTEX_POINT('',#69595);
#20825=VERTEX_POINT('',#69597);
#20826=VERTEX_POINT('',#69599);
#20827=VERTEX_POINT('',#69601);
#20828=VERTEX_POINT('',#69603);
#20829=VERTEX_POINT('',#69605);
#20830=VERTEX_POINT('',#69607);
#20831=VERTEX_POINT('',#69609);
#20832=VERTEX_POINT('',#69611);
#20833=VERTEX_POINT('',#69613);
#20834=VERTEX_POINT('',#69615);
#20835=VERTEX_POINT('',#69617);
#20836=VERTEX_POINT('',#69619);
#20837=VERTEX_POINT('',#69621);
#20838=VERTEX_POINT('',#69625);
#20839=VERTEX_POINT('',#69627);
#20840=VERTEX_POINT('',#69629);
#20841=VERTEX_POINT('',#69633);
#20842=VERTEX_POINT('',#69637);
#20843=VERTEX_POINT('',#69639);
#20844=VERTEX_POINT('',#69641);
#20845=VERTEX_POINT('',#69643);
#20846=VERTEX_POINT('',#69645);
#20847=VERTEX_POINT('',#69647);
#20848=VERTEX_POINT('',#69649);
#20849=VERTEX_POINT('',#69651);
#20850=VERTEX_POINT('',#69653);
#20851=VERTEX_POINT('',#69655);
#20852=VERTEX_POINT('',#69657);
#20853=VERTEX_POINT('',#69659);
#20854=VERTEX_POINT('',#69661);
#20855=VERTEX_POINT('',#69663);
#20856=VERTEX_POINT('',#69665);
#20857=VERTEX_POINT('',#69667);
#20858=VERTEX_POINT('',#69671);
#20859=VERTEX_POINT('',#69673);
#20860=VERTEX_POINT('',#69675);
#20861=VERTEX_POINT('',#69677);
#20862=VERTEX_POINT('',#69679);
#20863=VERTEX_POINT('',#69681);
#20864=VERTEX_POINT('',#69683);
#20865=VERTEX_POINT('',#69685);
#20866=VERTEX_POINT('',#69687);
#20867=VERTEX_POINT('',#69689);
#20868=VERTEX_POINT('',#69691);
#20869=VERTEX_POINT('',#69693);
#20870=VERTEX_POINT('',#69695);
#20871=VERTEX_POINT('',#69697);
#20872=VERTEX_POINT('',#69701);
#20873=VERTEX_POINT('',#69703);
#20874=VERTEX_POINT('',#69705);
#20875=VERTEX_POINT('',#69709);
#20876=VERTEX_POINT('',#69713);
#20877=VERTEX_POINT('',#69715);
#20878=VERTEX_POINT('',#69717);
#20879=VERTEX_POINT('',#69719);
#20880=VERTEX_POINT('',#69721);
#20881=VERTEX_POINT('',#69723);
#20882=VERTEX_POINT('',#69725);
#20883=VERTEX_POINT('',#69727);
#20884=VERTEX_POINT('',#69729);
#20885=VERTEX_POINT('',#69731);
#20886=VERTEX_POINT('',#69733);
#20887=VERTEX_POINT('',#69735);
#20888=VERTEX_POINT('',#69737);
#20889=VERTEX_POINT('',#69739);
#20890=VERTEX_POINT('',#69741);
#20891=VERTEX_POINT('',#69743);
#20892=VERTEX_POINT('',#69747);
#20893=VERTEX_POINT('',#69749);
#20894=VERTEX_POINT('',#69751);
#20895=VERTEX_POINT('',#69753);
#20896=VERTEX_POINT('',#69755);
#20897=VERTEX_POINT('',#69757);
#20898=VERTEX_POINT('',#69759);
#20899=VERTEX_POINT('',#69761);
#20900=VERTEX_POINT('',#69763);
#20901=VERTEX_POINT('',#69765);
#20902=VERTEX_POINT('',#69767);
#20903=VERTEX_POINT('',#69769);
#20904=VERTEX_POINT('',#69771);
#20905=VERTEX_POINT('',#69773);
#20906=VERTEX_POINT('',#69777);
#20907=VERTEX_POINT('',#69779);
#20908=VERTEX_POINT('',#69781);
#20909=VERTEX_POINT('',#69785);
#20910=VERTEX_POINT('',#69789);
#20911=VERTEX_POINT('',#69791);
#20912=VERTEX_POINT('',#69793);
#20913=VERTEX_POINT('',#69795);
#20914=VERTEX_POINT('',#69797);
#20915=VERTEX_POINT('',#69799);
#20916=VERTEX_POINT('',#69801);
#20917=VERTEX_POINT('',#69803);
#20918=VERTEX_POINT('',#69805);
#20919=VERTEX_POINT('',#69807);
#20920=VERTEX_POINT('',#69809);
#20921=VERTEX_POINT('',#69811);
#20922=VERTEX_POINT('',#69813);
#20923=VERTEX_POINT('',#69815);
#20924=VERTEX_POINT('',#69817);
#20925=VERTEX_POINT('',#69819);
#20926=VERTEX_POINT('',#69823);
#20927=VERTEX_POINT('',#69825);
#20928=VERTEX_POINT('',#69827);
#20929=VERTEX_POINT('',#69829);
#20930=VERTEX_POINT('',#69831);
#20931=VERTEX_POINT('',#69833);
#20932=VERTEX_POINT('',#69835);
#20933=VERTEX_POINT('',#69837);
#20934=VERTEX_POINT('',#69839);
#20935=VERTEX_POINT('',#69841);
#20936=VERTEX_POINT('',#69843);
#20937=VERTEX_POINT('',#69845);
#20938=VERTEX_POINT('',#69847);
#20939=VERTEX_POINT('',#69849);
#20940=VERTEX_POINT('',#69853);
#20941=VERTEX_POINT('',#69855);
#20942=VERTEX_POINT('',#69857);
#20943=VERTEX_POINT('',#69861);
#20944=VERTEX_POINT('',#69865);
#20945=VERTEX_POINT('',#69867);
#20946=VERTEX_POINT('',#69869);
#20947=VERTEX_POINT('',#69871);
#20948=VERTEX_POINT('',#69873);
#20949=VERTEX_POINT('',#69875);
#20950=VERTEX_POINT('',#69877);
#20951=VERTEX_POINT('',#69879);
#20952=VERTEX_POINT('',#69881);
#20953=VERTEX_POINT('',#69883);
#20954=VERTEX_POINT('',#69885);
#20955=VERTEX_POINT('',#69887);
#20956=VERTEX_POINT('',#69889);
#20957=VERTEX_POINT('',#69891);
#20958=VERTEX_POINT('',#69893);
#20959=VERTEX_POINT('',#69895);
#20960=VERTEX_POINT('',#69899);
#20961=VERTEX_POINT('',#69901);
#20962=VERTEX_POINT('',#69903);
#20963=VERTEX_POINT('',#69905);
#20964=VERTEX_POINT('',#69907);
#20965=VERTEX_POINT('',#69909);
#20966=VERTEX_POINT('',#69911);
#20967=VERTEX_POINT('',#69913);
#20968=VERTEX_POINT('',#69915);
#20969=VERTEX_POINT('',#69917);
#20970=VERTEX_POINT('',#69919);
#20971=VERTEX_POINT('',#69921);
#20972=VERTEX_POINT('',#69923);
#20973=VERTEX_POINT('',#69925);
#20974=VERTEX_POINT('',#69929);
#20975=VERTEX_POINT('',#69931);
#20976=VERTEX_POINT('',#69933);
#20977=VERTEX_POINT('',#69937);
#20978=VERTEX_POINT('',#69941);
#20979=VERTEX_POINT('',#69943);
#20980=VERTEX_POINT('',#69945);
#20981=VERTEX_POINT('',#69947);
#20982=VERTEX_POINT('',#69949);
#20983=VERTEX_POINT('',#69951);
#20984=VERTEX_POINT('',#69953);
#20985=VERTEX_POINT('',#69955);
#20986=VERTEX_POINT('',#69957);
#20987=VERTEX_POINT('',#69959);
#20988=VERTEX_POINT('',#69961);
#20989=VERTEX_POINT('',#69963);
#20990=VERTEX_POINT('',#69965);
#20991=VERTEX_POINT('',#69967);
#20992=VERTEX_POINT('',#69969);
#20993=VERTEX_POINT('',#69971);
#20994=VERTEX_POINT('',#69975);
#20995=VERTEX_POINT('',#69977);
#20996=VERTEX_POINT('',#69979);
#20997=VERTEX_POINT('',#69981);
#20998=VERTEX_POINT('',#69983);
#20999=VERTEX_POINT('',#69985);
#21000=VERTEX_POINT('',#69987);
#21001=VERTEX_POINT('',#69989);
#21002=VERTEX_POINT('',#69991);
#21003=VERTEX_POINT('',#69993);
#21004=VERTEX_POINT('',#69995);
#21005=VERTEX_POINT('',#69997);
#21006=VERTEX_POINT('',#69999);
#21007=VERTEX_POINT('',#70001);
#21008=VERTEX_POINT('',#70005);
#21009=VERTEX_POINT('',#70007);
#21010=VERTEX_POINT('',#70009);
#21011=VERTEX_POINT('',#70013);
#21012=VERTEX_POINT('',#70017);
#21013=VERTEX_POINT('',#70019);
#21014=VERTEX_POINT('',#70021);
#21015=VERTEX_POINT('',#70023);
#21016=VERTEX_POINT('',#70025);
#21017=VERTEX_POINT('',#70027);
#21018=VERTEX_POINT('',#70029);
#21019=VERTEX_POINT('',#70031);
#21020=VERTEX_POINT('',#70033);
#21021=VERTEX_POINT('',#70035);
#21022=VERTEX_POINT('',#70037);
#21023=VERTEX_POINT('',#70039);
#21024=VERTEX_POINT('',#70041);
#21025=VERTEX_POINT('',#70043);
#21026=VERTEX_POINT('',#70045);
#21027=VERTEX_POINT('',#70047);
#21028=VERTEX_POINT('',#70051);
#21029=VERTEX_POINT('',#70053);
#21030=VERTEX_POINT('',#70055);
#21031=VERTEX_POINT('',#70057);
#21032=VERTEX_POINT('',#70059);
#21033=VERTEX_POINT('',#70061);
#21034=VERTEX_POINT('',#70063);
#21035=VERTEX_POINT('',#70065);
#21036=VERTEX_POINT('',#70067);
#21037=VERTEX_POINT('',#70069);
#21038=VERTEX_POINT('',#70071);
#21039=VERTEX_POINT('',#70073);
#21040=VERTEX_POINT('',#70075);
#21041=VERTEX_POINT('',#70077);
#21042=VERTEX_POINT('',#70081);
#21043=VERTEX_POINT('',#70083);
#21044=VERTEX_POINT('',#70085);
#21045=VERTEX_POINT('',#70089);
#21046=VERTEX_POINT('',#70093);
#21047=VERTEX_POINT('',#70095);
#21048=VERTEX_POINT('',#70097);
#21049=VERTEX_POINT('',#70099);
#21050=VERTEX_POINT('',#70101);
#21051=VERTEX_POINT('',#70103);
#21052=VERTEX_POINT('',#70105);
#21053=VERTEX_POINT('',#70107);
#21054=VERTEX_POINT('',#70109);
#21055=VERTEX_POINT('',#70111);
#21056=VERTEX_POINT('',#70113);
#21057=VERTEX_POINT('',#70115);
#21058=VERTEX_POINT('',#70117);
#21059=VERTEX_POINT('',#70119);
#21060=VERTEX_POINT('',#70121);
#21061=VERTEX_POINT('',#70123);
#21062=VERTEX_POINT('',#70127);
#21063=VERTEX_POINT('',#70129);
#21064=VERTEX_POINT('',#70131);
#21065=VERTEX_POINT('',#70133);
#21066=VERTEX_POINT('',#70135);
#21067=VERTEX_POINT('',#70137);
#21068=VERTEX_POINT('',#70139);
#21069=VERTEX_POINT('',#70141);
#21070=VERTEX_POINT('',#70143);
#21071=VERTEX_POINT('',#70145);
#21072=VERTEX_POINT('',#70147);
#21073=VERTEX_POINT('',#70149);
#21074=VERTEX_POINT('',#70151);
#21075=VERTEX_POINT('',#70153);
#21076=VERTEX_POINT('',#70157);
#21077=VERTEX_POINT('',#70159);
#21078=VERTEX_POINT('',#70161);
#21079=VERTEX_POINT('',#70165);
#21080=VERTEX_POINT('',#70169);
#21081=VERTEX_POINT('',#70171);
#21082=VERTEX_POINT('',#70173);
#21083=VERTEX_POINT('',#70175);
#21084=VERTEX_POINT('',#70177);
#21085=VERTEX_POINT('',#70179);
#21086=VERTEX_POINT('',#70181);
#21087=VERTEX_POINT('',#70183);
#21088=VERTEX_POINT('',#70185);
#21089=VERTEX_POINT('',#70187);
#21090=VERTEX_POINT('',#70189);
#21091=VERTEX_POINT('',#70191);
#21092=VERTEX_POINT('',#70193);
#21093=VERTEX_POINT('',#70195);
#21094=VERTEX_POINT('',#70197);
#21095=VERTEX_POINT('',#70199);
#21096=VERTEX_POINT('',#70203);
#21097=VERTEX_POINT('',#70205);
#21098=VERTEX_POINT('',#70207);
#21099=VERTEX_POINT('',#70209);
#21100=VERTEX_POINT('',#70211);
#21101=VERTEX_POINT('',#70213);
#21102=VERTEX_POINT('',#70215);
#21103=VERTEX_POINT('',#70217);
#21104=VERTEX_POINT('',#70219);
#21105=VERTEX_POINT('',#70221);
#21106=VERTEX_POINT('',#70223);
#21107=VERTEX_POINT('',#70225);
#21108=VERTEX_POINT('',#70227);
#21109=VERTEX_POINT('',#70229);
#21110=VERTEX_POINT('',#70233);
#21111=VERTEX_POINT('',#70235);
#21112=VERTEX_POINT('',#70237);
#21113=VERTEX_POINT('',#70241);
#21114=VERTEX_POINT('',#70245);
#21115=VERTEX_POINT('',#70247);
#21116=VERTEX_POINT('',#70249);
#21117=VERTEX_POINT('',#70251);
#21118=VERTEX_POINT('',#70253);
#21119=VERTEX_POINT('',#70255);
#21120=VERTEX_POINT('',#70257);
#21121=VERTEX_POINT('',#70259);
#21122=VERTEX_POINT('',#70261);
#21123=VERTEX_POINT('',#70263);
#21124=VERTEX_POINT('',#70265);
#21125=VERTEX_POINT('',#70267);
#21126=VERTEX_POINT('',#70269);
#21127=VERTEX_POINT('',#70271);
#21128=VERTEX_POINT('',#70273);
#21129=VERTEX_POINT('',#70275);
#21130=VERTEX_POINT('',#70279);
#21131=VERTEX_POINT('',#70281);
#21132=VERTEX_POINT('',#70283);
#21133=VERTEX_POINT('',#70285);
#21134=VERTEX_POINT('',#70287);
#21135=VERTEX_POINT('',#70289);
#21136=VERTEX_POINT('',#70291);
#21137=VERTEX_POINT('',#70293);
#21138=VERTEX_POINT('',#70295);
#21139=VERTEX_POINT('',#70297);
#21140=VERTEX_POINT('',#70299);
#21141=VERTEX_POINT('',#70301);
#21142=VERTEX_POINT('',#70303);
#21143=VERTEX_POINT('',#70305);
#21144=VERTEX_POINT('',#70309);
#21145=VERTEX_POINT('',#70311);
#21146=VERTEX_POINT('',#70313);
#21147=VERTEX_POINT('',#70317);
#21148=VERTEX_POINT('',#70321);
#21149=VERTEX_POINT('',#70323);
#21150=VERTEX_POINT('',#70325);
#21151=VERTEX_POINT('',#70327);
#21152=VERTEX_POINT('',#70329);
#21153=VERTEX_POINT('',#70331);
#21154=VERTEX_POINT('',#70333);
#21155=VERTEX_POINT('',#70335);
#21156=VERTEX_POINT('',#70337);
#21157=VERTEX_POINT('',#70339);
#21158=VERTEX_POINT('',#70341);
#21159=VERTEX_POINT('',#70343);
#21160=VERTEX_POINT('',#70345);
#21161=VERTEX_POINT('',#70347);
#21162=VERTEX_POINT('',#70349);
#21163=VERTEX_POINT('',#70351);
#21164=VERTEX_POINT('',#70355);
#21165=VERTEX_POINT('',#70357);
#21166=VERTEX_POINT('',#70359);
#21167=VERTEX_POINT('',#70361);
#21168=VERTEX_POINT('',#70363);
#21169=VERTEX_POINT('',#70365);
#21170=VERTEX_POINT('',#70367);
#21171=VERTEX_POINT('',#70369);
#21172=VERTEX_POINT('',#70371);
#21173=VERTEX_POINT('',#70373);
#21174=VERTEX_POINT('',#70375);
#21175=VERTEX_POINT('',#70377);
#21176=VERTEX_POINT('',#70379);
#21177=VERTEX_POINT('',#70381);
#21178=VERTEX_POINT('',#70385);
#21179=VERTEX_POINT('',#70387);
#21180=VERTEX_POINT('',#70389);
#21181=VERTEX_POINT('',#70393);
#21182=VERTEX_POINT('',#70397);
#21183=VERTEX_POINT('',#70399);
#21184=VERTEX_POINT('',#70401);
#21185=VERTEX_POINT('',#70403);
#21186=VERTEX_POINT('',#70405);
#21187=VERTEX_POINT('',#70407);
#21188=VERTEX_POINT('',#70409);
#21189=VERTEX_POINT('',#70411);
#21190=VERTEX_POINT('',#70413);
#21191=VERTEX_POINT('',#70415);
#21192=VERTEX_POINT('',#70417);
#21193=VERTEX_POINT('',#70419);
#21194=VERTEX_POINT('',#70421);
#21195=VERTEX_POINT('',#70423);
#21196=VERTEX_POINT('',#70425);
#21197=VERTEX_POINT('',#70427);
#21198=VERTEX_POINT('',#70431);
#21199=VERTEX_POINT('',#70433);
#21200=VERTEX_POINT('',#70435);
#21201=VERTEX_POINT('',#70437);
#21202=VERTEX_POINT('',#70439);
#21203=VERTEX_POINT('',#70441);
#21204=VERTEX_POINT('',#70443);
#21205=VERTEX_POINT('',#70445);
#21206=VERTEX_POINT('',#70447);
#21207=VERTEX_POINT('',#70449);
#21208=VERTEX_POINT('',#70451);
#21209=VERTEX_POINT('',#70453);
#21210=VERTEX_POINT('',#70455);
#21211=VERTEX_POINT('',#70457);
#21212=VERTEX_POINT('',#70461);
#21213=VERTEX_POINT('',#70463);
#21214=VERTEX_POINT('',#70465);
#21215=VERTEX_POINT('',#70469);
#21216=VERTEX_POINT('',#70473);
#21217=VERTEX_POINT('',#70475);
#21218=VERTEX_POINT('',#70477);
#21219=VERTEX_POINT('',#70479);
#21220=VERTEX_POINT('',#70481);
#21221=VERTEX_POINT('',#70483);
#21222=VERTEX_POINT('',#70485);
#21223=VERTEX_POINT('',#70487);
#21224=VERTEX_POINT('',#70489);
#21225=VERTEX_POINT('',#70491);
#21226=VERTEX_POINT('',#70493);
#21227=VERTEX_POINT('',#70495);
#21228=VERTEX_POINT('',#70497);
#21229=VERTEX_POINT('',#70499);
#21230=VERTEX_POINT('',#70501);
#21231=VERTEX_POINT('',#70503);
#21232=VERTEX_POINT('',#70507);
#21233=VERTEX_POINT('',#70509);
#21234=VERTEX_POINT('',#70511);
#21235=VERTEX_POINT('',#70513);
#21236=VERTEX_POINT('',#70515);
#21237=VERTEX_POINT('',#70517);
#21238=VERTEX_POINT('',#70519);
#21239=VERTEX_POINT('',#70521);
#21240=VERTEX_POINT('',#70523);
#21241=VERTEX_POINT('',#70525);
#21242=VERTEX_POINT('',#70527);
#21243=VERTEX_POINT('',#70529);
#21244=VERTEX_POINT('',#70531);
#21245=VERTEX_POINT('',#70533);
#21246=VERTEX_POINT('',#70537);
#21247=VERTEX_POINT('',#70539);
#21248=VERTEX_POINT('',#70541);
#21249=VERTEX_POINT('',#70545);
#21250=VERTEX_POINT('',#70549);
#21251=VERTEX_POINT('',#70551);
#21252=VERTEX_POINT('',#70553);
#21253=VERTEX_POINT('',#70555);
#21254=VERTEX_POINT('',#70557);
#21255=VERTEX_POINT('',#70559);
#21256=VERTEX_POINT('',#70561);
#21257=VERTEX_POINT('',#70563);
#21258=VERTEX_POINT('',#70565);
#21259=VERTEX_POINT('',#70567);
#21260=VERTEX_POINT('',#70569);
#21261=VERTEX_POINT('',#70571);
#21262=VERTEX_POINT('',#70573);
#21263=VERTEX_POINT('',#70575);
#21264=VERTEX_POINT('',#70577);
#21265=VERTEX_POINT('',#70579);
#21266=VERTEX_POINT('',#70583);
#21267=VERTEX_POINT('',#70585);
#21268=VERTEX_POINT('',#70587);
#21269=VERTEX_POINT('',#70589);
#21270=VERTEX_POINT('',#70591);
#21271=VERTEX_POINT('',#70593);
#21272=VERTEX_POINT('',#70595);
#21273=VERTEX_POINT('',#70597);
#21274=VERTEX_POINT('',#70599);
#21275=VERTEX_POINT('',#70601);
#21276=VERTEX_POINT('',#70603);
#21277=VERTEX_POINT('',#70605);
#21278=VERTEX_POINT('',#70607);
#21279=VERTEX_POINT('',#70609);
#21280=VERTEX_POINT('',#70613);
#21281=VERTEX_POINT('',#70615);
#21282=VERTEX_POINT('',#70617);
#21283=VERTEX_POINT('',#70621);
#21284=VERTEX_POINT('',#70625);
#21285=VERTEX_POINT('',#70627);
#21286=VERTEX_POINT('',#70629);
#21287=VERTEX_POINT('',#70631);
#21288=VERTEX_POINT('',#70633);
#21289=VERTEX_POINT('',#70635);
#21290=VERTEX_POINT('',#70637);
#21291=VERTEX_POINT('',#70639);
#21292=VERTEX_POINT('',#70641);
#21293=VERTEX_POINT('',#70643);
#21294=VERTEX_POINT('',#70645);
#21295=VERTEX_POINT('',#70647);
#21296=VERTEX_POINT('',#70649);
#21297=VERTEX_POINT('',#70651);
#21298=VERTEX_POINT('',#70653);
#21299=VERTEX_POINT('',#70655);
#21300=VERTEX_POINT('',#70659);
#21301=VERTEX_POINT('',#70661);
#21302=VERTEX_POINT('',#70663);
#21303=VERTEX_POINT('',#70665);
#21304=VERTEX_POINT('',#70667);
#21305=VERTEX_POINT('',#70669);
#21306=VERTEX_POINT('',#70671);
#21307=VERTEX_POINT('',#70673);
#21308=VERTEX_POINT('',#70675);
#21309=VERTEX_POINT('',#70677);
#21310=VERTEX_POINT('',#70679);
#21311=VERTEX_POINT('',#70681);
#21312=VERTEX_POINT('',#70683);
#21313=VERTEX_POINT('',#70685);
#21314=VERTEX_POINT('',#70689);
#21315=VERTEX_POINT('',#70691);
#21316=VERTEX_POINT('',#70693);
#21317=VERTEX_POINT('',#70697);
#21318=VERTEX_POINT('',#70701);
#21319=VERTEX_POINT('',#70703);
#21320=VERTEX_POINT('',#70705);
#21321=VERTEX_POINT('',#70707);
#21322=VERTEX_POINT('',#70709);
#21323=VERTEX_POINT('',#70711);
#21324=VERTEX_POINT('',#70713);
#21325=VERTEX_POINT('',#70715);
#21326=VERTEX_POINT('',#70717);
#21327=VERTEX_POINT('',#70719);
#21328=VERTEX_POINT('',#70721);
#21329=VERTEX_POINT('',#70723);
#21330=VERTEX_POINT('',#70725);
#21331=VERTEX_POINT('',#70727);
#21332=VERTEX_POINT('',#70729);
#21333=VERTEX_POINT('',#70731);
#21334=VERTEX_POINT('',#70735);
#21335=VERTEX_POINT('',#70737);
#21336=VERTEX_POINT('',#70739);
#21337=VERTEX_POINT('',#70741);
#21338=VERTEX_POINT('',#70743);
#21339=VERTEX_POINT('',#70745);
#21340=VERTEX_POINT('',#70747);
#21341=VERTEX_POINT('',#70749);
#21342=VERTEX_POINT('',#70751);
#21343=VERTEX_POINT('',#70753);
#21344=VERTEX_POINT('',#70755);
#21345=VERTEX_POINT('',#70757);
#21346=VERTEX_POINT('',#70759);
#21347=VERTEX_POINT('',#70761);
#21348=VERTEX_POINT('',#70765);
#21349=VERTEX_POINT('',#70767);
#21350=VERTEX_POINT('',#70769);
#21351=VERTEX_POINT('',#70773);
#21352=VERTEX_POINT('',#70777);
#21353=VERTEX_POINT('',#70779);
#21354=VERTEX_POINT('',#70781);
#21355=VERTEX_POINT('',#70783);
#21356=VERTEX_POINT('',#70785);
#21357=VERTEX_POINT('',#70787);
#21358=VERTEX_POINT('',#70789);
#21359=VERTEX_POINT('',#70791);
#21360=VERTEX_POINT('',#70793);
#21361=VERTEX_POINT('',#70795);
#21362=VERTEX_POINT('',#70797);
#21363=VERTEX_POINT('',#70799);
#21364=VERTEX_POINT('',#70801);
#21365=VERTEX_POINT('',#70803);
#21366=VERTEX_POINT('',#70805);
#21367=VERTEX_POINT('',#70807);
#21368=VERTEX_POINT('',#70811);
#21369=VERTEX_POINT('',#70813);
#21370=VERTEX_POINT('',#70815);
#21371=VERTEX_POINT('',#70817);
#21372=VERTEX_POINT('',#70819);
#21373=VERTEX_POINT('',#70821);
#21374=VERTEX_POINT('',#70823);
#21375=VERTEX_POINT('',#70825);
#21376=VERTEX_POINT('',#70827);
#21377=VERTEX_POINT('',#70829);
#21378=VERTEX_POINT('',#70831);
#21379=VERTEX_POINT('',#70833);
#21380=VERTEX_POINT('',#70835);
#21381=VERTEX_POINT('',#70837);
#21382=VERTEX_POINT('',#70841);
#21383=VERTEX_POINT('',#70843);
#21384=VERTEX_POINT('',#70845);
#21385=VERTEX_POINT('',#70849);
#21386=VERTEX_POINT('',#70853);
#21387=VERTEX_POINT('',#70855);
#21388=VERTEX_POINT('',#70857);
#21389=VERTEX_POINT('',#70859);
#21390=VERTEX_POINT('',#70861);
#21391=VERTEX_POINT('',#70863);
#21392=VERTEX_POINT('',#70865);
#21393=VERTEX_POINT('',#70867);
#21394=VERTEX_POINT('',#70869);
#21395=VERTEX_POINT('',#70871);
#21396=VERTEX_POINT('',#70873);
#21397=VERTEX_POINT('',#70875);
#21398=VERTEX_POINT('',#70877);
#21399=VERTEX_POINT('',#70879);
#21400=VERTEX_POINT('',#70881);
#21401=VERTEX_POINT('',#70883);
#21402=VERTEX_POINT('',#70887);
#21403=VERTEX_POINT('',#70889);
#21404=VERTEX_POINT('',#70891);
#21405=VERTEX_POINT('',#70893);
#21406=VERTEX_POINT('',#70895);
#21407=VERTEX_POINT('',#70897);
#21408=VERTEX_POINT('',#70899);
#21409=VERTEX_POINT('',#70901);
#21410=VERTEX_POINT('',#70903);
#21411=VERTEX_POINT('',#70905);
#21412=VERTEX_POINT('',#70907);
#21413=VERTEX_POINT('',#70909);
#21414=VERTEX_POINT('',#70911);
#21415=VERTEX_POINT('',#70913);
#21416=VERTEX_POINT('',#70917);
#21417=VERTEX_POINT('',#70919);
#21418=VERTEX_POINT('',#70921);
#21419=VERTEX_POINT('',#70925);
#21420=VERTEX_POINT('',#70929);
#21421=VERTEX_POINT('',#70931);
#21422=VERTEX_POINT('',#70933);
#21423=VERTEX_POINT('',#70935);
#21424=VERTEX_POINT('',#70937);
#21425=VERTEX_POINT('',#70939);
#21426=VERTEX_POINT('',#70941);
#21427=VERTEX_POINT('',#70943);
#21428=VERTEX_POINT('',#70945);
#21429=VERTEX_POINT('',#70947);
#21430=VERTEX_POINT('',#70949);
#21431=VERTEX_POINT('',#70951);
#21432=VERTEX_POINT('',#70953);
#21433=VERTEX_POINT('',#70955);
#21434=VERTEX_POINT('',#70957);
#21435=VERTEX_POINT('',#70959);
#21436=VERTEX_POINT('',#70963);
#21437=VERTEX_POINT('',#70965);
#21438=VERTEX_POINT('',#70967);
#21439=VERTEX_POINT('',#70969);
#21440=VERTEX_POINT('',#70971);
#21441=VERTEX_POINT('',#70973);
#21442=VERTEX_POINT('',#70975);
#21443=VERTEX_POINT('',#70977);
#21444=VERTEX_POINT('',#70979);
#21445=VERTEX_POINT('',#70981);
#21446=VERTEX_POINT('',#70983);
#21447=VERTEX_POINT('',#70985);
#21448=VERTEX_POINT('',#70987);
#21449=VERTEX_POINT('',#70989);
#21450=VERTEX_POINT('',#70993);
#21451=VERTEX_POINT('',#70995);
#21452=VERTEX_POINT('',#70997);
#21453=VERTEX_POINT('',#71001);
#21454=VERTEX_POINT('',#71005);
#21455=VERTEX_POINT('',#71007);
#21456=VERTEX_POINT('',#71009);
#21457=VERTEX_POINT('',#71011);
#21458=VERTEX_POINT('',#71013);
#21459=VERTEX_POINT('',#71015);
#21460=VERTEX_POINT('',#71017);
#21461=VERTEX_POINT('',#71019);
#21462=VERTEX_POINT('',#71021);
#21463=VERTEX_POINT('',#71023);
#21464=VERTEX_POINT('',#71025);
#21465=VERTEX_POINT('',#71027);
#21466=VERTEX_POINT('',#71029);
#21467=VERTEX_POINT('',#71031);
#21468=VERTEX_POINT('',#71033);
#21469=VERTEX_POINT('',#71035);
#21470=VERTEX_POINT('',#71039);
#21471=VERTEX_POINT('',#71041);
#21472=VERTEX_POINT('',#71043);
#21473=VERTEX_POINT('',#71045);
#21474=VERTEX_POINT('',#71047);
#21475=VERTEX_POINT('',#71049);
#21476=VERTEX_POINT('',#71051);
#21477=VERTEX_POINT('',#71053);
#21478=VERTEX_POINT('',#71055);
#21479=VERTEX_POINT('',#71057);
#21480=VERTEX_POINT('',#71059);
#21481=VERTEX_POINT('',#71061);
#21482=VERTEX_POINT('',#71063);
#21483=VERTEX_POINT('',#71065);
#21484=VERTEX_POINT('',#71069);
#21485=VERTEX_POINT('',#71071);
#21486=VERTEX_POINT('',#71073);
#21487=VERTEX_POINT('',#71077);
#21488=VERTEX_POINT('',#71081);
#21489=VERTEX_POINT('',#71083);
#21490=VERTEX_POINT('',#71085);
#21491=VERTEX_POINT('',#71087);
#21492=VERTEX_POINT('',#71089);
#21493=VERTEX_POINT('',#71091);
#21494=VERTEX_POINT('',#71093);
#21495=VERTEX_POINT('',#71095);
#21496=VERTEX_POINT('',#71097);
#21497=VERTEX_POINT('',#71099);
#21498=VERTEX_POINT('',#71101);
#21499=VERTEX_POINT('',#71103);
#21500=VERTEX_POINT('',#71105);
#21501=VERTEX_POINT('',#71107);
#21502=VERTEX_POINT('',#71109);
#21503=VERTEX_POINT('',#71111);
#21504=VERTEX_POINT('',#71115);
#21505=VERTEX_POINT('',#71117);
#21506=VERTEX_POINT('',#71119);
#21507=VERTEX_POINT('',#71121);
#21508=VERTEX_POINT('',#71123);
#21509=VERTEX_POINT('',#71125);
#21510=VERTEX_POINT('',#71127);
#21511=VERTEX_POINT('',#71129);
#21512=VERTEX_POINT('',#71131);
#21513=VERTEX_POINT('',#71133);
#21514=VERTEX_POINT('',#71135);
#21515=VERTEX_POINT('',#71137);
#21516=VERTEX_POINT('',#71139);
#21517=VERTEX_POINT('',#71141);
#21518=VERTEX_POINT('',#71145);
#21519=VERTEX_POINT('',#71147);
#21520=VERTEX_POINT('',#71149);
#21521=VERTEX_POINT('',#71153);
#21522=VERTEX_POINT('',#71157);
#21523=VERTEX_POINT('',#71159);
#21524=VERTEX_POINT('',#71161);
#21525=VERTEX_POINT('',#71163);
#21526=VERTEX_POINT('',#71165);
#21527=VERTEX_POINT('',#71167);
#21528=VERTEX_POINT('',#71169);
#21529=VERTEX_POINT('',#71171);
#21530=VERTEX_POINT('',#71173);
#21531=VERTEX_POINT('',#71175);
#21532=VERTEX_POINT('',#71177);
#21533=VERTEX_POINT('',#71179);
#21534=VERTEX_POINT('',#71181);
#21535=VERTEX_POINT('',#71183);
#21536=VERTEX_POINT('',#71185);
#21537=VERTEX_POINT('',#71187);
#21538=VERTEX_POINT('',#71191);
#21539=VERTEX_POINT('',#71193);
#21540=VERTEX_POINT('',#71195);
#21541=VERTEX_POINT('',#71197);
#21542=VERTEX_POINT('',#71199);
#21543=VERTEX_POINT('',#71201);
#21544=VERTEX_POINT('',#71203);
#21545=VERTEX_POINT('',#71205);
#21546=VERTEX_POINT('',#71207);
#21547=VERTEX_POINT('',#71209);
#21548=VERTEX_POINT('',#71211);
#21549=VERTEX_POINT('',#71213);
#21550=VERTEX_POINT('',#71215);
#21551=VERTEX_POINT('',#71217);
#21552=VERTEX_POINT('',#71221);
#21553=VERTEX_POINT('',#71223);
#21554=VERTEX_POINT('',#71225);
#21555=VERTEX_POINT('',#71229);
#21556=VERTEX_POINT('',#71233);
#21557=VERTEX_POINT('',#71235);
#21558=VERTEX_POINT('',#71237);
#21559=VERTEX_POINT('',#71239);
#21560=VERTEX_POINT('',#71241);
#21561=VERTEX_POINT('',#71243);
#21562=VERTEX_POINT('',#71245);
#21563=VERTEX_POINT('',#71247);
#21564=VERTEX_POINT('',#71249);
#21565=VERTEX_POINT('',#71251);
#21566=VERTEX_POINT('',#71253);
#21567=VERTEX_POINT('',#71255);
#21568=VERTEX_POINT('',#71257);
#21569=VERTEX_POINT('',#71259);
#21570=VERTEX_POINT('',#71261);
#21571=VERTEX_POINT('',#71263);
#21572=VERTEX_POINT('',#71267);
#21573=VERTEX_POINT('',#71269);
#21574=VERTEX_POINT('',#71271);
#21575=VERTEX_POINT('',#71273);
#21576=VERTEX_POINT('',#71275);
#21577=VERTEX_POINT('',#71277);
#21578=VERTEX_POINT('',#71279);
#21579=VERTEX_POINT('',#71281);
#21580=VERTEX_POINT('',#71283);
#21581=VERTEX_POINT('',#71285);
#21582=VERTEX_POINT('',#71287);
#21583=VERTEX_POINT('',#71289);
#21584=VERTEX_POINT('',#71291);
#21585=VERTEX_POINT('',#71293);
#21586=VERTEX_POINT('',#71297);
#21587=VERTEX_POINT('',#71299);
#21588=VERTEX_POINT('',#71301);
#21589=VERTEX_POINT('',#71305);
#21590=VERTEX_POINT('',#71309);
#21591=VERTEX_POINT('',#71311);
#21592=VERTEX_POINT('',#71313);
#21593=VERTEX_POINT('',#71315);
#21594=VERTEX_POINT('',#71317);
#21595=VERTEX_POINT('',#71319);
#21596=VERTEX_POINT('',#71321);
#21597=VERTEX_POINT('',#71323);
#21598=VERTEX_POINT('',#71325);
#21599=VERTEX_POINT('',#71327);
#21600=VERTEX_POINT('',#71329);
#21601=VERTEX_POINT('',#71331);
#21602=VERTEX_POINT('',#71333);
#21603=VERTEX_POINT('',#71335);
#21604=VERTEX_POINT('',#71337);
#21605=VERTEX_POINT('',#71339);
#21606=VERTEX_POINT('',#71343);
#21607=VERTEX_POINT('',#71345);
#21608=VERTEX_POINT('',#71347);
#21609=VERTEX_POINT('',#71349);
#21610=VERTEX_POINT('',#71351);
#21611=VERTEX_POINT('',#71353);
#21612=VERTEX_POINT('',#71355);
#21613=VERTEX_POINT('',#71357);
#21614=VERTEX_POINT('',#71359);
#21615=VERTEX_POINT('',#71361);
#21616=VERTEX_POINT('',#71363);
#21617=VERTEX_POINT('',#71365);
#21618=VERTEX_POINT('',#71367);
#21619=VERTEX_POINT('',#71369);
#21620=VERTEX_POINT('',#71373);
#21621=VERTEX_POINT('',#71375);
#21622=VERTEX_POINT('',#71377);
#21623=VERTEX_POINT('',#71381);
#21624=VERTEX_POINT('',#71385);
#21625=VERTEX_POINT('',#71387);
#21626=VERTEX_POINT('',#71389);
#21627=VERTEX_POINT('',#71391);
#21628=VERTEX_POINT('',#71393);
#21629=VERTEX_POINT('',#71395);
#21630=VERTEX_POINT('',#71397);
#21631=VERTEX_POINT('',#71399);
#21632=VERTEX_POINT('',#71401);
#21633=VERTEX_POINT('',#71403);
#21634=VERTEX_POINT('',#71405);
#21635=VERTEX_POINT('',#71407);
#21636=VERTEX_POINT('',#71409);
#21637=VERTEX_POINT('',#71411);
#21638=VERTEX_POINT('',#71413);
#21639=VERTEX_POINT('',#71415);
#21640=VERTEX_POINT('',#71419);
#21641=VERTEX_POINT('',#71421);
#21642=VERTEX_POINT('',#71423);
#21643=VERTEX_POINT('',#71425);
#21644=VERTEX_POINT('',#71427);
#21645=VERTEX_POINT('',#71429);
#21646=VERTEX_POINT('',#71431);
#21647=VERTEX_POINT('',#71433);
#21648=VERTEX_POINT('',#71435);
#21649=VERTEX_POINT('',#71437);
#21650=VERTEX_POINT('',#71439);
#21651=VERTEX_POINT('',#71441);
#21652=VERTEX_POINT('',#71443);
#21653=VERTEX_POINT('',#71445);
#21654=VERTEX_POINT('',#71449);
#21655=VERTEX_POINT('',#71451);
#21656=VERTEX_POINT('',#71453);
#21657=VERTEX_POINT('',#71457);
#21658=VERTEX_POINT('',#71461);
#21659=VERTEX_POINT('',#71463);
#21660=VERTEX_POINT('',#71465);
#21661=VERTEX_POINT('',#71467);
#21662=VERTEX_POINT('',#71469);
#21663=VERTEX_POINT('',#71471);
#21664=VERTEX_POINT('',#71473);
#21665=VERTEX_POINT('',#71475);
#21666=VERTEX_POINT('',#71477);
#21667=VERTEX_POINT('',#71479);
#21668=VERTEX_POINT('',#71481);
#21669=VERTEX_POINT('',#71483);
#21670=VERTEX_POINT('',#71485);
#21671=VERTEX_POINT('',#71487);
#21672=VERTEX_POINT('',#71489);
#21673=VERTEX_POINT('',#71491);
#21674=VERTEX_POINT('',#71495);
#21675=VERTEX_POINT('',#71497);
#21676=VERTEX_POINT('',#71499);
#21677=VERTEX_POINT('',#71501);
#21678=VERTEX_POINT('',#71503);
#21679=VERTEX_POINT('',#71505);
#21680=VERTEX_POINT('',#71507);
#21681=VERTEX_POINT('',#71509);
#21682=VERTEX_POINT('',#71511);
#21683=VERTEX_POINT('',#71513);
#21684=VERTEX_POINT('',#71515);
#21685=VERTEX_POINT('',#71517);
#21686=VERTEX_POINT('',#71519);
#21687=VERTEX_POINT('',#71521);
#21688=VERTEX_POINT('',#71525);
#21689=VERTEX_POINT('',#71527);
#21690=VERTEX_POINT('',#71529);
#21691=VERTEX_POINT('',#71533);
#21692=VERTEX_POINT('',#71537);
#21693=VERTEX_POINT('',#71538);
#21694=VERTEX_POINT('',#71547);
#21695=VERTEX_POINT('',#71548);
#21696=VERTEX_POINT('',#71557);
#21697=VERTEX_POINT('',#71558);
#21698=VERTEX_POINT('',#71567);
#21699=VERTEX_POINT('',#71568);
#21700=VERTEX_POINT('',#71577);
#21701=VERTEX_POINT('',#71578);
#21702=VERTEX_POINT('',#71587);
#21703=VERTEX_POINT('',#71588);
#21704=VERTEX_POINT('',#71597);
#21705=VERTEX_POINT('',#71598);
#21706=VERTEX_POINT('',#71607);
#21707=VERTEX_POINT('',#71608);
#21708=VERTEX_POINT('',#71617);
#21709=VERTEX_POINT('',#71618);
#21710=VERTEX_POINT('',#71627);
#21711=VERTEX_POINT('',#71628);
#21712=VERTEX_POINT('',#71637);
#21713=VERTEX_POINT('',#71638);
#21714=VERTEX_POINT('',#71647);
#21715=VERTEX_POINT('',#71648);
#21716=VERTEX_POINT('',#71657);
#21717=VERTEX_POINT('',#71658);
#21718=VERTEX_POINT('',#71667);
#21719=VERTEX_POINT('',#71668);
#21720=VERTEX_POINT('',#71677);
#21721=VERTEX_POINT('',#71678);
#21722=VERTEX_POINT('',#71687);
#21723=VERTEX_POINT('',#71688);
#21724=VERTEX_POINT('',#71697);
#21725=VERTEX_POINT('',#71698);
#21726=VERTEX_POINT('',#71707);
#21727=VERTEX_POINT('',#71708);
#21728=VERTEX_POINT('',#71717);
#21729=VERTEX_POINT('',#71718);
#21730=VERTEX_POINT('',#71727);
#21731=VERTEX_POINT('',#71728);
#21732=VERTEX_POINT('',#71737);
#21733=VERTEX_POINT('',#71738);
#21734=VERTEX_POINT('',#71747);
#21735=VERTEX_POINT('',#71748);
#21736=VERTEX_POINT('',#71757);
#21737=VERTEX_POINT('',#71758);
#21738=VERTEX_POINT('',#71767);
#21739=VERTEX_POINT('',#71768);
#21740=VERTEX_POINT('',#71777);
#21741=VERTEX_POINT('',#71778);
#21742=VERTEX_POINT('',#71787);
#21743=VERTEX_POINT('',#71788);
#21744=VERTEX_POINT('',#71797);
#21745=VERTEX_POINT('',#71798);
#21746=VERTEX_POINT('',#71807);
#21747=VERTEX_POINT('',#71808);
#21748=VERTEX_POINT('',#71817);
#21749=VERTEX_POINT('',#71818);
#21750=VERTEX_POINT('',#71827);
#21751=VERTEX_POINT('',#71828);
#21752=VERTEX_POINT('',#71837);
#21753=VERTEX_POINT('',#71838);
#21754=VERTEX_POINT('',#71847);
#21755=VERTEX_POINT('',#71848);
#21756=VERTEX_POINT('',#71857);
#21757=VERTEX_POINT('',#71858);
#21758=VERTEX_POINT('',#71867);
#21759=VERTEX_POINT('',#71868);
#21760=VERTEX_POINT('',#71877);
#21761=VERTEX_POINT('',#71878);
#21762=VERTEX_POINT('',#71887);
#21763=VERTEX_POINT('',#71888);
#21764=VERTEX_POINT('',#71897);
#21765=VERTEX_POINT('',#71899);
#21766=VERTEX_POINT('',#71901);
#21767=VERTEX_POINT('',#71905);
#21768=VERTEX_POINT('',#71909);
#21769=VERTEX_POINT('',#71911);
#21770=VERTEX_POINT('',#71913);
#21771=VERTEX_POINT('',#71917);
#21772=VERTEX_POINT('',#71921);
#21773=VERTEX_POINT('',#71923);
#21774=VERTEX_POINT('',#71925);
#21775=VERTEX_POINT('',#71929);
#21776=VERTEX_POINT('',#71933);
#21777=VERTEX_POINT('',#71935);
#21778=VERTEX_POINT('',#71937);
#21779=VERTEX_POINT('',#71941);
#21780=VERTEX_POINT('',#71945);
#21781=VERTEX_POINT('',#71947);
#21782=VERTEX_POINT('',#71949);
#21783=VERTEX_POINT('',#71953);
#21784=VERTEX_POINT('',#71957);
#21785=VERTEX_POINT('',#71959);
#21786=VERTEX_POINT('',#71961);
#21787=VERTEX_POINT('',#71965);
#21788=VERTEX_POINT('',#71969);
#21789=VERTEX_POINT('',#71971);
#21790=VERTEX_POINT('',#71973);
#21791=VERTEX_POINT('',#71977);
#21792=VERTEX_POINT('',#71981);
#21793=VERTEX_POINT('',#71983);
#21794=VERTEX_POINT('',#71985);
#21795=VERTEX_POINT('',#71989);
#21796=VERTEX_POINT('',#71993);
#21797=VERTEX_POINT('',#71995);
#21798=VERTEX_POINT('',#71997);
#21799=VERTEX_POINT('',#72001);
#21800=VERTEX_POINT('',#72005);
#21801=VERTEX_POINT('',#72007);
#21802=VERTEX_POINT('',#72009);
#21803=VERTEX_POINT('',#72013);
#21804=VERTEX_POINT('',#72017);
#21805=VERTEX_POINT('',#72019);
#21806=VERTEX_POINT('',#72021);
#21807=VERTEX_POINT('',#72025);
#21808=VERTEX_POINT('',#72029);
#21809=VERTEX_POINT('',#72031);
#21810=VERTEX_POINT('',#72033);
#21811=VERTEX_POINT('',#72037);
#21812=VERTEX_POINT('',#72041);
#21813=VERTEX_POINT('',#72043);
#21814=VERTEX_POINT('',#72045);
#21815=VERTEX_POINT('',#72049);
#21816=VERTEX_POINT('',#72053);
#21817=VERTEX_POINT('',#72055);
#21818=VERTEX_POINT('',#72057);
#21819=VERTEX_POINT('',#72061);
#21820=VERTEX_POINT('',#72065);
#21821=VERTEX_POINT('',#72067);
#21822=VERTEX_POINT('',#72069);
#21823=VERTEX_POINT('',#72073);
#21824=VERTEX_POINT('',#72077);
#21825=VERTEX_POINT('',#72079);
#21826=VERTEX_POINT('',#72081);
#21827=VERTEX_POINT('',#72085);
#21828=VERTEX_POINT('',#72089);
#21829=VERTEX_POINT('',#72091);
#21830=VERTEX_POINT('',#72093);
#21831=VERTEX_POINT('',#72097);
#21832=VERTEX_POINT('',#72101);
#21833=VERTEX_POINT('',#72103);
#21834=VERTEX_POINT('',#72105);
#21835=VERTEX_POINT('',#72109);
#21836=VERTEX_POINT('',#72113);
#21837=VERTEX_POINT('',#72115);
#21838=VERTEX_POINT('',#72117);
#21839=VERTEX_POINT('',#72121);
#21840=VERTEX_POINT('',#72125);
#21841=VERTEX_POINT('',#72127);
#21842=VERTEX_POINT('',#72129);
#21843=VERTEX_POINT('',#72133);
#21844=VERTEX_POINT('',#72137);
#21845=VERTEX_POINT('',#72139);
#21846=VERTEX_POINT('',#72141);
#21847=VERTEX_POINT('',#72145);
#21848=VERTEX_POINT('',#72149);
#21849=VERTEX_POINT('',#72151);
#21850=VERTEX_POINT('',#72153);
#21851=VERTEX_POINT('',#72157);
#21852=VERTEX_POINT('',#72161);
#21853=VERTEX_POINT('',#72163);
#21854=VERTEX_POINT('',#72165);
#21855=VERTEX_POINT('',#72169);
#21856=VERTEX_POINT('',#72173);
#21857=VERTEX_POINT('',#72175);
#21858=VERTEX_POINT('',#72177);
#21859=VERTEX_POINT('',#72181);
#21860=VERTEX_POINT('',#72185);
#21861=VERTEX_POINT('',#72187);
#21862=VERTEX_POINT('',#72189);
#21863=VERTEX_POINT('',#72193);
#21864=VERTEX_POINT('',#72197);
#21865=VERTEX_POINT('',#72199);
#21866=VERTEX_POINT('',#72201);
#21867=VERTEX_POINT('',#72205);
#21868=VERTEX_POINT('',#72209);
#21869=VERTEX_POINT('',#72211);
#21870=VERTEX_POINT('',#72213);
#21871=VERTEX_POINT('',#72217);
#21872=VERTEX_POINT('',#72221);
#21873=VERTEX_POINT('',#72223);
#21874=VERTEX_POINT('',#72225);
#21875=VERTEX_POINT('',#72229);
#21876=VERTEX_POINT('',#72233);
#21877=VERTEX_POINT('',#72235);
#21878=VERTEX_POINT('',#72237);
#21879=VERTEX_POINT('',#72241);
#21880=VERTEX_POINT('',#72245);
#21881=VERTEX_POINT('',#72247);
#21882=VERTEX_POINT('',#72249);
#21883=VERTEX_POINT('',#72253);
#21884=VERTEX_POINT('',#72257);
#21885=VERTEX_POINT('',#72259);
#21886=VERTEX_POINT('',#72261);
#21887=VERTEX_POINT('',#72265);
#21888=VERTEX_POINT('',#72269);
#21889=VERTEX_POINT('',#72271);
#21890=VERTEX_POINT('',#72273);
#21891=VERTEX_POINT('',#72277);
#21892=VERTEX_POINT('',#72281);
#21893=VERTEX_POINT('',#72283);
#21894=VERTEX_POINT('',#72285);
#21895=VERTEX_POINT('',#72289);
#21896=VERTEX_POINT('',#72293);
#21897=VERTEX_POINT('',#72295);
#21898=VERTEX_POINT('',#72297);
#21899=VERTEX_POINT('',#72301);
#21900=VERTEX_POINT('',#72305);
#21901=VERTEX_POINT('',#72307);
#21902=VERTEX_POINT('',#72309);
#21903=VERTEX_POINT('',#72313);
#21904=VERTEX_POINT('',#72317);
#21905=VERTEX_POINT('',#72319);
#21906=VERTEX_POINT('',#72321);
#21907=VERTEX_POINT('',#72325);
#21908=VERTEX_POINT('',#72329);
#21909=VERTEX_POINT('',#72333);
#21910=VERTEX_POINT('',#72337);
#21911=VERTEX_POINT('',#72341);
#21912=VERTEX_POINT('',#72345);
#21913=VERTEX_POINT('',#72349);
#21914=VERTEX_POINT('',#72353);
#21915=VERTEX_POINT('',#72357);
#21916=VERTEX_POINT('',#72361);
#21917=VERTEX_POINT('',#72365);
#21918=VERTEX_POINT('',#72369);
#21919=VERTEX_POINT('',#72373);
#21920=VERTEX_POINT('',#72377);
#21921=VERTEX_POINT('',#72381);
#21922=VERTEX_POINT('',#72385);
#21923=VERTEX_POINT('',#72389);
#21924=VERTEX_POINT('',#72393);
#21925=VERTEX_POINT('',#72397);
#21926=VERTEX_POINT('',#72401);
#21927=VERTEX_POINT('',#72405);
#21928=VERTEX_POINT('',#72409);
#21929=VERTEX_POINT('',#72413);
#21930=VERTEX_POINT('',#72417);
#21931=VERTEX_POINT('',#72421);
#21932=VERTEX_POINT('',#72425);
#21933=VERTEX_POINT('',#72429);
#21934=VERTEX_POINT('',#72433);
#21935=VERTEX_POINT('',#72437);
#21936=VERTEX_POINT('',#72441);
#21937=VERTEX_POINT('',#72445);
#21938=VERTEX_POINT('',#72449);
#21939=VERTEX_POINT('',#72453);
#21940=VERTEX_POINT('',#72457);
#21941=VERTEX_POINT('',#72461);
#21942=VERTEX_POINT('',#72465);
#21943=VERTEX_POINT('',#72469);
#21944=VERTEX_POINT('',#72473);
#21945=VERTEX_POINT('',#72475);
#21946=VERTEX_POINT('',#72477);
#21947=VERTEX_POINT('',#72483);
#21948=VERTEX_POINT('',#72485);
#21949=VERTEX_POINT('',#72487);
#21950=VERTEX_POINT('',#72493);
#21951=VERTEX_POINT('',#72495);
#21952=VERTEX_POINT('',#72497);
#21953=VERTEX_POINT('',#72503);
#21954=VERTEX_POINT('',#72505);
#21955=VERTEX_POINT('',#72507);
#21956=VERTEX_POINT('',#72513);
#21957=VERTEX_POINT('',#72515);
#21958=VERTEX_POINT('',#72517);
#21959=VERTEX_POINT('',#72523);
#21960=VERTEX_POINT('',#72525);
#21961=VERTEX_POINT('',#72527);
#21962=VERTEX_POINT('',#72533);
#21963=VERTEX_POINT('',#72535);
#21964=VERTEX_POINT('',#72537);
#21965=VERTEX_POINT('',#72543);
#21966=VERTEX_POINT('',#72545);
#21967=VERTEX_POINT('',#72547);
#21968=VERTEX_POINT('',#72553);
#21969=VERTEX_POINT('',#72555);
#21970=VERTEX_POINT('',#72557);
#21971=VERTEX_POINT('',#72563);
#21972=VERTEX_POINT('',#72565);
#21973=VERTEX_POINT('',#72567);
#21974=VERTEX_POINT('',#72573);
#21975=VERTEX_POINT('',#72575);
#21976=VERTEX_POINT('',#72577);
#21977=VERTEX_POINT('',#72583);
#21978=VERTEX_POINT('',#72585);
#21979=VERTEX_POINT('',#72587);
#21980=VERTEX_POINT('',#72593);
#21981=VERTEX_POINT('',#72595);
#21982=VERTEX_POINT('',#72597);
#21983=VERTEX_POINT('',#72603);
#21984=VERTEX_POINT('',#72605);
#21985=VERTEX_POINT('',#72607);
#21986=VERTEX_POINT('',#72613);
#21987=VERTEX_POINT('',#72615);
#21988=VERTEX_POINT('',#72617);
#21989=VERTEX_POINT('',#72623);
#21990=VERTEX_POINT('',#72625);
#21991=VERTEX_POINT('',#72627);
#21992=VERTEX_POINT('',#72633);
#21993=VERTEX_POINT('',#72635);
#21994=VERTEX_POINT('',#72637);
#21995=VERTEX_POINT('',#72643);
#21996=VERTEX_POINT('',#72645);
#21997=VERTEX_POINT('',#72647);
#21998=VERTEX_POINT('',#72653);
#21999=VERTEX_POINT('',#72655);
#22000=VERTEX_POINT('',#72657);
#22001=VERTEX_POINT('',#72663);
#22002=VERTEX_POINT('',#72665);
#22003=VERTEX_POINT('',#72667);
#22004=VERTEX_POINT('',#72673);
#22005=VERTEX_POINT('',#72675);
#22006=VERTEX_POINT('',#72677);
#22007=VERTEX_POINT('',#72683);
#22008=VERTEX_POINT('',#72685);
#22009=VERTEX_POINT('',#72687);
#22010=VERTEX_POINT('',#72693);
#22011=VERTEX_POINT('',#72695);
#22012=VERTEX_POINT('',#72697);
#22013=VERTEX_POINT('',#72703);
#22014=VERTEX_POINT('',#72705);
#22015=VERTEX_POINT('',#72707);
#22016=VERTEX_POINT('',#72713);
#22017=VERTEX_POINT('',#72715);
#22018=VERTEX_POINT('',#72717);
#22019=VERTEX_POINT('',#72723);
#22020=VERTEX_POINT('',#72725);
#22021=VERTEX_POINT('',#72727);
#22022=VERTEX_POINT('',#72733);
#22023=VERTEX_POINT('',#72735);
#22024=VERTEX_POINT('',#72737);
#22025=VERTEX_POINT('',#72743);
#22026=VERTEX_POINT('',#72745);
#22027=VERTEX_POINT('',#72747);
#22028=VERTEX_POINT('',#72753);
#22029=VERTEX_POINT('',#72755);
#22030=VERTEX_POINT('',#72757);
#22031=VERTEX_POINT('',#72763);
#22032=VERTEX_POINT('',#72765);
#22033=VERTEX_POINT('',#72767);
#22034=VERTEX_POINT('',#72773);
#22035=VERTEX_POINT('',#72775);
#22036=VERTEX_POINT('',#72777);
#22037=VERTEX_POINT('',#72783);
#22038=VERTEX_POINT('',#72785);
#22039=VERTEX_POINT('',#72787);
#22040=VERTEX_POINT('',#72793);
#22041=VERTEX_POINT('',#72795);
#22042=VERTEX_POINT('',#72797);
#22043=VERTEX_POINT('',#72803);
#22044=VERTEX_POINT('',#72805);
#22045=VERTEX_POINT('',#72807);
#22046=VERTEX_POINT('',#72813);
#22047=VERTEX_POINT('',#72815);
#22048=VERTEX_POINT('',#72817);
#22049=VERTEX_POINT('',#72823);
#22050=VERTEX_POINT('',#72829);
#22051=VERTEX_POINT('',#72833);
#22052=VERTEX_POINT('',#72837);
#22053=VERTEX_POINT('',#72841);
#22054=VERTEX_POINT('',#72845);
#22055=VERTEX_POINT('',#72849);
#22056=VERTEX_POINT('',#72853);
#22057=VERTEX_POINT('',#72857);
#22058=VERTEX_POINT('',#72861);
#22059=VERTEX_POINT('',#72865);
#22060=VERTEX_POINT('',#72869);
#22061=VERTEX_POINT('',#72873);
#22062=VERTEX_POINT('',#72877);
#22063=VERTEX_POINT('',#72881);
#22064=VERTEX_POINT('',#72885);
#22065=VERTEX_POINT('',#72889);
#22066=VERTEX_POINT('',#72893);
#22067=VERTEX_POINT('',#72897);
#22068=VERTEX_POINT('',#72901);
#22069=VERTEX_POINT('',#72905);
#22070=VERTEX_POINT('',#72909);
#22071=VERTEX_POINT('',#72913);
#22072=VERTEX_POINT('',#72917);
#22073=VERTEX_POINT('',#72921);
#22074=VERTEX_POINT('',#72925);
#22075=VERTEX_POINT('',#72929);
#22076=VERTEX_POINT('',#72933);
#22077=VERTEX_POINT('',#72937);
#22078=VERTEX_POINT('',#72941);
#22079=VERTEX_POINT('',#72945);
#22080=VERTEX_POINT('',#72949);
#22081=VERTEX_POINT('',#72953);
#22082=VERTEX_POINT('',#72957);
#22083=VERTEX_POINT('',#72961);
#22084=VERTEX_POINT('',#72965);
#22085=VERTEX_POINT('',#72969);
#22086=VERTEX_POINT('',#72973);
#22087=VERTEX_POINT('',#72979);
#22088=VERTEX_POINT('',#72985);
#22089=VERTEX_POINT('',#72991);
#22090=VERTEX_POINT('',#72997);
#22091=VERTEX_POINT('',#73003);
#22092=VERTEX_POINT('',#73009);
#22093=VERTEX_POINT('',#73015);
#22094=VERTEX_POINT('',#73021);
#22095=VERTEX_POINT('',#73027);
#22096=VERTEX_POINT('',#73033);
#22097=VERTEX_POINT('',#73039);
#22098=VERTEX_POINT('',#73045);
#22099=VERTEX_POINT('',#73051);
#22100=VERTEX_POINT('',#73057);
#22101=VERTEX_POINT('',#73063);
#22102=VERTEX_POINT('',#73069);
#22103=VERTEX_POINT('',#73075);
#22104=VERTEX_POINT('',#73077);
#22105=VERTEX_POINT('',#73085);
#22106=VERTEX_POINT('',#73091);
#22107=VERTEX_POINT('',#73097);
#22108=VERTEX_POINT('',#73103);
#22109=VERTEX_POINT('',#73109);
#22110=VERTEX_POINT('',#73115);
#22111=VERTEX_POINT('',#73121);
#22112=VERTEX_POINT('',#73127);
#22113=VERTEX_POINT('',#73133);
#22114=VERTEX_POINT('',#73139);
#22115=VERTEX_POINT('',#73145);
#22116=VERTEX_POINT('',#73151);
#22117=VERTEX_POINT('',#73157);
#22118=VERTEX_POINT('',#73163);
#22119=VERTEX_POINT('',#73169);
#22120=VERTEX_POINT('',#73175);
#22121=VERTEX_POINT('',#73181);
#22122=VERTEX_POINT('',#73187);
#22123=VERTEX_POINT('',#73193);
#22124=VERTEX_POINT('',#73197);
#22125=VERTEX_POINT('',#73201);
#22126=VERTEX_POINT('',#73205);
#22127=VERTEX_POINT('',#73209);
#22128=VERTEX_POINT('',#73213);
#22129=VERTEX_POINT('',#73217);
#22130=VERTEX_POINT('',#73221);
#22131=VERTEX_POINT('',#73225);
#22132=VERTEX_POINT('',#73229);
#22133=VERTEX_POINT('',#73233);
#22134=VERTEX_POINT('',#73237);
#22135=VERTEX_POINT('',#73241);
#22136=VERTEX_POINT('',#73245);
#22137=VERTEX_POINT('',#73251);
#22138=VERTEX_POINT('',#73255);
#22139=VERTEX_POINT('',#73259);
#22140=VERTEX_POINT('',#73263);
#22141=VERTEX_POINT('',#73267);
#22142=VERTEX_POINT('',#73271);
#22143=VERTEX_POINT('',#73275);
#22144=VERTEX_POINT('',#73279);
#22145=VERTEX_POINT('',#73283);
#22146=VERTEX_POINT('',#73287);
#22147=VERTEX_POINT('',#73291);
#22148=VERTEX_POINT('',#73295);
#22149=VERTEX_POINT('',#73305);
#22150=VERTEX_POINT('',#73307);
#22151=VERTEX_POINT('',#73381);
#22152=VERTEX_POINT('',#73455);
#22153=VERTEX_POINT('',#73457);
#22154=VERTEX_POINT('',#73459);
#22155=VERTEX_POINT('',#73461);
#22156=VERTEX_POINT('',#73463);
#22157=VERTEX_POINT('',#73465);
#22158=VERTEX_POINT('',#73467);
#22159=VERTEX_POINT('',#73469);
#22160=VERTEX_POINT('',#73471);
#22161=VERTEX_POINT('',#73473);
#22162=VERTEX_POINT('',#73475);
#22163=VERTEX_POINT('',#73477);
#22164=VERTEX_POINT('',#73479);
#22165=VERTEX_POINT('',#73481);
#22166=VERTEX_POINT('',#73515);
#22167=VERTEX_POINT('',#73519);
#22168=VERTEX_POINT('',#73523);
#22169=VERTEX_POINT('',#73527);
#22170=VERTEX_POINT('',#73531);
#22171=VERTEX_POINT('',#73535);
#22172=VERTEX_POINT('',#73539);
#22173=VERTEX_POINT('',#73543);
#22174=VERTEX_POINT('',#73547);
#22175=VERTEX_POINT('',#73551);
#22176=VERTEX_POINT('',#73555);
#22177=VERTEX_POINT('',#73559);
#22178=VERTEX_POINT('',#73566);
#22179=VERTEX_POINT('',#73568);
#22180=VERTEX_POINT('',#73570);
#22181=VERTEX_POINT('',#73572);
#22182=VERTEX_POINT('',#73574);
#22183=VERTEX_POINT('',#73576);
#22184=VERTEX_POINT('',#73578);
#22185=VERTEX_POINT('',#73580);
#22186=VERTEX_POINT('',#73582);
#22187=VERTEX_POINT('',#73584);
#22188=VERTEX_POINT('',#73586);
#22189=VERTEX_POINT('',#73588);
#22190=VERTEX_POINT('',#73590);
#22191=VERTEX_POINT('',#73592);
#22192=VERTEX_POINT('',#73626);
#22193=VERTEX_POINT('',#73630);
#22194=VERTEX_POINT('',#73634);
#22195=VERTEX_POINT('',#73638);
#22196=VERTEX_POINT('',#73642);
#22197=VERTEX_POINT('',#73646);
#22198=VERTEX_POINT('',#73650);
#22199=VERTEX_POINT('',#73654);
#22200=VERTEX_POINT('',#73658);
#22201=VERTEX_POINT('',#73662);
#22202=VERTEX_POINT('',#73666);
#22203=VERTEX_POINT('',#73670);
#22204=VERTEX_POINT('',#73677);
#22205=VERTEX_POINT('',#73679);
#22206=VERTEX_POINT('',#73681);
#22207=VERTEX_POINT('',#73683);
#22208=VERTEX_POINT('',#73685);
#22209=VERTEX_POINT('',#73687);
#22210=VERTEX_POINT('',#73689);
#22211=VERTEX_POINT('',#73691);
#22212=VERTEX_POINT('',#73693);
#22213=VERTEX_POINT('',#73695);
#22214=VERTEX_POINT('',#73697);
#22215=VERTEX_POINT('',#73699);
#22216=VERTEX_POINT('',#73701);
#22217=VERTEX_POINT('',#73703);
#22218=VERTEX_POINT('',#73737);
#22219=VERTEX_POINT('',#73741);
#22220=VERTEX_POINT('',#73745);
#22221=VERTEX_POINT('',#73749);
#22222=VERTEX_POINT('',#73753);
#22223=VERTEX_POINT('',#73757);
#22224=VERTEX_POINT('',#73761);
#22225=VERTEX_POINT('',#73765);
#22226=VERTEX_POINT('',#73769);
#22227=VERTEX_POINT('',#73773);
#22228=VERTEX_POINT('',#73777);
#22229=VERTEX_POINT('',#73781);
#22230=VERTEX_POINT('',#73788);
#22231=VERTEX_POINT('',#73790);
#22232=VERTEX_POINT('',#73792);
#22233=VERTEX_POINT('',#73794);
#22234=VERTEX_POINT('',#73796);
#22235=VERTEX_POINT('',#73798);
#22236=VERTEX_POINT('',#73800);
#22237=VERTEX_POINT('',#73802);
#22238=VERTEX_POINT('',#73804);
#22239=VERTEX_POINT('',#73806);
#22240=VERTEX_POINT('',#73808);
#22241=VERTEX_POINT('',#73810);
#22242=VERTEX_POINT('',#73812);
#22243=VERTEX_POINT('',#73814);
#22244=VERTEX_POINT('',#73848);
#22245=VERTEX_POINT('',#73852);
#22246=VERTEX_POINT('',#73856);
#22247=VERTEX_POINT('',#73860);
#22248=VERTEX_POINT('',#73864);
#22249=VERTEX_POINT('',#73868);
#22250=VERTEX_POINT('',#73872);
#22251=VERTEX_POINT('',#73876);
#22252=VERTEX_POINT('',#73880);
#22253=VERTEX_POINT('',#73884);
#22254=VERTEX_POINT('',#73888);
#22255=VERTEX_POINT('',#73892);
#22256=VERTEX_POINT('',#73899);
#22257=VERTEX_POINT('',#73901);
#22258=VERTEX_POINT('',#73903);
#22259=VERTEX_POINT('',#73905);
#22260=VERTEX_POINT('',#73907);
#22261=VERTEX_POINT('',#73909);
#22262=VERTEX_POINT('',#73911);
#22263=VERTEX_POINT('',#73913);
#22264=VERTEX_POINT('',#73915);
#22265=VERTEX_POINT('',#73917);
#22266=VERTEX_POINT('',#73919);
#22267=VERTEX_POINT('',#73921);
#22268=VERTEX_POINT('',#73923);
#22269=VERTEX_POINT('',#73925);
#22270=VERTEX_POINT('',#73959);
#22271=VERTEX_POINT('',#73963);
#22272=VERTEX_POINT('',#73967);
#22273=VERTEX_POINT('',#73971);
#22274=VERTEX_POINT('',#73975);
#22275=VERTEX_POINT('',#73979);
#22276=VERTEX_POINT('',#73983);
#22277=VERTEX_POINT('',#73987);
#22278=VERTEX_POINT('',#73991);
#22279=VERTEX_POINT('',#73995);
#22280=VERTEX_POINT('',#73999);
#22281=VERTEX_POINT('',#74003);
#22282=VERTEX_POINT('',#74010);
#22283=VERTEX_POINT('',#74012);
#22284=VERTEX_POINT('',#74014);
#22285=VERTEX_POINT('',#74016);
#22286=VERTEX_POINT('',#74018);
#22287=VERTEX_POINT('',#74020);
#22288=VERTEX_POINT('',#74022);
#22289=VERTEX_POINT('',#74024);
#22290=VERTEX_POINT('',#74026);
#22291=VERTEX_POINT('',#74028);
#22292=VERTEX_POINT('',#74030);
#22293=VERTEX_POINT('',#74032);
#22294=VERTEX_POINT('',#74034);
#22295=VERTEX_POINT('',#74036);
#22296=VERTEX_POINT('',#74070);
#22297=VERTEX_POINT('',#74074);
#22298=VERTEX_POINT('',#74078);
#22299=VERTEX_POINT('',#74082);
#22300=VERTEX_POINT('',#74086);
#22301=VERTEX_POINT('',#74090);
#22302=VERTEX_POINT('',#74094);
#22303=VERTEX_POINT('',#74098);
#22304=VERTEX_POINT('',#74102);
#22305=VERTEX_POINT('',#74106);
#22306=VERTEX_POINT('',#74110);
#22307=VERTEX_POINT('',#74114);
#22308=VERTEX_POINT('',#74121);
#22309=VERTEX_POINT('',#74123);
#22310=VERTEX_POINT('',#74125);
#22311=VERTEX_POINT('',#74127);
#22312=VERTEX_POINT('',#74129);
#22313=VERTEX_POINT('',#74131);
#22314=VERTEX_POINT('',#74133);
#22315=VERTEX_POINT('',#74135);
#22316=VERTEX_POINT('',#74137);
#22317=VERTEX_POINT('',#74139);
#22318=VERTEX_POINT('',#74141);
#22319=VERTEX_POINT('',#74143);
#22320=VERTEX_POINT('',#74145);
#22321=VERTEX_POINT('',#74147);
#22322=VERTEX_POINT('',#74181);
#22323=VERTEX_POINT('',#74185);
#22324=VERTEX_POINT('',#74189);
#22325=VERTEX_POINT('',#74193);
#22326=VERTEX_POINT('',#74197);
#22327=VERTEX_POINT('',#74201);
#22328=VERTEX_POINT('',#74205);
#22329=VERTEX_POINT('',#74209);
#22330=VERTEX_POINT('',#74213);
#22331=VERTEX_POINT('',#74217);
#22332=VERTEX_POINT('',#74221);
#22333=VERTEX_POINT('',#74225);
#22334=VERTEX_POINT('',#74232);
#22335=VERTEX_POINT('',#74234);
#22336=VERTEX_POINT('',#74236);
#22337=VERTEX_POINT('',#74238);
#22338=VERTEX_POINT('',#74240);
#22339=VERTEX_POINT('',#74242);
#22340=VERTEX_POINT('',#74244);
#22341=VERTEX_POINT('',#74246);
#22342=VERTEX_POINT('',#74248);
#22343=VERTEX_POINT('',#74250);
#22344=VERTEX_POINT('',#74252);
#22345=VERTEX_POINT('',#74254);
#22346=VERTEX_POINT('',#74256);
#22347=VERTEX_POINT('',#74258);
#22348=VERTEX_POINT('',#74292);
#22349=VERTEX_POINT('',#74296);
#22350=VERTEX_POINT('',#74300);
#22351=VERTEX_POINT('',#74304);
#22352=VERTEX_POINT('',#74308);
#22353=VERTEX_POINT('',#74312);
#22354=VERTEX_POINT('',#74316);
#22355=VERTEX_POINT('',#74320);
#22356=VERTEX_POINT('',#74324);
#22357=VERTEX_POINT('',#74328);
#22358=VERTEX_POINT('',#74332);
#22359=VERTEX_POINT('',#74336);
#22360=VERTEX_POINT('',#74343);
#22361=VERTEX_POINT('',#74345);
#22362=VERTEX_POINT('',#74347);
#22363=VERTEX_POINT('',#74349);
#22364=VERTEX_POINT('',#74351);
#22365=VERTEX_POINT('',#74353);
#22366=VERTEX_POINT('',#74355);
#22367=VERTEX_POINT('',#74357);
#22368=VERTEX_POINT('',#74359);
#22369=VERTEX_POINT('',#74361);
#22370=VERTEX_POINT('',#74363);
#22371=VERTEX_POINT('',#74365);
#22372=VERTEX_POINT('',#74367);
#22373=VERTEX_POINT('',#74369);
#22374=VERTEX_POINT('',#74403);
#22375=VERTEX_POINT('',#74407);
#22376=VERTEX_POINT('',#74411);
#22377=VERTEX_POINT('',#74415);
#22378=VERTEX_POINT('',#74419);
#22379=VERTEX_POINT('',#74423);
#22380=VERTEX_POINT('',#74427);
#22381=VERTEX_POINT('',#74431);
#22382=VERTEX_POINT('',#74435);
#22383=VERTEX_POINT('',#74439);
#22384=VERTEX_POINT('',#74443);
#22385=VERTEX_POINT('',#74447);
#22386=VERTEX_POINT('',#74454);
#22387=VERTEX_POINT('',#74456);
#22388=VERTEX_POINT('',#74458);
#22389=VERTEX_POINT('',#74460);
#22390=VERTEX_POINT('',#74462);
#22391=VERTEX_POINT('',#74464);
#22392=VERTEX_POINT('',#74466);
#22393=VERTEX_POINT('',#74468);
#22394=VERTEX_POINT('',#74470);
#22395=VERTEX_POINT('',#74472);
#22396=VERTEX_POINT('',#74474);
#22397=VERTEX_POINT('',#74476);
#22398=VERTEX_POINT('',#74478);
#22399=VERTEX_POINT('',#74480);
#22400=VERTEX_POINT('',#74514);
#22401=VERTEX_POINT('',#74518);
#22402=VERTEX_POINT('',#74522);
#22403=VERTEX_POINT('',#74526);
#22404=VERTEX_POINT('',#74530);
#22405=VERTEX_POINT('',#74534);
#22406=VERTEX_POINT('',#74538);
#22407=VERTEX_POINT('',#74542);
#22408=VERTEX_POINT('',#74546);
#22409=VERTEX_POINT('',#74550);
#22410=VERTEX_POINT('',#74554);
#22411=VERTEX_POINT('',#74558);
#22412=VERTEX_POINT('',#74565);
#22413=VERTEX_POINT('',#74567);
#22414=VERTEX_POINT('',#74569);
#22415=VERTEX_POINT('',#74571);
#22416=VERTEX_POINT('',#74573);
#22417=VERTEX_POINT('',#74575);
#22418=VERTEX_POINT('',#74577);
#22419=VERTEX_POINT('',#74579);
#22420=VERTEX_POINT('',#74581);
#22421=VERTEX_POINT('',#74583);
#22422=VERTEX_POINT('',#74585);
#22423=VERTEX_POINT('',#74587);
#22424=VERTEX_POINT('',#74589);
#22425=VERTEX_POINT('',#74591);
#22426=VERTEX_POINT('',#74625);
#22427=VERTEX_POINT('',#74629);
#22428=VERTEX_POINT('',#74633);
#22429=VERTEX_POINT('',#74637);
#22430=VERTEX_POINT('',#74641);
#22431=VERTEX_POINT('',#74645);
#22432=VERTEX_POINT('',#74649);
#22433=VERTEX_POINT('',#74653);
#22434=VERTEX_POINT('',#74657);
#22435=VERTEX_POINT('',#74661);
#22436=VERTEX_POINT('',#74665);
#22437=VERTEX_POINT('',#74669);
#22438=VERTEX_POINT('',#74676);
#22439=VERTEX_POINT('',#74678);
#22440=VERTEX_POINT('',#74680);
#22441=VERTEX_POINT('',#74682);
#22442=VERTEX_POINT('',#74684);
#22443=VERTEX_POINT('',#74686);
#22444=VERTEX_POINT('',#74688);
#22445=VERTEX_POINT('',#74690);
#22446=VERTEX_POINT('',#74692);
#22447=VERTEX_POINT('',#74694);
#22448=VERTEX_POINT('',#74696);
#22449=VERTEX_POINT('',#74698);
#22450=VERTEX_POINT('',#74700);
#22451=VERTEX_POINT('',#74702);
#22452=VERTEX_POINT('',#74736);
#22453=VERTEX_POINT('',#74740);
#22454=VERTEX_POINT('',#74744);
#22455=VERTEX_POINT('',#74748);
#22456=VERTEX_POINT('',#74752);
#22457=VERTEX_POINT('',#74756);
#22458=VERTEX_POINT('',#74760);
#22459=VERTEX_POINT('',#74764);
#22460=VERTEX_POINT('',#74768);
#22461=VERTEX_POINT('',#74772);
#22462=VERTEX_POINT('',#74776);
#22463=VERTEX_POINT('',#74780);
#22464=VERTEX_POINT('',#74787);
#22465=VERTEX_POINT('',#74789);
#22466=VERTEX_POINT('',#74791);
#22467=VERTEX_POINT('',#74793);
#22468=VERTEX_POINT('',#74795);
#22469=VERTEX_POINT('',#74797);
#22470=VERTEX_POINT('',#74799);
#22471=VERTEX_POINT('',#74801);
#22472=VERTEX_POINT('',#74803);
#22473=VERTEX_POINT('',#74805);
#22474=VERTEX_POINT('',#74807);
#22475=VERTEX_POINT('',#74809);
#22476=VERTEX_POINT('',#74811);
#22477=VERTEX_POINT('',#74813);
#22478=VERTEX_POINT('',#74847);
#22479=VERTEX_POINT('',#74851);
#22480=VERTEX_POINT('',#74855);
#22481=VERTEX_POINT('',#74859);
#22482=VERTEX_POINT('',#74863);
#22483=VERTEX_POINT('',#74867);
#22484=VERTEX_POINT('',#74871);
#22485=VERTEX_POINT('',#74875);
#22486=VERTEX_POINT('',#74879);
#22487=VERTEX_POINT('',#74883);
#22488=VERTEX_POINT('',#74887);
#22489=VERTEX_POINT('',#74891);
#22490=VERTEX_POINT('',#74898);
#22491=VERTEX_POINT('',#74900);
#22492=VERTEX_POINT('',#74902);
#22493=VERTEX_POINT('',#74904);
#22494=VERTEX_POINT('',#74906);
#22495=VERTEX_POINT('',#74908);
#22496=VERTEX_POINT('',#74910);
#22497=VERTEX_POINT('',#74912);
#22498=VERTEX_POINT('',#74914);
#22499=VERTEX_POINT('',#74916);
#22500=VERTEX_POINT('',#74918);
#22501=VERTEX_POINT('',#74920);
#22502=VERTEX_POINT('',#74922);
#22503=VERTEX_POINT('',#74924);
#22504=VERTEX_POINT('',#74958);
#22505=VERTEX_POINT('',#74962);
#22506=VERTEX_POINT('',#74966);
#22507=VERTEX_POINT('',#74970);
#22508=VERTEX_POINT('',#74974);
#22509=VERTEX_POINT('',#74978);
#22510=VERTEX_POINT('',#74982);
#22511=VERTEX_POINT('',#74986);
#22512=VERTEX_POINT('',#74990);
#22513=VERTEX_POINT('',#74994);
#22514=VERTEX_POINT('',#74998);
#22515=VERTEX_POINT('',#75002);
#22516=VERTEX_POINT('',#75009);
#22517=VERTEX_POINT('',#75011);
#22518=VERTEX_POINT('',#75013);
#22519=VERTEX_POINT('',#75015);
#22520=VERTEX_POINT('',#75017);
#22521=VERTEX_POINT('',#75019);
#22522=VERTEX_POINT('',#75021);
#22523=VERTEX_POINT('',#75023);
#22524=VERTEX_POINT('',#75025);
#22525=VERTEX_POINT('',#75027);
#22526=VERTEX_POINT('',#75029);
#22527=VERTEX_POINT('',#75031);
#22528=VERTEX_POINT('',#75033);
#22529=VERTEX_POINT('',#75035);
#22530=VERTEX_POINT('',#75069);
#22531=VERTEX_POINT('',#75073);
#22532=VERTEX_POINT('',#75077);
#22533=VERTEX_POINT('',#75081);
#22534=VERTEX_POINT('',#75085);
#22535=VERTEX_POINT('',#75089);
#22536=VERTEX_POINT('',#75093);
#22537=VERTEX_POINT('',#75097);
#22538=VERTEX_POINT('',#75101);
#22539=VERTEX_POINT('',#75105);
#22540=VERTEX_POINT('',#75109);
#22541=VERTEX_POINT('',#75113);
#22542=VERTEX_POINT('',#75120);
#22543=VERTEX_POINT('',#75122);
#22544=VERTEX_POINT('',#75124);
#22545=VERTEX_POINT('',#75126);
#22546=VERTEX_POINT('',#75128);
#22547=VERTEX_POINT('',#75130);
#22548=VERTEX_POINT('',#75132);
#22549=VERTEX_POINT('',#75134);
#22550=VERTEX_POINT('',#75136);
#22551=VERTEX_POINT('',#75138);
#22552=VERTEX_POINT('',#75140);
#22553=VERTEX_POINT('',#75142);
#22554=VERTEX_POINT('',#75144);
#22555=VERTEX_POINT('',#75146);
#22556=VERTEX_POINT('',#75180);
#22557=VERTEX_POINT('',#75184);
#22558=VERTEX_POINT('',#75188);
#22559=VERTEX_POINT('',#75192);
#22560=VERTEX_POINT('',#75196);
#22561=VERTEX_POINT('',#75200);
#22562=VERTEX_POINT('',#75204);
#22563=VERTEX_POINT('',#75208);
#22564=VERTEX_POINT('',#75212);
#22565=VERTEX_POINT('',#75216);
#22566=VERTEX_POINT('',#75220);
#22567=VERTEX_POINT('',#75224);
#22568=VERTEX_POINT('',#75231);
#22569=VERTEX_POINT('',#75233);
#22570=VERTEX_POINT('',#75235);
#22571=VERTEX_POINT('',#75237);
#22572=VERTEX_POINT('',#75239);
#22573=VERTEX_POINT('',#75241);
#22574=VERTEX_POINT('',#75243);
#22575=VERTEX_POINT('',#75245);
#22576=VERTEX_POINT('',#75247);
#22577=VERTEX_POINT('',#75249);
#22578=VERTEX_POINT('',#75251);
#22579=VERTEX_POINT('',#75253);
#22580=VERTEX_POINT('',#75255);
#22581=VERTEX_POINT('',#75257);
#22582=VERTEX_POINT('',#75291);
#22583=VERTEX_POINT('',#75295);
#22584=VERTEX_POINT('',#75299);
#22585=VERTEX_POINT('',#75303);
#22586=VERTEX_POINT('',#75307);
#22587=VERTEX_POINT('',#75311);
#22588=VERTEX_POINT('',#75315);
#22589=VERTEX_POINT('',#75319);
#22590=VERTEX_POINT('',#75323);
#22591=VERTEX_POINT('',#75327);
#22592=VERTEX_POINT('',#75331);
#22593=VERTEX_POINT('',#75335);
#22594=VERTEX_POINT('',#75342);
#22595=VERTEX_POINT('',#75344);
#22596=VERTEX_POINT('',#75346);
#22597=VERTEX_POINT('',#75348);
#22598=VERTEX_POINT('',#75350);
#22599=VERTEX_POINT('',#75352);
#22600=VERTEX_POINT('',#75354);
#22601=VERTEX_POINT('',#75356);
#22602=VERTEX_POINT('',#75358);
#22603=VERTEX_POINT('',#75360);
#22604=VERTEX_POINT('',#75362);
#22605=VERTEX_POINT('',#75364);
#22606=VERTEX_POINT('',#75366);
#22607=VERTEX_POINT('',#75368);
#22608=VERTEX_POINT('',#75402);
#22609=VERTEX_POINT('',#75406);
#22610=VERTEX_POINT('',#75410);
#22611=VERTEX_POINT('',#75414);
#22612=VERTEX_POINT('',#75418);
#22613=VERTEX_POINT('',#75422);
#22614=VERTEX_POINT('',#75426);
#22615=VERTEX_POINT('',#75430);
#22616=VERTEX_POINT('',#75434);
#22617=VERTEX_POINT('',#75438);
#22618=VERTEX_POINT('',#75442);
#22619=VERTEX_POINT('',#75446);
#22620=VERTEX_POINT('',#75453);
#22621=VERTEX_POINT('',#75455);
#22622=VERTEX_POINT('',#75457);
#22623=VERTEX_POINT('',#75459);
#22624=VERTEX_POINT('',#75461);
#22625=VERTEX_POINT('',#75463);
#22626=VERTEX_POINT('',#75465);
#22627=VERTEX_POINT('',#75467);
#22628=VERTEX_POINT('',#75469);
#22629=VERTEX_POINT('',#75471);
#22630=VERTEX_POINT('',#75473);
#22631=VERTEX_POINT('',#75475);
#22632=VERTEX_POINT('',#75477);
#22633=VERTEX_POINT('',#75479);
#22634=VERTEX_POINT('',#75513);
#22635=VERTEX_POINT('',#75517);
#22636=VERTEX_POINT('',#75521);
#22637=VERTEX_POINT('',#75525);
#22638=VERTEX_POINT('',#75529);
#22639=VERTEX_POINT('',#75533);
#22640=VERTEX_POINT('',#75537);
#22641=VERTEX_POINT('',#75541);
#22642=VERTEX_POINT('',#75545);
#22643=VERTEX_POINT('',#75549);
#22644=VERTEX_POINT('',#75553);
#22645=VERTEX_POINT('',#75557);
#22646=VERTEX_POINT('',#75564);
#22647=VERTEX_POINT('',#75566);
#22648=VERTEX_POINT('',#75568);
#22649=VERTEX_POINT('',#75570);
#22650=VERTEX_POINT('',#75572);
#22651=VERTEX_POINT('',#75574);
#22652=VERTEX_POINT('',#75576);
#22653=VERTEX_POINT('',#75578);
#22654=VERTEX_POINT('',#75580);
#22655=VERTEX_POINT('',#75582);
#22656=VERTEX_POINT('',#75584);
#22657=VERTEX_POINT('',#75586);
#22658=VERTEX_POINT('',#75588);
#22659=VERTEX_POINT('',#75590);
#22660=VERTEX_POINT('',#75624);
#22661=VERTEX_POINT('',#75628);
#22662=VERTEX_POINT('',#75632);
#22663=VERTEX_POINT('',#75636);
#22664=VERTEX_POINT('',#75640);
#22665=VERTEX_POINT('',#75644);
#22666=VERTEX_POINT('',#75648);
#22667=VERTEX_POINT('',#75652);
#22668=VERTEX_POINT('',#75656);
#22669=VERTEX_POINT('',#75660);
#22670=VERTEX_POINT('',#75664);
#22671=VERTEX_POINT('',#75668);
#22672=VERTEX_POINT('',#75675);
#22673=VERTEX_POINT('',#75677);
#22674=VERTEX_POINT('',#75679);
#22675=VERTEX_POINT('',#75681);
#22676=VERTEX_POINT('',#75683);
#22677=VERTEX_POINT('',#75685);
#22678=VERTEX_POINT('',#75687);
#22679=VERTEX_POINT('',#75689);
#22680=VERTEX_POINT('',#75691);
#22681=VERTEX_POINT('',#75693);
#22682=VERTEX_POINT('',#75695);
#22683=VERTEX_POINT('',#75697);
#22684=VERTEX_POINT('',#75699);
#22685=VERTEX_POINT('',#75701);
#22686=VERTEX_POINT('',#75735);
#22687=VERTEX_POINT('',#75739);
#22688=VERTEX_POINT('',#75743);
#22689=VERTEX_POINT('',#75747);
#22690=VERTEX_POINT('',#75751);
#22691=VERTEX_POINT('',#75755);
#22692=VERTEX_POINT('',#75759);
#22693=VERTEX_POINT('',#75763);
#22694=VERTEX_POINT('',#75767);
#22695=VERTEX_POINT('',#75771);
#22696=VERTEX_POINT('',#75775);
#22697=VERTEX_POINT('',#75779);
#22698=VERTEX_POINT('',#75786);
#22699=VERTEX_POINT('',#75788);
#22700=VERTEX_POINT('',#75790);
#22701=VERTEX_POINT('',#75792);
#22702=VERTEX_POINT('',#75794);
#22703=VERTEX_POINT('',#75796);
#22704=VERTEX_POINT('',#75798);
#22705=VERTEX_POINT('',#75800);
#22706=VERTEX_POINT('',#75802);
#22707=VERTEX_POINT('',#75804);
#22708=VERTEX_POINT('',#75806);
#22709=VERTEX_POINT('',#75808);
#22710=VERTEX_POINT('',#75810);
#22711=VERTEX_POINT('',#75812);
#22712=VERTEX_POINT('',#75846);
#22713=VERTEX_POINT('',#75850);
#22714=VERTEX_POINT('',#75854);
#22715=VERTEX_POINT('',#75858);
#22716=VERTEX_POINT('',#75862);
#22717=VERTEX_POINT('',#75866);
#22718=VERTEX_POINT('',#75870);
#22719=VERTEX_POINT('',#75874);
#22720=VERTEX_POINT('',#75878);
#22721=VERTEX_POINT('',#75882);
#22722=VERTEX_POINT('',#75886);
#22723=VERTEX_POINT('',#75890);
#22724=VERTEX_POINT('',#75897);
#22725=VERTEX_POINT('',#75899);
#22726=VERTEX_POINT('',#75901);
#22727=VERTEX_POINT('',#75903);
#22728=VERTEX_POINT('',#75905);
#22729=VERTEX_POINT('',#75907);
#22730=VERTEX_POINT('',#75909);
#22731=VERTEX_POINT('',#75911);
#22732=VERTEX_POINT('',#75913);
#22733=VERTEX_POINT('',#75915);
#22734=VERTEX_POINT('',#75917);
#22735=VERTEX_POINT('',#75919);
#22736=VERTEX_POINT('',#75921);
#22737=VERTEX_POINT('',#75923);
#22738=VERTEX_POINT('',#75957);
#22739=VERTEX_POINT('',#75961);
#22740=VERTEX_POINT('',#75965);
#22741=VERTEX_POINT('',#75969);
#22742=VERTEX_POINT('',#75973);
#22743=VERTEX_POINT('',#75977);
#22744=VERTEX_POINT('',#75981);
#22745=VERTEX_POINT('',#75985);
#22746=VERTEX_POINT('',#75989);
#22747=VERTEX_POINT('',#75993);
#22748=VERTEX_POINT('',#75997);
#22749=VERTEX_POINT('',#76001);
#22750=VERTEX_POINT('',#76008);
#22751=VERTEX_POINT('',#76010);
#22752=VERTEX_POINT('',#76012);
#22753=VERTEX_POINT('',#76014);
#22754=VERTEX_POINT('',#76016);
#22755=VERTEX_POINT('',#76018);
#22756=VERTEX_POINT('',#76020);
#22757=VERTEX_POINT('',#76022);
#22758=VERTEX_POINT('',#76024);
#22759=VERTEX_POINT('',#76026);
#22760=VERTEX_POINT('',#76028);
#22761=VERTEX_POINT('',#76030);
#22762=VERTEX_POINT('',#76032);
#22763=VERTEX_POINT('',#76034);
#22764=VERTEX_POINT('',#76068);
#22765=VERTEX_POINT('',#76072);
#22766=VERTEX_POINT('',#76076);
#22767=VERTEX_POINT('',#76080);
#22768=VERTEX_POINT('',#76084);
#22769=VERTEX_POINT('',#76088);
#22770=VERTEX_POINT('',#76092);
#22771=VERTEX_POINT('',#76096);
#22772=VERTEX_POINT('',#76100);
#22773=VERTEX_POINT('',#76104);
#22774=VERTEX_POINT('',#76108);
#22775=VERTEX_POINT('',#76112);
#22776=VERTEX_POINT('',#76119);
#22777=VERTEX_POINT('',#76121);
#22778=VERTEX_POINT('',#76123);
#22779=VERTEX_POINT('',#76125);
#22780=VERTEX_POINT('',#76127);
#22781=VERTEX_POINT('',#76129);
#22782=VERTEX_POINT('',#76131);
#22783=VERTEX_POINT('',#76133);
#22784=VERTEX_POINT('',#76135);
#22785=VERTEX_POINT('',#76137);
#22786=VERTEX_POINT('',#76139);
#22787=VERTEX_POINT('',#76141);
#22788=VERTEX_POINT('',#76143);
#22789=VERTEX_POINT('',#76145);
#22790=VERTEX_POINT('',#76179);
#22791=VERTEX_POINT('',#76183);
#22792=VERTEX_POINT('',#76187);
#22793=VERTEX_POINT('',#76191);
#22794=VERTEX_POINT('',#76195);
#22795=VERTEX_POINT('',#76199);
#22796=VERTEX_POINT('',#76203);
#22797=VERTEX_POINT('',#76207);
#22798=VERTEX_POINT('',#76211);
#22799=VERTEX_POINT('',#76215);
#22800=VERTEX_POINT('',#76219);
#22801=VERTEX_POINT('',#76223);
#22802=VERTEX_POINT('',#76230);
#22803=VERTEX_POINT('',#76232);
#22804=VERTEX_POINT('',#76234);
#22805=VERTEX_POINT('',#76236);
#22806=VERTEX_POINT('',#76238);
#22807=VERTEX_POINT('',#76240);
#22808=VERTEX_POINT('',#76242);
#22809=VERTEX_POINT('',#76244);
#22810=VERTEX_POINT('',#76246);
#22811=VERTEX_POINT('',#76248);
#22812=VERTEX_POINT('',#76250);
#22813=VERTEX_POINT('',#76252);
#22814=VERTEX_POINT('',#76254);
#22815=VERTEX_POINT('',#76256);
#22816=VERTEX_POINT('',#76290);
#22817=VERTEX_POINT('',#76294);
#22818=VERTEX_POINT('',#76298);
#22819=VERTEX_POINT('',#76302);
#22820=VERTEX_POINT('',#76306);
#22821=VERTEX_POINT('',#76310);
#22822=VERTEX_POINT('',#76314);
#22823=VERTEX_POINT('',#76318);
#22824=VERTEX_POINT('',#76322);
#22825=VERTEX_POINT('',#76326);
#22826=VERTEX_POINT('',#76330);
#22827=VERTEX_POINT('',#76334);
#22828=VERTEX_POINT('',#76341);
#22829=VERTEX_POINT('',#76343);
#22830=VERTEX_POINT('',#76345);
#22831=VERTEX_POINT('',#76347);
#22832=VERTEX_POINT('',#76349);
#22833=VERTEX_POINT('',#76351);
#22834=VERTEX_POINT('',#76353);
#22835=VERTEX_POINT('',#76355);
#22836=VERTEX_POINT('',#76357);
#22837=VERTEX_POINT('',#76359);
#22838=VERTEX_POINT('',#76361);
#22839=VERTEX_POINT('',#76363);
#22840=VERTEX_POINT('',#76365);
#22841=VERTEX_POINT('',#76367);
#22842=VERTEX_POINT('',#76401);
#22843=VERTEX_POINT('',#76405);
#22844=VERTEX_POINT('',#76409);
#22845=VERTEX_POINT('',#76413);
#22846=VERTEX_POINT('',#76417);
#22847=VERTEX_POINT('',#76421);
#22848=VERTEX_POINT('',#76425);
#22849=VERTEX_POINT('',#76429);
#22850=VERTEX_POINT('',#76433);
#22851=VERTEX_POINT('',#76437);
#22852=VERTEX_POINT('',#76441);
#22853=VERTEX_POINT('',#76445);
#22854=VERTEX_POINT('',#76452);
#22855=VERTEX_POINT('',#76454);
#22856=VERTEX_POINT('',#76456);
#22857=VERTEX_POINT('',#76458);
#22858=VERTEX_POINT('',#76460);
#22859=VERTEX_POINT('',#76462);
#22860=VERTEX_POINT('',#76464);
#22861=VERTEX_POINT('',#76466);
#22862=VERTEX_POINT('',#76468);
#22863=VERTEX_POINT('',#76470);
#22864=VERTEX_POINT('',#76472);
#22865=VERTEX_POINT('',#76474);
#22866=VERTEX_POINT('',#76476);
#22867=VERTEX_POINT('',#76478);
#22868=VERTEX_POINT('',#76512);
#22869=VERTEX_POINT('',#76516);
#22870=VERTEX_POINT('',#76520);
#22871=VERTEX_POINT('',#76524);
#22872=VERTEX_POINT('',#76528);
#22873=VERTEX_POINT('',#76532);
#22874=VERTEX_POINT('',#76536);
#22875=VERTEX_POINT('',#76540);
#22876=VERTEX_POINT('',#76544);
#22877=VERTEX_POINT('',#76548);
#22878=VERTEX_POINT('',#76552);
#22879=VERTEX_POINT('',#76556);
#22880=VERTEX_POINT('',#76563);
#22881=VERTEX_POINT('',#76565);
#22882=VERTEX_POINT('',#76567);
#22883=VERTEX_POINT('',#76569);
#22884=VERTEX_POINT('',#76571);
#22885=VERTEX_POINT('',#76573);
#22886=VERTEX_POINT('',#76575);
#22887=VERTEX_POINT('',#76577);
#22888=VERTEX_POINT('',#76579);
#22889=VERTEX_POINT('',#76581);
#22890=VERTEX_POINT('',#76583);
#22891=VERTEX_POINT('',#76585);
#22892=VERTEX_POINT('',#76587);
#22893=VERTEX_POINT('',#76589);
#22894=VERTEX_POINT('',#76623);
#22895=VERTEX_POINT('',#76627);
#22896=VERTEX_POINT('',#76631);
#22897=VERTEX_POINT('',#76635);
#22898=VERTEX_POINT('',#76639);
#22899=VERTEX_POINT('',#76643);
#22900=VERTEX_POINT('',#76647);
#22901=VERTEX_POINT('',#76651);
#22902=VERTEX_POINT('',#76655);
#22903=VERTEX_POINT('',#76659);
#22904=VERTEX_POINT('',#76663);
#22905=VERTEX_POINT('',#76667);
#22906=VERTEX_POINT('',#76674);
#22907=VERTEX_POINT('',#76676);
#22908=VERTEX_POINT('',#76678);
#22909=VERTEX_POINT('',#76680);
#22910=VERTEX_POINT('',#76682);
#22911=VERTEX_POINT('',#76684);
#22912=VERTEX_POINT('',#76686);
#22913=VERTEX_POINT('',#76688);
#22914=VERTEX_POINT('',#76690);
#22915=VERTEX_POINT('',#76692);
#22916=VERTEX_POINT('',#76694);
#22917=VERTEX_POINT('',#76696);
#22918=VERTEX_POINT('',#76698);
#22919=VERTEX_POINT('',#76700);
#22920=VERTEX_POINT('',#76734);
#22921=VERTEX_POINT('',#76738);
#22922=VERTEX_POINT('',#76742);
#22923=VERTEX_POINT('',#76746);
#22924=VERTEX_POINT('',#76750);
#22925=VERTEX_POINT('',#76754);
#22926=VERTEX_POINT('',#76758);
#22927=VERTEX_POINT('',#76762);
#22928=VERTEX_POINT('',#76766);
#22929=VERTEX_POINT('',#76770);
#22930=VERTEX_POINT('',#76774);
#22931=VERTEX_POINT('',#76778);
#22932=VERTEX_POINT('',#76785);
#22933=VERTEX_POINT('',#76787);
#22934=VERTEX_POINT('',#76789);
#22935=VERTEX_POINT('',#76791);
#22936=VERTEX_POINT('',#76793);
#22937=VERTEX_POINT('',#76795);
#22938=VERTEX_POINT('',#76797);
#22939=VERTEX_POINT('',#76799);
#22940=VERTEX_POINT('',#76801);
#22941=VERTEX_POINT('',#76803);
#22942=VERTEX_POINT('',#76805);
#22943=VERTEX_POINT('',#76807);
#22944=VERTEX_POINT('',#76809);
#22945=VERTEX_POINT('',#76811);
#22946=VERTEX_POINT('',#76845);
#22947=VERTEX_POINT('',#76849);
#22948=VERTEX_POINT('',#76853);
#22949=VERTEX_POINT('',#76857);
#22950=VERTEX_POINT('',#76861);
#22951=VERTEX_POINT('',#76865);
#22952=VERTEX_POINT('',#76869);
#22953=VERTEX_POINT('',#76873);
#22954=VERTEX_POINT('',#76877);
#22955=VERTEX_POINT('',#76881);
#22956=VERTEX_POINT('',#76885);
#22957=VERTEX_POINT('',#76889);
#22958=VERTEX_POINT('',#76896);
#22959=VERTEX_POINT('',#76898);
#22960=VERTEX_POINT('',#76900);
#22961=VERTEX_POINT('',#76902);
#22962=VERTEX_POINT('',#76904);
#22963=VERTEX_POINT('',#76906);
#22964=VERTEX_POINT('',#76908);
#22965=VERTEX_POINT('',#76910);
#22966=VERTEX_POINT('',#76912);
#22967=VERTEX_POINT('',#76914);
#22968=VERTEX_POINT('',#76916);
#22969=VERTEX_POINT('',#76918);
#22970=VERTEX_POINT('',#76920);
#22971=VERTEX_POINT('',#76922);
#22972=VERTEX_POINT('',#76956);
#22973=VERTEX_POINT('',#76960);
#22974=VERTEX_POINT('',#76964);
#22975=VERTEX_POINT('',#76968);
#22976=VERTEX_POINT('',#76972);
#22977=VERTEX_POINT('',#76976);
#22978=VERTEX_POINT('',#76980);
#22979=VERTEX_POINT('',#76984);
#22980=VERTEX_POINT('',#76988);
#22981=VERTEX_POINT('',#76992);
#22982=VERTEX_POINT('',#76996);
#22983=VERTEX_POINT('',#77000);
#22984=VERTEX_POINT('',#77007);
#22985=VERTEX_POINT('',#77009);
#22986=VERTEX_POINT('',#77011);
#22987=VERTEX_POINT('',#77013);
#22988=VERTEX_POINT('',#77015);
#22989=VERTEX_POINT('',#77017);
#22990=VERTEX_POINT('',#77019);
#22991=VERTEX_POINT('',#77021);
#22992=VERTEX_POINT('',#77023);
#22993=VERTEX_POINT('',#77025);
#22994=VERTEX_POINT('',#77027);
#22995=VERTEX_POINT('',#77029);
#22996=VERTEX_POINT('',#77031);
#22997=VERTEX_POINT('',#77033);
#22998=VERTEX_POINT('',#77067);
#22999=VERTEX_POINT('',#77071);
#23000=VERTEX_POINT('',#77075);
#23001=VERTEX_POINT('',#77079);
#23002=VERTEX_POINT('',#77083);
#23003=VERTEX_POINT('',#77087);
#23004=VERTEX_POINT('',#77091);
#23005=VERTEX_POINT('',#77095);
#23006=VERTEX_POINT('',#77099);
#23007=VERTEX_POINT('',#77103);
#23008=VERTEX_POINT('',#77107);
#23009=VERTEX_POINT('',#77111);
#23010=VERTEX_POINT('',#77118);
#23011=VERTEX_POINT('',#77120);
#23012=VERTEX_POINT('',#77122);
#23013=VERTEX_POINT('',#77124);
#23014=VERTEX_POINT('',#77126);
#23015=VERTEX_POINT('',#77128);
#23016=VERTEX_POINT('',#77130);
#23017=VERTEX_POINT('',#77132);
#23018=VERTEX_POINT('',#77134);
#23019=VERTEX_POINT('',#77136);
#23020=VERTEX_POINT('',#77138);
#23021=VERTEX_POINT('',#77140);
#23022=VERTEX_POINT('',#77142);
#23023=VERTEX_POINT('',#77144);
#23024=VERTEX_POINT('',#77178);
#23025=VERTEX_POINT('',#77182);
#23026=VERTEX_POINT('',#77186);
#23027=VERTEX_POINT('',#77190);
#23028=VERTEX_POINT('',#77194);
#23029=VERTEX_POINT('',#77198);
#23030=VERTEX_POINT('',#77202);
#23031=VERTEX_POINT('',#77206);
#23032=VERTEX_POINT('',#77210);
#23033=VERTEX_POINT('',#77214);
#23034=VERTEX_POINT('',#77218);
#23035=VERTEX_POINT('',#77222);
#23036=VERTEX_POINT('',#77229);
#23037=VERTEX_POINT('',#77231);
#23038=VERTEX_POINT('',#77233);
#23039=VERTEX_POINT('',#77235);
#23040=VERTEX_POINT('',#77237);
#23041=VERTEX_POINT('',#77239);
#23042=VERTEX_POINT('',#77241);
#23043=VERTEX_POINT('',#77243);
#23044=VERTEX_POINT('',#77245);
#23045=VERTEX_POINT('',#77247);
#23046=VERTEX_POINT('',#77249);
#23047=VERTEX_POINT('',#77251);
#23048=VERTEX_POINT('',#77253);
#23049=VERTEX_POINT('',#77255);
#23050=VERTEX_POINT('',#77259);
#23051=VERTEX_POINT('',#77263);
#23052=VERTEX_POINT('',#77267);
#23053=VERTEX_POINT('',#77271);
#23054=VERTEX_POINT('',#77275);
#23055=VERTEX_POINT('',#77279);
#23056=VERTEX_POINT('',#77283);
#23057=VERTEX_POINT('',#77287);
#23058=VERTEX_POINT('',#77291);
#23059=VERTEX_POINT('',#77295);
#23060=VERTEX_POINT('',#77299);
#23061=VERTEX_POINT('',#77303);
#23062=VERTEX_POINT('',#77307);
#23063=VERTEX_POINT('',#77344);
#23064=VERTEX_POINT('',#77348);
#23065=VERTEX_POINT('',#77350);
#23066=VERTEX_POINT('',#77352);
#23067=VERTEX_POINT('',#77356);
#23068=VERTEX_POINT('',#77358);
#23069=VERTEX_POINT('',#77363);
#23070=VERTEX_POINT('',#77365);
#23071=VERTEX_POINT('',#77369);
#23072=VERTEX_POINT('',#77373);
#23073=VERTEX_POINT('',#77374);
#23074=VERTEX_POINT('',#77376);
#23075=VERTEX_POINT('',#77381);
#23076=VERTEX_POINT('',#77383);
#23077=VERTEX_POINT('',#77387);
#23078=VERTEX_POINT('',#77390);
#23079=VERTEX_POINT('',#77394);
#23080=VERTEX_POINT('',#77398);
#23081=VERTEX_POINT('',#77401);
#23082=VERTEX_POINT('',#77405);
#23083=VERTEX_POINT('',#77411);
#25321=EDGE_CURVE('',#20324,#20325,#19574,.T.);
#25322=EDGE_CURVE('',#20326,#20324,#18698,.T.);
#25323=EDGE_CURVE('',#20327,#20326,#18699,.T.);
#25324=EDGE_CURVE('',#20325,#20327,#18700,.T.);
#25325=EDGE_CURVE('',#20328,#20329,#19575,.T.);
#25326=EDGE_CURVE('',#20330,#20328,#18701,.T.);
#25327=EDGE_CURVE('',#20331,#20330,#18702,.T.);
#25328=EDGE_CURVE('',#20329,#20331,#18703,.T.);
#25329=EDGE_CURVE('',#20332,#20333,#19576,.T.);
#25330=EDGE_CURVE('',#20334,#20332,#18704,.T.);
#25331=EDGE_CURVE('',#20335,#20334,#18705,.T.);
#25332=EDGE_CURVE('',#20333,#20335,#18706,.T.);
#25333=EDGE_CURVE('',#20336,#20337,#19577,.T.);
#25334=EDGE_CURVE('',#20338,#20336,#18707,.T.);
#25335=EDGE_CURVE('',#20339,#20338,#18708,.T.);
#25336=EDGE_CURVE('',#20337,#20339,#18709,.T.);
#25337=EDGE_CURVE('',#20340,#20341,#19578,.T.);
#25338=EDGE_CURVE('',#20342,#20340,#18710,.T.);
#25339=EDGE_CURVE('',#20343,#20342,#18711,.T.);
#25340=EDGE_CURVE('',#20341,#20343,#18712,.T.);
#25341=EDGE_CURVE('',#20344,#20345,#19579,.T.);
#25342=EDGE_CURVE('',#20346,#20344,#18713,.T.);
#25343=EDGE_CURVE('',#20347,#20346,#18714,.T.);
#25344=EDGE_CURVE('',#20345,#20347,#18715,.T.);
#25345=EDGE_CURVE('',#20348,#20349,#19580,.T.);
#25346=EDGE_CURVE('',#20350,#20348,#18716,.T.);
#25347=EDGE_CURVE('',#20351,#20350,#18717,.T.);
#25348=EDGE_CURVE('',#20349,#20351,#18718,.T.);
#25349=EDGE_CURVE('',#20352,#20353,#19581,.T.);
#25350=EDGE_CURVE('',#20354,#20352,#18719,.T.);
#25351=EDGE_CURVE('',#20355,#20354,#18720,.T.);
#25352=EDGE_CURVE('',#20353,#20355,#18721,.T.);
#25353=EDGE_CURVE('',#20356,#20357,#19582,.T.);
#25354=EDGE_CURVE('',#20358,#20356,#18722,.T.);
#25355=EDGE_CURVE('',#20359,#20358,#18723,.T.);
#25356=EDGE_CURVE('',#20357,#20359,#18724,.T.);
#25357=EDGE_CURVE('',#20360,#20361,#19583,.T.);
#25358=EDGE_CURVE('',#20362,#20360,#18725,.T.);
#25359=EDGE_CURVE('',#20363,#20362,#18726,.T.);
#25360=EDGE_CURVE('',#20361,#20363,#18727,.T.);
#25361=EDGE_CURVE('',#20364,#20365,#19584,.T.);
#25362=EDGE_CURVE('',#20366,#20364,#18728,.T.);
#25363=EDGE_CURVE('',#20367,#20366,#18729,.T.);
#25364=EDGE_CURVE('',#20365,#20367,#18730,.T.);
#25365=EDGE_CURVE('',#20368,#20369,#19585,.T.);
#25366=EDGE_CURVE('',#20370,#20368,#18731,.T.);
#25367=EDGE_CURVE('',#20371,#20370,#18732,.T.);
#25368=EDGE_CURVE('',#20369,#20371,#18733,.T.);
#25369=EDGE_CURVE('',#20372,#20373,#19586,.T.);
#25370=EDGE_CURVE('',#20374,#20372,#18734,.T.);
#25371=EDGE_CURVE('',#20375,#20374,#18735,.T.);
#25372=EDGE_CURVE('',#20373,#20375,#18736,.T.);
#25373=EDGE_CURVE('',#20376,#20377,#19587,.T.);
#25374=EDGE_CURVE('',#20378,#20376,#18737,.T.);
#25375=EDGE_CURVE('',#20379,#20378,#18738,.T.);
#25376=EDGE_CURVE('',#20377,#20379,#18739,.T.);
#25377=EDGE_CURVE('',#20380,#20381,#19588,.T.);
#25378=EDGE_CURVE('',#20382,#20380,#18740,.T.);
#25379=EDGE_CURVE('',#20383,#20382,#18741,.T.);
#25380=EDGE_CURVE('',#20381,#20383,#18742,.T.);
#25381=EDGE_CURVE('',#20384,#20385,#19589,.T.);
#25382=EDGE_CURVE('',#20386,#20384,#18743,.T.);
#25383=EDGE_CURVE('',#20387,#20386,#18744,.T.);
#25384=EDGE_CURVE('',#20385,#20387,#18745,.T.);
#25385=EDGE_CURVE('',#20388,#20389,#19590,.T.);
#25386=EDGE_CURVE('',#20390,#20388,#18746,.T.);
#25387=EDGE_CURVE('',#20391,#20390,#18747,.T.);
#25388=EDGE_CURVE('',#20389,#20391,#18748,.T.);
#25389=EDGE_CURVE('',#20392,#20393,#19591,.T.);
#25390=EDGE_CURVE('',#20394,#20392,#18749,.T.);
#25391=EDGE_CURVE('',#20395,#20394,#18750,.T.);
#25392=EDGE_CURVE('',#20393,#20395,#18751,.T.);
#25393=EDGE_CURVE('',#20396,#20397,#19592,.T.);
#25394=EDGE_CURVE('',#20398,#20396,#18752,.T.);
#25395=EDGE_CURVE('',#20399,#20398,#18753,.T.);
#25396=EDGE_CURVE('',#20397,#20399,#18754,.T.);
#25397=EDGE_CURVE('',#20400,#20401,#19593,.T.);
#25398=EDGE_CURVE('',#20402,#20400,#18755,.T.);
#25399=EDGE_CURVE('',#20403,#20402,#18756,.T.);
#25400=EDGE_CURVE('',#20401,#20403,#18757,.T.);
#25401=EDGE_CURVE('',#20404,#20405,#19594,.T.);
#25402=EDGE_CURVE('',#20406,#20404,#18758,.T.);
#25403=EDGE_CURVE('',#20407,#20406,#18759,.T.);
#25404=EDGE_CURVE('',#20405,#20407,#18760,.T.);
#25405=EDGE_CURVE('',#20408,#20409,#19595,.T.);
#25406=EDGE_CURVE('',#20410,#20408,#18761,.T.);
#25407=EDGE_CURVE('',#20411,#20410,#18762,.T.);
#25408=EDGE_CURVE('',#20409,#20411,#18763,.T.);
#25409=EDGE_CURVE('',#20412,#20413,#19596,.T.);
#25410=EDGE_CURVE('',#20414,#20412,#18764,.T.);
#25411=EDGE_CURVE('',#20415,#20414,#18765,.T.);
#25412=EDGE_CURVE('',#20413,#20415,#18766,.T.);
#25413=EDGE_CURVE('',#20416,#20417,#19597,.T.);
#25414=EDGE_CURVE('',#20418,#20416,#18767,.T.);
#25415=EDGE_CURVE('',#20419,#20418,#18768,.T.);
#25416=EDGE_CURVE('',#20417,#20419,#18769,.T.);
#25417=EDGE_CURVE('',#20420,#20421,#19598,.T.);
#25418=EDGE_CURVE('',#20422,#20420,#18770,.T.);
#25419=EDGE_CURVE('',#20423,#20422,#18771,.T.);
#25420=EDGE_CURVE('',#20421,#20423,#18772,.T.);
#25421=EDGE_CURVE('',#20424,#20425,#19599,.T.);
#25422=EDGE_CURVE('',#20426,#20424,#18773,.T.);
#25423=EDGE_CURVE('',#20427,#20426,#18774,.T.);
#25424=EDGE_CURVE('',#20425,#20427,#18775,.T.);
#25425=EDGE_CURVE('',#20428,#20429,#19600,.T.);
#25426=EDGE_CURVE('',#20430,#20428,#18776,.T.);
#25427=EDGE_CURVE('',#20431,#20430,#18777,.T.);
#25428=EDGE_CURVE('',#20429,#20431,#18778,.T.);
#25429=EDGE_CURVE('',#20432,#20433,#19601,.T.);
#25430=EDGE_CURVE('',#20434,#20432,#18779,.T.);
#25431=EDGE_CURVE('',#20435,#20434,#18780,.T.);
#25432=EDGE_CURVE('',#20433,#20435,#18781,.T.);
#25433=EDGE_CURVE('',#20436,#20437,#19602,.T.);
#25434=EDGE_CURVE('',#20438,#20436,#18782,.T.);
#25435=EDGE_CURVE('',#20439,#20438,#18783,.T.);
#25436=EDGE_CURVE('',#20437,#20439,#18784,.T.);
#25437=EDGE_CURVE('',#20440,#20441,#19603,.T.);
#25438=EDGE_CURVE('',#20442,#20440,#18785,.T.);
#25439=EDGE_CURVE('',#20443,#20442,#18786,.T.);
#25440=EDGE_CURVE('',#20441,#20443,#18787,.T.);
#25441=EDGE_CURVE('',#20444,#20445,#19604,.T.);
#25442=EDGE_CURVE('',#20446,#20444,#18788,.T.);
#25443=EDGE_CURVE('',#20447,#20446,#18789,.T.);
#25444=EDGE_CURVE('',#20445,#20447,#18790,.T.);
#25445=EDGE_CURVE('',#20448,#20449,#19605,.T.);
#25446=EDGE_CURVE('',#20450,#20448,#18791,.T.);
#25447=EDGE_CURVE('',#20451,#20450,#18792,.T.);
#25448=EDGE_CURVE('',#20449,#20451,#18793,.T.);
#25449=EDGE_CURVE('',#20452,#20453,#19606,.T.);
#25450=EDGE_CURVE('',#20454,#20452,#18794,.T.);
#25451=EDGE_CURVE('',#20455,#20454,#18795,.T.);
#25452=EDGE_CURVE('',#20453,#20455,#18796,.T.);
#25453=EDGE_CURVE('',#20456,#20457,#19607,.T.);
#25454=EDGE_CURVE('',#20458,#20456,#18797,.T.);
#25455=EDGE_CURVE('',#20459,#20458,#18798,.T.);
#25456=EDGE_CURVE('',#20457,#20459,#18799,.T.);
#25457=EDGE_CURVE('',#20460,#20461,#19608,.T.);
#25458=EDGE_CURVE('',#20462,#20460,#18800,.T.);
#25459=EDGE_CURVE('',#20463,#20462,#18801,.T.);
#25460=EDGE_CURVE('',#20461,#20463,#18802,.T.);
#25461=EDGE_CURVE('',#20464,#20465,#19609,.T.);
#25462=EDGE_CURVE('',#20466,#20464,#18803,.T.);
#25463=EDGE_CURVE('',#20467,#20466,#18804,.T.);
#25464=EDGE_CURVE('',#20465,#20467,#18805,.T.);
#25465=EDGE_CURVE('',#20468,#20466,#2160,.T.);
#25466=EDGE_CURVE('',#20469,#20468,#2161,.T.);
#25467=EDGE_CURVE('',#20470,#20469,#2162,.T.);
#25468=EDGE_CURVE('',#20471,#20470,#2163,.T.);
#25469=EDGE_CURVE('',#20472,#20471,#2164,.T.);
#25470=EDGE_CURVE('',#20473,#20472,#2165,.T.);
#25471=EDGE_CURVE('',#20474,#20473,#2166,.T.);
#25472=EDGE_CURVE('',#20475,#20474,#2167,.T.);
#25473=EDGE_CURVE('',#20476,#20475,#2168,.T.);
#25474=EDGE_CURVE('',#20477,#20476,#2169,.T.);
#25475=EDGE_CURVE('',#20478,#20477,#2170,.T.);
#25476=EDGE_CURVE('',#20479,#20478,#2171,.T.);
#25477=EDGE_CURVE('',#20480,#20479,#2172,.T.);
#25478=EDGE_CURVE('',#20481,#20480,#2173,.T.);
#25479=EDGE_CURVE('',#20482,#20481,#2174,.T.);
#25480=EDGE_CURVE('',#20482,#20483,#18806,.T.);
#25481=EDGE_CURVE('',#20484,#20483,#2175,.T.);
#25482=EDGE_CURVE('',#20485,#20484,#2176,.T.);
#25483=EDGE_CURVE('',#20486,#20485,#2177,.T.);
#25484=EDGE_CURVE('',#20487,#20486,#2178,.T.);
#25485=EDGE_CURVE('',#20488,#20487,#2179,.T.);
#25486=EDGE_CURVE('',#20489,#20488,#2180,.T.);
#25487=EDGE_CURVE('',#20490,#20489,#2181,.T.);
#25488=EDGE_CURVE('',#20491,#20490,#2182,.T.);
#25489=EDGE_CURVE('',#20492,#20491,#2183,.T.);
#25490=EDGE_CURVE('',#20493,#20492,#2184,.T.);
#25491=EDGE_CURVE('',#20494,#20493,#2185,.T.);
#25492=EDGE_CURVE('',#20495,#20494,#2186,.T.);
#25493=EDGE_CURVE('',#20496,#20495,#2187,.T.);
#25494=EDGE_CURVE('',#20497,#20496,#2188,.T.);
#25495=EDGE_CURVE('',#20467,#20497,#2189,.T.);
#25496=EDGE_CURVE('',#20464,#20498,#2190,.T.);
#25497=EDGE_CURVE('',#20498,#20499,#2191,.T.);
#25498=EDGE_CURVE('',#20500,#20499,#18807,.T.);
#25499=EDGE_CURVE('',#20501,#20500,#1288,.T.);
#25500=EDGE_CURVE('',#20468,#20501,#2192,.T.);
#25501=EDGE_CURVE('',#20502,#20462,#2193,.T.);
#25502=EDGE_CURVE('',#20503,#20502,#2194,.T.);
#25503=EDGE_CURVE('',#20504,#20503,#2195,.T.);
#25504=EDGE_CURVE('',#20505,#20504,#2196,.T.);
#25505=EDGE_CURVE('',#20506,#20505,#2197,.T.);
#25506=EDGE_CURVE('',#20507,#20506,#2198,.T.);
#25507=EDGE_CURVE('',#20508,#20507,#2199,.T.);
#25508=EDGE_CURVE('',#20509,#20508,#2200,.T.);
#25509=EDGE_CURVE('',#20510,#20509,#2201,.T.);
#25510=EDGE_CURVE('',#20511,#20510,#2202,.T.);
#25511=EDGE_CURVE('',#20512,#20511,#2203,.T.);
#25512=EDGE_CURVE('',#20513,#20512,#2204,.T.);
#25513=EDGE_CURVE('',#20514,#20513,#2205,.T.);
#25514=EDGE_CURVE('',#20515,#20514,#2206,.T.);
#25515=EDGE_CURVE('',#20516,#20515,#2207,.T.);
#25516=EDGE_CURVE('',#20516,#20517,#18808,.T.);
#25517=EDGE_CURVE('',#20518,#20517,#2208,.T.);
#25518=EDGE_CURVE('',#20519,#20518,#2209,.T.);
#25519=EDGE_CURVE('',#20520,#20519,#2210,.T.);
#25520=EDGE_CURVE('',#20521,#20520,#2211,.T.);
#25521=EDGE_CURVE('',#20522,#20521,#2212,.T.);
#25522=EDGE_CURVE('',#20523,#20522,#2213,.T.);
#25523=EDGE_CURVE('',#20524,#20523,#2214,.T.);
#25524=EDGE_CURVE('',#20525,#20524,#2215,.T.);
#25525=EDGE_CURVE('',#20526,#20525,#2216,.T.);
#25526=EDGE_CURVE('',#20527,#20526,#2217,.T.);
#25527=EDGE_CURVE('',#20528,#20527,#2218,.T.);
#25528=EDGE_CURVE('',#20529,#20528,#2219,.T.);
#25529=EDGE_CURVE('',#20530,#20529,#2220,.T.);
#25530=EDGE_CURVE('',#20531,#20530,#2221,.T.);
#25531=EDGE_CURVE('',#20463,#20531,#2222,.T.);
#25532=EDGE_CURVE('',#20460,#20532,#2223,.T.);
#25533=EDGE_CURVE('',#20532,#20533,#2224,.T.);
#25534=EDGE_CURVE('',#20534,#20533,#18809,.T.);
#25535=EDGE_CURVE('',#20535,#20534,#1289,.T.);
#25536=EDGE_CURVE('',#20502,#20535,#2225,.T.);
#25537=EDGE_CURVE('',#20536,#20458,#2226,.T.);
#25538=EDGE_CURVE('',#20537,#20536,#2227,.T.);
#25539=EDGE_CURVE('',#20538,#20537,#2228,.T.);
#25540=EDGE_CURVE('',#20539,#20538,#2229,.T.);
#25541=EDGE_CURVE('',#20540,#20539,#2230,.T.);
#25542=EDGE_CURVE('',#20541,#20540,#2231,.T.);
#25543=EDGE_CURVE('',#20542,#20541,#2232,.T.);
#25544=EDGE_CURVE('',#20543,#20542,#2233,.T.);
#25545=EDGE_CURVE('',#20544,#20543,#2234,.T.);
#25546=EDGE_CURVE('',#20545,#20544,#2235,.T.);
#25547=EDGE_CURVE('',#20546,#20545,#2236,.T.);
#25548=EDGE_CURVE('',#20547,#20546,#2237,.T.);
#25549=EDGE_CURVE('',#20548,#20547,#2238,.T.);
#25550=EDGE_CURVE('',#20549,#20548,#2239,.T.);
#25551=EDGE_CURVE('',#20550,#20549,#2240,.T.);
#25552=EDGE_CURVE('',#20550,#20551,#18810,.T.);
#25553=EDGE_CURVE('',#20552,#20551,#2241,.T.);
#25554=EDGE_CURVE('',#20553,#20552,#2242,.T.);
#25555=EDGE_CURVE('',#20554,#20553,#2243,.T.);
#25556=EDGE_CURVE('',#20555,#20554,#2244,.T.);
#25557=EDGE_CURVE('',#20556,#20555,#2245,.T.);
#25558=EDGE_CURVE('',#20557,#20556,#2246,.T.);
#25559=EDGE_CURVE('',#20558,#20557,#2247,.T.);
#25560=EDGE_CURVE('',#20559,#20558,#2248,.T.);
#25561=EDGE_CURVE('',#20560,#20559,#2249,.T.);
#25562=EDGE_CURVE('',#20561,#20560,#2250,.T.);
#25563=EDGE_CURVE('',#20562,#20561,#2251,.T.);
#25564=EDGE_CURVE('',#20563,#20562,#2252,.T.);
#25565=EDGE_CURVE('',#20564,#20563,#2253,.T.);
#25566=EDGE_CURVE('',#20565,#20564,#2254,.T.);
#25567=EDGE_CURVE('',#20459,#20565,#2255,.T.);
#25568=EDGE_CURVE('',#20456,#20566,#2256,.T.);
#25569=EDGE_CURVE('',#20566,#20567,#2257,.T.);
#25570=EDGE_CURVE('',#20568,#20567,#18811,.T.);
#25571=EDGE_CURVE('',#20569,#20568,#1290,.T.);
#25572=EDGE_CURVE('',#20536,#20569,#2258,.T.);
#25573=EDGE_CURVE('',#20570,#20454,#2259,.T.);
#25574=EDGE_CURVE('',#20571,#20570,#2260,.T.);
#25575=EDGE_CURVE('',#20572,#20571,#2261,.T.);
#25576=EDGE_CURVE('',#20573,#20572,#2262,.T.);
#25577=EDGE_CURVE('',#20574,#20573,#2263,.T.);
#25578=EDGE_CURVE('',#20575,#20574,#2264,.T.);
#25579=EDGE_CURVE('',#20576,#20575,#2265,.T.);
#25580=EDGE_CURVE('',#20577,#20576,#2266,.T.);
#25581=EDGE_CURVE('',#20578,#20577,#2267,.T.);
#25582=EDGE_CURVE('',#20579,#20578,#2268,.T.);
#25583=EDGE_CURVE('',#20580,#20579,#2269,.T.);
#25584=EDGE_CURVE('',#20581,#20580,#2270,.T.);
#25585=EDGE_CURVE('',#20582,#20581,#2271,.T.);
#25586=EDGE_CURVE('',#20583,#20582,#2272,.T.);
#25587=EDGE_CURVE('',#20584,#20583,#2273,.T.);
#25588=EDGE_CURVE('',#20584,#20585,#18812,.T.);
#25589=EDGE_CURVE('',#20586,#20585,#2274,.T.);
#25590=EDGE_CURVE('',#20587,#20586,#2275,.T.);
#25591=EDGE_CURVE('',#20588,#20587,#2276,.T.);
#25592=EDGE_CURVE('',#20589,#20588,#2277,.T.);
#25593=EDGE_CURVE('',#20590,#20589,#2278,.T.);
#25594=EDGE_CURVE('',#20591,#20590,#2279,.T.);
#25595=EDGE_CURVE('',#20592,#20591,#2280,.T.);
#25596=EDGE_CURVE('',#20593,#20592,#2281,.T.);
#25597=EDGE_CURVE('',#20594,#20593,#2282,.T.);
#25598=EDGE_CURVE('',#20595,#20594,#2283,.T.);
#25599=EDGE_CURVE('',#20596,#20595,#2284,.T.);
#25600=EDGE_CURVE('',#20597,#20596,#2285,.T.);
#25601=EDGE_CURVE('',#20598,#20597,#2286,.T.);
#25602=EDGE_CURVE('',#20599,#20598,#2287,.T.);
#25603=EDGE_CURVE('',#20455,#20599,#2288,.T.);
#25604=EDGE_CURVE('',#20452,#20600,#2289,.T.);
#25605=EDGE_CURVE('',#20600,#20601,#2290,.T.);
#25606=EDGE_CURVE('',#20602,#20601,#18813,.T.);
#25607=EDGE_CURVE('',#20603,#20602,#1291,.T.);
#25608=EDGE_CURVE('',#20570,#20603,#2291,.T.);
#25609=EDGE_CURVE('',#20604,#20450,#2292,.T.);
#25610=EDGE_CURVE('',#20605,#20604,#2293,.T.);
#25611=EDGE_CURVE('',#20606,#20605,#2294,.T.);
#25612=EDGE_CURVE('',#20607,#20606,#2295,.T.);
#25613=EDGE_CURVE('',#20608,#20607,#2296,.T.);
#25614=EDGE_CURVE('',#20609,#20608,#2297,.T.);
#25615=EDGE_CURVE('',#20610,#20609,#2298,.T.);
#25616=EDGE_CURVE('',#20611,#20610,#2299,.T.);
#25617=EDGE_CURVE('',#20612,#20611,#2300,.T.);
#25618=EDGE_CURVE('',#20613,#20612,#2301,.T.);
#25619=EDGE_CURVE('',#20614,#20613,#2302,.T.);
#25620=EDGE_CURVE('',#20615,#20614,#2303,.T.);
#25621=EDGE_CURVE('',#20616,#20615,#2304,.T.);
#25622=EDGE_CURVE('',#20617,#20616,#2305,.T.);
#25623=EDGE_CURVE('',#20618,#20617,#2306,.T.);
#25624=EDGE_CURVE('',#20618,#20619,#18814,.T.);
#25625=EDGE_CURVE('',#20620,#20619,#2307,.T.);
#25626=EDGE_CURVE('',#20621,#20620,#2308,.T.);
#25627=EDGE_CURVE('',#20622,#20621,#2309,.T.);
#25628=EDGE_CURVE('',#20623,#20622,#2310,.T.);
#25629=EDGE_CURVE('',#20624,#20623,#2311,.T.);
#25630=EDGE_CURVE('',#20625,#20624,#2312,.T.);
#25631=EDGE_CURVE('',#20626,#20625,#2313,.T.);
#25632=EDGE_CURVE('',#20627,#20626,#2314,.T.);
#25633=EDGE_CURVE('',#20628,#20627,#2315,.T.);
#25634=EDGE_CURVE('',#20629,#20628,#2316,.T.);
#25635=EDGE_CURVE('',#20630,#20629,#2317,.T.);
#25636=EDGE_CURVE('',#20631,#20630,#2318,.T.);
#25637=EDGE_CURVE('',#20632,#20631,#2319,.T.);
#25638=EDGE_CURVE('',#20633,#20632,#2320,.T.);
#25639=EDGE_CURVE('',#20451,#20633,#2321,.T.);
#25640=EDGE_CURVE('',#20448,#20634,#2322,.T.);
#25641=EDGE_CURVE('',#20634,#20635,#2323,.T.);
#25642=EDGE_CURVE('',#20636,#20635,#18815,.T.);
#25643=EDGE_CURVE('',#20637,#20636,#1292,.T.);
#25644=EDGE_CURVE('',#20604,#20637,#2324,.T.);
#25645=EDGE_CURVE('',#20638,#20446,#2325,.T.);
#25646=EDGE_CURVE('',#20639,#20638,#2326,.T.);
#25647=EDGE_CURVE('',#20640,#20639,#2327,.T.);
#25648=EDGE_CURVE('',#20641,#20640,#2328,.T.);
#25649=EDGE_CURVE('',#20642,#20641,#2329,.T.);
#25650=EDGE_CURVE('',#20643,#20642,#2330,.T.);
#25651=EDGE_CURVE('',#20644,#20643,#2331,.T.);
#25652=EDGE_CURVE('',#20645,#20644,#2332,.T.);
#25653=EDGE_CURVE('',#20646,#20645,#2333,.T.);
#25654=EDGE_CURVE('',#20647,#20646,#2334,.T.);
#25655=EDGE_CURVE('',#20648,#20647,#2335,.T.);
#25656=EDGE_CURVE('',#20649,#20648,#2336,.T.);
#25657=EDGE_CURVE('',#20650,#20649,#2337,.T.);
#25658=EDGE_CURVE('',#20651,#20650,#2338,.T.);
#25659=EDGE_CURVE('',#20652,#20651,#2339,.T.);
#25660=EDGE_CURVE('',#20652,#20653,#18816,.T.);
#25661=EDGE_CURVE('',#20654,#20653,#2340,.T.);
#25662=EDGE_CURVE('',#20655,#20654,#2341,.T.);
#25663=EDGE_CURVE('',#20656,#20655,#2342,.T.);
#25664=EDGE_CURVE('',#20657,#20656,#2343,.T.);
#25665=EDGE_CURVE('',#20658,#20657,#2344,.T.);
#25666=EDGE_CURVE('',#20659,#20658,#2345,.T.);
#25667=EDGE_CURVE('',#20660,#20659,#2346,.T.);
#25668=EDGE_CURVE('',#20661,#20660,#2347,.T.);
#25669=EDGE_CURVE('',#20662,#20661,#2348,.T.);
#25670=EDGE_CURVE('',#20663,#20662,#2349,.T.);
#25671=EDGE_CURVE('',#20664,#20663,#2350,.T.);
#25672=EDGE_CURVE('',#20665,#20664,#2351,.T.);
#25673=EDGE_CURVE('',#20666,#20665,#2352,.T.);
#25674=EDGE_CURVE('',#20667,#20666,#2353,.T.);
#25675=EDGE_CURVE('',#20447,#20667,#2354,.T.);
#25676=EDGE_CURVE('',#20444,#20668,#2355,.T.);
#25677=EDGE_CURVE('',#20668,#20669,#2356,.T.);
#25678=EDGE_CURVE('',#20670,#20669,#18817,.T.);
#25679=EDGE_CURVE('',#20671,#20670,#1293,.T.);
#25680=EDGE_CURVE('',#20638,#20671,#2357,.T.);
#25681=EDGE_CURVE('',#20672,#20442,#2358,.T.);
#25682=EDGE_CURVE('',#20673,#20672,#2359,.T.);
#25683=EDGE_CURVE('',#20674,#20673,#2360,.T.);
#25684=EDGE_CURVE('',#20675,#20674,#2361,.T.);
#25685=EDGE_CURVE('',#20676,#20675,#2362,.T.);
#25686=EDGE_CURVE('',#20677,#20676,#2363,.T.);
#25687=EDGE_CURVE('',#20678,#20677,#2364,.T.);
#25688=EDGE_CURVE('',#20679,#20678,#2365,.T.);
#25689=EDGE_CURVE('',#20680,#20679,#2366,.T.);
#25690=EDGE_CURVE('',#20681,#20680,#2367,.T.);
#25691=EDGE_CURVE('',#20682,#20681,#2368,.T.);
#25692=EDGE_CURVE('',#20683,#20682,#2369,.T.);
#25693=EDGE_CURVE('',#20684,#20683,#2370,.T.);
#25694=EDGE_CURVE('',#20685,#20684,#2371,.T.);
#25695=EDGE_CURVE('',#20686,#20685,#2372,.T.);
#25696=EDGE_CURVE('',#20686,#20687,#18818,.T.);
#25697=EDGE_CURVE('',#20688,#20687,#2373,.T.);
#25698=EDGE_CURVE('',#20689,#20688,#2374,.T.);
#25699=EDGE_CURVE('',#20690,#20689,#2375,.T.);
#25700=EDGE_CURVE('',#20691,#20690,#2376,.T.);
#25701=EDGE_CURVE('',#20692,#20691,#2377,.T.);
#25702=EDGE_CURVE('',#20693,#20692,#2378,.T.);
#25703=EDGE_CURVE('',#20694,#20693,#2379,.T.);
#25704=EDGE_CURVE('',#20695,#20694,#2380,.T.);
#25705=EDGE_CURVE('',#20696,#20695,#2381,.T.);
#25706=EDGE_CURVE('',#20697,#20696,#2382,.T.);
#25707=EDGE_CURVE('',#20698,#20697,#2383,.T.);
#25708=EDGE_CURVE('',#20699,#20698,#2384,.T.);
#25709=EDGE_CURVE('',#20700,#20699,#2385,.T.);
#25710=EDGE_CURVE('',#20701,#20700,#2386,.T.);
#25711=EDGE_CURVE('',#20443,#20701,#2387,.T.);
#25712=EDGE_CURVE('',#20440,#20702,#2388,.T.);
#25713=EDGE_CURVE('',#20702,#20703,#2389,.T.);
#25714=EDGE_CURVE('',#20704,#20703,#18819,.T.);
#25715=EDGE_CURVE('',#20705,#20704,#1294,.T.);
#25716=EDGE_CURVE('',#20672,#20705,#2390,.T.);
#25717=EDGE_CURVE('',#20706,#20438,#2391,.T.);
#25718=EDGE_CURVE('',#20707,#20706,#2392,.T.);
#25719=EDGE_CURVE('',#20708,#20707,#2393,.T.);
#25720=EDGE_CURVE('',#20709,#20708,#2394,.T.);
#25721=EDGE_CURVE('',#20710,#20709,#2395,.T.);
#25722=EDGE_CURVE('',#20711,#20710,#2396,.T.);
#25723=EDGE_CURVE('',#20712,#20711,#2397,.T.);
#25724=EDGE_CURVE('',#20713,#20712,#2398,.T.);
#25725=EDGE_CURVE('',#20714,#20713,#2399,.T.);
#25726=EDGE_CURVE('',#20715,#20714,#2400,.T.);
#25727=EDGE_CURVE('',#20716,#20715,#2401,.T.);
#25728=EDGE_CURVE('',#20717,#20716,#2402,.T.);
#25729=EDGE_CURVE('',#20718,#20717,#2403,.T.);
#25730=EDGE_CURVE('',#20719,#20718,#2404,.T.);
#25731=EDGE_CURVE('',#20720,#20719,#2405,.T.);
#25732=EDGE_CURVE('',#20720,#20721,#18820,.T.);
#25733=EDGE_CURVE('',#20722,#20721,#2406,.T.);
#25734=EDGE_CURVE('',#20723,#20722,#2407,.T.);
#25735=EDGE_CURVE('',#20724,#20723,#2408,.T.);
#25736=EDGE_CURVE('',#20725,#20724,#2409,.T.);
#25737=EDGE_CURVE('',#20726,#20725,#2410,.T.);
#25738=EDGE_CURVE('',#20727,#20726,#2411,.T.);
#25739=EDGE_CURVE('',#20728,#20727,#2412,.T.);
#25740=EDGE_CURVE('',#20729,#20728,#2413,.T.);
#25741=EDGE_CURVE('',#20730,#20729,#2414,.T.);
#25742=EDGE_CURVE('',#20731,#20730,#2415,.T.);
#25743=EDGE_CURVE('',#20732,#20731,#2416,.T.);
#25744=EDGE_CURVE('',#20733,#20732,#2417,.T.);
#25745=EDGE_CURVE('',#20734,#20733,#2418,.T.);
#25746=EDGE_CURVE('',#20735,#20734,#2419,.T.);
#25747=EDGE_CURVE('',#20439,#20735,#2420,.T.);
#25748=EDGE_CURVE('',#20436,#20736,#2421,.T.);
#25749=EDGE_CURVE('',#20736,#20737,#2422,.T.);
#25750=EDGE_CURVE('',#20738,#20737,#18821,.T.);
#25751=EDGE_CURVE('',#20739,#20738,#1295,.T.);
#25752=EDGE_CURVE('',#20706,#20739,#2423,.T.);
#25753=EDGE_CURVE('',#20740,#20434,#2424,.T.);
#25754=EDGE_CURVE('',#20741,#20740,#2425,.T.);
#25755=EDGE_CURVE('',#20742,#20741,#2426,.T.);
#25756=EDGE_CURVE('',#20743,#20742,#2427,.T.);
#25757=EDGE_CURVE('',#20744,#20743,#2428,.T.);
#25758=EDGE_CURVE('',#20745,#20744,#2429,.T.);
#25759=EDGE_CURVE('',#20746,#20745,#2430,.T.);
#25760=EDGE_CURVE('',#20747,#20746,#2431,.T.);
#25761=EDGE_CURVE('',#20748,#20747,#2432,.T.);
#25762=EDGE_CURVE('',#20749,#20748,#2433,.T.);
#25763=EDGE_CURVE('',#20750,#20749,#2434,.T.);
#25764=EDGE_CURVE('',#20751,#20750,#2435,.T.);
#25765=EDGE_CURVE('',#20752,#20751,#2436,.T.);
#25766=EDGE_CURVE('',#20753,#20752,#2437,.T.);
#25767=EDGE_CURVE('',#20754,#20753,#2438,.T.);
#25768=EDGE_CURVE('',#20754,#20755,#18822,.T.);
#25769=EDGE_CURVE('',#20756,#20755,#2439,.T.);
#25770=EDGE_CURVE('',#20757,#20756,#2440,.T.);
#25771=EDGE_CURVE('',#20758,#20757,#2441,.T.);
#25772=EDGE_CURVE('',#20759,#20758,#2442,.T.);
#25773=EDGE_CURVE('',#20760,#20759,#2443,.T.);
#25774=EDGE_CURVE('',#20761,#20760,#2444,.T.);
#25775=EDGE_CURVE('',#20762,#20761,#2445,.T.);
#25776=EDGE_CURVE('',#20763,#20762,#2446,.T.);
#25777=EDGE_CURVE('',#20764,#20763,#2447,.T.);
#25778=EDGE_CURVE('',#20765,#20764,#2448,.T.);
#25779=EDGE_CURVE('',#20766,#20765,#2449,.T.);
#25780=EDGE_CURVE('',#20767,#20766,#2450,.T.);
#25781=EDGE_CURVE('',#20768,#20767,#2451,.T.);
#25782=EDGE_CURVE('',#20769,#20768,#2452,.T.);
#25783=EDGE_CURVE('',#20435,#20769,#2453,.T.);
#25784=EDGE_CURVE('',#20432,#20770,#2454,.T.);
#25785=EDGE_CURVE('',#20770,#20771,#2455,.T.);
#25786=EDGE_CURVE('',#20772,#20771,#18823,.T.);
#25787=EDGE_CURVE('',#20773,#20772,#1296,.T.);
#25788=EDGE_CURVE('',#20740,#20773,#2456,.T.);
#25789=EDGE_CURVE('',#20774,#20430,#2457,.T.);
#25790=EDGE_CURVE('',#20775,#20774,#2458,.T.);
#25791=EDGE_CURVE('',#20776,#20775,#2459,.T.);
#25792=EDGE_CURVE('',#20777,#20776,#2460,.T.);
#25793=EDGE_CURVE('',#20778,#20777,#2461,.T.);
#25794=EDGE_CURVE('',#20779,#20778,#2462,.T.);
#25795=EDGE_CURVE('',#20780,#20779,#2463,.T.);
#25796=EDGE_CURVE('',#20781,#20780,#2464,.T.);
#25797=EDGE_CURVE('',#20782,#20781,#2465,.T.);
#25798=EDGE_CURVE('',#20783,#20782,#2466,.T.);
#25799=EDGE_CURVE('',#20784,#20783,#2467,.T.);
#25800=EDGE_CURVE('',#20785,#20784,#2468,.T.);
#25801=EDGE_CURVE('',#20786,#20785,#2469,.T.);
#25802=EDGE_CURVE('',#20787,#20786,#2470,.T.);
#25803=EDGE_CURVE('',#20788,#20787,#2471,.T.);
#25804=EDGE_CURVE('',#20788,#20789,#18824,.T.);
#25805=EDGE_CURVE('',#20790,#20789,#2472,.T.);
#25806=EDGE_CURVE('',#20791,#20790,#2473,.T.);
#25807=EDGE_CURVE('',#20792,#20791,#2474,.T.);
#25808=EDGE_CURVE('',#20793,#20792,#2475,.T.);
#25809=EDGE_CURVE('',#20794,#20793,#2476,.T.);
#25810=EDGE_CURVE('',#20795,#20794,#2477,.T.);
#25811=EDGE_CURVE('',#20796,#20795,#2478,.T.);
#25812=EDGE_CURVE('',#20797,#20796,#2479,.T.);
#25813=EDGE_CURVE('',#20798,#20797,#2480,.T.);
#25814=EDGE_CURVE('',#20799,#20798,#2481,.T.);
#25815=EDGE_CURVE('',#20800,#20799,#2482,.T.);
#25816=EDGE_CURVE('',#20801,#20800,#2483,.T.);
#25817=EDGE_CURVE('',#20802,#20801,#2484,.T.);
#25818=EDGE_CURVE('',#20803,#20802,#2485,.T.);
#25819=EDGE_CURVE('',#20431,#20803,#2486,.T.);
#25820=EDGE_CURVE('',#20428,#20804,#2487,.T.);
#25821=EDGE_CURVE('',#20804,#20805,#2488,.T.);
#25822=EDGE_CURVE('',#20806,#20805,#18825,.T.);
#25823=EDGE_CURVE('',#20807,#20806,#1297,.T.);
#25824=EDGE_CURVE('',#20774,#20807,#2489,.T.);
#25825=EDGE_CURVE('',#20808,#20426,#2490,.T.);
#25826=EDGE_CURVE('',#20809,#20808,#2491,.T.);
#25827=EDGE_CURVE('',#20810,#20809,#2492,.T.);
#25828=EDGE_CURVE('',#20811,#20810,#2493,.T.);
#25829=EDGE_CURVE('',#20812,#20811,#2494,.T.);
#25830=EDGE_CURVE('',#20813,#20812,#2495,.T.);
#25831=EDGE_CURVE('',#20814,#20813,#2496,.T.);
#25832=EDGE_CURVE('',#20815,#20814,#2497,.T.);
#25833=EDGE_CURVE('',#20816,#20815,#2498,.T.);
#25834=EDGE_CURVE('',#20817,#20816,#2499,.T.);
#25835=EDGE_CURVE('',#20818,#20817,#2500,.T.);
#25836=EDGE_CURVE('',#20819,#20818,#2501,.T.);
#25837=EDGE_CURVE('',#20820,#20819,#2502,.T.);
#25838=EDGE_CURVE('',#20821,#20820,#2503,.T.);
#25839=EDGE_CURVE('',#20822,#20821,#2504,.T.);
#25840=EDGE_CURVE('',#20822,#20823,#18826,.T.);
#25841=EDGE_CURVE('',#20824,#20823,#2505,.T.);
#25842=EDGE_CURVE('',#20825,#20824,#2506,.T.);
#25843=EDGE_CURVE('',#20826,#20825,#2507,.T.);
#25844=EDGE_CURVE('',#20827,#20826,#2508,.T.);
#25845=EDGE_CURVE('',#20828,#20827,#2509,.T.);
#25846=EDGE_CURVE('',#20829,#20828,#2510,.T.);
#25847=EDGE_CURVE('',#20830,#20829,#2511,.T.);
#25848=EDGE_CURVE('',#20831,#20830,#2512,.T.);
#25849=EDGE_CURVE('',#20832,#20831,#2513,.T.);
#25850=EDGE_CURVE('',#20833,#20832,#2514,.T.);
#25851=EDGE_CURVE('',#20834,#20833,#2515,.T.);
#25852=EDGE_CURVE('',#20835,#20834,#2516,.T.);
#25853=EDGE_CURVE('',#20836,#20835,#2517,.T.);
#25854=EDGE_CURVE('',#20837,#20836,#2518,.T.);
#25855=EDGE_CURVE('',#20427,#20837,#2519,.T.);
#25856=EDGE_CURVE('',#20424,#20838,#2520,.T.);
#25857=EDGE_CURVE('',#20838,#20839,#2521,.T.);
#25858=EDGE_CURVE('',#20840,#20839,#18827,.T.);
#25859=EDGE_CURVE('',#20841,#20840,#1298,.T.);
#25860=EDGE_CURVE('',#20808,#20841,#2522,.T.);
#25861=EDGE_CURVE('',#20842,#20422,#2523,.T.);
#25862=EDGE_CURVE('',#20843,#20842,#2524,.T.);
#25863=EDGE_CURVE('',#20844,#20843,#2525,.T.);
#25864=EDGE_CURVE('',#20845,#20844,#2526,.T.);
#25865=EDGE_CURVE('',#20846,#20845,#2527,.T.);
#25866=EDGE_CURVE('',#20847,#20846,#2528,.T.);
#25867=EDGE_CURVE('',#20848,#20847,#2529,.T.);
#25868=EDGE_CURVE('',#20849,#20848,#2530,.T.);
#25869=EDGE_CURVE('',#20850,#20849,#2531,.T.);
#25870=EDGE_CURVE('',#20851,#20850,#2532,.T.);
#25871=EDGE_CURVE('',#20852,#20851,#2533,.T.);
#25872=EDGE_CURVE('',#20853,#20852,#2534,.T.);
#25873=EDGE_CURVE('',#20854,#20853,#2535,.T.);
#25874=EDGE_CURVE('',#20855,#20854,#2536,.T.);
#25875=EDGE_CURVE('',#20856,#20855,#2537,.T.);
#25876=EDGE_CURVE('',#20856,#20857,#18828,.T.);
#25877=EDGE_CURVE('',#20858,#20857,#2538,.T.);
#25878=EDGE_CURVE('',#20859,#20858,#2539,.T.);
#25879=EDGE_CURVE('',#20860,#20859,#2540,.T.);
#25880=EDGE_CURVE('',#20861,#20860,#2541,.T.);
#25881=EDGE_CURVE('',#20862,#20861,#2542,.T.);
#25882=EDGE_CURVE('',#20863,#20862,#2543,.T.);
#25883=EDGE_CURVE('',#20864,#20863,#2544,.T.);
#25884=EDGE_CURVE('',#20865,#20864,#2545,.T.);
#25885=EDGE_CURVE('',#20866,#20865,#2546,.T.);
#25886=EDGE_CURVE('',#20867,#20866,#2547,.T.);
#25887=EDGE_CURVE('',#20868,#20867,#2548,.T.);
#25888=EDGE_CURVE('',#20869,#20868,#2549,.T.);
#25889=EDGE_CURVE('',#20870,#20869,#2550,.T.);
#25890=EDGE_CURVE('',#20871,#20870,#2551,.T.);
#25891=EDGE_CURVE('',#20423,#20871,#2552,.T.);
#25892=EDGE_CURVE('',#20420,#20872,#2553,.T.);
#25893=EDGE_CURVE('',#20872,#20873,#2554,.T.);
#25894=EDGE_CURVE('',#20874,#20873,#18829,.T.);
#25895=EDGE_CURVE('',#20875,#20874,#1299,.T.);
#25896=EDGE_CURVE('',#20842,#20875,#2555,.T.);
#25897=EDGE_CURVE('',#20876,#20418,#2556,.T.);
#25898=EDGE_CURVE('',#20877,#20876,#2557,.T.);
#25899=EDGE_CURVE('',#20878,#20877,#2558,.T.);
#25900=EDGE_CURVE('',#20879,#20878,#2559,.T.);
#25901=EDGE_CURVE('',#20880,#20879,#2560,.T.);
#25902=EDGE_CURVE('',#20881,#20880,#2561,.T.);
#25903=EDGE_CURVE('',#20882,#20881,#2562,.T.);
#25904=EDGE_CURVE('',#20883,#20882,#2563,.T.);
#25905=EDGE_CURVE('',#20884,#20883,#2564,.T.);
#25906=EDGE_CURVE('',#20885,#20884,#2565,.T.);
#25907=EDGE_CURVE('',#20886,#20885,#2566,.T.);
#25908=EDGE_CURVE('',#20887,#20886,#2567,.T.);
#25909=EDGE_CURVE('',#20888,#20887,#2568,.T.);
#25910=EDGE_CURVE('',#20889,#20888,#2569,.T.);
#25911=EDGE_CURVE('',#20890,#20889,#2570,.T.);
#25912=EDGE_CURVE('',#20890,#20891,#18830,.T.);
#25913=EDGE_CURVE('',#20892,#20891,#2571,.T.);
#25914=EDGE_CURVE('',#20893,#20892,#2572,.T.);
#25915=EDGE_CURVE('',#20894,#20893,#2573,.T.);
#25916=EDGE_CURVE('',#20895,#20894,#2574,.T.);
#25917=EDGE_CURVE('',#20896,#20895,#2575,.T.);
#25918=EDGE_CURVE('',#20897,#20896,#2576,.T.);
#25919=EDGE_CURVE('',#20898,#20897,#2577,.T.);
#25920=EDGE_CURVE('',#20899,#20898,#2578,.T.);
#25921=EDGE_CURVE('',#20900,#20899,#2579,.T.);
#25922=EDGE_CURVE('',#20901,#20900,#2580,.T.);
#25923=EDGE_CURVE('',#20902,#20901,#2581,.T.);
#25924=EDGE_CURVE('',#20903,#20902,#2582,.T.);
#25925=EDGE_CURVE('',#20904,#20903,#2583,.T.);
#25926=EDGE_CURVE('',#20905,#20904,#2584,.T.);
#25927=EDGE_CURVE('',#20419,#20905,#2585,.T.);
#25928=EDGE_CURVE('',#20416,#20906,#2586,.T.);
#25929=EDGE_CURVE('',#20906,#20907,#2587,.T.);
#25930=EDGE_CURVE('',#20908,#20907,#18831,.T.);
#25931=EDGE_CURVE('',#20909,#20908,#1300,.T.);
#25932=EDGE_CURVE('',#20876,#20909,#2588,.T.);
#25933=EDGE_CURVE('',#20910,#20414,#2589,.T.);
#25934=EDGE_CURVE('',#20911,#20910,#2590,.T.);
#25935=EDGE_CURVE('',#20912,#20911,#2591,.T.);
#25936=EDGE_CURVE('',#20913,#20912,#2592,.T.);
#25937=EDGE_CURVE('',#20914,#20913,#2593,.T.);
#25938=EDGE_CURVE('',#20915,#20914,#2594,.T.);
#25939=EDGE_CURVE('',#20916,#20915,#2595,.T.);
#25940=EDGE_CURVE('',#20917,#20916,#2596,.T.);
#25941=EDGE_CURVE('',#20918,#20917,#2597,.T.);
#25942=EDGE_CURVE('',#20919,#20918,#2598,.T.);
#25943=EDGE_CURVE('',#20920,#20919,#2599,.T.);
#25944=EDGE_CURVE('',#20921,#20920,#2600,.T.);
#25945=EDGE_CURVE('',#20922,#20921,#2601,.T.);
#25946=EDGE_CURVE('',#20923,#20922,#2602,.T.);
#25947=EDGE_CURVE('',#20924,#20923,#2603,.T.);
#25948=EDGE_CURVE('',#20924,#20925,#18832,.T.);
#25949=EDGE_CURVE('',#20926,#20925,#2604,.T.);
#25950=EDGE_CURVE('',#20927,#20926,#2605,.T.);
#25951=EDGE_CURVE('',#20928,#20927,#2606,.T.);
#25952=EDGE_CURVE('',#20929,#20928,#2607,.T.);
#25953=EDGE_CURVE('',#20930,#20929,#2608,.T.);
#25954=EDGE_CURVE('',#20931,#20930,#2609,.T.);
#25955=EDGE_CURVE('',#20932,#20931,#2610,.T.);
#25956=EDGE_CURVE('',#20933,#20932,#2611,.T.);
#25957=EDGE_CURVE('',#20934,#20933,#2612,.T.);
#25958=EDGE_CURVE('',#20935,#20934,#2613,.T.);
#25959=EDGE_CURVE('',#20936,#20935,#2614,.T.);
#25960=EDGE_CURVE('',#20937,#20936,#2615,.T.);
#25961=EDGE_CURVE('',#20938,#20937,#2616,.T.);
#25962=EDGE_CURVE('',#20939,#20938,#2617,.T.);
#25963=EDGE_CURVE('',#20415,#20939,#2618,.T.);
#25964=EDGE_CURVE('',#20412,#20940,#2619,.T.);
#25965=EDGE_CURVE('',#20940,#20941,#2620,.T.);
#25966=EDGE_CURVE('',#20942,#20941,#18833,.T.);
#25967=EDGE_CURVE('',#20943,#20942,#1301,.T.);
#25968=EDGE_CURVE('',#20910,#20943,#2621,.T.);
#25969=EDGE_CURVE('',#20944,#20410,#2622,.T.);
#25970=EDGE_CURVE('',#20945,#20944,#2623,.T.);
#25971=EDGE_CURVE('',#20946,#20945,#2624,.T.);
#25972=EDGE_CURVE('',#20947,#20946,#2625,.T.);
#25973=EDGE_CURVE('',#20948,#20947,#2626,.T.);
#25974=EDGE_CURVE('',#20949,#20948,#2627,.T.);
#25975=EDGE_CURVE('',#20950,#20949,#2628,.T.);
#25976=EDGE_CURVE('',#20951,#20950,#2629,.T.);
#25977=EDGE_CURVE('',#20952,#20951,#2630,.T.);
#25978=EDGE_CURVE('',#20953,#20952,#2631,.T.);
#25979=EDGE_CURVE('',#20954,#20953,#2632,.T.);
#25980=EDGE_CURVE('',#20955,#20954,#2633,.T.);
#25981=EDGE_CURVE('',#20956,#20955,#2634,.T.);
#25982=EDGE_CURVE('',#20957,#20956,#2635,.T.);
#25983=EDGE_CURVE('',#20958,#20957,#2636,.T.);
#25984=EDGE_CURVE('',#20958,#20959,#18834,.T.);
#25985=EDGE_CURVE('',#20960,#20959,#2637,.T.);
#25986=EDGE_CURVE('',#20961,#20960,#2638,.T.);
#25987=EDGE_CURVE('',#20962,#20961,#2639,.T.);
#25988=EDGE_CURVE('',#20963,#20962,#2640,.T.);
#25989=EDGE_CURVE('',#20964,#20963,#2641,.T.);
#25990=EDGE_CURVE('',#20965,#20964,#2642,.T.);
#25991=EDGE_CURVE('',#20966,#20965,#2643,.T.);
#25992=EDGE_CURVE('',#20967,#20966,#2644,.T.);
#25993=EDGE_CURVE('',#20968,#20967,#2645,.T.);
#25994=EDGE_CURVE('',#20969,#20968,#2646,.T.);
#25995=EDGE_CURVE('',#20970,#20969,#2647,.T.);
#25996=EDGE_CURVE('',#20971,#20970,#2648,.T.);
#25997=EDGE_CURVE('',#20972,#20971,#2649,.T.);
#25998=EDGE_CURVE('',#20973,#20972,#2650,.T.);
#25999=EDGE_CURVE('',#20411,#20973,#2651,.T.);
#26000=EDGE_CURVE('',#20408,#20974,#2652,.T.);
#26001=EDGE_CURVE('',#20974,#20975,#2653,.T.);
#26002=EDGE_CURVE('',#20976,#20975,#18835,.T.);
#26003=EDGE_CURVE('',#20977,#20976,#1302,.T.);
#26004=EDGE_CURVE('',#20944,#20977,#2654,.T.);
#26005=EDGE_CURVE('',#20978,#20406,#2655,.T.);
#26006=EDGE_CURVE('',#20979,#20978,#2656,.T.);
#26007=EDGE_CURVE('',#20980,#20979,#2657,.T.);
#26008=EDGE_CURVE('',#20981,#20980,#2658,.T.);
#26009=EDGE_CURVE('',#20982,#20981,#2659,.T.);
#26010=EDGE_CURVE('',#20983,#20982,#2660,.T.);
#26011=EDGE_CURVE('',#20984,#20983,#2661,.T.);
#26012=EDGE_CURVE('',#20985,#20984,#2662,.T.);
#26013=EDGE_CURVE('',#20986,#20985,#2663,.T.);
#26014=EDGE_CURVE('',#20987,#20986,#2664,.T.);
#26015=EDGE_CURVE('',#20988,#20987,#2665,.T.);
#26016=EDGE_CURVE('',#20989,#20988,#2666,.T.);
#26017=EDGE_CURVE('',#20990,#20989,#2667,.T.);
#26018=EDGE_CURVE('',#20991,#20990,#2668,.T.);
#26019=EDGE_CURVE('',#20992,#20991,#2669,.T.);
#26020=EDGE_CURVE('',#20992,#20993,#18836,.T.);
#26021=EDGE_CURVE('',#20994,#20993,#2670,.T.);
#26022=EDGE_CURVE('',#20995,#20994,#2671,.T.);
#26023=EDGE_CURVE('',#20996,#20995,#2672,.T.);
#26024=EDGE_CURVE('',#20997,#20996,#2673,.T.);
#26025=EDGE_CURVE('',#20998,#20997,#2674,.T.);
#26026=EDGE_CURVE('',#20999,#20998,#2675,.T.);
#26027=EDGE_CURVE('',#21000,#20999,#2676,.T.);
#26028=EDGE_CURVE('',#21001,#21000,#2677,.T.);
#26029=EDGE_CURVE('',#21002,#21001,#2678,.T.);
#26030=EDGE_CURVE('',#21003,#21002,#2679,.T.);
#26031=EDGE_CURVE('',#21004,#21003,#2680,.T.);
#26032=EDGE_CURVE('',#21005,#21004,#2681,.T.);
#26033=EDGE_CURVE('',#21006,#21005,#2682,.T.);
#26034=EDGE_CURVE('',#21007,#21006,#2683,.T.);
#26035=EDGE_CURVE('',#20407,#21007,#2684,.T.);
#26036=EDGE_CURVE('',#20404,#21008,#2685,.T.);
#26037=EDGE_CURVE('',#21008,#21009,#2686,.T.);
#26038=EDGE_CURVE('',#21010,#21009,#18837,.T.);
#26039=EDGE_CURVE('',#21011,#21010,#1303,.T.);
#26040=EDGE_CURVE('',#20978,#21011,#2687,.T.);
#26041=EDGE_CURVE('',#21012,#20402,#2688,.T.);
#26042=EDGE_CURVE('',#21013,#21012,#2689,.T.);
#26043=EDGE_CURVE('',#21014,#21013,#2690,.T.);
#26044=EDGE_CURVE('',#21015,#21014,#2691,.T.);
#26045=EDGE_CURVE('',#21016,#21015,#2692,.T.);
#26046=EDGE_CURVE('',#21017,#21016,#2693,.T.);
#26047=EDGE_CURVE('',#21018,#21017,#2694,.T.);
#26048=EDGE_CURVE('',#21019,#21018,#2695,.T.);
#26049=EDGE_CURVE('',#21020,#21019,#2696,.T.);
#26050=EDGE_CURVE('',#21021,#21020,#2697,.T.);
#26051=EDGE_CURVE('',#21022,#21021,#2698,.T.);
#26052=EDGE_CURVE('',#21023,#21022,#2699,.T.);
#26053=EDGE_CURVE('',#21024,#21023,#2700,.T.);
#26054=EDGE_CURVE('',#21025,#21024,#2701,.T.);
#26055=EDGE_CURVE('',#21026,#21025,#2702,.T.);
#26056=EDGE_CURVE('',#21026,#21027,#18838,.T.);
#26057=EDGE_CURVE('',#21028,#21027,#2703,.T.);
#26058=EDGE_CURVE('',#21029,#21028,#2704,.T.);
#26059=EDGE_CURVE('',#21030,#21029,#2705,.T.);
#26060=EDGE_CURVE('',#21031,#21030,#2706,.T.);
#26061=EDGE_CURVE('',#21032,#21031,#2707,.T.);
#26062=EDGE_CURVE('',#21033,#21032,#2708,.T.);
#26063=EDGE_CURVE('',#21034,#21033,#2709,.T.);
#26064=EDGE_CURVE('',#21035,#21034,#2710,.T.);
#26065=EDGE_CURVE('',#21036,#21035,#2711,.T.);
#26066=EDGE_CURVE('',#21037,#21036,#2712,.T.);
#26067=EDGE_CURVE('',#21038,#21037,#2713,.T.);
#26068=EDGE_CURVE('',#21039,#21038,#2714,.T.);
#26069=EDGE_CURVE('',#21040,#21039,#2715,.T.);
#26070=EDGE_CURVE('',#21041,#21040,#2716,.T.);
#26071=EDGE_CURVE('',#20403,#21041,#2717,.T.);
#26072=EDGE_CURVE('',#20400,#21042,#2718,.T.);
#26073=EDGE_CURVE('',#21042,#21043,#2719,.T.);
#26074=EDGE_CURVE('',#21044,#21043,#18839,.T.);
#26075=EDGE_CURVE('',#21045,#21044,#1304,.T.);
#26076=EDGE_CURVE('',#21012,#21045,#2720,.T.);
#26077=EDGE_CURVE('',#21046,#20398,#2721,.T.);
#26078=EDGE_CURVE('',#21047,#21046,#2722,.T.);
#26079=EDGE_CURVE('',#21048,#21047,#2723,.T.);
#26080=EDGE_CURVE('',#21049,#21048,#2724,.T.);
#26081=EDGE_CURVE('',#21050,#21049,#2725,.T.);
#26082=EDGE_CURVE('',#21051,#21050,#2726,.T.);
#26083=EDGE_CURVE('',#21052,#21051,#2727,.T.);
#26084=EDGE_CURVE('',#21053,#21052,#2728,.T.);
#26085=EDGE_CURVE('',#21054,#21053,#2729,.T.);
#26086=EDGE_CURVE('',#21055,#21054,#2730,.T.);
#26087=EDGE_CURVE('',#21056,#21055,#2731,.T.);
#26088=EDGE_CURVE('',#21057,#21056,#2732,.T.);
#26089=EDGE_CURVE('',#21058,#21057,#2733,.T.);
#26090=EDGE_CURVE('',#21059,#21058,#2734,.T.);
#26091=EDGE_CURVE('',#21060,#21059,#2735,.T.);
#26092=EDGE_CURVE('',#21060,#21061,#18840,.T.);
#26093=EDGE_CURVE('',#21062,#21061,#2736,.T.);
#26094=EDGE_CURVE('',#21063,#21062,#2737,.T.);
#26095=EDGE_CURVE('',#21064,#21063,#2738,.T.);
#26096=EDGE_CURVE('',#21065,#21064,#2739,.T.);
#26097=EDGE_CURVE('',#21066,#21065,#2740,.T.);
#26098=EDGE_CURVE('',#21067,#21066,#2741,.T.);
#26099=EDGE_CURVE('',#21068,#21067,#2742,.T.);
#26100=EDGE_CURVE('',#21069,#21068,#2743,.T.);
#26101=EDGE_CURVE('',#21070,#21069,#2744,.T.);
#26102=EDGE_CURVE('',#21071,#21070,#2745,.T.);
#26103=EDGE_CURVE('',#21072,#21071,#2746,.T.);
#26104=EDGE_CURVE('',#21073,#21072,#2747,.T.);
#26105=EDGE_CURVE('',#21074,#21073,#2748,.T.);
#26106=EDGE_CURVE('',#21075,#21074,#2749,.T.);
#26107=EDGE_CURVE('',#20399,#21075,#2750,.T.);
#26108=EDGE_CURVE('',#20396,#21076,#2751,.T.);
#26109=EDGE_CURVE('',#21076,#21077,#2752,.T.);
#26110=EDGE_CURVE('',#21078,#21077,#18841,.T.);
#26111=EDGE_CURVE('',#21079,#21078,#1305,.T.);
#26112=EDGE_CURVE('',#21046,#21079,#2753,.T.);
#26113=EDGE_CURVE('',#21080,#20394,#2754,.T.);
#26114=EDGE_CURVE('',#21081,#21080,#2755,.T.);
#26115=EDGE_CURVE('',#21082,#21081,#2756,.T.);
#26116=EDGE_CURVE('',#21083,#21082,#2757,.T.);
#26117=EDGE_CURVE('',#21084,#21083,#2758,.T.);
#26118=EDGE_CURVE('',#21085,#21084,#2759,.T.);
#26119=EDGE_CURVE('',#21086,#21085,#2760,.T.);
#26120=EDGE_CURVE('',#21087,#21086,#2761,.T.);
#26121=EDGE_CURVE('',#21088,#21087,#2762,.T.);
#26122=EDGE_CURVE('',#21089,#21088,#2763,.T.);
#26123=EDGE_CURVE('',#21090,#21089,#2764,.T.);
#26124=EDGE_CURVE('',#21091,#21090,#2765,.T.);
#26125=EDGE_CURVE('',#21092,#21091,#2766,.T.);
#26126=EDGE_CURVE('',#21093,#21092,#2767,.T.);
#26127=EDGE_CURVE('',#21094,#21093,#2768,.T.);
#26128=EDGE_CURVE('',#21094,#21095,#18842,.T.);
#26129=EDGE_CURVE('',#21096,#21095,#2769,.T.);
#26130=EDGE_CURVE('',#21097,#21096,#2770,.T.);
#26131=EDGE_CURVE('',#21098,#21097,#2771,.T.);
#26132=EDGE_CURVE('',#21099,#21098,#2772,.T.);
#26133=EDGE_CURVE('',#21100,#21099,#2773,.T.);
#26134=EDGE_CURVE('',#21101,#21100,#2774,.T.);
#26135=EDGE_CURVE('',#21102,#21101,#2775,.T.);
#26136=EDGE_CURVE('',#21103,#21102,#2776,.T.);
#26137=EDGE_CURVE('',#21104,#21103,#2777,.T.);
#26138=EDGE_CURVE('',#21105,#21104,#2778,.T.);
#26139=EDGE_CURVE('',#21106,#21105,#2779,.T.);
#26140=EDGE_CURVE('',#21107,#21106,#2780,.T.);
#26141=EDGE_CURVE('',#21108,#21107,#2781,.T.);
#26142=EDGE_CURVE('',#21109,#21108,#2782,.T.);
#26143=EDGE_CURVE('',#20395,#21109,#2783,.T.);
#26144=EDGE_CURVE('',#20392,#21110,#2784,.T.);
#26145=EDGE_CURVE('',#21110,#21111,#2785,.T.);
#26146=EDGE_CURVE('',#21112,#21111,#18843,.T.);
#26147=EDGE_CURVE('',#21113,#21112,#1306,.T.);
#26148=EDGE_CURVE('',#21080,#21113,#2786,.T.);
#26149=EDGE_CURVE('',#21114,#20390,#2787,.T.);
#26150=EDGE_CURVE('',#21115,#21114,#2788,.T.);
#26151=EDGE_CURVE('',#21116,#21115,#2789,.T.);
#26152=EDGE_CURVE('',#21117,#21116,#2790,.T.);
#26153=EDGE_CURVE('',#21118,#21117,#2791,.T.);
#26154=EDGE_CURVE('',#21119,#21118,#2792,.T.);
#26155=EDGE_CURVE('',#21120,#21119,#2793,.T.);
#26156=EDGE_CURVE('',#21121,#21120,#2794,.T.);
#26157=EDGE_CURVE('',#21122,#21121,#2795,.T.);
#26158=EDGE_CURVE('',#21123,#21122,#2796,.T.);
#26159=EDGE_CURVE('',#21124,#21123,#2797,.T.);
#26160=EDGE_CURVE('',#21125,#21124,#2798,.T.);
#26161=EDGE_CURVE('',#21126,#21125,#2799,.T.);
#26162=EDGE_CURVE('',#21127,#21126,#2800,.T.);
#26163=EDGE_CURVE('',#21128,#21127,#2801,.T.);
#26164=EDGE_CURVE('',#21128,#21129,#18844,.T.);
#26165=EDGE_CURVE('',#21130,#21129,#2802,.T.);
#26166=EDGE_CURVE('',#21131,#21130,#2803,.T.);
#26167=EDGE_CURVE('',#21132,#21131,#2804,.T.);
#26168=EDGE_CURVE('',#21133,#21132,#2805,.T.);
#26169=EDGE_CURVE('',#21134,#21133,#2806,.T.);
#26170=EDGE_CURVE('',#21135,#21134,#2807,.T.);
#26171=EDGE_CURVE('',#21136,#21135,#2808,.T.);
#26172=EDGE_CURVE('',#21137,#21136,#2809,.T.);
#26173=EDGE_CURVE('',#21138,#21137,#2810,.T.);
#26174=EDGE_CURVE('',#21139,#21138,#2811,.T.);
#26175=EDGE_CURVE('',#21140,#21139,#2812,.T.);
#26176=EDGE_CURVE('',#21141,#21140,#2813,.T.);
#26177=EDGE_CURVE('',#21142,#21141,#2814,.T.);
#26178=EDGE_CURVE('',#21143,#21142,#2815,.T.);
#26179=EDGE_CURVE('',#20391,#21143,#2816,.T.);
#26180=EDGE_CURVE('',#20388,#21144,#2817,.T.);
#26181=EDGE_CURVE('',#21144,#21145,#2818,.T.);
#26182=EDGE_CURVE('',#21146,#21145,#18845,.T.);
#26183=EDGE_CURVE('',#21147,#21146,#1307,.T.);
#26184=EDGE_CURVE('',#21114,#21147,#2819,.T.);
#26185=EDGE_CURVE('',#21148,#20386,#2820,.T.);
#26186=EDGE_CURVE('',#21149,#21148,#2821,.T.);
#26187=EDGE_CURVE('',#21150,#21149,#2822,.T.);
#26188=EDGE_CURVE('',#21151,#21150,#2823,.T.);
#26189=EDGE_CURVE('',#21152,#21151,#2824,.T.);
#26190=EDGE_CURVE('',#21153,#21152,#2825,.T.);
#26191=EDGE_CURVE('',#21154,#21153,#2826,.T.);
#26192=EDGE_CURVE('',#21155,#21154,#2827,.T.);
#26193=EDGE_CURVE('',#21156,#21155,#2828,.T.);
#26194=EDGE_CURVE('',#21157,#21156,#2829,.T.);
#26195=EDGE_CURVE('',#21158,#21157,#2830,.T.);
#26196=EDGE_CURVE('',#21159,#21158,#2831,.T.);
#26197=EDGE_CURVE('',#21160,#21159,#2832,.T.);
#26198=EDGE_CURVE('',#21161,#21160,#2833,.T.);
#26199=EDGE_CURVE('',#21162,#21161,#2834,.T.);
#26200=EDGE_CURVE('',#21162,#21163,#18846,.T.);
#26201=EDGE_CURVE('',#21164,#21163,#2835,.T.);
#26202=EDGE_CURVE('',#21165,#21164,#2836,.T.);
#26203=EDGE_CURVE('',#21166,#21165,#2837,.T.);
#26204=EDGE_CURVE('',#21167,#21166,#2838,.T.);
#26205=EDGE_CURVE('',#21168,#21167,#2839,.T.);
#26206=EDGE_CURVE('',#21169,#21168,#2840,.T.);
#26207=EDGE_CURVE('',#21170,#21169,#2841,.T.);
#26208=EDGE_CURVE('',#21171,#21170,#2842,.T.);
#26209=EDGE_CURVE('',#21172,#21171,#2843,.T.);
#26210=EDGE_CURVE('',#21173,#21172,#2844,.T.);
#26211=EDGE_CURVE('',#21174,#21173,#2845,.T.);
#26212=EDGE_CURVE('',#21175,#21174,#2846,.T.);
#26213=EDGE_CURVE('',#21176,#21175,#2847,.T.);
#26214=EDGE_CURVE('',#21177,#21176,#2848,.T.);
#26215=EDGE_CURVE('',#20387,#21177,#2849,.T.);
#26216=EDGE_CURVE('',#20384,#21178,#2850,.T.);
#26217=EDGE_CURVE('',#21178,#21179,#2851,.T.);
#26218=EDGE_CURVE('',#21180,#21179,#18847,.T.);
#26219=EDGE_CURVE('',#21181,#21180,#1308,.T.);
#26220=EDGE_CURVE('',#21148,#21181,#2852,.T.);
#26221=EDGE_CURVE('',#21182,#20382,#2853,.T.);
#26222=EDGE_CURVE('',#21183,#21182,#2854,.T.);
#26223=EDGE_CURVE('',#21184,#21183,#2855,.T.);
#26224=EDGE_CURVE('',#21185,#21184,#2856,.T.);
#26225=EDGE_CURVE('',#21186,#21185,#2857,.T.);
#26226=EDGE_CURVE('',#21187,#21186,#2858,.T.);
#26227=EDGE_CURVE('',#21188,#21187,#2859,.T.);
#26228=EDGE_CURVE('',#21189,#21188,#2860,.T.);
#26229=EDGE_CURVE('',#21190,#21189,#2861,.T.);
#26230=EDGE_CURVE('',#21191,#21190,#2862,.T.);
#26231=EDGE_CURVE('',#21192,#21191,#2863,.T.);
#26232=EDGE_CURVE('',#21193,#21192,#2864,.T.);
#26233=EDGE_CURVE('',#21194,#21193,#2865,.T.);
#26234=EDGE_CURVE('',#21195,#21194,#2866,.T.);
#26235=EDGE_CURVE('',#21196,#21195,#2867,.T.);
#26236=EDGE_CURVE('',#21196,#21197,#18848,.T.);
#26237=EDGE_CURVE('',#21198,#21197,#2868,.T.);
#26238=EDGE_CURVE('',#21199,#21198,#2869,.T.);
#26239=EDGE_CURVE('',#21200,#21199,#2870,.T.);
#26240=EDGE_CURVE('',#21201,#21200,#2871,.T.);
#26241=EDGE_CURVE('',#21202,#21201,#2872,.T.);
#26242=EDGE_CURVE('',#21203,#21202,#2873,.T.);
#26243=EDGE_CURVE('',#21204,#21203,#2874,.T.);
#26244=EDGE_CURVE('',#21205,#21204,#2875,.T.);
#26245=EDGE_CURVE('',#21206,#21205,#2876,.T.);
#26246=EDGE_CURVE('',#21207,#21206,#2877,.T.);
#26247=EDGE_CURVE('',#21208,#21207,#2878,.T.);
#26248=EDGE_CURVE('',#21209,#21208,#2879,.T.);
#26249=EDGE_CURVE('',#21210,#21209,#2880,.T.);
#26250=EDGE_CURVE('',#21211,#21210,#2881,.T.);
#26251=EDGE_CURVE('',#20383,#21211,#2882,.T.);
#26252=EDGE_CURVE('',#20380,#21212,#2883,.T.);
#26253=EDGE_CURVE('',#21212,#21213,#2884,.T.);
#26254=EDGE_CURVE('',#21214,#21213,#18849,.T.);
#26255=EDGE_CURVE('',#21215,#21214,#1309,.T.);
#26256=EDGE_CURVE('',#21182,#21215,#2885,.T.);
#26257=EDGE_CURVE('',#21216,#20378,#2886,.T.);
#26258=EDGE_CURVE('',#21217,#21216,#2887,.T.);
#26259=EDGE_CURVE('',#21218,#21217,#2888,.T.);
#26260=EDGE_CURVE('',#21219,#21218,#2889,.T.);
#26261=EDGE_CURVE('',#21220,#21219,#2890,.T.);
#26262=EDGE_CURVE('',#21221,#21220,#2891,.T.);
#26263=EDGE_CURVE('',#21222,#21221,#2892,.T.);
#26264=EDGE_CURVE('',#21223,#21222,#2893,.T.);
#26265=EDGE_CURVE('',#21224,#21223,#2894,.T.);
#26266=EDGE_CURVE('',#21225,#21224,#2895,.T.);
#26267=EDGE_CURVE('',#21226,#21225,#2896,.T.);
#26268=EDGE_CURVE('',#21227,#21226,#2897,.T.);
#26269=EDGE_CURVE('',#21228,#21227,#2898,.T.);
#26270=EDGE_CURVE('',#21229,#21228,#2899,.T.);
#26271=EDGE_CURVE('',#21230,#21229,#2900,.T.);
#26272=EDGE_CURVE('',#21230,#21231,#18850,.T.);
#26273=EDGE_CURVE('',#21232,#21231,#2901,.T.);
#26274=EDGE_CURVE('',#21233,#21232,#2902,.T.);
#26275=EDGE_CURVE('',#21234,#21233,#2903,.T.);
#26276=EDGE_CURVE('',#21235,#21234,#2904,.T.);
#26277=EDGE_CURVE('',#21236,#21235,#2905,.T.);
#26278=EDGE_CURVE('',#21237,#21236,#2906,.T.);
#26279=EDGE_CURVE('',#21238,#21237,#2907,.T.);
#26280=EDGE_CURVE('',#21239,#21238,#2908,.T.);
#26281=EDGE_CURVE('',#21240,#21239,#2909,.T.);
#26282=EDGE_CURVE('',#21241,#21240,#2910,.T.);
#26283=EDGE_CURVE('',#21242,#21241,#2911,.T.);
#26284=EDGE_CURVE('',#21243,#21242,#2912,.T.);
#26285=EDGE_CURVE('',#21244,#21243,#2913,.T.);
#26286=EDGE_CURVE('',#21245,#21244,#2914,.T.);
#26287=EDGE_CURVE('',#20379,#21245,#2915,.T.);
#26288=EDGE_CURVE('',#20376,#21246,#2916,.T.);
#26289=EDGE_CURVE('',#21246,#21247,#2917,.T.);
#26290=EDGE_CURVE('',#21248,#21247,#18851,.T.);
#26291=EDGE_CURVE('',#21249,#21248,#1310,.T.);
#26292=EDGE_CURVE('',#21216,#21249,#2918,.T.);
#26293=EDGE_CURVE('',#21250,#20374,#2919,.T.);
#26294=EDGE_CURVE('',#21251,#21250,#2920,.T.);
#26295=EDGE_CURVE('',#21252,#21251,#2921,.T.);
#26296=EDGE_CURVE('',#21253,#21252,#2922,.T.);
#26297=EDGE_CURVE('',#21254,#21253,#2923,.T.);
#26298=EDGE_CURVE('',#21255,#21254,#2924,.T.);
#26299=EDGE_CURVE('',#21256,#21255,#2925,.T.);
#26300=EDGE_CURVE('',#21257,#21256,#2926,.T.);
#26301=EDGE_CURVE('',#21258,#21257,#2927,.T.);
#26302=EDGE_CURVE('',#21259,#21258,#2928,.T.);
#26303=EDGE_CURVE('',#21260,#21259,#2929,.T.);
#26304=EDGE_CURVE('',#21261,#21260,#2930,.T.);
#26305=EDGE_CURVE('',#21262,#21261,#2931,.T.);
#26306=EDGE_CURVE('',#21263,#21262,#2932,.T.);
#26307=EDGE_CURVE('',#21264,#21263,#2933,.T.);
#26308=EDGE_CURVE('',#21264,#21265,#18852,.T.);
#26309=EDGE_CURVE('',#21266,#21265,#2934,.T.);
#26310=EDGE_CURVE('',#21267,#21266,#2935,.T.);
#26311=EDGE_CURVE('',#21268,#21267,#2936,.T.);
#26312=EDGE_CURVE('',#21269,#21268,#2937,.T.);
#26313=EDGE_CURVE('',#21270,#21269,#2938,.T.);
#26314=EDGE_CURVE('',#21271,#21270,#2939,.T.);
#26315=EDGE_CURVE('',#21272,#21271,#2940,.T.);
#26316=EDGE_CURVE('',#21273,#21272,#2941,.T.);
#26317=EDGE_CURVE('',#21274,#21273,#2942,.T.);
#26318=EDGE_CURVE('',#21275,#21274,#2943,.T.);
#26319=EDGE_CURVE('',#21276,#21275,#2944,.T.);
#26320=EDGE_CURVE('',#21277,#21276,#2945,.T.);
#26321=EDGE_CURVE('',#21278,#21277,#2946,.T.);
#26322=EDGE_CURVE('',#21279,#21278,#2947,.T.);
#26323=EDGE_CURVE('',#20375,#21279,#2948,.T.);
#26324=EDGE_CURVE('',#20372,#21280,#2949,.T.);
#26325=EDGE_CURVE('',#21280,#21281,#2950,.T.);
#26326=EDGE_CURVE('',#21282,#21281,#18853,.T.);
#26327=EDGE_CURVE('',#21283,#21282,#1311,.T.);
#26328=EDGE_CURVE('',#21250,#21283,#2951,.T.);
#26329=EDGE_CURVE('',#21284,#20370,#2952,.T.);
#26330=EDGE_CURVE('',#21285,#21284,#2953,.T.);
#26331=EDGE_CURVE('',#21286,#21285,#2954,.T.);
#26332=EDGE_CURVE('',#21287,#21286,#2955,.T.);
#26333=EDGE_CURVE('',#21288,#21287,#2956,.T.);
#26334=EDGE_CURVE('',#21289,#21288,#2957,.T.);
#26335=EDGE_CURVE('',#21290,#21289,#2958,.T.);
#26336=EDGE_CURVE('',#21291,#21290,#2959,.T.);
#26337=EDGE_CURVE('',#21292,#21291,#2960,.T.);
#26338=EDGE_CURVE('',#21293,#21292,#2961,.T.);
#26339=EDGE_CURVE('',#21294,#21293,#2962,.T.);
#26340=EDGE_CURVE('',#21295,#21294,#2963,.T.);
#26341=EDGE_CURVE('',#21296,#21295,#2964,.T.);
#26342=EDGE_CURVE('',#21297,#21296,#2965,.T.);
#26343=EDGE_CURVE('',#21298,#21297,#2966,.T.);
#26344=EDGE_CURVE('',#21298,#21299,#18854,.T.);
#26345=EDGE_CURVE('',#21300,#21299,#2967,.T.);
#26346=EDGE_CURVE('',#21301,#21300,#2968,.T.);
#26347=EDGE_CURVE('',#21302,#21301,#2969,.T.);
#26348=EDGE_CURVE('',#21303,#21302,#2970,.T.);
#26349=EDGE_CURVE('',#21304,#21303,#2971,.T.);
#26350=EDGE_CURVE('',#21305,#21304,#2972,.T.);
#26351=EDGE_CURVE('',#21306,#21305,#2973,.T.);
#26352=EDGE_CURVE('',#21307,#21306,#2974,.T.);
#26353=EDGE_CURVE('',#21308,#21307,#2975,.T.);
#26354=EDGE_CURVE('',#21309,#21308,#2976,.T.);
#26355=EDGE_CURVE('',#21310,#21309,#2977,.T.);
#26356=EDGE_CURVE('',#21311,#21310,#2978,.T.);
#26357=EDGE_CURVE('',#21312,#21311,#2979,.T.);
#26358=EDGE_CURVE('',#21313,#21312,#2980,.T.);
#26359=EDGE_CURVE('',#20371,#21313,#2981,.T.);
#26360=EDGE_CURVE('',#20368,#21314,#2982,.T.);
#26361=EDGE_CURVE('',#21314,#21315,#2983,.T.);
#26362=EDGE_CURVE('',#21316,#21315,#18855,.T.);
#26363=EDGE_CURVE('',#21317,#21316,#1312,.T.);
#26364=EDGE_CURVE('',#21284,#21317,#2984,.T.);
#26365=EDGE_CURVE('',#21318,#20366,#2985,.T.);
#26366=EDGE_CURVE('',#21319,#21318,#2986,.T.);
#26367=EDGE_CURVE('',#21320,#21319,#2987,.T.);
#26368=EDGE_CURVE('',#21321,#21320,#2988,.T.);
#26369=EDGE_CURVE('',#21322,#21321,#2989,.T.);
#26370=EDGE_CURVE('',#21323,#21322,#2990,.T.);
#26371=EDGE_CURVE('',#21324,#21323,#2991,.T.);
#26372=EDGE_CURVE('',#21325,#21324,#2992,.T.);
#26373=EDGE_CURVE('',#21326,#21325,#2993,.T.);
#26374=EDGE_CURVE('',#21327,#21326,#2994,.T.);
#26375=EDGE_CURVE('',#21328,#21327,#2995,.T.);
#26376=EDGE_CURVE('',#21329,#21328,#2996,.T.);
#26377=EDGE_CURVE('',#21330,#21329,#2997,.T.);
#26378=EDGE_CURVE('',#21331,#21330,#2998,.T.);
#26379=EDGE_CURVE('',#21332,#21331,#2999,.T.);
#26380=EDGE_CURVE('',#21332,#21333,#18856,.T.);
#26381=EDGE_CURVE('',#21334,#21333,#3000,.T.);
#26382=EDGE_CURVE('',#21335,#21334,#3001,.T.);
#26383=EDGE_CURVE('',#21336,#21335,#3002,.T.);
#26384=EDGE_CURVE('',#21337,#21336,#3003,.T.);
#26385=EDGE_CURVE('',#21338,#21337,#3004,.T.);
#26386=EDGE_CURVE('',#21339,#21338,#3005,.T.);
#26387=EDGE_CURVE('',#21340,#21339,#3006,.T.);
#26388=EDGE_CURVE('',#21341,#21340,#3007,.T.);
#26389=EDGE_CURVE('',#21342,#21341,#3008,.T.);
#26390=EDGE_CURVE('',#21343,#21342,#3009,.T.);
#26391=EDGE_CURVE('',#21344,#21343,#3010,.T.);
#26392=EDGE_CURVE('',#21345,#21344,#3011,.T.);
#26393=EDGE_CURVE('',#21346,#21345,#3012,.T.);
#26394=EDGE_CURVE('',#21347,#21346,#3013,.T.);
#26395=EDGE_CURVE('',#20367,#21347,#3014,.T.);
#26396=EDGE_CURVE('',#20364,#21348,#3015,.T.);
#26397=EDGE_CURVE('',#21348,#21349,#3016,.T.);
#26398=EDGE_CURVE('',#21350,#21349,#18857,.T.);
#26399=EDGE_CURVE('',#21351,#21350,#1313,.T.);
#26400=EDGE_CURVE('',#21318,#21351,#3017,.T.);
#26401=EDGE_CURVE('',#21352,#20362,#3018,.T.);
#26402=EDGE_CURVE('',#21353,#21352,#3019,.T.);
#26403=EDGE_CURVE('',#21354,#21353,#3020,.T.);
#26404=EDGE_CURVE('',#21355,#21354,#3021,.T.);
#26405=EDGE_CURVE('',#21356,#21355,#3022,.T.);
#26406=EDGE_CURVE('',#21357,#21356,#3023,.T.);
#26407=EDGE_CURVE('',#21358,#21357,#3024,.T.);
#26408=EDGE_CURVE('',#21359,#21358,#3025,.T.);
#26409=EDGE_CURVE('',#21360,#21359,#3026,.T.);
#26410=EDGE_CURVE('',#21361,#21360,#3027,.T.);
#26411=EDGE_CURVE('',#21362,#21361,#3028,.T.);
#26412=EDGE_CURVE('',#21363,#21362,#3029,.T.);
#26413=EDGE_CURVE('',#21364,#21363,#3030,.T.);
#26414=EDGE_CURVE('',#21365,#21364,#3031,.T.);
#26415=EDGE_CURVE('',#21366,#21365,#3032,.T.);
#26416=EDGE_CURVE('',#21366,#21367,#18858,.T.);
#26417=EDGE_CURVE('',#21368,#21367,#3033,.T.);
#26418=EDGE_CURVE('',#21369,#21368,#3034,.T.);
#26419=EDGE_CURVE('',#21370,#21369,#3035,.T.);
#26420=EDGE_CURVE('',#21371,#21370,#3036,.T.);
#26421=EDGE_CURVE('',#21372,#21371,#3037,.T.);
#26422=EDGE_CURVE('',#21373,#21372,#3038,.T.);
#26423=EDGE_CURVE('',#21374,#21373,#3039,.T.);
#26424=EDGE_CURVE('',#21375,#21374,#3040,.T.);
#26425=EDGE_CURVE('',#21376,#21375,#3041,.T.);
#26426=EDGE_CURVE('',#21377,#21376,#3042,.T.);
#26427=EDGE_CURVE('',#21378,#21377,#3043,.T.);
#26428=EDGE_CURVE('',#21379,#21378,#3044,.T.);
#26429=EDGE_CURVE('',#21380,#21379,#3045,.T.);
#26430=EDGE_CURVE('',#21381,#21380,#3046,.T.);
#26431=EDGE_CURVE('',#20363,#21381,#3047,.T.);
#26432=EDGE_CURVE('',#20360,#21382,#3048,.T.);
#26433=EDGE_CURVE('',#21382,#21383,#3049,.T.);
#26434=EDGE_CURVE('',#21384,#21383,#18859,.T.);
#26435=EDGE_CURVE('',#21385,#21384,#1314,.T.);
#26436=EDGE_CURVE('',#21352,#21385,#3050,.T.);
#26437=EDGE_CURVE('',#21386,#20358,#3051,.T.);
#26438=EDGE_CURVE('',#21387,#21386,#3052,.T.);
#26439=EDGE_CURVE('',#21388,#21387,#3053,.T.);
#26440=EDGE_CURVE('',#21389,#21388,#3054,.T.);
#26441=EDGE_CURVE('',#21390,#21389,#3055,.T.);
#26442=EDGE_CURVE('',#21391,#21390,#3056,.T.);
#26443=EDGE_CURVE('',#21392,#21391,#3057,.T.);
#26444=EDGE_CURVE('',#21393,#21392,#3058,.T.);
#26445=EDGE_CURVE('',#21394,#21393,#3059,.T.);
#26446=EDGE_CURVE('',#21395,#21394,#3060,.T.);
#26447=EDGE_CURVE('',#21396,#21395,#3061,.T.);
#26448=EDGE_CURVE('',#21397,#21396,#3062,.T.);
#26449=EDGE_CURVE('',#21398,#21397,#3063,.T.);
#26450=EDGE_CURVE('',#21399,#21398,#3064,.T.);
#26451=EDGE_CURVE('',#21400,#21399,#3065,.T.);
#26452=EDGE_CURVE('',#21400,#21401,#18860,.T.);
#26453=EDGE_CURVE('',#21402,#21401,#3066,.T.);
#26454=EDGE_CURVE('',#21403,#21402,#3067,.T.);
#26455=EDGE_CURVE('',#21404,#21403,#3068,.T.);
#26456=EDGE_CURVE('',#21405,#21404,#3069,.T.);
#26457=EDGE_CURVE('',#21406,#21405,#3070,.T.);
#26458=EDGE_CURVE('',#21407,#21406,#3071,.T.);
#26459=EDGE_CURVE('',#21408,#21407,#3072,.T.);
#26460=EDGE_CURVE('',#21409,#21408,#3073,.T.);
#26461=EDGE_CURVE('',#21410,#21409,#3074,.T.);
#26462=EDGE_CURVE('',#21411,#21410,#3075,.T.);
#26463=EDGE_CURVE('',#21412,#21411,#3076,.T.);
#26464=EDGE_CURVE('',#21413,#21412,#3077,.T.);
#26465=EDGE_CURVE('',#21414,#21413,#3078,.T.);
#26466=EDGE_CURVE('',#21415,#21414,#3079,.T.);
#26467=EDGE_CURVE('',#20359,#21415,#3080,.T.);
#26468=EDGE_CURVE('',#20356,#21416,#3081,.T.);
#26469=EDGE_CURVE('',#21416,#21417,#3082,.T.);
#26470=EDGE_CURVE('',#21418,#21417,#18861,.T.);
#26471=EDGE_CURVE('',#21419,#21418,#1315,.T.);
#26472=EDGE_CURVE('',#21386,#21419,#3083,.T.);
#26473=EDGE_CURVE('',#21420,#20354,#3084,.T.);
#26474=EDGE_CURVE('',#21421,#21420,#3085,.T.);
#26475=EDGE_CURVE('',#21422,#21421,#3086,.T.);
#26476=EDGE_CURVE('',#21423,#21422,#3087,.T.);
#26477=EDGE_CURVE('',#21424,#21423,#3088,.T.);
#26478=EDGE_CURVE('',#21425,#21424,#3089,.T.);
#26479=EDGE_CURVE('',#21426,#21425,#3090,.T.);
#26480=EDGE_CURVE('',#21427,#21426,#3091,.T.);
#26481=EDGE_CURVE('',#21428,#21427,#3092,.T.);
#26482=EDGE_CURVE('',#21429,#21428,#3093,.T.);
#26483=EDGE_CURVE('',#21430,#21429,#3094,.T.);
#26484=EDGE_CURVE('',#21431,#21430,#3095,.T.);
#26485=EDGE_CURVE('',#21432,#21431,#3096,.T.);
#26486=EDGE_CURVE('',#21433,#21432,#3097,.T.);
#26487=EDGE_CURVE('',#21434,#21433,#3098,.T.);
#26488=EDGE_CURVE('',#21434,#21435,#18862,.T.);
#26489=EDGE_CURVE('',#21436,#21435,#3099,.T.);
#26490=EDGE_CURVE('',#21437,#21436,#3100,.T.);
#26491=EDGE_CURVE('',#21438,#21437,#3101,.T.);
#26492=EDGE_CURVE('',#21439,#21438,#3102,.T.);
#26493=EDGE_CURVE('',#21440,#21439,#3103,.T.);
#26494=EDGE_CURVE('',#21441,#21440,#3104,.T.);
#26495=EDGE_CURVE('',#21442,#21441,#3105,.T.);
#26496=EDGE_CURVE('',#21443,#21442,#3106,.T.);
#26497=EDGE_CURVE('',#21444,#21443,#3107,.T.);
#26498=EDGE_CURVE('',#21445,#21444,#3108,.T.);
#26499=EDGE_CURVE('',#21446,#21445,#3109,.T.);
#26500=EDGE_CURVE('',#21447,#21446,#3110,.T.);
#26501=EDGE_CURVE('',#21448,#21447,#3111,.T.);
#26502=EDGE_CURVE('',#21449,#21448,#3112,.T.);
#26503=EDGE_CURVE('',#20355,#21449,#3113,.T.);
#26504=EDGE_CURVE('',#20352,#21450,#3114,.T.);
#26505=EDGE_CURVE('',#21450,#21451,#3115,.T.);
#26506=EDGE_CURVE('',#21452,#21451,#18863,.T.);
#26507=EDGE_CURVE('',#21453,#21452,#1316,.T.);
#26508=EDGE_CURVE('',#21420,#21453,#3116,.T.);
#26509=EDGE_CURVE('',#21454,#20350,#3117,.T.);
#26510=EDGE_CURVE('',#21455,#21454,#3118,.T.);
#26511=EDGE_CURVE('',#21456,#21455,#3119,.T.);
#26512=EDGE_CURVE('',#21457,#21456,#3120,.T.);
#26513=EDGE_CURVE('',#21458,#21457,#3121,.T.);
#26514=EDGE_CURVE('',#21459,#21458,#3122,.T.);
#26515=EDGE_CURVE('',#21460,#21459,#3123,.T.);
#26516=EDGE_CURVE('',#21461,#21460,#3124,.T.);
#26517=EDGE_CURVE('',#21462,#21461,#3125,.T.);
#26518=EDGE_CURVE('',#21463,#21462,#3126,.T.);
#26519=EDGE_CURVE('',#21464,#21463,#3127,.T.);
#26520=EDGE_CURVE('',#21465,#21464,#3128,.T.);
#26521=EDGE_CURVE('',#21466,#21465,#3129,.T.);
#26522=EDGE_CURVE('',#21467,#21466,#3130,.T.);
#26523=EDGE_CURVE('',#21468,#21467,#3131,.T.);
#26524=EDGE_CURVE('',#21468,#21469,#18864,.T.);
#26525=EDGE_CURVE('',#21470,#21469,#3132,.T.);
#26526=EDGE_CURVE('',#21471,#21470,#3133,.T.);
#26527=EDGE_CURVE('',#21472,#21471,#3134,.T.);
#26528=EDGE_CURVE('',#21473,#21472,#3135,.T.);
#26529=EDGE_CURVE('',#21474,#21473,#3136,.T.);
#26530=EDGE_CURVE('',#21475,#21474,#3137,.T.);
#26531=EDGE_CURVE('',#21476,#21475,#3138,.T.);
#26532=EDGE_CURVE('',#21477,#21476,#3139,.T.);
#26533=EDGE_CURVE('',#21478,#21477,#3140,.T.);
#26534=EDGE_CURVE('',#21479,#21478,#3141,.T.);
#26535=EDGE_CURVE('',#21480,#21479,#3142,.T.);
#26536=EDGE_CURVE('',#21481,#21480,#3143,.T.);
#26537=EDGE_CURVE('',#21482,#21481,#3144,.T.);
#26538=EDGE_CURVE('',#21483,#21482,#3145,.T.);
#26539=EDGE_CURVE('',#20351,#21483,#3146,.T.);
#26540=EDGE_CURVE('',#20348,#21484,#3147,.T.);
#26541=EDGE_CURVE('',#21484,#21485,#3148,.T.);
#26542=EDGE_CURVE('',#21486,#21485,#18865,.T.);
#26543=EDGE_CURVE('',#21487,#21486,#1317,.T.);
#26544=EDGE_CURVE('',#21454,#21487,#3149,.T.);
#26545=EDGE_CURVE('',#21488,#20346,#3150,.T.);
#26546=EDGE_CURVE('',#21489,#21488,#3151,.T.);
#26547=EDGE_CURVE('',#21490,#21489,#3152,.T.);
#26548=EDGE_CURVE('',#21491,#21490,#3153,.T.);
#26549=EDGE_CURVE('',#21492,#21491,#3154,.T.);
#26550=EDGE_CURVE('',#21493,#21492,#3155,.T.);
#26551=EDGE_CURVE('',#21494,#21493,#3156,.T.);
#26552=EDGE_CURVE('',#21495,#21494,#3157,.T.);
#26553=EDGE_CURVE('',#21496,#21495,#3158,.T.);
#26554=EDGE_CURVE('',#21497,#21496,#3159,.T.);
#26555=EDGE_CURVE('',#21498,#21497,#3160,.T.);
#26556=EDGE_CURVE('',#21499,#21498,#3161,.T.);
#26557=EDGE_CURVE('',#21500,#21499,#3162,.T.);
#26558=EDGE_CURVE('',#21501,#21500,#3163,.T.);
#26559=EDGE_CURVE('',#21502,#21501,#3164,.T.);
#26560=EDGE_CURVE('',#21502,#21503,#18866,.T.);
#26561=EDGE_CURVE('',#21504,#21503,#3165,.T.);
#26562=EDGE_CURVE('',#21505,#21504,#3166,.T.);
#26563=EDGE_CURVE('',#21506,#21505,#3167,.T.);
#26564=EDGE_CURVE('',#21507,#21506,#3168,.T.);
#26565=EDGE_CURVE('',#21508,#21507,#3169,.T.);
#26566=EDGE_CURVE('',#21509,#21508,#3170,.T.);
#26567=EDGE_CURVE('',#21510,#21509,#3171,.T.);
#26568=EDGE_CURVE('',#21511,#21510,#3172,.T.);
#26569=EDGE_CURVE('',#21512,#21511,#3173,.T.);
#26570=EDGE_CURVE('',#21513,#21512,#3174,.T.);
#26571=EDGE_CURVE('',#21514,#21513,#3175,.T.);
#26572=EDGE_CURVE('',#21515,#21514,#3176,.T.);
#26573=EDGE_CURVE('',#21516,#21515,#3177,.T.);
#26574=EDGE_CURVE('',#21517,#21516,#3178,.T.);
#26575=EDGE_CURVE('',#20347,#21517,#3179,.T.);
#26576=EDGE_CURVE('',#20344,#21518,#3180,.T.);
#26577=EDGE_CURVE('',#21518,#21519,#3181,.T.);
#26578=EDGE_CURVE('',#21520,#21519,#18867,.T.);
#26579=EDGE_CURVE('',#21521,#21520,#1318,.T.);
#26580=EDGE_CURVE('',#21488,#21521,#3182,.T.);
#26581=EDGE_CURVE('',#21522,#20342,#3183,.T.);
#26582=EDGE_CURVE('',#21523,#21522,#3184,.T.);
#26583=EDGE_CURVE('',#21524,#21523,#3185,.T.);
#26584=EDGE_CURVE('',#21525,#21524,#3186,.T.);
#26585=EDGE_CURVE('',#21526,#21525,#3187,.T.);
#26586=EDGE_CURVE('',#21527,#21526,#3188,.T.);
#26587=EDGE_CURVE('',#21528,#21527,#3189,.T.);
#26588=EDGE_CURVE('',#21529,#21528,#3190,.T.);
#26589=EDGE_CURVE('',#21530,#21529,#3191,.T.);
#26590=EDGE_CURVE('',#21531,#21530,#3192,.T.);
#26591=EDGE_CURVE('',#21532,#21531,#3193,.T.);
#26592=EDGE_CURVE('',#21533,#21532,#3194,.T.);
#26593=EDGE_CURVE('',#21534,#21533,#3195,.T.);
#26594=EDGE_CURVE('',#21535,#21534,#3196,.T.);
#26595=EDGE_CURVE('',#21536,#21535,#3197,.T.);
#26596=EDGE_CURVE('',#21536,#21537,#18868,.T.);
#26597=EDGE_CURVE('',#21538,#21537,#3198,.T.);
#26598=EDGE_CURVE('',#21539,#21538,#3199,.T.);
#26599=EDGE_CURVE('',#21540,#21539,#3200,.T.);
#26600=EDGE_CURVE('',#21541,#21540,#3201,.T.);
#26601=EDGE_CURVE('',#21542,#21541,#3202,.T.);
#26602=EDGE_CURVE('',#21543,#21542,#3203,.T.);
#26603=EDGE_CURVE('',#21544,#21543,#3204,.T.);
#26604=EDGE_CURVE('',#21545,#21544,#3205,.T.);
#26605=EDGE_CURVE('',#21546,#21545,#3206,.T.);
#26606=EDGE_CURVE('',#21547,#21546,#3207,.T.);
#26607=EDGE_CURVE('',#21548,#21547,#3208,.T.);
#26608=EDGE_CURVE('',#21549,#21548,#3209,.T.);
#26609=EDGE_CURVE('',#21550,#21549,#3210,.T.);
#26610=EDGE_CURVE('',#21551,#21550,#3211,.T.);
#26611=EDGE_CURVE('',#20343,#21551,#3212,.T.);
#26612=EDGE_CURVE('',#20340,#21552,#3213,.T.);
#26613=EDGE_CURVE('',#21552,#21553,#3214,.T.);
#26614=EDGE_CURVE('',#21554,#21553,#18869,.T.);
#26615=EDGE_CURVE('',#21555,#21554,#1319,.T.);
#26616=EDGE_CURVE('',#21522,#21555,#3215,.T.);
#26617=EDGE_CURVE('',#21556,#20338,#3216,.T.);
#26618=EDGE_CURVE('',#21557,#21556,#3217,.T.);
#26619=EDGE_CURVE('',#21558,#21557,#3218,.T.);
#26620=EDGE_CURVE('',#21559,#21558,#3219,.T.);
#26621=EDGE_CURVE('',#21560,#21559,#3220,.T.);
#26622=EDGE_CURVE('',#21561,#21560,#3221,.T.);
#26623=EDGE_CURVE('',#21562,#21561,#3222,.T.);
#26624=EDGE_CURVE('',#21563,#21562,#3223,.T.);
#26625=EDGE_CURVE('',#21564,#21563,#3224,.T.);
#26626=EDGE_CURVE('',#21565,#21564,#3225,.T.);
#26627=EDGE_CURVE('',#21566,#21565,#3226,.T.);
#26628=EDGE_CURVE('',#21567,#21566,#3227,.T.);
#26629=EDGE_CURVE('',#21568,#21567,#3228,.T.);
#26630=EDGE_CURVE('',#21569,#21568,#3229,.T.);
#26631=EDGE_CURVE('',#21570,#21569,#3230,.T.);
#26632=EDGE_CURVE('',#21570,#21571,#18870,.T.);
#26633=EDGE_CURVE('',#21572,#21571,#3231,.T.);
#26634=EDGE_CURVE('',#21573,#21572,#3232,.T.);
#26635=EDGE_CURVE('',#21574,#21573,#3233,.T.);
#26636=EDGE_CURVE('',#21575,#21574,#3234,.T.);
#26637=EDGE_CURVE('',#21576,#21575,#3235,.T.);
#26638=EDGE_CURVE('',#21577,#21576,#3236,.T.);
#26639=EDGE_CURVE('',#21578,#21577,#3237,.T.);
#26640=EDGE_CURVE('',#21579,#21578,#3238,.T.);
#26641=EDGE_CURVE('',#21580,#21579,#3239,.T.);
#26642=EDGE_CURVE('',#21581,#21580,#3240,.T.);
#26643=EDGE_CURVE('',#21582,#21581,#3241,.T.);
#26644=EDGE_CURVE('',#21583,#21582,#3242,.T.);
#26645=EDGE_CURVE('',#21584,#21583,#3243,.T.);
#26646=EDGE_CURVE('',#21585,#21584,#3244,.T.);
#26647=EDGE_CURVE('',#20339,#21585,#3245,.T.);
#26648=EDGE_CURVE('',#20336,#21586,#3246,.T.);
#26649=EDGE_CURVE('',#21586,#21587,#3247,.T.);
#26650=EDGE_CURVE('',#21588,#21587,#18871,.T.);
#26651=EDGE_CURVE('',#21589,#21588,#1320,.T.);
#26652=EDGE_CURVE('',#21556,#21589,#3248,.T.);
#26653=EDGE_CURVE('',#21590,#20334,#3249,.T.);
#26654=EDGE_CURVE('',#21591,#21590,#3250,.T.);
#26655=EDGE_CURVE('',#21592,#21591,#3251,.T.);
#26656=EDGE_CURVE('',#21593,#21592,#3252,.T.);
#26657=EDGE_CURVE('',#21594,#21593,#3253,.T.);
#26658=EDGE_CURVE('',#21595,#21594,#3254,.T.);
#26659=EDGE_CURVE('',#21596,#21595,#3255,.T.);
#26660=EDGE_CURVE('',#21597,#21596,#3256,.T.);
#26661=EDGE_CURVE('',#21598,#21597,#3257,.T.);
#26662=EDGE_CURVE('',#21599,#21598,#3258,.T.);
#26663=EDGE_CURVE('',#21600,#21599,#3259,.T.);
#26664=EDGE_CURVE('',#21601,#21600,#3260,.T.);
#26665=EDGE_CURVE('',#21602,#21601,#3261,.T.);
#26666=EDGE_CURVE('',#21603,#21602,#3262,.T.);
#26667=EDGE_CURVE('',#21604,#21603,#3263,.T.);
#26668=EDGE_CURVE('',#21604,#21605,#18872,.T.);
#26669=EDGE_CURVE('',#21606,#21605,#3264,.T.);
#26670=EDGE_CURVE('',#21607,#21606,#3265,.T.);
#26671=EDGE_CURVE('',#21608,#21607,#3266,.T.);
#26672=EDGE_CURVE('',#21609,#21608,#3267,.T.);
#26673=EDGE_CURVE('',#21610,#21609,#3268,.T.);
#26674=EDGE_CURVE('',#21611,#21610,#3269,.T.);
#26675=EDGE_CURVE('',#21612,#21611,#3270,.T.);
#26676=EDGE_CURVE('',#21613,#21612,#3271,.T.);
#26677=EDGE_CURVE('',#21614,#21613,#3272,.T.);
#26678=EDGE_CURVE('',#21615,#21614,#3273,.T.);
#26679=EDGE_CURVE('',#21616,#21615,#3274,.T.);
#26680=EDGE_CURVE('',#21617,#21616,#3275,.T.);
#26681=EDGE_CURVE('',#21618,#21617,#3276,.T.);
#26682=EDGE_CURVE('',#21619,#21618,#3277,.T.);
#26683=EDGE_CURVE('',#20335,#21619,#3278,.T.);
#26684=EDGE_CURVE('',#20332,#21620,#3279,.T.);
#26685=EDGE_CURVE('',#21620,#21621,#3280,.T.);
#26686=EDGE_CURVE('',#21622,#21621,#18873,.T.);
#26687=EDGE_CURVE('',#21623,#21622,#1321,.T.);
#26688=EDGE_CURVE('',#21590,#21623,#3281,.T.);
#26689=EDGE_CURVE('',#21624,#20330,#3282,.T.);
#26690=EDGE_CURVE('',#21625,#21624,#3283,.T.);
#26691=EDGE_CURVE('',#21626,#21625,#3284,.T.);
#26692=EDGE_CURVE('',#21627,#21626,#3285,.T.);
#26693=EDGE_CURVE('',#21628,#21627,#3286,.T.);
#26694=EDGE_CURVE('',#21629,#21628,#3287,.T.);
#26695=EDGE_CURVE('',#21630,#21629,#3288,.T.);
#26696=EDGE_CURVE('',#21631,#21630,#3289,.T.);
#26697=EDGE_CURVE('',#21632,#21631,#3290,.T.);
#26698=EDGE_CURVE('',#21633,#21632,#3291,.T.);
#26699=EDGE_CURVE('',#21634,#21633,#3292,.T.);
#26700=EDGE_CURVE('',#21635,#21634,#3293,.T.);
#26701=EDGE_CURVE('',#21636,#21635,#3294,.T.);
#26702=EDGE_CURVE('',#21637,#21636,#3295,.T.);
#26703=EDGE_CURVE('',#21638,#21637,#3296,.T.);
#26704=EDGE_CURVE('',#21638,#21639,#18874,.T.);
#26705=EDGE_CURVE('',#21640,#21639,#3297,.T.);
#26706=EDGE_CURVE('',#21641,#21640,#3298,.T.);
#26707=EDGE_CURVE('',#21642,#21641,#3299,.T.);
#26708=EDGE_CURVE('',#21643,#21642,#3300,.T.);
#26709=EDGE_CURVE('',#21644,#21643,#3301,.T.);
#26710=EDGE_CURVE('',#21645,#21644,#3302,.T.);
#26711=EDGE_CURVE('',#21646,#21645,#3303,.T.);
#26712=EDGE_CURVE('',#21647,#21646,#3304,.T.);
#26713=EDGE_CURVE('',#21648,#21647,#3305,.T.);
#26714=EDGE_CURVE('',#21649,#21648,#3306,.T.);
#26715=EDGE_CURVE('',#21650,#21649,#3307,.T.);
#26716=EDGE_CURVE('',#21651,#21650,#3308,.T.);
#26717=EDGE_CURVE('',#21652,#21651,#3309,.T.);
#26718=EDGE_CURVE('',#21653,#21652,#3310,.T.);
#26719=EDGE_CURVE('',#20331,#21653,#3311,.T.);
#26720=EDGE_CURVE('',#20328,#21654,#3312,.T.);
#26721=EDGE_CURVE('',#21654,#21655,#3313,.T.);
#26722=EDGE_CURVE('',#21656,#21655,#18875,.T.);
#26723=EDGE_CURVE('',#21657,#21656,#1322,.T.);
#26724=EDGE_CURVE('',#21624,#21657,#3314,.T.);
#26725=EDGE_CURVE('',#21658,#20326,#3315,.T.);
#26726=EDGE_CURVE('',#21659,#21658,#3316,.T.);
#26727=EDGE_CURVE('',#21660,#21659,#3317,.T.);
#26728=EDGE_CURVE('',#21661,#21660,#3318,.T.);
#26729=EDGE_CURVE('',#21662,#21661,#3319,.T.);
#26730=EDGE_CURVE('',#21663,#21662,#3320,.T.);
#26731=EDGE_CURVE('',#21664,#21663,#3321,.T.);
#26732=EDGE_CURVE('',#21665,#21664,#3322,.T.);
#26733=EDGE_CURVE('',#21666,#21665,#3323,.T.);
#26734=EDGE_CURVE('',#21667,#21666,#3324,.T.);
#26735=EDGE_CURVE('',#21668,#21667,#3325,.T.);
#26736=EDGE_CURVE('',#21669,#21668,#3326,.T.);
#26737=EDGE_CURVE('',#21670,#21669,#3327,.T.);
#26738=EDGE_CURVE('',#21671,#21670,#3328,.T.);
#26739=EDGE_CURVE('',#21672,#21671,#3329,.T.);
#26740=EDGE_CURVE('',#21672,#21673,#18876,.T.);
#26741=EDGE_CURVE('',#21674,#21673,#3330,.T.);
#26742=EDGE_CURVE('',#21675,#21674,#3331,.T.);
#26743=EDGE_CURVE('',#21676,#21675,#3332,.T.);
#26744=EDGE_CURVE('',#21677,#21676,#3333,.T.);
#26745=EDGE_CURVE('',#21678,#21677,#3334,.T.);
#26746=EDGE_CURVE('',#21679,#21678,#3335,.T.);
#26747=EDGE_CURVE('',#21680,#21679,#3336,.T.);
#26748=EDGE_CURVE('',#21681,#21680,#3337,.T.);
#26749=EDGE_CURVE('',#21682,#21681,#3338,.T.);
#26750=EDGE_CURVE('',#21683,#21682,#3339,.T.);
#26751=EDGE_CURVE('',#21684,#21683,#3340,.T.);
#26752=EDGE_CURVE('',#21685,#21684,#3341,.T.);
#26753=EDGE_CURVE('',#21686,#21685,#3342,.T.);
#26754=EDGE_CURVE('',#21687,#21686,#3343,.T.);
#26755=EDGE_CURVE('',#20327,#21687,#3344,.T.);
#26756=EDGE_CURVE('',#20324,#21688,#3345,.T.);
#26757=EDGE_CURVE('',#21688,#21689,#3346,.T.);
#26758=EDGE_CURVE('',#21690,#21689,#18877,.T.);
#26759=EDGE_CURVE('',#21691,#21690,#1323,.T.);
#26760=EDGE_CURVE('',#21658,#21691,#3347,.T.);
#26761=EDGE_CURVE('',#21692,#21693,#19610,.T.);
#26762=EDGE_CURVE('',#21673,#21692,#18878,.T.);
#26763=EDGE_CURVE('',#21693,#21672,#18879,.T.);
#26764=EDGE_CURVE('',#21694,#21695,#19611,.T.);
#26765=EDGE_CURVE('',#21639,#21694,#18880,.T.);
#26766=EDGE_CURVE('',#21695,#21638,#18881,.T.);
#26767=EDGE_CURVE('',#21696,#21697,#19612,.T.);
#26768=EDGE_CURVE('',#21605,#21696,#18882,.T.);
#26769=EDGE_CURVE('',#21697,#21604,#18883,.T.);
#26770=EDGE_CURVE('',#21698,#21699,#19613,.T.);
#26771=EDGE_CURVE('',#21571,#21698,#18884,.T.);
#26772=EDGE_CURVE('',#21699,#21570,#18885,.T.);
#26773=EDGE_CURVE('',#21700,#21701,#19614,.T.);
#26774=EDGE_CURVE('',#21537,#21700,#18886,.T.);
#26775=EDGE_CURVE('',#21701,#21536,#18887,.T.);
#26776=EDGE_CURVE('',#21702,#21703,#19615,.T.);
#26777=EDGE_CURVE('',#21503,#21702,#18888,.T.);
#26778=EDGE_CURVE('',#21703,#21502,#18889,.T.);
#26779=EDGE_CURVE('',#21704,#21705,#19616,.T.);
#26780=EDGE_CURVE('',#21469,#21704,#18890,.T.);
#26781=EDGE_CURVE('',#21705,#21468,#18891,.T.);
#26782=EDGE_CURVE('',#21706,#21707,#19617,.T.);
#26783=EDGE_CURVE('',#21435,#21706,#18892,.T.);
#26784=EDGE_CURVE('',#21707,#21434,#18893,.T.);
#26785=EDGE_CURVE('',#21708,#21709,#19618,.T.);
#26786=EDGE_CURVE('',#21401,#21708,#18894,.T.);
#26787=EDGE_CURVE('',#21709,#21400,#18895,.T.);
#26788=EDGE_CURVE('',#21710,#21711,#19619,.T.);
#26789=EDGE_CURVE('',#21367,#21710,#18896,.T.);
#26790=EDGE_CURVE('',#21711,#21366,#18897,.T.);
#26791=EDGE_CURVE('',#21712,#21713,#19620,.T.);
#26792=EDGE_CURVE('',#21333,#21712,#18898,.T.);
#26793=EDGE_CURVE('',#21713,#21332,#18899,.T.);
#26794=EDGE_CURVE('',#21714,#21715,#19621,.T.);
#26795=EDGE_CURVE('',#21299,#21714,#18900,.T.);
#26796=EDGE_CURVE('',#21715,#21298,#18901,.T.);
#26797=EDGE_CURVE('',#21716,#21717,#19622,.T.);
#26798=EDGE_CURVE('',#21265,#21716,#18902,.T.);
#26799=EDGE_CURVE('',#21717,#21264,#18903,.T.);
#26800=EDGE_CURVE('',#21718,#21719,#19623,.T.);
#26801=EDGE_CURVE('',#21231,#21718,#18904,.T.);
#26802=EDGE_CURVE('',#21719,#21230,#18905,.T.);
#26803=EDGE_CURVE('',#21720,#21721,#19624,.T.);
#26804=EDGE_CURVE('',#21197,#21720,#18906,.T.);
#26805=EDGE_CURVE('',#21721,#21196,#18907,.T.);
#26806=EDGE_CURVE('',#21722,#21723,#19625,.T.);
#26807=EDGE_CURVE('',#21163,#21722,#18908,.T.);
#26808=EDGE_CURVE('',#21723,#21162,#18909,.T.);
#26809=EDGE_CURVE('',#21724,#21725,#19626,.T.);
#26810=EDGE_CURVE('',#21129,#21724,#18910,.T.);
#26811=EDGE_CURVE('',#21725,#21128,#18911,.T.);
#26812=EDGE_CURVE('',#21726,#21727,#19627,.T.);
#26813=EDGE_CURVE('',#21095,#21726,#18912,.T.);
#26814=EDGE_CURVE('',#21727,#21094,#18913,.T.);
#26815=EDGE_CURVE('',#21728,#21729,#19628,.T.);
#26816=EDGE_CURVE('',#21061,#21728,#18914,.T.);
#26817=EDGE_CURVE('',#21729,#21060,#18915,.T.);
#26818=EDGE_CURVE('',#21730,#21731,#19629,.T.);
#26819=EDGE_CURVE('',#21027,#21730,#18916,.T.);
#26820=EDGE_CURVE('',#21731,#21026,#18917,.T.);
#26821=EDGE_CURVE('',#21732,#21733,#19630,.T.);
#26822=EDGE_CURVE('',#20993,#21732,#18918,.T.);
#26823=EDGE_CURVE('',#21733,#20992,#18919,.T.);
#26824=EDGE_CURVE('',#21734,#21735,#19631,.T.);
#26825=EDGE_CURVE('',#20959,#21734,#18920,.T.);
#26826=EDGE_CURVE('',#21735,#20958,#18921,.T.);
#26827=EDGE_CURVE('',#21736,#21737,#19632,.T.);
#26828=EDGE_CURVE('',#20925,#21736,#18922,.T.);
#26829=EDGE_CURVE('',#21737,#20924,#18923,.T.);
#26830=EDGE_CURVE('',#21738,#21739,#19633,.T.);
#26831=EDGE_CURVE('',#20891,#21738,#18924,.T.);
#26832=EDGE_CURVE('',#21739,#20890,#18925,.T.);
#26833=EDGE_CURVE('',#21740,#21741,#19634,.T.);
#26834=EDGE_CURVE('',#20857,#21740,#18926,.T.);
#26835=EDGE_CURVE('',#21741,#20856,#18927,.T.);
#26836=EDGE_CURVE('',#21742,#21743,#19635,.T.);
#26837=EDGE_CURVE('',#20823,#21742,#18928,.T.);
#26838=EDGE_CURVE('',#21743,#20822,#18929,.T.);
#26839=EDGE_CURVE('',#21744,#21745,#19636,.T.);
#26840=EDGE_CURVE('',#20789,#21744,#18930,.T.);
#26841=EDGE_CURVE('',#21745,#20788,#18931,.T.);
#26842=EDGE_CURVE('',#21746,#21747,#19637,.T.);
#26843=EDGE_CURVE('',#20755,#21746,#18932,.T.);
#26844=EDGE_CURVE('',#21747,#20754,#18933,.T.);
#26845=EDGE_CURVE('',#21748,#21749,#19638,.T.);
#26846=EDGE_CURVE('',#20721,#21748,#18934,.T.);
#26847=EDGE_CURVE('',#21749,#20720,#18935,.T.);
#26848=EDGE_CURVE('',#21750,#21751,#19639,.T.);
#26849=EDGE_CURVE('',#20687,#21750,#18936,.T.);
#26850=EDGE_CURVE('',#21751,#20686,#18937,.T.);
#26851=EDGE_CURVE('',#21752,#21753,#19640,.T.);
#26852=EDGE_CURVE('',#20653,#21752,#18938,.T.);
#26853=EDGE_CURVE('',#21753,#20652,#18939,.T.);
#26854=EDGE_CURVE('',#21754,#21755,#19641,.T.);
#26855=EDGE_CURVE('',#20619,#21754,#18940,.T.);
#26856=EDGE_CURVE('',#21755,#20618,#18941,.T.);
#26857=EDGE_CURVE('',#21756,#21757,#19642,.T.);
#26858=EDGE_CURVE('',#20585,#21756,#18942,.T.);
#26859=EDGE_CURVE('',#21757,#20584,#18943,.T.);
#26860=EDGE_CURVE('',#21758,#21759,#19643,.T.);
#26861=EDGE_CURVE('',#20551,#21758,#18944,.T.);
#26862=EDGE_CURVE('',#21759,#20550,#18945,.T.);
#26863=EDGE_CURVE('',#21760,#21761,#19644,.T.);
#26864=EDGE_CURVE('',#20517,#21760,#18946,.T.);
#26865=EDGE_CURVE('',#21761,#20516,#18947,.T.);
#26866=EDGE_CURVE('',#21762,#21763,#19645,.T.);
#26867=EDGE_CURVE('',#20483,#21762,#18948,.T.);
#26868=EDGE_CURVE('',#21763,#20482,#18949,.T.);
#26869=EDGE_CURVE('',#21762,#21764,#3348,.T.);
#26870=EDGE_CURVE('',#21764,#21765,#3349,.T.);
#26871=EDGE_CURVE('',#21766,#21765,#18950,.T.);
#26872=EDGE_CURVE('',#21767,#21766,#1324,.T.);
#26873=EDGE_CURVE('',#20484,#21767,#3350,.T.);
#26874=EDGE_CURVE('',#21760,#21768,#3351,.T.);
#26875=EDGE_CURVE('',#21768,#21769,#3352,.T.);
#26876=EDGE_CURVE('',#21770,#21769,#18951,.T.);
#26877=EDGE_CURVE('',#21771,#21770,#1325,.T.);
#26878=EDGE_CURVE('',#20518,#21771,#3353,.T.);
#26879=EDGE_CURVE('',#21758,#21772,#3354,.T.);
#26880=EDGE_CURVE('',#21772,#21773,#3355,.T.);
#26881=EDGE_CURVE('',#21774,#21773,#18952,.T.);
#26882=EDGE_CURVE('',#21775,#21774,#1326,.T.);
#26883=EDGE_CURVE('',#20552,#21775,#3356,.T.);
#26884=EDGE_CURVE('',#21756,#21776,#3357,.T.);
#26885=EDGE_CURVE('',#21776,#21777,#3358,.T.);
#26886=EDGE_CURVE('',#21778,#21777,#18953,.T.);
#26887=EDGE_CURVE('',#21779,#21778,#1327,.T.);
#26888=EDGE_CURVE('',#20586,#21779,#3359,.T.);
#26889=EDGE_CURVE('',#21754,#21780,#3360,.T.);
#26890=EDGE_CURVE('',#21780,#21781,#3361,.T.);
#26891=EDGE_CURVE('',#21782,#21781,#18954,.T.);
#26892=EDGE_CURVE('',#21783,#21782,#1328,.T.);
#26893=EDGE_CURVE('',#20620,#21783,#3362,.T.);
#26894=EDGE_CURVE('',#21752,#21784,#3363,.T.);
#26895=EDGE_CURVE('',#21784,#21785,#3364,.T.);
#26896=EDGE_CURVE('',#21786,#21785,#18955,.T.);
#26897=EDGE_CURVE('',#21787,#21786,#1329,.T.);
#26898=EDGE_CURVE('',#20654,#21787,#3365,.T.);
#26899=EDGE_CURVE('',#21750,#21788,#3366,.T.);
#26900=EDGE_CURVE('',#21788,#21789,#3367,.T.);
#26901=EDGE_CURVE('',#21790,#21789,#18956,.T.);
#26902=EDGE_CURVE('',#21791,#21790,#1330,.T.);
#26903=EDGE_CURVE('',#20688,#21791,#3368,.T.);
#26904=EDGE_CURVE('',#21748,#21792,#3369,.T.);
#26905=EDGE_CURVE('',#21792,#21793,#3370,.T.);
#26906=EDGE_CURVE('',#21794,#21793,#18957,.T.);
#26907=EDGE_CURVE('',#21795,#21794,#1331,.T.);
#26908=EDGE_CURVE('',#20722,#21795,#3371,.T.);
#26909=EDGE_CURVE('',#21746,#21796,#3372,.T.);
#26910=EDGE_CURVE('',#21796,#21797,#3373,.T.);
#26911=EDGE_CURVE('',#21798,#21797,#18958,.T.);
#26912=EDGE_CURVE('',#21799,#21798,#1332,.T.);
#26913=EDGE_CURVE('',#20756,#21799,#3374,.T.);
#26914=EDGE_CURVE('',#21744,#21800,#3375,.T.);
#26915=EDGE_CURVE('',#21800,#21801,#3376,.T.);
#26916=EDGE_CURVE('',#21802,#21801,#18959,.T.);
#26917=EDGE_CURVE('',#21803,#21802,#1333,.T.);
#26918=EDGE_CURVE('',#20790,#21803,#3377,.T.);
#26919=EDGE_CURVE('',#21742,#21804,#3378,.T.);
#26920=EDGE_CURVE('',#21804,#21805,#3379,.T.);
#26921=EDGE_CURVE('',#21806,#21805,#18960,.T.);
#26922=EDGE_CURVE('',#21807,#21806,#1334,.T.);
#26923=EDGE_CURVE('',#20824,#21807,#3380,.T.);
#26924=EDGE_CURVE('',#21740,#21808,#3381,.T.);
#26925=EDGE_CURVE('',#21808,#21809,#3382,.T.);
#26926=EDGE_CURVE('',#21810,#21809,#18961,.T.);
#26927=EDGE_CURVE('',#21811,#21810,#1335,.T.);
#26928=EDGE_CURVE('',#20858,#21811,#3383,.T.);
#26929=EDGE_CURVE('',#21738,#21812,#3384,.T.);
#26930=EDGE_CURVE('',#21812,#21813,#3385,.T.);
#26931=EDGE_CURVE('',#21814,#21813,#18962,.T.);
#26932=EDGE_CURVE('',#21815,#21814,#1336,.T.);
#26933=EDGE_CURVE('',#20892,#21815,#3386,.T.);
#26934=EDGE_CURVE('',#21736,#21816,#3387,.T.);
#26935=EDGE_CURVE('',#21816,#21817,#3388,.T.);
#26936=EDGE_CURVE('',#21818,#21817,#18963,.T.);
#26937=EDGE_CURVE('',#21819,#21818,#1337,.T.);
#26938=EDGE_CURVE('',#20926,#21819,#3389,.T.);
#26939=EDGE_CURVE('',#21734,#21820,#3390,.T.);
#26940=EDGE_CURVE('',#21820,#21821,#3391,.T.);
#26941=EDGE_CURVE('',#21822,#21821,#18964,.T.);
#26942=EDGE_CURVE('',#21823,#21822,#1338,.T.);
#26943=EDGE_CURVE('',#20960,#21823,#3392,.T.);
#26944=EDGE_CURVE('',#21732,#21824,#3393,.T.);
#26945=EDGE_CURVE('',#21824,#21825,#3394,.T.);
#26946=EDGE_CURVE('',#21826,#21825,#18965,.T.);
#26947=EDGE_CURVE('',#21827,#21826,#1339,.T.);
#26948=EDGE_CURVE('',#20994,#21827,#3395,.T.);
#26949=EDGE_CURVE('',#21730,#21828,#3396,.T.);
#26950=EDGE_CURVE('',#21828,#21829,#3397,.T.);
#26951=EDGE_CURVE('',#21830,#21829,#18966,.T.);
#26952=EDGE_CURVE('',#21831,#21830,#1340,.T.);
#26953=EDGE_CURVE('',#21028,#21831,#3398,.T.);
#26954=EDGE_CURVE('',#21728,#21832,#3399,.T.);
#26955=EDGE_CURVE('',#21832,#21833,#3400,.T.);
#26956=EDGE_CURVE('',#21834,#21833,#18967,.T.);
#26957=EDGE_CURVE('',#21835,#21834,#1341,.T.);
#26958=EDGE_CURVE('',#21062,#21835,#3401,.T.);
#26959=EDGE_CURVE('',#21726,#21836,#3402,.T.);
#26960=EDGE_CURVE('',#21836,#21837,#3403,.T.);
#26961=EDGE_CURVE('',#21838,#21837,#18968,.T.);
#26962=EDGE_CURVE('',#21839,#21838,#1342,.T.);
#26963=EDGE_CURVE('',#21096,#21839,#3404,.T.);
#26964=EDGE_CURVE('',#21724,#21840,#3405,.T.);
#26965=EDGE_CURVE('',#21840,#21841,#3406,.T.);
#26966=EDGE_CURVE('',#21842,#21841,#18969,.T.);
#26967=EDGE_CURVE('',#21843,#21842,#1343,.T.);
#26968=EDGE_CURVE('',#21130,#21843,#3407,.T.);
#26969=EDGE_CURVE('',#21722,#21844,#3408,.T.);
#26970=EDGE_CURVE('',#21844,#21845,#3409,.T.);
#26971=EDGE_CURVE('',#21846,#21845,#18970,.T.);
#26972=EDGE_CURVE('',#21847,#21846,#1344,.T.);
#26973=EDGE_CURVE('',#21164,#21847,#3410,.T.);
#26974=EDGE_CURVE('',#21720,#21848,#3411,.T.);
#26975=EDGE_CURVE('',#21848,#21849,#3412,.T.);
#26976=EDGE_CURVE('',#21850,#21849,#18971,.T.);
#26977=EDGE_CURVE('',#21851,#21850,#1345,.T.);
#26978=EDGE_CURVE('',#21198,#21851,#3413,.T.);
#26979=EDGE_CURVE('',#21718,#21852,#3414,.T.);
#26980=EDGE_CURVE('',#21852,#21853,#3415,.T.);
#26981=EDGE_CURVE('',#21854,#21853,#18972,.T.);
#26982=EDGE_CURVE('',#21855,#21854,#1346,.T.);
#26983=EDGE_CURVE('',#21232,#21855,#3416,.T.);
#26984=EDGE_CURVE('',#21716,#21856,#3417,.T.);
#26985=EDGE_CURVE('',#21856,#21857,#3418,.T.);
#26986=EDGE_CURVE('',#21858,#21857,#18973,.T.);
#26987=EDGE_CURVE('',#21859,#21858,#1347,.T.);
#26988=EDGE_CURVE('',#21266,#21859,#3419,.T.);
#26989=EDGE_CURVE('',#21714,#21860,#3420,.T.);
#26990=EDGE_CURVE('',#21860,#21861,#3421,.T.);
#26991=EDGE_CURVE('',#21862,#21861,#18974,.T.);
#26992=EDGE_CURVE('',#21863,#21862,#1348,.T.);
#26993=EDGE_CURVE('',#21300,#21863,#3422,.T.);
#26994=EDGE_CURVE('',#21712,#21864,#3423,.T.);
#26995=EDGE_CURVE('',#21864,#21865,#3424,.T.);
#26996=EDGE_CURVE('',#21866,#21865,#18975,.T.);
#26997=EDGE_CURVE('',#21867,#21866,#1349,.T.);
#26998=EDGE_CURVE('',#21334,#21867,#3425,.T.);
#26999=EDGE_CURVE('',#21710,#21868,#3426,.T.);
#27000=EDGE_CURVE('',#21868,#21869,#3427,.T.);
#27001=EDGE_CURVE('',#21870,#21869,#18976,.T.);
#27002=EDGE_CURVE('',#21871,#21870,#1350,.T.);
#27003=EDGE_CURVE('',#21368,#21871,#3428,.T.);
#27004=EDGE_CURVE('',#21708,#21872,#3429,.T.);
#27005=EDGE_CURVE('',#21872,#21873,#3430,.T.);
#27006=EDGE_CURVE('',#21874,#21873,#18977,.T.);
#27007=EDGE_CURVE('',#21875,#21874,#1351,.T.);
#27008=EDGE_CURVE('',#21402,#21875,#3431,.T.);
#27009=EDGE_CURVE('',#21706,#21876,#3432,.T.);
#27010=EDGE_CURVE('',#21876,#21877,#3433,.T.);
#27011=EDGE_CURVE('',#21878,#21877,#18978,.T.);
#27012=EDGE_CURVE('',#21879,#21878,#1352,.T.);
#27013=EDGE_CURVE('',#21436,#21879,#3434,.T.);
#27014=EDGE_CURVE('',#21704,#21880,#3435,.T.);
#27015=EDGE_CURVE('',#21880,#21881,#3436,.T.);
#27016=EDGE_CURVE('',#21882,#21881,#18979,.T.);
#27017=EDGE_CURVE('',#21883,#21882,#1353,.T.);
#27018=EDGE_CURVE('',#21470,#21883,#3437,.T.);
#27019=EDGE_CURVE('',#21702,#21884,#3438,.T.);
#27020=EDGE_CURVE('',#21884,#21885,#3439,.T.);
#27021=EDGE_CURVE('',#21886,#21885,#18980,.T.);
#27022=EDGE_CURVE('',#21887,#21886,#1354,.T.);
#27023=EDGE_CURVE('',#21504,#21887,#3440,.T.);
#27024=EDGE_CURVE('',#21700,#21888,#3441,.T.);
#27025=EDGE_CURVE('',#21888,#21889,#3442,.T.);
#27026=EDGE_CURVE('',#21890,#21889,#18981,.T.);
#27027=EDGE_CURVE('',#21891,#21890,#1355,.T.);
#27028=EDGE_CURVE('',#21538,#21891,#3443,.T.);
#27029=EDGE_CURVE('',#21698,#21892,#3444,.T.);
#27030=EDGE_CURVE('',#21892,#21893,#3445,.T.);
#27031=EDGE_CURVE('',#21894,#21893,#18982,.T.);
#27032=EDGE_CURVE('',#21895,#21894,#1356,.T.);
#27033=EDGE_CURVE('',#21572,#21895,#3446,.T.);
#27034=EDGE_CURVE('',#21696,#21896,#3447,.T.);
#27035=EDGE_CURVE('',#21896,#21897,#3448,.T.);
#27036=EDGE_CURVE('',#21898,#21897,#18983,.T.);
#27037=EDGE_CURVE('',#21899,#21898,#1357,.T.);
#27038=EDGE_CURVE('',#21606,#21899,#3449,.T.);
#27039=EDGE_CURVE('',#21694,#21900,#3450,.T.);
#27040=EDGE_CURVE('',#21900,#21901,#3451,.T.);
#27041=EDGE_CURVE('',#21902,#21901,#18984,.T.);
#27042=EDGE_CURVE('',#21903,#21902,#1358,.T.);
#27043=EDGE_CURVE('',#21640,#21903,#3452,.T.);
#27044=EDGE_CURVE('',#21692,#21904,#3453,.T.);
#27045=EDGE_CURVE('',#21904,#21905,#3454,.T.);
#27046=EDGE_CURVE('',#21906,#21905,#18985,.T.);
#27047=EDGE_CURVE('',#21907,#21906,#1359,.T.);
#27048=EDGE_CURVE('',#21674,#21907,#3455,.T.);
#27049=EDGE_CURVE('',#21908,#20465,#3456,.T.);
#27050=EDGE_CURVE('',#20498,#21908,#3457,.T.);
#27051=EDGE_CURVE('',#21909,#20461,#3458,.T.);
#27052=EDGE_CURVE('',#20532,#21909,#3459,.T.);
#27053=EDGE_CURVE('',#21910,#20457,#3460,.T.);
#27054=EDGE_CURVE('',#20566,#21910,#3461,.T.);
#27055=EDGE_CURVE('',#21911,#20453,#3462,.T.);
#27056=EDGE_CURVE('',#20600,#21911,#3463,.T.);
#27057=EDGE_CURVE('',#21912,#20449,#3464,.T.);
#27058=EDGE_CURVE('',#20634,#21912,#3465,.T.);
#27059=EDGE_CURVE('',#21913,#20445,#3466,.T.);
#27060=EDGE_CURVE('',#20668,#21913,#3467,.T.);
#27061=EDGE_CURVE('',#21914,#20441,#3468,.T.);
#27062=EDGE_CURVE('',#20702,#21914,#3469,.T.);
#27063=EDGE_CURVE('',#21915,#20437,#3470,.T.);
#27064=EDGE_CURVE('',#20736,#21915,#3471,.T.);
#27065=EDGE_CURVE('',#21916,#20433,#3472,.T.);
#27066=EDGE_CURVE('',#20770,#21916,#3473,.T.);
#27067=EDGE_CURVE('',#21917,#20429,#3474,.T.);
#27068=EDGE_CURVE('',#20804,#21917,#3475,.T.);
#27069=EDGE_CURVE('',#21918,#20425,#3476,.T.);
#27070=EDGE_CURVE('',#20838,#21918,#3477,.T.);
#27071=EDGE_CURVE('',#21919,#20421,#3478,.T.);
#27072=EDGE_CURVE('',#20872,#21919,#3479,.T.);
#27073=EDGE_CURVE('',#21920,#20417,#3480,.T.);
#27074=EDGE_CURVE('',#20906,#21920,#3481,.T.);
#27075=EDGE_CURVE('',#21921,#20413,#3482,.T.);
#27076=EDGE_CURVE('',#20940,#21921,#3483,.T.);
#27077=EDGE_CURVE('',#21922,#20409,#3484,.T.);
#27078=EDGE_CURVE('',#20974,#21922,#3485,.T.);
#27079=EDGE_CURVE('',#21923,#20405,#3486,.T.);
#27080=EDGE_CURVE('',#21008,#21923,#3487,.T.);
#27081=EDGE_CURVE('',#21924,#20401,#3488,.T.);
#27082=EDGE_CURVE('',#21042,#21924,#3489,.T.);
#27083=EDGE_CURVE('',#21925,#20397,#3490,.T.);
#27084=EDGE_CURVE('',#21076,#21925,#3491,.T.);
#27085=EDGE_CURVE('',#21926,#20393,#3492,.T.);
#27086=EDGE_CURVE('',#21110,#21926,#3493,.T.);
#27087=EDGE_CURVE('',#21927,#20389,#3494,.T.);
#27088=EDGE_CURVE('',#21144,#21927,#3495,.T.);
#27089=EDGE_CURVE('',#21928,#20385,#3496,.T.);
#27090=EDGE_CURVE('',#21178,#21928,#3497,.T.);
#27091=EDGE_CURVE('',#21929,#20381,#3498,.T.);
#27092=EDGE_CURVE('',#21212,#21929,#3499,.T.);
#27093=EDGE_CURVE('',#21930,#20377,#3500,.T.);
#27094=EDGE_CURVE('',#21246,#21930,#3501,.T.);
#27095=EDGE_CURVE('',#21931,#20373,#3502,.T.);
#27096=EDGE_CURVE('',#21280,#21931,#3503,.T.);
#27097=EDGE_CURVE('',#21932,#20369,#3504,.T.);
#27098=EDGE_CURVE('',#21314,#21932,#3505,.T.);
#27099=EDGE_CURVE('',#21933,#20365,#3506,.T.);
#27100=EDGE_CURVE('',#21348,#21933,#3507,.T.);
#27101=EDGE_CURVE('',#21934,#20361,#3508,.T.);
#27102=EDGE_CURVE('',#21382,#21934,#3509,.T.);
#27103=EDGE_CURVE('',#21935,#20357,#3510,.T.);
#27104=EDGE_CURVE('',#21416,#21935,#3511,.T.);
#27105=EDGE_CURVE('',#21936,#20353,#3512,.T.);
#27106=EDGE_CURVE('',#21450,#21936,#3513,.T.);
#27107=EDGE_CURVE('',#21937,#20349,#3514,.T.);
#27108=EDGE_CURVE('',#21484,#21937,#3515,.T.);
#27109=EDGE_CURVE('',#21938,#20345,#3516,.T.);
#27110=EDGE_CURVE('',#21518,#21938,#3517,.T.);
#27111=EDGE_CURVE('',#21939,#20341,#3518,.T.);
#27112=EDGE_CURVE('',#21552,#21939,#3519,.T.);
#27113=EDGE_CURVE('',#21940,#20337,#3520,.T.);
#27114=EDGE_CURVE('',#21586,#21940,#3521,.T.);
#27115=EDGE_CURVE('',#21941,#20333,#3522,.T.);
#27116=EDGE_CURVE('',#21620,#21941,#3523,.T.);
#27117=EDGE_CURVE('',#21942,#20329,#3524,.T.);
#27118=EDGE_CURVE('',#21654,#21942,#3525,.T.);
#27119=EDGE_CURVE('',#21943,#20325,#3526,.T.);
#27120=EDGE_CURVE('',#21688,#21943,#3527,.T.);
#27121=EDGE_CURVE('',#21687,#21944,#3528,.T.);
#27122=EDGE_CURVE('',#21945,#21944,#1360,.T.);
#27123=EDGE_CURVE('',#21946,#21945,#18986,.T.);
#27124=EDGE_CURVE('',#21946,#21943,#3529,.T.);
#27125=EDGE_CURVE('',#21653,#21947,#3530,.T.);
#27126=EDGE_CURVE('',#21948,#21947,#1361,.T.);
#27127=EDGE_CURVE('',#21949,#21948,#18987,.T.);
#27128=EDGE_CURVE('',#21949,#21942,#3531,.T.);
#27129=EDGE_CURVE('',#21619,#21950,#3532,.T.);
#27130=EDGE_CURVE('',#21951,#21950,#1362,.T.);
#27131=EDGE_CURVE('',#21952,#21951,#18988,.T.);
#27132=EDGE_CURVE('',#21952,#21941,#3533,.T.);
#27133=EDGE_CURVE('',#21585,#21953,#3534,.T.);
#27134=EDGE_CURVE('',#21954,#21953,#1363,.T.);
#27135=EDGE_CURVE('',#21955,#21954,#18989,.T.);
#27136=EDGE_CURVE('',#21955,#21940,#3535,.T.);
#27137=EDGE_CURVE('',#21551,#21956,#3536,.T.);
#27138=EDGE_CURVE('',#21957,#21956,#1364,.T.);
#27139=EDGE_CURVE('',#21958,#21957,#18990,.T.);
#27140=EDGE_CURVE('',#21958,#21939,#3537,.T.);
#27141=EDGE_CURVE('',#21517,#21959,#3538,.T.);
#27142=EDGE_CURVE('',#21960,#21959,#1365,.T.);
#27143=EDGE_CURVE('',#21961,#21960,#18991,.T.);
#27144=EDGE_CURVE('',#21961,#21938,#3539,.T.);
#27145=EDGE_CURVE('',#21483,#21962,#3540,.T.);
#27146=EDGE_CURVE('',#21963,#21962,#1366,.T.);
#27147=EDGE_CURVE('',#21964,#21963,#18992,.T.);
#27148=EDGE_CURVE('',#21964,#21937,#3541,.T.);
#27149=EDGE_CURVE('',#21449,#21965,#3542,.T.);
#27150=EDGE_CURVE('',#21966,#21965,#1367,.T.);
#27151=EDGE_CURVE('',#21967,#21966,#18993,.T.);
#27152=EDGE_CURVE('',#21967,#21936,#3543,.T.);
#27153=EDGE_CURVE('',#21415,#21968,#3544,.T.);
#27154=EDGE_CURVE('',#21969,#21968,#1368,.T.);
#27155=EDGE_CURVE('',#21970,#21969,#18994,.T.);
#27156=EDGE_CURVE('',#21970,#21935,#3545,.T.);
#27157=EDGE_CURVE('',#21381,#21971,#3546,.T.);
#27158=EDGE_CURVE('',#21972,#21971,#1369,.T.);
#27159=EDGE_CURVE('',#21973,#21972,#18995,.T.);
#27160=EDGE_CURVE('',#21973,#21934,#3547,.T.);
#27161=EDGE_CURVE('',#21347,#21974,#3548,.T.);
#27162=EDGE_CURVE('',#21975,#21974,#1370,.T.);
#27163=EDGE_CURVE('',#21976,#21975,#18996,.T.);
#27164=EDGE_CURVE('',#21976,#21933,#3549,.T.);
#27165=EDGE_CURVE('',#21313,#21977,#3550,.T.);
#27166=EDGE_CURVE('',#21978,#21977,#1371,.T.);
#27167=EDGE_CURVE('',#21979,#21978,#18997,.T.);
#27168=EDGE_CURVE('',#21979,#21932,#3551,.T.);
#27169=EDGE_CURVE('',#21279,#21980,#3552,.T.);
#27170=EDGE_CURVE('',#21981,#21980,#1372,.T.);
#27171=EDGE_CURVE('',#21982,#21981,#18998,.T.);
#27172=EDGE_CURVE('',#21982,#21931,#3553,.T.);
#27173=EDGE_CURVE('',#21245,#21983,#3554,.T.);
#27174=EDGE_CURVE('',#21984,#21983,#1373,.T.);
#27175=EDGE_CURVE('',#21985,#21984,#18999,.T.);
#27176=EDGE_CURVE('',#21985,#21930,#3555,.T.);
#27177=EDGE_CURVE('',#21211,#21986,#3556,.T.);
#27178=EDGE_CURVE('',#21987,#21986,#1374,.T.);
#27179=EDGE_CURVE('',#21988,#21987,#19000,.T.);
#27180=EDGE_CURVE('',#21988,#21929,#3557,.T.);
#27181=EDGE_CURVE('',#21177,#21989,#3558,.T.);
#27182=EDGE_CURVE('',#21990,#21989,#1375,.T.);
#27183=EDGE_CURVE('',#21991,#21990,#19001,.T.);
#27184=EDGE_CURVE('',#21991,#21928,#3559,.T.);
#27185=EDGE_CURVE('',#21143,#21992,#3560,.T.);
#27186=EDGE_CURVE('',#21993,#21992,#1376,.T.);
#27187=EDGE_CURVE('',#21994,#21993,#19002,.T.);
#27188=EDGE_CURVE('',#21994,#21927,#3561,.T.);
#27189=EDGE_CURVE('',#21109,#21995,#3562,.T.);
#27190=EDGE_CURVE('',#21996,#21995,#1377,.T.);
#27191=EDGE_CURVE('',#21997,#21996,#19003,.T.);
#27192=EDGE_CURVE('',#21997,#21926,#3563,.T.);
#27193=EDGE_CURVE('',#21075,#21998,#3564,.T.);
#27194=EDGE_CURVE('',#21999,#21998,#1378,.T.);
#27195=EDGE_CURVE('',#22000,#21999,#19004,.T.);
#27196=EDGE_CURVE('',#22000,#21925,#3565,.T.);
#27197=EDGE_CURVE('',#21041,#22001,#3566,.T.);
#27198=EDGE_CURVE('',#22002,#22001,#1379,.T.);
#27199=EDGE_CURVE('',#22003,#22002,#19005,.T.);
#27200=EDGE_CURVE('',#22003,#21924,#3567,.T.);
#27201=EDGE_CURVE('',#21007,#22004,#3568,.T.);
#27202=EDGE_CURVE('',#22005,#22004,#1380,.T.);
#27203=EDGE_CURVE('',#22006,#22005,#19006,.T.);
#27204=EDGE_CURVE('',#22006,#21923,#3569,.T.);
#27205=EDGE_CURVE('',#20973,#22007,#3570,.T.);
#27206=EDGE_CURVE('',#22008,#22007,#1381,.T.);
#27207=EDGE_CURVE('',#22009,#22008,#19007,.T.);
#27208=EDGE_CURVE('',#22009,#21922,#3571,.T.);
#27209=EDGE_CURVE('',#20939,#22010,#3572,.T.);
#27210=EDGE_CURVE('',#22011,#22010,#1382,.T.);
#27211=EDGE_CURVE('',#22012,#22011,#19008,.T.);
#27212=EDGE_CURVE('',#22012,#21921,#3573,.T.);
#27213=EDGE_CURVE('',#20905,#22013,#3574,.T.);
#27214=EDGE_CURVE('',#22014,#22013,#1383,.T.);
#27215=EDGE_CURVE('',#22015,#22014,#19009,.T.);
#27216=EDGE_CURVE('',#22015,#21920,#3575,.T.);
#27217=EDGE_CURVE('',#20871,#22016,#3576,.T.);
#27218=EDGE_CURVE('',#22017,#22016,#1384,.T.);
#27219=EDGE_CURVE('',#22018,#22017,#19010,.T.);
#27220=EDGE_CURVE('',#22018,#21919,#3577,.T.);
#27221=EDGE_CURVE('',#20837,#22019,#3578,.T.);
#27222=EDGE_CURVE('',#22020,#22019,#1385,.T.);
#27223=EDGE_CURVE('',#22021,#22020,#19011,.T.);
#27224=EDGE_CURVE('',#22021,#21918,#3579,.T.);
#27225=EDGE_CURVE('',#20803,#22022,#3580,.T.);
#27226=EDGE_CURVE('',#22023,#22022,#1386,.T.);
#27227=EDGE_CURVE('',#22024,#22023,#19012,.T.);
#27228=EDGE_CURVE('',#22024,#21917,#3581,.T.);
#27229=EDGE_CURVE('',#20769,#22025,#3582,.T.);
#27230=EDGE_CURVE('',#22026,#22025,#1387,.T.);
#27231=EDGE_CURVE('',#22027,#22026,#19013,.T.);
#27232=EDGE_CURVE('',#22027,#21916,#3583,.T.);
#27233=EDGE_CURVE('',#20735,#22028,#3584,.T.);
#27234=EDGE_CURVE('',#22029,#22028,#1388,.T.);
#27235=EDGE_CURVE('',#22030,#22029,#19014,.T.);
#27236=EDGE_CURVE('',#22030,#21915,#3585,.T.);
#27237=EDGE_CURVE('',#20701,#22031,#3586,.T.);
#27238=EDGE_CURVE('',#22032,#22031,#1389,.T.);
#27239=EDGE_CURVE('',#22033,#22032,#19015,.T.);
#27240=EDGE_CURVE('',#22033,#21914,#3587,.T.);
#27241=EDGE_CURVE('',#20667,#22034,#3588,.T.);
#27242=EDGE_CURVE('',#22035,#22034,#1390,.T.);
#27243=EDGE_CURVE('',#22036,#22035,#19016,.T.);
#27244=EDGE_CURVE('',#22036,#21913,#3589,.T.);
#27245=EDGE_CURVE('',#20633,#22037,#3590,.T.);
#27246=EDGE_CURVE('',#22038,#22037,#1391,.T.);
#27247=EDGE_CURVE('',#22039,#22038,#19017,.T.);
#27248=EDGE_CURVE('',#22039,#21912,#3591,.T.);
#27249=EDGE_CURVE('',#20599,#22040,#3592,.T.);
#27250=EDGE_CURVE('',#22041,#22040,#1392,.T.);
#27251=EDGE_CURVE('',#22042,#22041,#19018,.T.);
#27252=EDGE_CURVE('',#22042,#21911,#3593,.T.);
#27253=EDGE_CURVE('',#20565,#22043,#3594,.T.);
#27254=EDGE_CURVE('',#22044,#22043,#1393,.T.);
#27255=EDGE_CURVE('',#22045,#22044,#19019,.T.);
#27256=EDGE_CURVE('',#22045,#21910,#3595,.T.);
#27257=EDGE_CURVE('',#20531,#22046,#3596,.T.);
#27258=EDGE_CURVE('',#22047,#22046,#1394,.T.);
#27259=EDGE_CURVE('',#22048,#22047,#19020,.T.);
#27260=EDGE_CURVE('',#22048,#21909,#3597,.T.);
#27261=EDGE_CURVE('',#22049,#21908,#3598,.T.);
#27262=EDGE_CURVE('',#20499,#22049,#19021,.T.);
#27263=EDGE_CURVE('',#22050,#21763,#3599,.T.);
#27264=EDGE_CURVE('',#21764,#22050,#3600,.T.);
#27265=EDGE_CURVE('',#22051,#21761,#3601,.T.);
#27266=EDGE_CURVE('',#21768,#22051,#3602,.T.);
#27267=EDGE_CURVE('',#22052,#21759,#3603,.T.);
#27268=EDGE_CURVE('',#21772,#22052,#3604,.T.);
#27269=EDGE_CURVE('',#22053,#21757,#3605,.T.);
#27270=EDGE_CURVE('',#21776,#22053,#3606,.T.);
#27271=EDGE_CURVE('',#22054,#21755,#3607,.T.);
#27272=EDGE_CURVE('',#21780,#22054,#3608,.T.);
#27273=EDGE_CURVE('',#22055,#21753,#3609,.T.);
#27274=EDGE_CURVE('',#21784,#22055,#3610,.T.);
#27275=EDGE_CURVE('',#22056,#21751,#3611,.T.);
#27276=EDGE_CURVE('',#21788,#22056,#3612,.T.);
#27277=EDGE_CURVE('',#22057,#21749,#3613,.T.);
#27278=EDGE_CURVE('',#21792,#22057,#3614,.T.);
#27279=EDGE_CURVE('',#22058,#21747,#3615,.T.);
#27280=EDGE_CURVE('',#21796,#22058,#3616,.T.);
#27281=EDGE_CURVE('',#22059,#21745,#3617,.T.);
#27282=EDGE_CURVE('',#21800,#22059,#3618,.T.);
#27283=EDGE_CURVE('',#22060,#21743,#3619,.T.);
#27284=EDGE_CURVE('',#21804,#22060,#3620,.T.);
#27285=EDGE_CURVE('',#22061,#21741,#3621,.T.);
#27286=EDGE_CURVE('',#21808,#22061,#3622,.T.);
#27287=EDGE_CURVE('',#22062,#21739,#3623,.T.);
#27288=EDGE_CURVE('',#21812,#22062,#3624,.T.);
#27289=EDGE_CURVE('',#22063,#21737,#3625,.T.);
#27290=EDGE_CURVE('',#21816,#22063,#3626,.T.);
#27291=EDGE_CURVE('',#22064,#21735,#3627,.T.);
#27292=EDGE_CURVE('',#21820,#22064,#3628,.T.);
#27293=EDGE_CURVE('',#22065,#21733,#3629,.T.);
#27294=EDGE_CURVE('',#21824,#22065,#3630,.T.);
#27295=EDGE_CURVE('',#22066,#21731,#3631,.T.);
#27296=EDGE_CURVE('',#21828,#22066,#3632,.T.);
#27297=EDGE_CURVE('',#22067,#21729,#3633,.T.);
#27298=EDGE_CURVE('',#21832,#22067,#3634,.T.);
#27299=EDGE_CURVE('',#22068,#21727,#3635,.T.);
#27300=EDGE_CURVE('',#21836,#22068,#3636,.T.);
#27301=EDGE_CURVE('',#22069,#21725,#3637,.T.);
#27302=EDGE_CURVE('',#21840,#22069,#3638,.T.);
#27303=EDGE_CURVE('',#22070,#21723,#3639,.T.);
#27304=EDGE_CURVE('',#21844,#22070,#3640,.T.);
#27305=EDGE_CURVE('',#22071,#21721,#3641,.T.);
#27306=EDGE_CURVE('',#21848,#22071,#3642,.T.);
#27307=EDGE_CURVE('',#22072,#21719,#3643,.T.);
#27308=EDGE_CURVE('',#21852,#22072,#3644,.T.);
#27309=EDGE_CURVE('',#22073,#21717,#3645,.T.);
#27310=EDGE_CURVE('',#21856,#22073,#3646,.T.);
#27311=EDGE_CURVE('',#22074,#21715,#3647,.T.);
#27312=EDGE_CURVE('',#21860,#22074,#3648,.T.);
#27313=EDGE_CURVE('',#22075,#21713,#3649,.T.);
#27314=EDGE_CURVE('',#21864,#22075,#3650,.T.);
#27315=EDGE_CURVE('',#22076,#21711,#3651,.T.);
#27316=EDGE_CURVE('',#21868,#22076,#3652,.T.);
#27317=EDGE_CURVE('',#22077,#21709,#3653,.T.);
#27318=EDGE_CURVE('',#21872,#22077,#3654,.T.);
#27319=EDGE_CURVE('',#22078,#21707,#3655,.T.);
#27320=EDGE_CURVE('',#21876,#22078,#3656,.T.);
#27321=EDGE_CURVE('',#22079,#21705,#3657,.T.);
#27322=EDGE_CURVE('',#21880,#22079,#3658,.T.);
#27323=EDGE_CURVE('',#22080,#21703,#3659,.T.);
#27324=EDGE_CURVE('',#21884,#22080,#3660,.T.);
#27325=EDGE_CURVE('',#22081,#21701,#3661,.T.);
#27326=EDGE_CURVE('',#21888,#22081,#3662,.T.);
#27327=EDGE_CURVE('',#22082,#21699,#3663,.T.);
#27328=EDGE_CURVE('',#21892,#22082,#3664,.T.);
#27329=EDGE_CURVE('',#22083,#21697,#3665,.T.);
#27330=EDGE_CURVE('',#21896,#22083,#3666,.T.);
#27331=EDGE_CURVE('',#22084,#21695,#3667,.T.);
#27332=EDGE_CURVE('',#21900,#22084,#3668,.T.);
#27333=EDGE_CURVE('',#22085,#21693,#3669,.T.);
#27334=EDGE_CURVE('',#21904,#22085,#3670,.T.);
#27335=EDGE_CURVE('',#22086,#22085,#3671,.T.);
#27336=EDGE_CURVE('',#21905,#22086,#19022,.T.);
#27337=EDGE_CURVE('',#22087,#22084,#3672,.T.);
#27338=EDGE_CURVE('',#21901,#22087,#19023,.T.);
#27339=EDGE_CURVE('',#22088,#22083,#3673,.T.);
#27340=EDGE_CURVE('',#21897,#22088,#19024,.T.);
#27341=EDGE_CURVE('',#22089,#22082,#3674,.T.);
#27342=EDGE_CURVE('',#21893,#22089,#19025,.T.);
#27343=EDGE_CURVE('',#22090,#22081,#3675,.T.);
#27344=EDGE_CURVE('',#21889,#22090,#19026,.T.);
#27345=EDGE_CURVE('',#22091,#22080,#3676,.T.);
#27346=EDGE_CURVE('',#21885,#22091,#19027,.T.);
#27347=EDGE_CURVE('',#22092,#22079,#3677,.T.);
#27348=EDGE_CURVE('',#21881,#22092,#19028,.T.);
#27349=EDGE_CURVE('',#22093,#22078,#3678,.T.);
#27350=EDGE_CURVE('',#21877,#22093,#19029,.T.);
#27351=EDGE_CURVE('',#22094,#22077,#3679,.T.);
#27352=EDGE_CURVE('',#21873,#22094,#19030,.T.);
#27353=EDGE_CURVE('',#22095,#22076,#3680,.T.);
#27354=EDGE_CURVE('',#21869,#22095,#19031,.T.);
#27355=EDGE_CURVE('',#22096,#22075,#3681,.T.);
#27356=EDGE_CURVE('',#21865,#22096,#19032,.T.);
#27357=EDGE_CURVE('',#22097,#22074,#3682,.T.);
#27358=EDGE_CURVE('',#21861,#22097,#19033,.T.);
#27359=EDGE_CURVE('',#22098,#22073,#3683,.T.);
#27360=EDGE_CURVE('',#21857,#22098,#19034,.T.);
#27361=EDGE_CURVE('',#22099,#22072,#3684,.T.);
#27362=EDGE_CURVE('',#21853,#22099,#19035,.T.);
#27363=EDGE_CURVE('',#22100,#22071,#3685,.T.);
#27364=EDGE_CURVE('',#21849,#22100,#19036,.T.);
#27365=EDGE_CURVE('',#22101,#22070,#3686,.T.);
#27366=EDGE_CURVE('',#21845,#22101,#19037,.T.);
#27367=EDGE_CURVE('',#22102,#22069,#3687,.T.);
#27368=EDGE_CURVE('',#21841,#22102,#19038,.T.);
#27369=EDGE_CURVE('',#22103,#22068,#3688,.T.);
#27370=EDGE_CURVE('',#22104,#22103,#19039,.T.);
#27371=EDGE_CURVE('',#21837,#22104,#19040,.T.);
#27372=EDGE_CURVE('',#22105,#22067,#3689,.T.);
#27373=EDGE_CURVE('',#21833,#22105,#19041,.T.);
#27374=EDGE_CURVE('',#22106,#22066,#3690,.T.);
#27375=EDGE_CURVE('',#21829,#22106,#19042,.T.);
#27376=EDGE_CURVE('',#22107,#22065,#3691,.T.);
#27377=EDGE_CURVE('',#21825,#22107,#19043,.T.);
#27378=EDGE_CURVE('',#22108,#22064,#3692,.T.);
#27379=EDGE_CURVE('',#21821,#22108,#19044,.T.);
#27380=EDGE_CURVE('',#22109,#22063,#3693,.T.);
#27381=EDGE_CURVE('',#21817,#22109,#19045,.T.);
#27382=EDGE_CURVE('',#22110,#22062,#3694,.T.);
#27383=EDGE_CURVE('',#21813,#22110,#19046,.T.);
#27384=EDGE_CURVE('',#22111,#22061,#3695,.T.);
#27385=EDGE_CURVE('',#21809,#22111,#19047,.T.);
#27386=EDGE_CURVE('',#22112,#22060,#3696,.T.);
#27387=EDGE_CURVE('',#21805,#22112,#19048,.T.);
#27388=EDGE_CURVE('',#22113,#22059,#3697,.T.);
#27389=EDGE_CURVE('',#21801,#22113,#19049,.T.);
#27390=EDGE_CURVE('',#22114,#22058,#3698,.T.);
#27391=EDGE_CURVE('',#21797,#22114,#19050,.T.);
#27392=EDGE_CURVE('',#22115,#22057,#3699,.T.);
#27393=EDGE_CURVE('',#21793,#22115,#19051,.T.);
#27394=EDGE_CURVE('',#22116,#22056,#3700,.T.);
#27395=EDGE_CURVE('',#21789,#22116,#19052,.T.);
#27396=EDGE_CURVE('',#22117,#22055,#3701,.T.);
#27397=EDGE_CURVE('',#21785,#22117,#19053,.T.);
#27398=EDGE_CURVE('',#22118,#22054,#3702,.T.);
#27399=EDGE_CURVE('',#21781,#22118,#19054,.T.);
#27400=EDGE_CURVE('',#22119,#22053,#3703,.T.);
#27401=EDGE_CURVE('',#21777,#22119,#19055,.T.);
#27402=EDGE_CURVE('',#22120,#22052,#3704,.T.);
#27403=EDGE_CURVE('',#21773,#22120,#19056,.T.);
#27404=EDGE_CURVE('',#22121,#22051,#3705,.T.);
#27405=EDGE_CURVE('',#21769,#22121,#19057,.T.);
#27406=EDGE_CURVE('',#22122,#22050,#3706,.T.);
#27407=EDGE_CURVE('',#21765,#22122,#19058,.T.);
#27408=EDGE_CURVE('',#22123,#21691,#3707,.T.);
#27409=EDGE_CURVE('',#21659,#22123,#3708,.T.);
#27410=EDGE_CURVE('',#22124,#22123,#1395,.T.);
#27411=EDGE_CURVE('',#21660,#22124,#3709,.T.);
#27412=EDGE_CURVE('',#22125,#22124,#1396,.T.);
#27413=EDGE_CURVE('',#21661,#22125,#3710,.T.);
#27414=EDGE_CURVE('',#22126,#22125,#1397,.T.);
#27415=EDGE_CURVE('',#21662,#22126,#3711,.T.);
#27416=EDGE_CURVE('',#22127,#22126,#1398,.T.);
#27417=EDGE_CURVE('',#21663,#22127,#3712,.T.);
#27418=EDGE_CURVE('',#22128,#22127,#1399,.T.);
#27419=EDGE_CURVE('',#21664,#22128,#3713,.T.);
#27420=EDGE_CURVE('',#22129,#22128,#3714,.T.);
#27421=EDGE_CURVE('',#21665,#22129,#3715,.T.);
#27422=EDGE_CURVE('',#22130,#22129,#1400,.T.);
#27423=EDGE_CURVE('',#21666,#22130,#3716,.T.);
#27424=EDGE_CURVE('',#22131,#22130,#1401,.T.);
#27425=EDGE_CURVE('',#21667,#22131,#3717,.T.);
#27426=EDGE_CURVE('',#22132,#22131,#1402,.T.);
#27427=EDGE_CURVE('',#21668,#22132,#3718,.T.);
#27428=EDGE_CURVE('',#22133,#22132,#1403,.T.);
#27429=EDGE_CURVE('',#21669,#22133,#3719,.T.);
#27430=EDGE_CURVE('',#22134,#22133,#1404,.T.);
#27431=EDGE_CURVE('',#21670,#22134,#3720,.T.);
#27432=EDGE_CURVE('',#22135,#22134,#3721,.T.);
#27433=EDGE_CURVE('',#21671,#22135,#3722,.T.);
#27434=EDGE_CURVE('',#22136,#22135,#1405,.T.);
#27435=EDGE_CURVE('',#22086,#22136,#19059,.T.);
#27436=EDGE_CURVE('',#22137,#21907,#3723,.T.);
#27437=EDGE_CURVE('',#21675,#22137,#3724,.T.);
#27438=EDGE_CURVE('',#22138,#22137,#1406,.T.);
#27439=EDGE_CURVE('',#21676,#22138,#3725,.T.);
#27440=EDGE_CURVE('',#22139,#22138,#1407,.T.);
#27441=EDGE_CURVE('',#21677,#22139,#3726,.T.);
#27442=EDGE_CURVE('',#22140,#22139,#1408,.T.);
#27443=EDGE_CURVE('',#21678,#22140,#3727,.T.);
#27444=EDGE_CURVE('',#22141,#22140,#1409,.T.);
#27445=EDGE_CURVE('',#21679,#22141,#3728,.T.);
#27446=EDGE_CURVE('',#22142,#22141,#1410,.T.);
#27447=EDGE_CURVE('',#21680,#22142,#3729,.T.);
#27448=EDGE_CURVE('',#22143,#22142,#3730,.T.);
#27449=EDGE_CURVE('',#21681,#22143,#3731,.T.);
#27450=EDGE_CURVE('',#22144,#22143,#1411,.T.);
#27451=EDGE_CURVE('',#21682,#22144,#3732,.T.);
#27452=EDGE_CURVE('',#22145,#22144,#1412,.T.);
#27453=EDGE_CURVE('',#21683,#22145,#3733,.T.);
#27454=EDGE_CURVE('',#22146,#22145,#1413,.T.);
#27455=EDGE_CURVE('',#21684,#22146,#3734,.T.);
#27456=EDGE_CURVE('',#22147,#22146,#1414,.T.);
#27457=EDGE_CURVE('',#21685,#22147,#3735,.T.);
#27458=EDGE_CURVE('',#22148,#22147,#1415,.T.);
#27459=EDGE_CURVE('',#21686,#22148,#3736,.T.);
#27460=EDGE_CURVE('',#21944,#22148,#3737,.T.);
#27461=EDGE_CURVE('',#21689,#21946,#19060,.T.);
#27462=EDGE_CURVE('',#22149,#22149,#19646,.T.);
#27463=EDGE_CURVE('',#22149,#22150,#3738,.T.);
#27464=EDGE_CURVE('',#22150,#21997,#19061,.T.);
#27465=EDGE_CURVE('',#21078,#21996,#19647,.T.);
#27466=EDGE_CURVE('',#21077,#22000,#19062,.T.);
#27467=EDGE_CURVE('',#21044,#21999,#19648,.T.);
#27468=EDGE_CURVE('',#21043,#22003,#19063,.T.);
#27469=EDGE_CURVE('',#21010,#22002,#19649,.T.);
#27470=EDGE_CURVE('',#21009,#22006,#19064,.T.);
#27471=EDGE_CURVE('',#20976,#22005,#19650,.T.);
#27472=EDGE_CURVE('',#20975,#22009,#19065,.T.);
#27473=EDGE_CURVE('',#20942,#22008,#19651,.T.);
#27474=EDGE_CURVE('',#20941,#22012,#19066,.T.);
#27475=EDGE_CURVE('',#20908,#22011,#19652,.T.);
#27476=EDGE_CURVE('',#20907,#22015,#19067,.T.);
#27477=EDGE_CURVE('',#20874,#22014,#19653,.T.);
#27478=EDGE_CURVE('',#20873,#22018,#19068,.T.);
#27479=EDGE_CURVE('',#20840,#22017,#19654,.T.);
#27480=EDGE_CURVE('',#20839,#22021,#19069,.T.);
#27481=EDGE_CURVE('',#20806,#22020,#19655,.T.);
#27482=EDGE_CURVE('',#20805,#22024,#19070,.T.);
#27483=EDGE_CURVE('',#20772,#22023,#19656,.T.);
#27484=EDGE_CURVE('',#20771,#22027,#19071,.T.);
#27485=EDGE_CURVE('',#20738,#22026,#19657,.T.);
#27486=EDGE_CURVE('',#20737,#22030,#19072,.T.);
#27487=EDGE_CURVE('',#20704,#22029,#19658,.T.);
#27488=EDGE_CURVE('',#20703,#22033,#19073,.T.);
#27489=EDGE_CURVE('',#20670,#22032,#19659,.T.);
#27490=EDGE_CURVE('',#20669,#22036,#19074,.T.);
#27491=EDGE_CURVE('',#20636,#22035,#19660,.T.);
#27492=EDGE_CURVE('',#20635,#22039,#19075,.T.);
#27493=EDGE_CURVE('',#20602,#22038,#19661,.T.);
#27494=EDGE_CURVE('',#20601,#22042,#19076,.T.);
#27495=EDGE_CURVE('',#20568,#22041,#19662,.T.);
#27496=EDGE_CURVE('',#20567,#22045,#19077,.T.);
#27497=EDGE_CURVE('',#20534,#22044,#19663,.T.);
#27498=EDGE_CURVE('',#20533,#22048,#19078,.T.);
#27499=EDGE_CURVE('',#20500,#22047,#19664,.T.);
#27500=EDGE_CURVE('',#22049,#22151,#19079,.T.);
#27501=EDGE_CURVE('',#21690,#22151,#19665,.T.);
#27502=EDGE_CURVE('',#21656,#21945,#19666,.T.);
#27503=EDGE_CURVE('',#21655,#21949,#19080,.T.);
#27504=EDGE_CURVE('',#21622,#21948,#19667,.T.);
#27505=EDGE_CURVE('',#21621,#21952,#19081,.T.);
#27506=EDGE_CURVE('',#21588,#21951,#19668,.T.);
#27507=EDGE_CURVE('',#21587,#21955,#19082,.T.);
#27508=EDGE_CURVE('',#21554,#21954,#19669,.T.);
#27509=EDGE_CURVE('',#21553,#21958,#19083,.T.);
#27510=EDGE_CURVE('',#21520,#21957,#19670,.T.);
#27511=EDGE_CURVE('',#21519,#21961,#19084,.T.);
#27512=EDGE_CURVE('',#21486,#21960,#19671,.T.);
#27513=EDGE_CURVE('',#21485,#21964,#19085,.T.);
#27514=EDGE_CURVE('',#21452,#21963,#19672,.T.);
#27515=EDGE_CURVE('',#21451,#21967,#19086,.T.);
#27516=EDGE_CURVE('',#21418,#21966,#19673,.T.);
#27517=EDGE_CURVE('',#21417,#21970,#19087,.T.);
#27518=EDGE_CURVE('',#21384,#21969,#19674,.T.);
#27519=EDGE_CURVE('',#21383,#21973,#19088,.T.);
#27520=EDGE_CURVE('',#21350,#21972,#19675,.T.);
#27521=EDGE_CURVE('',#21349,#21976,#19089,.T.);
#27522=EDGE_CURVE('',#21316,#21975,#19676,.T.);
#27523=EDGE_CURVE('',#21315,#21979,#19090,.T.);
#27524=EDGE_CURVE('',#21282,#21978,#19677,.T.);
#27525=EDGE_CURVE('',#21281,#21982,#19091,.T.);
#27526=EDGE_CURVE('',#21248,#21981,#19678,.T.);
#27527=EDGE_CURVE('',#21247,#21985,#19092,.T.);
#27528=EDGE_CURVE('',#21214,#21984,#19679,.T.);
#27529=EDGE_CURVE('',#21213,#21988,#19093,.T.);
#27530=EDGE_CURVE('',#21180,#21987,#19680,.T.);
#27531=EDGE_CURVE('',#21179,#21991,#19094,.T.);
#27532=EDGE_CURVE('',#21146,#21990,#19681,.T.);
#27533=EDGE_CURVE('',#21145,#21994,#19095,.T.);
#27534=EDGE_CURVE('',#21112,#21993,#19682,.T.);
#27535=EDGE_CURVE('',#21111,#22150,#19096,.T.);
#27536=EDGE_CURVE('',#22152,#21906,#19683,.T.);
#27537=EDGE_CURVE('',#22152,#22153,#1416,.T.);
#27538=EDGE_CURVE('',#22153,#22154,#3739,.T.);
#27539=EDGE_CURVE('',#22154,#22155,#1417,.T.);
#27540=EDGE_CURVE('',#22155,#22156,#1418,.T.);
#27541=EDGE_CURVE('',#22156,#22157,#1419,.T.);
#27542=EDGE_CURVE('',#22157,#22158,#1420,.T.);
#27543=EDGE_CURVE('',#22158,#22159,#1421,.T.);
#27544=EDGE_CURVE('',#22159,#22160,#3740,.T.);
#27545=EDGE_CURVE('',#22160,#22161,#1422,.T.);
#27546=EDGE_CURVE('',#22161,#22162,#1423,.T.);
#27547=EDGE_CURVE('',#22162,#22163,#1424,.T.);
#27548=EDGE_CURVE('',#22163,#22164,#1425,.T.);
#27549=EDGE_CURVE('',#22164,#22165,#1426,.T.);
#27550=EDGE_CURVE('',#22165,#21657,#3741,.T.);
#27551=EDGE_CURVE('',#21625,#22165,#3742,.T.);
#27552=EDGE_CURVE('',#21626,#22164,#3743,.T.);
#27553=EDGE_CURVE('',#21627,#22163,#3744,.T.);
#27554=EDGE_CURVE('',#21628,#22162,#3745,.T.);
#27555=EDGE_CURVE('',#21629,#22161,#3746,.T.);
#27556=EDGE_CURVE('',#21630,#22160,#3747,.T.);
#27557=EDGE_CURVE('',#21631,#22159,#3748,.T.);
#27558=EDGE_CURVE('',#21632,#22158,#3749,.T.);
#27559=EDGE_CURVE('',#21633,#22157,#3750,.T.);
#27560=EDGE_CURVE('',#21634,#22156,#3751,.T.);
#27561=EDGE_CURVE('',#21635,#22155,#3752,.T.);
#27562=EDGE_CURVE('',#21636,#22154,#3753,.T.);
#27563=EDGE_CURVE('',#21637,#22153,#3754,.T.);
#27564=EDGE_CURVE('',#22087,#22152,#19097,.T.);
#27565=EDGE_CURVE('',#22166,#21903,#3755,.T.);
#27566=EDGE_CURVE('',#21641,#22166,#3756,.T.);
#27567=EDGE_CURVE('',#22167,#22166,#1427,.T.);
#27568=EDGE_CURVE('',#21642,#22167,#3757,.T.);
#27569=EDGE_CURVE('',#22168,#22167,#1428,.T.);
#27570=EDGE_CURVE('',#21643,#22168,#3758,.T.);
#27571=EDGE_CURVE('',#22169,#22168,#1429,.T.);
#27572=EDGE_CURVE('',#21644,#22169,#3759,.T.);
#27573=EDGE_CURVE('',#22170,#22169,#1430,.T.);
#27574=EDGE_CURVE('',#21645,#22170,#3760,.T.);
#27575=EDGE_CURVE('',#22171,#22170,#1431,.T.);
#27576=EDGE_CURVE('',#21646,#22171,#3761,.T.);
#27577=EDGE_CURVE('',#22172,#22171,#3762,.T.);
#27578=EDGE_CURVE('',#21647,#22172,#3763,.T.);
#27579=EDGE_CURVE('',#22173,#22172,#1432,.T.);
#27580=EDGE_CURVE('',#21648,#22173,#3764,.T.);
#27581=EDGE_CURVE('',#22174,#22173,#1433,.T.);
#27582=EDGE_CURVE('',#21649,#22174,#3765,.T.);
#27583=EDGE_CURVE('',#22175,#22174,#1434,.T.);
#27584=EDGE_CURVE('',#21650,#22175,#3766,.T.);
#27585=EDGE_CURVE('',#22176,#22175,#1435,.T.);
#27586=EDGE_CURVE('',#21651,#22176,#3767,.T.);
#27587=EDGE_CURVE('',#22177,#22176,#1436,.T.);
#27588=EDGE_CURVE('',#21652,#22177,#3768,.T.);
#27589=EDGE_CURVE('',#21947,#22177,#3769,.T.);
#27590=EDGE_CURVE('',#22178,#21902,#19684,.T.);
#27591=EDGE_CURVE('',#22178,#22179,#1437,.T.);
#27592=EDGE_CURVE('',#22179,#22180,#3770,.T.);
#27593=EDGE_CURVE('',#22180,#22181,#1438,.T.);
#27594=EDGE_CURVE('',#22181,#22182,#1439,.T.);
#27595=EDGE_CURVE('',#22182,#22183,#1440,.T.);
#27596=EDGE_CURVE('',#22183,#22184,#1441,.T.);
#27597=EDGE_CURVE('',#22184,#22185,#1442,.T.);
#27598=EDGE_CURVE('',#22185,#22186,#3771,.T.);
#27599=EDGE_CURVE('',#22186,#22187,#1443,.T.);
#27600=EDGE_CURVE('',#22187,#22188,#1444,.T.);
#27601=EDGE_CURVE('',#22188,#22189,#1445,.T.);
#27602=EDGE_CURVE('',#22189,#22190,#1446,.T.);
#27603=EDGE_CURVE('',#22190,#22191,#1447,.T.);
#27604=EDGE_CURVE('',#22191,#21623,#3772,.T.);
#27605=EDGE_CURVE('',#21591,#22191,#3773,.T.);
#27606=EDGE_CURVE('',#21592,#22190,#3774,.T.);
#27607=EDGE_CURVE('',#21593,#22189,#3775,.T.);
#27608=EDGE_CURVE('',#21594,#22188,#3776,.T.);
#27609=EDGE_CURVE('',#21595,#22187,#3777,.T.);
#27610=EDGE_CURVE('',#21596,#22186,#3778,.T.);
#27611=EDGE_CURVE('',#21597,#22185,#3779,.T.);
#27612=EDGE_CURVE('',#21598,#22184,#3780,.T.);
#27613=EDGE_CURVE('',#21599,#22183,#3781,.T.);
#27614=EDGE_CURVE('',#21600,#22182,#3782,.T.);
#27615=EDGE_CURVE('',#21601,#22181,#3783,.T.);
#27616=EDGE_CURVE('',#21602,#22180,#3784,.T.);
#27617=EDGE_CURVE('',#21603,#22179,#3785,.T.);
#27618=EDGE_CURVE('',#22088,#22178,#19098,.T.);
#27619=EDGE_CURVE('',#22192,#21899,#3786,.T.);
#27620=EDGE_CURVE('',#21607,#22192,#3787,.T.);
#27621=EDGE_CURVE('',#22193,#22192,#1448,.T.);
#27622=EDGE_CURVE('',#21608,#22193,#3788,.T.);
#27623=EDGE_CURVE('',#22194,#22193,#1449,.T.);
#27624=EDGE_CURVE('',#21609,#22194,#3789,.T.);
#27625=EDGE_CURVE('',#22195,#22194,#1450,.T.);
#27626=EDGE_CURVE('',#21610,#22195,#3790,.T.);
#27627=EDGE_CURVE('',#22196,#22195,#1451,.T.);
#27628=EDGE_CURVE('',#21611,#22196,#3791,.T.);
#27629=EDGE_CURVE('',#22197,#22196,#1452,.T.);
#27630=EDGE_CURVE('',#21612,#22197,#3792,.T.);
#27631=EDGE_CURVE('',#22198,#22197,#3793,.T.);
#27632=EDGE_CURVE('',#21613,#22198,#3794,.T.);
#27633=EDGE_CURVE('',#22199,#22198,#1453,.T.);
#27634=EDGE_CURVE('',#21614,#22199,#3795,.T.);
#27635=EDGE_CURVE('',#22200,#22199,#1454,.T.);
#27636=EDGE_CURVE('',#21615,#22200,#3796,.T.);
#27637=EDGE_CURVE('',#22201,#22200,#1455,.T.);
#27638=EDGE_CURVE('',#21616,#22201,#3797,.T.);
#27639=EDGE_CURVE('',#22202,#22201,#1456,.T.);
#27640=EDGE_CURVE('',#21617,#22202,#3798,.T.);
#27641=EDGE_CURVE('',#22203,#22202,#1457,.T.);
#27642=EDGE_CURVE('',#21618,#22203,#3799,.T.);
#27643=EDGE_CURVE('',#21950,#22203,#3800,.T.);
#27644=EDGE_CURVE('',#22204,#21898,#19685,.T.);
#27645=EDGE_CURVE('',#22204,#22205,#1458,.T.);
#27646=EDGE_CURVE('',#22205,#22206,#3801,.T.);
#27647=EDGE_CURVE('',#22206,#22207,#1459,.T.);
#27648=EDGE_CURVE('',#22207,#22208,#1460,.T.);
#27649=EDGE_CURVE('',#22208,#22209,#1461,.T.);
#27650=EDGE_CURVE('',#22209,#22210,#1462,.T.);
#27651=EDGE_CURVE('',#22210,#22211,#1463,.T.);
#27652=EDGE_CURVE('',#22211,#22212,#3802,.T.);
#27653=EDGE_CURVE('',#22212,#22213,#1464,.T.);
#27654=EDGE_CURVE('',#22213,#22214,#1465,.T.);
#27655=EDGE_CURVE('',#22214,#22215,#1466,.T.);
#27656=EDGE_CURVE('',#22215,#22216,#1467,.T.);
#27657=EDGE_CURVE('',#22216,#22217,#1468,.T.);
#27658=EDGE_CURVE('',#22217,#21589,#3803,.T.);
#27659=EDGE_CURVE('',#21557,#22217,#3804,.T.);
#27660=EDGE_CURVE('',#21558,#22216,#3805,.T.);
#27661=EDGE_CURVE('',#21559,#22215,#3806,.T.);
#27662=EDGE_CURVE('',#21560,#22214,#3807,.T.);
#27663=EDGE_CURVE('',#21561,#22213,#3808,.T.);
#27664=EDGE_CURVE('',#21562,#22212,#3809,.T.);
#27665=EDGE_CURVE('',#21563,#22211,#3810,.T.);
#27666=EDGE_CURVE('',#21564,#22210,#3811,.T.);
#27667=EDGE_CURVE('',#21565,#22209,#3812,.T.);
#27668=EDGE_CURVE('',#21566,#22208,#3813,.T.);
#27669=EDGE_CURVE('',#21567,#22207,#3814,.T.);
#27670=EDGE_CURVE('',#21568,#22206,#3815,.T.);
#27671=EDGE_CURVE('',#21569,#22205,#3816,.T.);
#27672=EDGE_CURVE('',#22089,#22204,#19099,.T.);
#27673=EDGE_CURVE('',#22218,#21895,#3817,.T.);
#27674=EDGE_CURVE('',#21573,#22218,#3818,.T.);
#27675=EDGE_CURVE('',#22219,#22218,#1469,.T.);
#27676=EDGE_CURVE('',#21574,#22219,#3819,.T.);
#27677=EDGE_CURVE('',#22220,#22219,#1470,.T.);
#27678=EDGE_CURVE('',#21575,#22220,#3820,.T.);
#27679=EDGE_CURVE('',#22221,#22220,#1471,.T.);
#27680=EDGE_CURVE('',#21576,#22221,#3821,.T.);
#27681=EDGE_CURVE('',#22222,#22221,#1472,.T.);
#27682=EDGE_CURVE('',#21577,#22222,#3822,.T.);
#27683=EDGE_CURVE('',#22223,#22222,#1473,.T.);
#27684=EDGE_CURVE('',#21578,#22223,#3823,.T.);
#27685=EDGE_CURVE('',#22224,#22223,#3824,.T.);
#27686=EDGE_CURVE('',#21579,#22224,#3825,.T.);
#27687=EDGE_CURVE('',#22225,#22224,#1474,.T.);
#27688=EDGE_CURVE('',#21580,#22225,#3826,.T.);
#27689=EDGE_CURVE('',#22226,#22225,#1475,.T.);
#27690=EDGE_CURVE('',#21581,#22226,#3827,.T.);
#27691=EDGE_CURVE('',#22227,#22226,#1476,.T.);
#27692=EDGE_CURVE('',#21582,#22227,#3828,.T.);
#27693=EDGE_CURVE('',#22228,#22227,#1477,.T.);
#27694=EDGE_CURVE('',#21583,#22228,#3829,.T.);
#27695=EDGE_CURVE('',#22229,#22228,#1478,.T.);
#27696=EDGE_CURVE('',#21584,#22229,#3830,.T.);
#27697=EDGE_CURVE('',#21953,#22229,#3831,.T.);
#27698=EDGE_CURVE('',#22230,#21894,#19686,.T.);
#27699=EDGE_CURVE('',#22230,#22231,#1479,.T.);
#27700=EDGE_CURVE('',#22231,#22232,#3832,.T.);
#27701=EDGE_CURVE('',#22232,#22233,#1480,.T.);
#27702=EDGE_CURVE('',#22233,#22234,#1481,.T.);
#27703=EDGE_CURVE('',#22234,#22235,#1482,.T.);
#27704=EDGE_CURVE('',#22235,#22236,#1483,.T.);
#27705=EDGE_CURVE('',#22236,#22237,#1484,.T.);
#27706=EDGE_CURVE('',#22237,#22238,#3833,.T.);
#27707=EDGE_CURVE('',#22238,#22239,#1485,.T.);
#27708=EDGE_CURVE('',#22239,#22240,#1486,.T.);
#27709=EDGE_CURVE('',#22240,#22241,#1487,.T.);
#27710=EDGE_CURVE('',#22241,#22242,#1488,.T.);
#27711=EDGE_CURVE('',#22242,#22243,#1489,.T.);
#27712=EDGE_CURVE('',#22243,#21555,#3834,.T.);
#27713=EDGE_CURVE('',#21523,#22243,#3835,.T.);
#27714=EDGE_CURVE('',#21524,#22242,#3836,.T.);
#27715=EDGE_CURVE('',#21525,#22241,#3837,.T.);
#27716=EDGE_CURVE('',#21526,#22240,#3838,.T.);
#27717=EDGE_CURVE('',#21527,#22239,#3839,.T.);
#27718=EDGE_CURVE('',#21528,#22238,#3840,.T.);
#27719=EDGE_CURVE('',#21529,#22237,#3841,.T.);
#27720=EDGE_CURVE('',#21530,#22236,#3842,.T.);
#27721=EDGE_CURVE('',#21531,#22235,#3843,.T.);
#27722=EDGE_CURVE('',#21532,#22234,#3844,.T.);
#27723=EDGE_CURVE('',#21533,#22233,#3845,.T.);
#27724=EDGE_CURVE('',#21534,#22232,#3846,.T.);
#27725=EDGE_CURVE('',#21535,#22231,#3847,.T.);
#27726=EDGE_CURVE('',#22090,#22230,#19100,.T.);
#27727=EDGE_CURVE('',#22244,#21891,#3848,.T.);
#27728=EDGE_CURVE('',#21539,#22244,#3849,.T.);
#27729=EDGE_CURVE('',#22245,#22244,#1490,.T.);
#27730=EDGE_CURVE('',#21540,#22245,#3850,.T.);
#27731=EDGE_CURVE('',#22246,#22245,#1491,.T.);
#27732=EDGE_CURVE('',#21541,#22246,#3851,.T.);
#27733=EDGE_CURVE('',#22247,#22246,#1492,.T.);
#27734=EDGE_CURVE('',#21542,#22247,#3852,.T.);
#27735=EDGE_CURVE('',#22248,#22247,#1493,.T.);
#27736=EDGE_CURVE('',#21543,#22248,#3853,.T.);
#27737=EDGE_CURVE('',#22249,#22248,#1494,.T.);
#27738=EDGE_CURVE('',#21544,#22249,#3854,.T.);
#27739=EDGE_CURVE('',#22250,#22249,#3855,.T.);
#27740=EDGE_CURVE('',#21545,#22250,#3856,.T.);
#27741=EDGE_CURVE('',#22251,#22250,#1495,.T.);
#27742=EDGE_CURVE('',#21546,#22251,#3857,.T.);
#27743=EDGE_CURVE('',#22252,#22251,#1496,.T.);
#27744=EDGE_CURVE('',#21547,#22252,#3858,.T.);
#27745=EDGE_CURVE('',#22253,#22252,#1497,.T.);
#27746=EDGE_CURVE('',#21548,#22253,#3859,.T.);
#27747=EDGE_CURVE('',#22254,#22253,#1498,.T.);
#27748=EDGE_CURVE('',#21549,#22254,#3860,.T.);
#27749=EDGE_CURVE('',#22255,#22254,#1499,.T.);
#27750=EDGE_CURVE('',#21550,#22255,#3861,.T.);
#27751=EDGE_CURVE('',#21956,#22255,#3862,.T.);
#27752=EDGE_CURVE('',#22256,#21890,#19687,.T.);
#27753=EDGE_CURVE('',#22256,#22257,#1500,.T.);
#27754=EDGE_CURVE('',#22257,#22258,#3863,.T.);
#27755=EDGE_CURVE('',#22258,#22259,#1501,.T.);
#27756=EDGE_CURVE('',#22259,#22260,#1502,.T.);
#27757=EDGE_CURVE('',#22260,#22261,#1503,.T.);
#27758=EDGE_CURVE('',#22261,#22262,#1504,.T.);
#27759=EDGE_CURVE('',#22262,#22263,#1505,.T.);
#27760=EDGE_CURVE('',#22263,#22264,#3864,.T.);
#27761=EDGE_CURVE('',#22264,#22265,#1506,.T.);
#27762=EDGE_CURVE('',#22265,#22266,#1507,.T.);
#27763=EDGE_CURVE('',#22266,#22267,#1508,.T.);
#27764=EDGE_CURVE('',#22267,#22268,#1509,.T.);
#27765=EDGE_CURVE('',#22268,#22269,#1510,.T.);
#27766=EDGE_CURVE('',#22269,#21521,#3865,.T.);
#27767=EDGE_CURVE('',#21489,#22269,#3866,.T.);
#27768=EDGE_CURVE('',#21490,#22268,#3867,.T.);
#27769=EDGE_CURVE('',#21491,#22267,#3868,.T.);
#27770=EDGE_CURVE('',#21492,#22266,#3869,.T.);
#27771=EDGE_CURVE('',#21493,#22265,#3870,.T.);
#27772=EDGE_CURVE('',#21494,#22264,#3871,.T.);
#27773=EDGE_CURVE('',#21495,#22263,#3872,.T.);
#27774=EDGE_CURVE('',#21496,#22262,#3873,.T.);
#27775=EDGE_CURVE('',#21497,#22261,#3874,.T.);
#27776=EDGE_CURVE('',#21498,#22260,#3875,.T.);
#27777=EDGE_CURVE('',#21499,#22259,#3876,.T.);
#27778=EDGE_CURVE('',#21500,#22258,#3877,.T.);
#27779=EDGE_CURVE('',#21501,#22257,#3878,.T.);
#27780=EDGE_CURVE('',#22091,#22256,#19101,.T.);
#27781=EDGE_CURVE('',#22270,#21887,#3879,.T.);
#27782=EDGE_CURVE('',#21505,#22270,#3880,.T.);
#27783=EDGE_CURVE('',#22271,#22270,#1511,.T.);
#27784=EDGE_CURVE('',#21506,#22271,#3881,.T.);
#27785=EDGE_CURVE('',#22272,#22271,#1512,.T.);
#27786=EDGE_CURVE('',#21507,#22272,#3882,.T.);
#27787=EDGE_CURVE('',#22273,#22272,#1513,.T.);
#27788=EDGE_CURVE('',#21508,#22273,#3883,.T.);
#27789=EDGE_CURVE('',#22274,#22273,#1514,.T.);
#27790=EDGE_CURVE('',#21509,#22274,#3884,.T.);
#27791=EDGE_CURVE('',#22275,#22274,#1515,.T.);
#27792=EDGE_CURVE('',#21510,#22275,#3885,.T.);
#27793=EDGE_CURVE('',#22276,#22275,#3886,.T.);
#27794=EDGE_CURVE('',#21511,#22276,#3887,.T.);
#27795=EDGE_CURVE('',#22277,#22276,#1516,.T.);
#27796=EDGE_CURVE('',#21512,#22277,#3888,.T.);
#27797=EDGE_CURVE('',#22278,#22277,#1517,.T.);
#27798=EDGE_CURVE('',#21513,#22278,#3889,.T.);
#27799=EDGE_CURVE('',#22279,#22278,#1518,.T.);
#27800=EDGE_CURVE('',#21514,#22279,#3890,.T.);
#27801=EDGE_CURVE('',#22280,#22279,#1519,.T.);
#27802=EDGE_CURVE('',#21515,#22280,#3891,.T.);
#27803=EDGE_CURVE('',#22281,#22280,#1520,.T.);
#27804=EDGE_CURVE('',#21516,#22281,#3892,.T.);
#27805=EDGE_CURVE('',#21959,#22281,#3893,.T.);
#27806=EDGE_CURVE('',#22282,#21886,#19688,.T.);
#27807=EDGE_CURVE('',#22282,#22283,#1521,.T.);
#27808=EDGE_CURVE('',#22283,#22284,#3894,.T.);
#27809=EDGE_CURVE('',#22284,#22285,#1522,.T.);
#27810=EDGE_CURVE('',#22285,#22286,#1523,.T.);
#27811=EDGE_CURVE('',#22286,#22287,#1524,.T.);
#27812=EDGE_CURVE('',#22287,#22288,#1525,.T.);
#27813=EDGE_CURVE('',#22288,#22289,#1526,.T.);
#27814=EDGE_CURVE('',#22289,#22290,#3895,.T.);
#27815=EDGE_CURVE('',#22290,#22291,#1527,.T.);
#27816=EDGE_CURVE('',#22291,#22292,#1528,.T.);
#27817=EDGE_CURVE('',#22292,#22293,#1529,.T.);
#27818=EDGE_CURVE('',#22293,#22294,#1530,.T.);
#27819=EDGE_CURVE('',#22294,#22295,#1531,.T.);
#27820=EDGE_CURVE('',#22295,#21487,#3896,.T.);
#27821=EDGE_CURVE('',#21455,#22295,#3897,.T.);
#27822=EDGE_CURVE('',#21456,#22294,#3898,.T.);
#27823=EDGE_CURVE('',#21457,#22293,#3899,.T.);
#27824=EDGE_CURVE('',#21458,#22292,#3900,.T.);
#27825=EDGE_CURVE('',#21459,#22291,#3901,.T.);
#27826=EDGE_CURVE('',#21460,#22290,#3902,.T.);
#27827=EDGE_CURVE('',#21461,#22289,#3903,.T.);
#27828=EDGE_CURVE('',#21462,#22288,#3904,.T.);
#27829=EDGE_CURVE('',#21463,#22287,#3905,.T.);
#27830=EDGE_CURVE('',#21464,#22286,#3906,.T.);
#27831=EDGE_CURVE('',#21465,#22285,#3907,.T.);
#27832=EDGE_CURVE('',#21466,#22284,#3908,.T.);
#27833=EDGE_CURVE('',#21467,#22283,#3909,.T.);
#27834=EDGE_CURVE('',#22092,#22282,#19102,.T.);
#27835=EDGE_CURVE('',#22296,#21883,#3910,.T.);
#27836=EDGE_CURVE('',#21471,#22296,#3911,.T.);
#27837=EDGE_CURVE('',#22297,#22296,#1532,.T.);
#27838=EDGE_CURVE('',#21472,#22297,#3912,.T.);
#27839=EDGE_CURVE('',#22298,#22297,#1533,.T.);
#27840=EDGE_CURVE('',#21473,#22298,#3913,.T.);
#27841=EDGE_CURVE('',#22299,#22298,#1534,.T.);
#27842=EDGE_CURVE('',#21474,#22299,#3914,.T.);
#27843=EDGE_CURVE('',#22300,#22299,#1535,.T.);
#27844=EDGE_CURVE('',#21475,#22300,#3915,.T.);
#27845=EDGE_CURVE('',#22301,#22300,#1536,.T.);
#27846=EDGE_CURVE('',#21476,#22301,#3916,.T.);
#27847=EDGE_CURVE('',#22302,#22301,#3917,.T.);
#27848=EDGE_CURVE('',#21477,#22302,#3918,.T.);
#27849=EDGE_CURVE('',#22303,#22302,#1537,.T.);
#27850=EDGE_CURVE('',#21478,#22303,#3919,.T.);
#27851=EDGE_CURVE('',#22304,#22303,#1538,.T.);
#27852=EDGE_CURVE('',#21479,#22304,#3920,.T.);
#27853=EDGE_CURVE('',#22305,#22304,#1539,.T.);
#27854=EDGE_CURVE('',#21480,#22305,#3921,.T.);
#27855=EDGE_CURVE('',#22306,#22305,#1540,.T.);
#27856=EDGE_CURVE('',#21481,#22306,#3922,.T.);
#27857=EDGE_CURVE('',#22307,#22306,#1541,.T.);
#27858=EDGE_CURVE('',#21482,#22307,#3923,.T.);
#27859=EDGE_CURVE('',#21962,#22307,#3924,.T.);
#27860=EDGE_CURVE('',#22308,#21882,#19689,.T.);
#27861=EDGE_CURVE('',#22308,#22309,#1542,.T.);
#27862=EDGE_CURVE('',#22309,#22310,#3925,.T.);
#27863=EDGE_CURVE('',#22310,#22311,#1543,.T.);
#27864=EDGE_CURVE('',#22311,#22312,#1544,.T.);
#27865=EDGE_CURVE('',#22312,#22313,#1545,.T.);
#27866=EDGE_CURVE('',#22313,#22314,#1546,.T.);
#27867=EDGE_CURVE('',#22314,#22315,#1547,.T.);
#27868=EDGE_CURVE('',#22315,#22316,#3926,.T.);
#27869=EDGE_CURVE('',#22316,#22317,#1548,.T.);
#27870=EDGE_CURVE('',#22317,#22318,#1549,.T.);
#27871=EDGE_CURVE('',#22318,#22319,#1550,.T.);
#27872=EDGE_CURVE('',#22319,#22320,#1551,.T.);
#27873=EDGE_CURVE('',#22320,#22321,#1552,.T.);
#27874=EDGE_CURVE('',#22321,#21453,#3927,.T.);
#27875=EDGE_CURVE('',#21421,#22321,#3928,.T.);
#27876=EDGE_CURVE('',#21422,#22320,#3929,.T.);
#27877=EDGE_CURVE('',#21423,#22319,#3930,.T.);
#27878=EDGE_CURVE('',#21424,#22318,#3931,.T.);
#27879=EDGE_CURVE('',#21425,#22317,#3932,.T.);
#27880=EDGE_CURVE('',#21426,#22316,#3933,.T.);
#27881=EDGE_CURVE('',#21427,#22315,#3934,.T.);
#27882=EDGE_CURVE('',#21428,#22314,#3935,.T.);
#27883=EDGE_CURVE('',#21429,#22313,#3936,.T.);
#27884=EDGE_CURVE('',#21430,#22312,#3937,.T.);
#27885=EDGE_CURVE('',#21431,#22311,#3938,.T.);
#27886=EDGE_CURVE('',#21432,#22310,#3939,.T.);
#27887=EDGE_CURVE('',#21433,#22309,#3940,.T.);
#27888=EDGE_CURVE('',#22093,#22308,#19103,.T.);
#27889=EDGE_CURVE('',#22322,#21879,#3941,.T.);
#27890=EDGE_CURVE('',#21437,#22322,#3942,.T.);
#27891=EDGE_CURVE('',#22323,#22322,#1553,.T.);
#27892=EDGE_CURVE('',#21438,#22323,#3943,.T.);
#27893=EDGE_CURVE('',#22324,#22323,#1554,.T.);
#27894=EDGE_CURVE('',#21439,#22324,#3944,.T.);
#27895=EDGE_CURVE('',#22325,#22324,#1555,.T.);
#27896=EDGE_CURVE('',#21440,#22325,#3945,.T.);
#27897=EDGE_CURVE('',#22326,#22325,#1556,.T.);
#27898=EDGE_CURVE('',#21441,#22326,#3946,.T.);
#27899=EDGE_CURVE('',#22327,#22326,#1557,.T.);
#27900=EDGE_CURVE('',#21442,#22327,#3947,.T.);
#27901=EDGE_CURVE('',#22328,#22327,#3948,.T.);
#27902=EDGE_CURVE('',#21443,#22328,#3949,.T.);
#27903=EDGE_CURVE('',#22329,#22328,#1558,.T.);
#27904=EDGE_CURVE('',#21444,#22329,#3950,.T.);
#27905=EDGE_CURVE('',#22330,#22329,#1559,.T.);
#27906=EDGE_CURVE('',#21445,#22330,#3951,.T.);
#27907=EDGE_CURVE('',#22331,#22330,#1560,.T.);
#27908=EDGE_CURVE('',#21446,#22331,#3952,.T.);
#27909=EDGE_CURVE('',#22332,#22331,#1561,.T.);
#27910=EDGE_CURVE('',#21447,#22332,#3953,.T.);
#27911=EDGE_CURVE('',#22333,#22332,#1562,.T.);
#27912=EDGE_CURVE('',#21448,#22333,#3954,.T.);
#27913=EDGE_CURVE('',#21965,#22333,#3955,.T.);
#27914=EDGE_CURVE('',#22334,#21878,#19690,.T.);
#27915=EDGE_CURVE('',#22334,#22335,#1563,.T.);
#27916=EDGE_CURVE('',#22335,#22336,#3956,.T.);
#27917=EDGE_CURVE('',#22336,#22337,#1564,.T.);
#27918=EDGE_CURVE('',#22337,#22338,#1565,.T.);
#27919=EDGE_CURVE('',#22338,#22339,#1566,.T.);
#27920=EDGE_CURVE('',#22339,#22340,#1567,.T.);
#27921=EDGE_CURVE('',#22340,#22341,#1568,.T.);
#27922=EDGE_CURVE('',#22341,#22342,#3957,.T.);
#27923=EDGE_CURVE('',#22342,#22343,#1569,.T.);
#27924=EDGE_CURVE('',#22343,#22344,#1570,.T.);
#27925=EDGE_CURVE('',#22344,#22345,#1571,.T.);
#27926=EDGE_CURVE('',#22345,#22346,#1572,.T.);
#27927=EDGE_CURVE('',#22346,#22347,#1573,.T.);
#27928=EDGE_CURVE('',#22347,#21419,#3958,.T.);
#27929=EDGE_CURVE('',#21387,#22347,#3959,.T.);
#27930=EDGE_CURVE('',#21388,#22346,#3960,.T.);
#27931=EDGE_CURVE('',#21389,#22345,#3961,.T.);
#27932=EDGE_CURVE('',#21390,#22344,#3962,.T.);
#27933=EDGE_CURVE('',#21391,#22343,#3963,.T.);
#27934=EDGE_CURVE('',#21392,#22342,#3964,.T.);
#27935=EDGE_CURVE('',#21393,#22341,#3965,.T.);
#27936=EDGE_CURVE('',#21394,#22340,#3966,.T.);
#27937=EDGE_CURVE('',#21395,#22339,#3967,.T.);
#27938=EDGE_CURVE('',#21396,#22338,#3968,.T.);
#27939=EDGE_CURVE('',#21397,#22337,#3969,.T.);
#27940=EDGE_CURVE('',#21398,#22336,#3970,.T.);
#27941=EDGE_CURVE('',#21399,#22335,#3971,.T.);
#27942=EDGE_CURVE('',#22094,#22334,#19104,.T.);
#27943=EDGE_CURVE('',#22348,#21875,#3972,.T.);
#27944=EDGE_CURVE('',#21403,#22348,#3973,.T.);
#27945=EDGE_CURVE('',#22349,#22348,#1574,.T.);
#27946=EDGE_CURVE('',#21404,#22349,#3974,.T.);
#27947=EDGE_CURVE('',#22350,#22349,#1575,.T.);
#27948=EDGE_CURVE('',#21405,#22350,#3975,.T.);
#27949=EDGE_CURVE('',#22351,#22350,#1576,.T.);
#27950=EDGE_CURVE('',#21406,#22351,#3976,.T.);
#27951=EDGE_CURVE('',#22352,#22351,#1577,.T.);
#27952=EDGE_CURVE('',#21407,#22352,#3977,.T.);
#27953=EDGE_CURVE('',#22353,#22352,#1578,.T.);
#27954=EDGE_CURVE('',#21408,#22353,#3978,.T.);
#27955=EDGE_CURVE('',#22354,#22353,#3979,.T.);
#27956=EDGE_CURVE('',#21409,#22354,#3980,.T.);
#27957=EDGE_CURVE('',#22355,#22354,#1579,.T.);
#27958=EDGE_CURVE('',#21410,#22355,#3981,.T.);
#27959=EDGE_CURVE('',#22356,#22355,#1580,.T.);
#27960=EDGE_CURVE('',#21411,#22356,#3982,.T.);
#27961=EDGE_CURVE('',#22357,#22356,#1581,.T.);
#27962=EDGE_CURVE('',#21412,#22357,#3983,.T.);
#27963=EDGE_CURVE('',#22358,#22357,#1582,.T.);
#27964=EDGE_CURVE('',#21413,#22358,#3984,.T.);
#27965=EDGE_CURVE('',#22359,#22358,#1583,.T.);
#27966=EDGE_CURVE('',#21414,#22359,#3985,.T.);
#27967=EDGE_CURVE('',#21968,#22359,#3986,.T.);
#27968=EDGE_CURVE('',#22360,#21874,#19691,.T.);
#27969=EDGE_CURVE('',#22360,#22361,#1584,.T.);
#27970=EDGE_CURVE('',#22361,#22362,#3987,.T.);
#27971=EDGE_CURVE('',#22362,#22363,#1585,.T.);
#27972=EDGE_CURVE('',#22363,#22364,#1586,.T.);
#27973=EDGE_CURVE('',#22364,#22365,#1587,.T.);
#27974=EDGE_CURVE('',#22365,#22366,#1588,.T.);
#27975=EDGE_CURVE('',#22366,#22367,#1589,.T.);
#27976=EDGE_CURVE('',#22367,#22368,#3988,.T.);
#27977=EDGE_CURVE('',#22368,#22369,#1590,.T.);
#27978=EDGE_CURVE('',#22369,#22370,#1591,.T.);
#27979=EDGE_CURVE('',#22370,#22371,#1592,.T.);
#27980=EDGE_CURVE('',#22371,#22372,#1593,.T.);
#27981=EDGE_CURVE('',#22372,#22373,#1594,.T.);
#27982=EDGE_CURVE('',#22373,#21385,#3989,.T.);
#27983=EDGE_CURVE('',#21353,#22373,#3990,.T.);
#27984=EDGE_CURVE('',#21354,#22372,#3991,.T.);
#27985=EDGE_CURVE('',#21355,#22371,#3992,.T.);
#27986=EDGE_CURVE('',#21356,#22370,#3993,.T.);
#27987=EDGE_CURVE('',#21357,#22369,#3994,.T.);
#27988=EDGE_CURVE('',#21358,#22368,#3995,.T.);
#27989=EDGE_CURVE('',#21359,#22367,#3996,.T.);
#27990=EDGE_CURVE('',#21360,#22366,#3997,.T.);
#27991=EDGE_CURVE('',#21361,#22365,#3998,.T.);
#27992=EDGE_CURVE('',#21362,#22364,#3999,.T.);
#27993=EDGE_CURVE('',#21363,#22363,#4000,.T.);
#27994=EDGE_CURVE('',#21364,#22362,#4001,.T.);
#27995=EDGE_CURVE('',#21365,#22361,#4002,.T.);
#27996=EDGE_CURVE('',#22095,#22360,#19105,.T.);
#27997=EDGE_CURVE('',#22374,#21871,#4003,.T.);
#27998=EDGE_CURVE('',#21369,#22374,#4004,.T.);
#27999=EDGE_CURVE('',#22375,#22374,#1595,.T.);
#28000=EDGE_CURVE('',#21370,#22375,#4005,.T.);
#28001=EDGE_CURVE('',#22376,#22375,#1596,.T.);
#28002=EDGE_CURVE('',#21371,#22376,#4006,.T.);
#28003=EDGE_CURVE('',#22377,#22376,#1597,.T.);
#28004=EDGE_CURVE('',#21372,#22377,#4007,.T.);
#28005=EDGE_CURVE('',#22378,#22377,#1598,.T.);
#28006=EDGE_CURVE('',#21373,#22378,#4008,.T.);
#28007=EDGE_CURVE('',#22379,#22378,#1599,.T.);
#28008=EDGE_CURVE('',#21374,#22379,#4009,.T.);
#28009=EDGE_CURVE('',#22380,#22379,#4010,.T.);
#28010=EDGE_CURVE('',#21375,#22380,#4011,.T.);
#28011=EDGE_CURVE('',#22381,#22380,#1600,.T.);
#28012=EDGE_CURVE('',#21376,#22381,#4012,.T.);
#28013=EDGE_CURVE('',#22382,#22381,#1601,.T.);
#28014=EDGE_CURVE('',#21377,#22382,#4013,.T.);
#28015=EDGE_CURVE('',#22383,#22382,#1602,.T.);
#28016=EDGE_CURVE('',#21378,#22383,#4014,.T.);
#28017=EDGE_CURVE('',#22384,#22383,#1603,.T.);
#28018=EDGE_CURVE('',#21379,#22384,#4015,.T.);
#28019=EDGE_CURVE('',#22385,#22384,#1604,.T.);
#28020=EDGE_CURVE('',#21380,#22385,#4016,.T.);
#28021=EDGE_CURVE('',#21971,#22385,#4017,.T.);
#28022=EDGE_CURVE('',#22386,#21870,#19692,.T.);
#28023=EDGE_CURVE('',#22386,#22387,#1605,.T.);
#28024=EDGE_CURVE('',#22387,#22388,#4018,.T.);
#28025=EDGE_CURVE('',#22388,#22389,#1606,.T.);
#28026=EDGE_CURVE('',#22389,#22390,#1607,.T.);
#28027=EDGE_CURVE('',#22390,#22391,#1608,.T.);
#28028=EDGE_CURVE('',#22391,#22392,#1609,.T.);
#28029=EDGE_CURVE('',#22392,#22393,#1610,.T.);
#28030=EDGE_CURVE('',#22393,#22394,#4019,.T.);
#28031=EDGE_CURVE('',#22394,#22395,#1611,.T.);
#28032=EDGE_CURVE('',#22395,#22396,#1612,.T.);
#28033=EDGE_CURVE('',#22396,#22397,#1613,.T.);
#28034=EDGE_CURVE('',#22397,#22398,#1614,.T.);
#28035=EDGE_CURVE('',#22398,#22399,#1615,.T.);
#28036=EDGE_CURVE('',#22399,#21351,#4020,.T.);
#28037=EDGE_CURVE('',#21319,#22399,#4021,.T.);
#28038=EDGE_CURVE('',#21320,#22398,#4022,.T.);
#28039=EDGE_CURVE('',#21321,#22397,#4023,.T.);
#28040=EDGE_CURVE('',#21322,#22396,#4024,.T.);
#28041=EDGE_CURVE('',#21323,#22395,#4025,.T.);
#28042=EDGE_CURVE('',#21324,#22394,#4026,.T.);
#28043=EDGE_CURVE('',#21325,#22393,#4027,.T.);
#28044=EDGE_CURVE('',#21326,#22392,#4028,.T.);
#28045=EDGE_CURVE('',#21327,#22391,#4029,.T.);
#28046=EDGE_CURVE('',#21328,#22390,#4030,.T.);
#28047=EDGE_CURVE('',#21329,#22389,#4031,.T.);
#28048=EDGE_CURVE('',#21330,#22388,#4032,.T.);
#28049=EDGE_CURVE('',#21331,#22387,#4033,.T.);
#28050=EDGE_CURVE('',#22096,#22386,#19106,.T.);
#28051=EDGE_CURVE('',#22400,#21867,#4034,.T.);
#28052=EDGE_CURVE('',#21335,#22400,#4035,.T.);
#28053=EDGE_CURVE('',#22401,#22400,#1616,.T.);
#28054=EDGE_CURVE('',#21336,#22401,#4036,.T.);
#28055=EDGE_CURVE('',#22402,#22401,#1617,.T.);
#28056=EDGE_CURVE('',#21337,#22402,#4037,.T.);
#28057=EDGE_CURVE('',#22403,#22402,#1618,.T.);
#28058=EDGE_CURVE('',#21338,#22403,#4038,.T.);
#28059=EDGE_CURVE('',#22404,#22403,#1619,.T.);
#28060=EDGE_CURVE('',#21339,#22404,#4039,.T.);
#28061=EDGE_CURVE('',#22405,#22404,#1620,.T.);
#28062=EDGE_CURVE('',#21340,#22405,#4040,.T.);
#28063=EDGE_CURVE('',#22406,#22405,#4041,.T.);
#28064=EDGE_CURVE('',#21341,#22406,#4042,.T.);
#28065=EDGE_CURVE('',#22407,#22406,#1621,.T.);
#28066=EDGE_CURVE('',#21342,#22407,#4043,.T.);
#28067=EDGE_CURVE('',#22408,#22407,#1622,.T.);
#28068=EDGE_CURVE('',#21343,#22408,#4044,.T.);
#28069=EDGE_CURVE('',#22409,#22408,#1623,.T.);
#28070=EDGE_CURVE('',#21344,#22409,#4045,.T.);
#28071=EDGE_CURVE('',#22410,#22409,#1624,.T.);
#28072=EDGE_CURVE('',#21345,#22410,#4046,.T.);
#28073=EDGE_CURVE('',#22411,#22410,#1625,.T.);
#28074=EDGE_CURVE('',#21346,#22411,#4047,.T.);
#28075=EDGE_CURVE('',#21974,#22411,#4048,.T.);
#28076=EDGE_CURVE('',#22412,#21866,#19693,.T.);
#28077=EDGE_CURVE('',#22412,#22413,#1626,.T.);
#28078=EDGE_CURVE('',#22413,#22414,#4049,.T.);
#28079=EDGE_CURVE('',#22414,#22415,#1627,.T.);
#28080=EDGE_CURVE('',#22415,#22416,#1628,.T.);
#28081=EDGE_CURVE('',#22416,#22417,#1629,.T.);
#28082=EDGE_CURVE('',#22417,#22418,#1630,.T.);
#28083=EDGE_CURVE('',#22418,#22419,#1631,.T.);
#28084=EDGE_CURVE('',#22419,#22420,#4050,.T.);
#28085=EDGE_CURVE('',#22420,#22421,#1632,.T.);
#28086=EDGE_CURVE('',#22421,#22422,#1633,.T.);
#28087=EDGE_CURVE('',#22422,#22423,#1634,.T.);
#28088=EDGE_CURVE('',#22423,#22424,#1635,.T.);
#28089=EDGE_CURVE('',#22424,#22425,#1636,.T.);
#28090=EDGE_CURVE('',#22425,#21317,#4051,.T.);
#28091=EDGE_CURVE('',#21285,#22425,#4052,.T.);
#28092=EDGE_CURVE('',#21286,#22424,#4053,.T.);
#28093=EDGE_CURVE('',#21287,#22423,#4054,.T.);
#28094=EDGE_CURVE('',#21288,#22422,#4055,.T.);
#28095=EDGE_CURVE('',#21289,#22421,#4056,.T.);
#28096=EDGE_CURVE('',#21290,#22420,#4057,.T.);
#28097=EDGE_CURVE('',#21291,#22419,#4058,.T.);
#28098=EDGE_CURVE('',#21292,#22418,#4059,.T.);
#28099=EDGE_CURVE('',#21293,#22417,#4060,.T.);
#28100=EDGE_CURVE('',#21294,#22416,#4061,.T.);
#28101=EDGE_CURVE('',#21295,#22415,#4062,.T.);
#28102=EDGE_CURVE('',#21296,#22414,#4063,.T.);
#28103=EDGE_CURVE('',#21297,#22413,#4064,.T.);
#28104=EDGE_CURVE('',#22097,#22412,#19107,.T.);
#28105=EDGE_CURVE('',#22426,#21863,#4065,.T.);
#28106=EDGE_CURVE('',#21301,#22426,#4066,.T.);
#28107=EDGE_CURVE('',#22427,#22426,#1637,.T.);
#28108=EDGE_CURVE('',#21302,#22427,#4067,.T.);
#28109=EDGE_CURVE('',#22428,#22427,#1638,.T.);
#28110=EDGE_CURVE('',#21303,#22428,#4068,.T.);
#28111=EDGE_CURVE('',#22429,#22428,#1639,.T.);
#28112=EDGE_CURVE('',#21304,#22429,#4069,.T.);
#28113=EDGE_CURVE('',#22430,#22429,#1640,.T.);
#28114=EDGE_CURVE('',#21305,#22430,#4070,.T.);
#28115=EDGE_CURVE('',#22431,#22430,#1641,.T.);
#28116=EDGE_CURVE('',#21306,#22431,#4071,.T.);
#28117=EDGE_CURVE('',#22432,#22431,#4072,.T.);
#28118=EDGE_CURVE('',#21307,#22432,#4073,.T.);
#28119=EDGE_CURVE('',#22433,#22432,#1642,.T.);
#28120=EDGE_CURVE('',#21308,#22433,#4074,.T.);
#28121=EDGE_CURVE('',#22434,#22433,#1643,.T.);
#28122=EDGE_CURVE('',#21309,#22434,#4075,.T.);
#28123=EDGE_CURVE('',#22435,#22434,#1644,.T.);
#28124=EDGE_CURVE('',#21310,#22435,#4076,.T.);
#28125=EDGE_CURVE('',#22436,#22435,#1645,.T.);
#28126=EDGE_CURVE('',#21311,#22436,#4077,.T.);
#28127=EDGE_CURVE('',#22437,#22436,#1646,.T.);
#28128=EDGE_CURVE('',#21312,#22437,#4078,.T.);
#28129=EDGE_CURVE('',#21977,#22437,#4079,.T.);
#28130=EDGE_CURVE('',#22438,#21862,#19694,.T.);
#28131=EDGE_CURVE('',#22438,#22439,#1647,.T.);
#28132=EDGE_CURVE('',#22439,#22440,#4080,.T.);
#28133=EDGE_CURVE('',#22440,#22441,#1648,.T.);
#28134=EDGE_CURVE('',#22441,#22442,#1649,.T.);
#28135=EDGE_CURVE('',#22442,#22443,#1650,.T.);
#28136=EDGE_CURVE('',#22443,#22444,#1651,.T.);
#28137=EDGE_CURVE('',#22444,#22445,#1652,.T.);
#28138=EDGE_CURVE('',#22445,#22446,#4081,.T.);
#28139=EDGE_CURVE('',#22446,#22447,#1653,.T.);
#28140=EDGE_CURVE('',#22447,#22448,#1654,.T.);
#28141=EDGE_CURVE('',#22448,#22449,#1655,.T.);
#28142=EDGE_CURVE('',#22449,#22450,#1656,.T.);
#28143=EDGE_CURVE('',#22450,#22451,#1657,.T.);
#28144=EDGE_CURVE('',#22451,#21283,#4082,.T.);
#28145=EDGE_CURVE('',#21251,#22451,#4083,.T.);
#28146=EDGE_CURVE('',#21252,#22450,#4084,.T.);
#28147=EDGE_CURVE('',#21253,#22449,#4085,.T.);
#28148=EDGE_CURVE('',#21254,#22448,#4086,.T.);
#28149=EDGE_CURVE('',#21255,#22447,#4087,.T.);
#28150=EDGE_CURVE('',#21256,#22446,#4088,.T.);
#28151=EDGE_CURVE('',#21257,#22445,#4089,.T.);
#28152=EDGE_CURVE('',#21258,#22444,#4090,.T.);
#28153=EDGE_CURVE('',#21259,#22443,#4091,.T.);
#28154=EDGE_CURVE('',#21260,#22442,#4092,.T.);
#28155=EDGE_CURVE('',#21261,#22441,#4093,.T.);
#28156=EDGE_CURVE('',#21262,#22440,#4094,.T.);
#28157=EDGE_CURVE('',#21263,#22439,#4095,.T.);
#28158=EDGE_CURVE('',#22098,#22438,#19108,.T.);
#28159=EDGE_CURVE('',#22452,#21859,#4096,.T.);
#28160=EDGE_CURVE('',#21267,#22452,#4097,.T.);
#28161=EDGE_CURVE('',#22453,#22452,#1658,.T.);
#28162=EDGE_CURVE('',#21268,#22453,#4098,.T.);
#28163=EDGE_CURVE('',#22454,#22453,#1659,.T.);
#28164=EDGE_CURVE('',#21269,#22454,#4099,.T.);
#28165=EDGE_CURVE('',#22455,#22454,#1660,.T.);
#28166=EDGE_CURVE('',#21270,#22455,#4100,.T.);
#28167=EDGE_CURVE('',#22456,#22455,#1661,.T.);
#28168=EDGE_CURVE('',#21271,#22456,#4101,.T.);
#28169=EDGE_CURVE('',#22457,#22456,#1662,.T.);
#28170=EDGE_CURVE('',#21272,#22457,#4102,.T.);
#28171=EDGE_CURVE('',#22458,#22457,#4103,.T.);
#28172=EDGE_CURVE('',#21273,#22458,#4104,.T.);
#28173=EDGE_CURVE('',#22459,#22458,#1663,.T.);
#28174=EDGE_CURVE('',#21274,#22459,#4105,.T.);
#28175=EDGE_CURVE('',#22460,#22459,#1664,.T.);
#28176=EDGE_CURVE('',#21275,#22460,#4106,.T.);
#28177=EDGE_CURVE('',#22461,#22460,#1665,.T.);
#28178=EDGE_CURVE('',#21276,#22461,#4107,.T.);
#28179=EDGE_CURVE('',#22462,#22461,#1666,.T.);
#28180=EDGE_CURVE('',#21277,#22462,#4108,.T.);
#28181=EDGE_CURVE('',#22463,#22462,#1667,.T.);
#28182=EDGE_CURVE('',#21278,#22463,#4109,.T.);
#28183=EDGE_CURVE('',#21980,#22463,#4110,.T.);
#28184=EDGE_CURVE('',#22464,#21858,#19695,.T.);
#28185=EDGE_CURVE('',#22464,#22465,#1668,.T.);
#28186=EDGE_CURVE('',#22465,#22466,#4111,.T.);
#28187=EDGE_CURVE('',#22466,#22467,#1669,.T.);
#28188=EDGE_CURVE('',#22467,#22468,#1670,.T.);
#28189=EDGE_CURVE('',#22468,#22469,#1671,.T.);
#28190=EDGE_CURVE('',#22469,#22470,#1672,.T.);
#28191=EDGE_CURVE('',#22470,#22471,#1673,.T.);
#28192=EDGE_CURVE('',#22471,#22472,#4112,.T.);
#28193=EDGE_CURVE('',#22472,#22473,#1674,.T.);
#28194=EDGE_CURVE('',#22473,#22474,#1675,.T.);
#28195=EDGE_CURVE('',#22474,#22475,#1676,.T.);
#28196=EDGE_CURVE('',#22475,#22476,#1677,.T.);
#28197=EDGE_CURVE('',#22476,#22477,#1678,.T.);
#28198=EDGE_CURVE('',#22477,#21249,#4113,.T.);
#28199=EDGE_CURVE('',#21217,#22477,#4114,.T.);
#28200=EDGE_CURVE('',#21218,#22476,#4115,.T.);
#28201=EDGE_CURVE('',#21219,#22475,#4116,.T.);
#28202=EDGE_CURVE('',#21220,#22474,#4117,.T.);
#28203=EDGE_CURVE('',#21221,#22473,#4118,.T.);
#28204=EDGE_CURVE('',#21222,#22472,#4119,.T.);
#28205=EDGE_CURVE('',#21223,#22471,#4120,.T.);
#28206=EDGE_CURVE('',#21224,#22470,#4121,.T.);
#28207=EDGE_CURVE('',#21225,#22469,#4122,.T.);
#28208=EDGE_CURVE('',#21226,#22468,#4123,.T.);
#28209=EDGE_CURVE('',#21227,#22467,#4124,.T.);
#28210=EDGE_CURVE('',#21228,#22466,#4125,.T.);
#28211=EDGE_CURVE('',#21229,#22465,#4126,.T.);
#28212=EDGE_CURVE('',#22099,#22464,#19109,.T.);
#28213=EDGE_CURVE('',#22478,#21855,#4127,.T.);
#28214=EDGE_CURVE('',#21233,#22478,#4128,.T.);
#28215=EDGE_CURVE('',#22479,#22478,#1679,.T.);
#28216=EDGE_CURVE('',#21234,#22479,#4129,.T.);
#28217=EDGE_CURVE('',#22480,#22479,#1680,.T.);
#28218=EDGE_CURVE('',#21235,#22480,#4130,.T.);
#28219=EDGE_CURVE('',#22481,#22480,#1681,.T.);
#28220=EDGE_CURVE('',#21236,#22481,#4131,.T.);
#28221=EDGE_CURVE('',#22482,#22481,#1682,.T.);
#28222=EDGE_CURVE('',#21237,#22482,#4132,.T.);
#28223=EDGE_CURVE('',#22483,#22482,#1683,.T.);
#28224=EDGE_CURVE('',#21238,#22483,#4133,.T.);
#28225=EDGE_CURVE('',#22484,#22483,#4134,.T.);
#28226=EDGE_CURVE('',#21239,#22484,#4135,.T.);
#28227=EDGE_CURVE('',#22485,#22484,#1684,.T.);
#28228=EDGE_CURVE('',#21240,#22485,#4136,.T.);
#28229=EDGE_CURVE('',#22486,#22485,#1685,.T.);
#28230=EDGE_CURVE('',#21241,#22486,#4137,.T.);
#28231=EDGE_CURVE('',#22487,#22486,#1686,.T.);
#28232=EDGE_CURVE('',#21242,#22487,#4138,.T.);
#28233=EDGE_CURVE('',#22488,#22487,#1687,.T.);
#28234=EDGE_CURVE('',#21243,#22488,#4139,.T.);
#28235=EDGE_CURVE('',#22489,#22488,#1688,.T.);
#28236=EDGE_CURVE('',#21244,#22489,#4140,.T.);
#28237=EDGE_CURVE('',#21983,#22489,#4141,.T.);
#28238=EDGE_CURVE('',#22490,#21854,#19696,.T.);
#28239=EDGE_CURVE('',#22490,#22491,#1689,.T.);
#28240=EDGE_CURVE('',#22491,#22492,#4142,.T.);
#28241=EDGE_CURVE('',#22492,#22493,#1690,.T.);
#28242=EDGE_CURVE('',#22493,#22494,#1691,.T.);
#28243=EDGE_CURVE('',#22494,#22495,#1692,.T.);
#28244=EDGE_CURVE('',#22495,#22496,#1693,.T.);
#28245=EDGE_CURVE('',#22496,#22497,#1694,.T.);
#28246=EDGE_CURVE('',#22497,#22498,#4143,.T.);
#28247=EDGE_CURVE('',#22498,#22499,#1695,.T.);
#28248=EDGE_CURVE('',#22499,#22500,#1696,.T.);
#28249=EDGE_CURVE('',#22500,#22501,#1697,.T.);
#28250=EDGE_CURVE('',#22501,#22502,#1698,.T.);
#28251=EDGE_CURVE('',#22502,#22503,#1699,.T.);
#28252=EDGE_CURVE('',#22503,#21215,#4144,.T.);
#28253=EDGE_CURVE('',#21183,#22503,#4145,.T.);
#28254=EDGE_CURVE('',#21184,#22502,#4146,.T.);
#28255=EDGE_CURVE('',#21185,#22501,#4147,.T.);
#28256=EDGE_CURVE('',#21186,#22500,#4148,.T.);
#28257=EDGE_CURVE('',#21187,#22499,#4149,.T.);
#28258=EDGE_CURVE('',#21188,#22498,#4150,.T.);
#28259=EDGE_CURVE('',#21189,#22497,#4151,.T.);
#28260=EDGE_CURVE('',#21190,#22496,#4152,.T.);
#28261=EDGE_CURVE('',#21191,#22495,#4153,.T.);
#28262=EDGE_CURVE('',#21192,#22494,#4154,.T.);
#28263=EDGE_CURVE('',#21193,#22493,#4155,.T.);
#28264=EDGE_CURVE('',#21194,#22492,#4156,.T.);
#28265=EDGE_CURVE('',#21195,#22491,#4157,.T.);
#28266=EDGE_CURVE('',#22100,#22490,#19110,.T.);
#28267=EDGE_CURVE('',#22504,#21851,#4158,.T.);
#28268=EDGE_CURVE('',#21199,#22504,#4159,.T.);
#28269=EDGE_CURVE('',#22505,#22504,#1700,.T.);
#28270=EDGE_CURVE('',#21200,#22505,#4160,.T.);
#28271=EDGE_CURVE('',#22506,#22505,#1701,.T.);
#28272=EDGE_CURVE('',#21201,#22506,#4161,.T.);
#28273=EDGE_CURVE('',#22507,#22506,#1702,.T.);
#28274=EDGE_CURVE('',#21202,#22507,#4162,.T.);
#28275=EDGE_CURVE('',#22508,#22507,#1703,.T.);
#28276=EDGE_CURVE('',#21203,#22508,#4163,.T.);
#28277=EDGE_CURVE('',#22509,#22508,#1704,.T.);
#28278=EDGE_CURVE('',#21204,#22509,#4164,.T.);
#28279=EDGE_CURVE('',#22510,#22509,#4165,.T.);
#28280=EDGE_CURVE('',#21205,#22510,#4166,.T.);
#28281=EDGE_CURVE('',#22511,#22510,#1705,.T.);
#28282=EDGE_CURVE('',#21206,#22511,#4167,.T.);
#28283=EDGE_CURVE('',#22512,#22511,#1706,.T.);
#28284=EDGE_CURVE('',#21207,#22512,#4168,.T.);
#28285=EDGE_CURVE('',#22513,#22512,#1707,.T.);
#28286=EDGE_CURVE('',#21208,#22513,#4169,.T.);
#28287=EDGE_CURVE('',#22514,#22513,#1708,.T.);
#28288=EDGE_CURVE('',#21209,#22514,#4170,.T.);
#28289=EDGE_CURVE('',#22515,#22514,#1709,.T.);
#28290=EDGE_CURVE('',#21210,#22515,#4171,.T.);
#28291=EDGE_CURVE('',#21986,#22515,#4172,.T.);
#28292=EDGE_CURVE('',#22516,#21850,#19697,.T.);
#28293=EDGE_CURVE('',#22516,#22517,#1710,.T.);
#28294=EDGE_CURVE('',#22517,#22518,#4173,.T.);
#28295=EDGE_CURVE('',#22518,#22519,#1711,.T.);
#28296=EDGE_CURVE('',#22519,#22520,#1712,.T.);
#28297=EDGE_CURVE('',#22520,#22521,#1713,.T.);
#28298=EDGE_CURVE('',#22521,#22522,#1714,.T.);
#28299=EDGE_CURVE('',#22522,#22523,#1715,.T.);
#28300=EDGE_CURVE('',#22523,#22524,#4174,.T.);
#28301=EDGE_CURVE('',#22524,#22525,#1716,.T.);
#28302=EDGE_CURVE('',#22525,#22526,#1717,.T.);
#28303=EDGE_CURVE('',#22526,#22527,#1718,.T.);
#28304=EDGE_CURVE('',#22527,#22528,#1719,.T.);
#28305=EDGE_CURVE('',#22528,#22529,#1720,.T.);
#28306=EDGE_CURVE('',#22529,#21181,#4175,.T.);
#28307=EDGE_CURVE('',#21149,#22529,#4176,.T.);
#28308=EDGE_CURVE('',#21150,#22528,#4177,.T.);
#28309=EDGE_CURVE('',#21151,#22527,#4178,.T.);
#28310=EDGE_CURVE('',#21152,#22526,#4179,.T.);
#28311=EDGE_CURVE('',#21153,#22525,#4180,.T.);
#28312=EDGE_CURVE('',#21154,#22524,#4181,.T.);
#28313=EDGE_CURVE('',#21155,#22523,#4182,.T.);
#28314=EDGE_CURVE('',#21156,#22522,#4183,.T.);
#28315=EDGE_CURVE('',#21157,#22521,#4184,.T.);
#28316=EDGE_CURVE('',#21158,#22520,#4185,.T.);
#28317=EDGE_CURVE('',#21159,#22519,#4186,.T.);
#28318=EDGE_CURVE('',#21160,#22518,#4187,.T.);
#28319=EDGE_CURVE('',#21161,#22517,#4188,.T.);
#28320=EDGE_CURVE('',#22101,#22516,#19111,.T.);
#28321=EDGE_CURVE('',#22530,#21847,#4189,.T.);
#28322=EDGE_CURVE('',#21165,#22530,#4190,.T.);
#28323=EDGE_CURVE('',#22531,#22530,#1721,.T.);
#28324=EDGE_CURVE('',#21166,#22531,#4191,.T.);
#28325=EDGE_CURVE('',#22532,#22531,#1722,.T.);
#28326=EDGE_CURVE('',#21167,#22532,#4192,.T.);
#28327=EDGE_CURVE('',#22533,#22532,#1723,.T.);
#28328=EDGE_CURVE('',#21168,#22533,#4193,.T.);
#28329=EDGE_CURVE('',#22534,#22533,#1724,.T.);
#28330=EDGE_CURVE('',#21169,#22534,#4194,.T.);
#28331=EDGE_CURVE('',#22535,#22534,#1725,.T.);
#28332=EDGE_CURVE('',#21170,#22535,#4195,.T.);
#28333=EDGE_CURVE('',#22536,#22535,#4196,.T.);
#28334=EDGE_CURVE('',#21171,#22536,#4197,.T.);
#28335=EDGE_CURVE('',#22537,#22536,#1726,.T.);
#28336=EDGE_CURVE('',#21172,#22537,#4198,.T.);
#28337=EDGE_CURVE('',#22538,#22537,#1727,.T.);
#28338=EDGE_CURVE('',#21173,#22538,#4199,.T.);
#28339=EDGE_CURVE('',#22539,#22538,#1728,.T.);
#28340=EDGE_CURVE('',#21174,#22539,#4200,.T.);
#28341=EDGE_CURVE('',#22540,#22539,#1729,.T.);
#28342=EDGE_CURVE('',#21175,#22540,#4201,.T.);
#28343=EDGE_CURVE('',#22541,#22540,#1730,.T.);
#28344=EDGE_CURVE('',#21176,#22541,#4202,.T.);
#28345=EDGE_CURVE('',#21989,#22541,#4203,.T.);
#28346=EDGE_CURVE('',#22542,#21846,#19698,.T.);
#28347=EDGE_CURVE('',#22542,#22543,#1731,.T.);
#28348=EDGE_CURVE('',#22543,#22544,#4204,.T.);
#28349=EDGE_CURVE('',#22544,#22545,#1732,.T.);
#28350=EDGE_CURVE('',#22545,#22546,#1733,.T.);
#28351=EDGE_CURVE('',#22546,#22547,#1734,.T.);
#28352=EDGE_CURVE('',#22547,#22548,#1735,.T.);
#28353=EDGE_CURVE('',#22548,#22549,#1736,.T.);
#28354=EDGE_CURVE('',#22549,#22550,#4205,.T.);
#28355=EDGE_CURVE('',#22550,#22551,#1737,.T.);
#28356=EDGE_CURVE('',#22551,#22552,#1738,.T.);
#28357=EDGE_CURVE('',#22552,#22553,#1739,.T.);
#28358=EDGE_CURVE('',#22553,#22554,#1740,.T.);
#28359=EDGE_CURVE('',#22554,#22555,#1741,.T.);
#28360=EDGE_CURVE('',#22555,#21147,#4206,.T.);
#28361=EDGE_CURVE('',#21115,#22555,#4207,.T.);
#28362=EDGE_CURVE('',#21116,#22554,#4208,.T.);
#28363=EDGE_CURVE('',#21117,#22553,#4209,.T.);
#28364=EDGE_CURVE('',#21118,#22552,#4210,.T.);
#28365=EDGE_CURVE('',#21119,#22551,#4211,.T.);
#28366=EDGE_CURVE('',#21120,#22550,#4212,.T.);
#28367=EDGE_CURVE('',#21121,#22549,#4213,.T.);
#28368=EDGE_CURVE('',#21122,#22548,#4214,.T.);
#28369=EDGE_CURVE('',#21123,#22547,#4215,.T.);
#28370=EDGE_CURVE('',#21124,#22546,#4216,.T.);
#28371=EDGE_CURVE('',#21125,#22545,#4217,.T.);
#28372=EDGE_CURVE('',#21126,#22544,#4218,.T.);
#28373=EDGE_CURVE('',#21127,#22543,#4219,.T.);
#28374=EDGE_CURVE('',#22102,#22542,#19112,.T.);
#28375=EDGE_CURVE('',#22556,#21843,#4220,.T.);
#28376=EDGE_CURVE('',#21131,#22556,#4221,.T.);
#28377=EDGE_CURVE('',#22557,#22556,#1742,.T.);
#28378=EDGE_CURVE('',#21132,#22557,#4222,.T.);
#28379=EDGE_CURVE('',#22558,#22557,#1743,.T.);
#28380=EDGE_CURVE('',#21133,#22558,#4223,.T.);
#28381=EDGE_CURVE('',#22559,#22558,#1744,.T.);
#28382=EDGE_CURVE('',#21134,#22559,#4224,.T.);
#28383=EDGE_CURVE('',#22560,#22559,#1745,.T.);
#28384=EDGE_CURVE('',#21135,#22560,#4225,.T.);
#28385=EDGE_CURVE('',#22561,#22560,#1746,.T.);
#28386=EDGE_CURVE('',#21136,#22561,#4226,.T.);
#28387=EDGE_CURVE('',#22562,#22561,#4227,.T.);
#28388=EDGE_CURVE('',#21137,#22562,#4228,.T.);
#28389=EDGE_CURVE('',#22563,#22562,#1747,.T.);
#28390=EDGE_CURVE('',#21138,#22563,#4229,.T.);
#28391=EDGE_CURVE('',#22564,#22563,#1748,.T.);
#28392=EDGE_CURVE('',#21139,#22564,#4230,.T.);
#28393=EDGE_CURVE('',#22565,#22564,#1749,.T.);
#28394=EDGE_CURVE('',#21140,#22565,#4231,.T.);
#28395=EDGE_CURVE('',#22566,#22565,#1750,.T.);
#28396=EDGE_CURVE('',#21141,#22566,#4232,.T.);
#28397=EDGE_CURVE('',#22567,#22566,#1751,.T.);
#28398=EDGE_CURVE('',#21142,#22567,#4233,.T.);
#28399=EDGE_CURVE('',#21992,#22567,#4234,.T.);
#28400=EDGE_CURVE('',#22568,#21842,#19699,.T.);
#28401=EDGE_CURVE('',#22568,#22569,#1752,.T.);
#28402=EDGE_CURVE('',#22569,#22570,#4235,.T.);
#28403=EDGE_CURVE('',#22570,#22571,#1753,.T.);
#28404=EDGE_CURVE('',#22571,#22572,#1754,.T.);
#28405=EDGE_CURVE('',#22572,#22573,#1755,.T.);
#28406=EDGE_CURVE('',#22573,#22574,#1756,.T.);
#28407=EDGE_CURVE('',#22574,#22575,#1757,.T.);
#28408=EDGE_CURVE('',#22575,#22576,#4236,.T.);
#28409=EDGE_CURVE('',#22576,#22577,#1758,.T.);
#28410=EDGE_CURVE('',#22577,#22578,#1759,.T.);
#28411=EDGE_CURVE('',#22578,#22579,#1760,.T.);
#28412=EDGE_CURVE('',#22579,#22580,#1761,.T.);
#28413=EDGE_CURVE('',#22580,#22581,#1762,.T.);
#28414=EDGE_CURVE('',#22581,#21113,#4237,.T.);
#28415=EDGE_CURVE('',#21081,#22581,#4238,.T.);
#28416=EDGE_CURVE('',#21082,#22580,#4239,.T.);
#28417=EDGE_CURVE('',#21083,#22579,#4240,.T.);
#28418=EDGE_CURVE('',#21084,#22578,#4241,.T.);
#28419=EDGE_CURVE('',#21085,#22577,#4242,.T.);
#28420=EDGE_CURVE('',#21086,#22576,#4243,.T.);
#28421=EDGE_CURVE('',#21087,#22575,#4244,.T.);
#28422=EDGE_CURVE('',#21088,#22574,#4245,.T.);
#28423=EDGE_CURVE('',#21089,#22573,#4246,.T.);
#28424=EDGE_CURVE('',#21090,#22572,#4247,.T.);
#28425=EDGE_CURVE('',#21091,#22571,#4248,.T.);
#28426=EDGE_CURVE('',#21092,#22570,#4249,.T.);
#28427=EDGE_CURVE('',#21093,#22569,#4250,.T.);
#28428=EDGE_CURVE('',#22103,#22568,#19113,.T.);
#28429=EDGE_CURVE('',#22582,#21839,#4251,.T.);
#28430=EDGE_CURVE('',#21097,#22582,#4252,.T.);
#28431=EDGE_CURVE('',#22583,#22582,#1763,.T.);
#28432=EDGE_CURVE('',#21098,#22583,#4253,.T.);
#28433=EDGE_CURVE('',#22584,#22583,#1764,.T.);
#28434=EDGE_CURVE('',#21099,#22584,#4254,.T.);
#28435=EDGE_CURVE('',#22585,#22584,#1765,.T.);
#28436=EDGE_CURVE('',#21100,#22585,#4255,.T.);
#28437=EDGE_CURVE('',#22586,#22585,#1766,.T.);
#28438=EDGE_CURVE('',#21101,#22586,#4256,.T.);
#28439=EDGE_CURVE('',#22587,#22586,#1767,.T.);
#28440=EDGE_CURVE('',#21102,#22587,#4257,.T.);
#28441=EDGE_CURVE('',#22588,#22587,#4258,.T.);
#28442=EDGE_CURVE('',#21103,#22588,#4259,.T.);
#28443=EDGE_CURVE('',#22589,#22588,#1768,.T.);
#28444=EDGE_CURVE('',#21104,#22589,#4260,.T.);
#28445=EDGE_CURVE('',#22590,#22589,#1769,.T.);
#28446=EDGE_CURVE('',#21105,#22590,#4261,.T.);
#28447=EDGE_CURVE('',#22591,#22590,#1770,.T.);
#28448=EDGE_CURVE('',#21106,#22591,#4262,.T.);
#28449=EDGE_CURVE('',#22592,#22591,#1771,.T.);
#28450=EDGE_CURVE('',#21107,#22592,#4263,.T.);
#28451=EDGE_CURVE('',#22593,#22592,#1772,.T.);
#28452=EDGE_CURVE('',#21108,#22593,#4264,.T.);
#28453=EDGE_CURVE('',#21995,#22593,#4265,.T.);
#28454=EDGE_CURVE('',#22594,#21838,#19700,.T.);
#28455=EDGE_CURVE('',#22594,#22595,#1773,.T.);
#28456=EDGE_CURVE('',#22595,#22596,#4266,.T.);
#28457=EDGE_CURVE('',#22596,#22597,#1774,.T.);
#28458=EDGE_CURVE('',#22597,#22598,#1775,.T.);
#28459=EDGE_CURVE('',#22598,#22599,#1776,.T.);
#28460=EDGE_CURVE('',#22599,#22600,#1777,.T.);
#28461=EDGE_CURVE('',#22600,#22601,#1778,.T.);
#28462=EDGE_CURVE('',#22601,#22602,#4267,.T.);
#28463=EDGE_CURVE('',#22602,#22603,#1779,.T.);
#28464=EDGE_CURVE('',#22603,#22604,#1780,.T.);
#28465=EDGE_CURVE('',#22604,#22605,#1781,.T.);
#28466=EDGE_CURVE('',#22605,#22606,#1782,.T.);
#28467=EDGE_CURVE('',#22606,#22607,#1783,.T.);
#28468=EDGE_CURVE('',#22607,#21079,#4268,.T.);
#28469=EDGE_CURVE('',#21047,#22607,#4269,.T.);
#28470=EDGE_CURVE('',#21048,#22606,#4270,.T.);
#28471=EDGE_CURVE('',#21049,#22605,#4271,.T.);
#28472=EDGE_CURVE('',#21050,#22604,#4272,.T.);
#28473=EDGE_CURVE('',#21051,#22603,#4273,.T.);
#28474=EDGE_CURVE('',#21052,#22602,#4274,.T.);
#28475=EDGE_CURVE('',#21053,#22601,#4275,.T.);
#28476=EDGE_CURVE('',#21054,#22600,#4276,.T.);
#28477=EDGE_CURVE('',#21055,#22599,#4277,.T.);
#28478=EDGE_CURVE('',#21056,#22598,#4278,.T.);
#28479=EDGE_CURVE('',#21057,#22597,#4279,.T.);
#28480=EDGE_CURVE('',#21058,#22596,#4280,.T.);
#28481=EDGE_CURVE('',#21059,#22595,#4281,.T.);
#28482=EDGE_CURVE('',#22105,#22594,#19114,.T.);
#28483=EDGE_CURVE('',#22608,#21835,#4282,.T.);
#28484=EDGE_CURVE('',#21063,#22608,#4283,.T.);
#28485=EDGE_CURVE('',#22609,#22608,#1784,.T.);
#28486=EDGE_CURVE('',#21064,#22609,#4284,.T.);
#28487=EDGE_CURVE('',#22610,#22609,#1785,.T.);
#28488=EDGE_CURVE('',#21065,#22610,#4285,.T.);
#28489=EDGE_CURVE('',#22611,#22610,#1786,.T.);
#28490=EDGE_CURVE('',#21066,#22611,#4286,.T.);
#28491=EDGE_CURVE('',#22612,#22611,#1787,.T.);
#28492=EDGE_CURVE('',#21067,#22612,#4287,.T.);
#28493=EDGE_CURVE('',#22613,#22612,#1788,.T.);
#28494=EDGE_CURVE('',#21068,#22613,#4288,.T.);
#28495=EDGE_CURVE('',#22614,#22613,#4289,.T.);
#28496=EDGE_CURVE('',#21069,#22614,#4290,.T.);
#28497=EDGE_CURVE('',#22615,#22614,#1789,.T.);
#28498=EDGE_CURVE('',#21070,#22615,#4291,.T.);
#28499=EDGE_CURVE('',#22616,#22615,#1790,.T.);
#28500=EDGE_CURVE('',#21071,#22616,#4292,.T.);
#28501=EDGE_CURVE('',#22617,#22616,#1791,.T.);
#28502=EDGE_CURVE('',#21072,#22617,#4293,.T.);
#28503=EDGE_CURVE('',#22618,#22617,#1792,.T.);
#28504=EDGE_CURVE('',#21073,#22618,#4294,.T.);
#28505=EDGE_CURVE('',#22619,#22618,#1793,.T.);
#28506=EDGE_CURVE('',#21074,#22619,#4295,.T.);
#28507=EDGE_CURVE('',#21998,#22619,#4296,.T.);
#28508=EDGE_CURVE('',#22620,#21834,#19701,.T.);
#28509=EDGE_CURVE('',#22620,#22621,#1794,.T.);
#28510=EDGE_CURVE('',#22621,#22622,#4297,.T.);
#28511=EDGE_CURVE('',#22622,#22623,#1795,.T.);
#28512=EDGE_CURVE('',#22623,#22624,#1796,.T.);
#28513=EDGE_CURVE('',#22624,#22625,#1797,.T.);
#28514=EDGE_CURVE('',#22625,#22626,#1798,.T.);
#28515=EDGE_CURVE('',#22626,#22627,#1799,.T.);
#28516=EDGE_CURVE('',#22627,#22628,#4298,.T.);
#28517=EDGE_CURVE('',#22628,#22629,#1800,.T.);
#28518=EDGE_CURVE('',#22629,#22630,#1801,.T.);
#28519=EDGE_CURVE('',#22630,#22631,#1802,.T.);
#28520=EDGE_CURVE('',#22631,#22632,#1803,.T.);
#28521=EDGE_CURVE('',#22632,#22633,#1804,.T.);
#28522=EDGE_CURVE('',#22633,#21045,#4299,.T.);
#28523=EDGE_CURVE('',#21013,#22633,#4300,.T.);
#28524=EDGE_CURVE('',#21014,#22632,#4301,.T.);
#28525=EDGE_CURVE('',#21015,#22631,#4302,.T.);
#28526=EDGE_CURVE('',#21016,#22630,#4303,.T.);
#28527=EDGE_CURVE('',#21017,#22629,#4304,.T.);
#28528=EDGE_CURVE('',#21018,#22628,#4305,.T.);
#28529=EDGE_CURVE('',#21019,#22627,#4306,.T.);
#28530=EDGE_CURVE('',#21020,#22626,#4307,.T.);
#28531=EDGE_CURVE('',#21021,#22625,#4308,.T.);
#28532=EDGE_CURVE('',#21022,#22624,#4309,.T.);
#28533=EDGE_CURVE('',#21023,#22623,#4310,.T.);
#28534=EDGE_CURVE('',#21024,#22622,#4311,.T.);
#28535=EDGE_CURVE('',#21025,#22621,#4312,.T.);
#28536=EDGE_CURVE('',#22106,#22620,#19115,.T.);
#28537=EDGE_CURVE('',#22634,#21831,#4313,.T.);
#28538=EDGE_CURVE('',#21029,#22634,#4314,.T.);
#28539=EDGE_CURVE('',#22635,#22634,#1805,.T.);
#28540=EDGE_CURVE('',#21030,#22635,#4315,.T.);
#28541=EDGE_CURVE('',#22636,#22635,#1806,.T.);
#28542=EDGE_CURVE('',#21031,#22636,#4316,.T.);
#28543=EDGE_CURVE('',#22637,#22636,#1807,.T.);
#28544=EDGE_CURVE('',#21032,#22637,#4317,.T.);
#28545=EDGE_CURVE('',#22638,#22637,#1808,.T.);
#28546=EDGE_CURVE('',#21033,#22638,#4318,.T.);
#28547=EDGE_CURVE('',#22639,#22638,#1809,.T.);
#28548=EDGE_CURVE('',#21034,#22639,#4319,.T.);
#28549=EDGE_CURVE('',#22640,#22639,#4320,.T.);
#28550=EDGE_CURVE('',#21035,#22640,#4321,.T.);
#28551=EDGE_CURVE('',#22641,#22640,#1810,.T.);
#28552=EDGE_CURVE('',#21036,#22641,#4322,.T.);
#28553=EDGE_CURVE('',#22642,#22641,#1811,.T.);
#28554=EDGE_CURVE('',#21037,#22642,#4323,.T.);
#28555=EDGE_CURVE('',#22643,#22642,#1812,.T.);
#28556=EDGE_CURVE('',#21038,#22643,#4324,.T.);
#28557=EDGE_CURVE('',#22644,#22643,#1813,.T.);
#28558=EDGE_CURVE('',#21039,#22644,#4325,.T.);
#28559=EDGE_CURVE('',#22645,#22644,#1814,.T.);
#28560=EDGE_CURVE('',#21040,#22645,#4326,.T.);
#28561=EDGE_CURVE('',#22001,#22645,#4327,.T.);
#28562=EDGE_CURVE('',#22646,#21830,#19702,.T.);
#28563=EDGE_CURVE('',#22646,#22647,#1815,.T.);
#28564=EDGE_CURVE('',#22647,#22648,#4328,.T.);
#28565=EDGE_CURVE('',#22648,#22649,#1816,.T.);
#28566=EDGE_CURVE('',#22649,#22650,#1817,.T.);
#28567=EDGE_CURVE('',#22650,#22651,#1818,.T.);
#28568=EDGE_CURVE('',#22651,#22652,#1819,.T.);
#28569=EDGE_CURVE('',#22652,#22653,#1820,.T.);
#28570=EDGE_CURVE('',#22653,#22654,#4329,.T.);
#28571=EDGE_CURVE('',#22654,#22655,#1821,.T.);
#28572=EDGE_CURVE('',#22655,#22656,#1822,.T.);
#28573=EDGE_CURVE('',#22656,#22657,#1823,.T.);
#28574=EDGE_CURVE('',#22657,#22658,#1824,.T.);
#28575=EDGE_CURVE('',#22658,#22659,#1825,.T.);
#28576=EDGE_CURVE('',#22659,#21011,#4330,.T.);
#28577=EDGE_CURVE('',#20979,#22659,#4331,.T.);
#28578=EDGE_CURVE('',#20980,#22658,#4332,.T.);
#28579=EDGE_CURVE('',#20981,#22657,#4333,.T.);
#28580=EDGE_CURVE('',#20982,#22656,#4334,.T.);
#28581=EDGE_CURVE('',#20983,#22655,#4335,.T.);
#28582=EDGE_CURVE('',#20984,#22654,#4336,.T.);
#28583=EDGE_CURVE('',#20985,#22653,#4337,.T.);
#28584=EDGE_CURVE('',#20986,#22652,#4338,.T.);
#28585=EDGE_CURVE('',#20987,#22651,#4339,.T.);
#28586=EDGE_CURVE('',#20988,#22650,#4340,.T.);
#28587=EDGE_CURVE('',#20989,#22649,#4341,.T.);
#28588=EDGE_CURVE('',#20990,#22648,#4342,.T.);
#28589=EDGE_CURVE('',#20991,#22647,#4343,.T.);
#28590=EDGE_CURVE('',#22107,#22646,#19116,.T.);
#28591=EDGE_CURVE('',#22660,#21827,#4344,.T.);
#28592=EDGE_CURVE('',#20995,#22660,#4345,.T.);
#28593=EDGE_CURVE('',#22661,#22660,#1826,.T.);
#28594=EDGE_CURVE('',#20996,#22661,#4346,.T.);
#28595=EDGE_CURVE('',#22662,#22661,#1827,.T.);
#28596=EDGE_CURVE('',#20997,#22662,#4347,.T.);
#28597=EDGE_CURVE('',#22663,#22662,#1828,.T.);
#28598=EDGE_CURVE('',#20998,#22663,#4348,.T.);
#28599=EDGE_CURVE('',#22664,#22663,#1829,.T.);
#28600=EDGE_CURVE('',#20999,#22664,#4349,.T.);
#28601=EDGE_CURVE('',#22665,#22664,#1830,.T.);
#28602=EDGE_CURVE('',#21000,#22665,#4350,.T.);
#28603=EDGE_CURVE('',#22666,#22665,#4351,.T.);
#28604=EDGE_CURVE('',#21001,#22666,#4352,.T.);
#28605=EDGE_CURVE('',#22667,#22666,#1831,.T.);
#28606=EDGE_CURVE('',#21002,#22667,#4353,.T.);
#28607=EDGE_CURVE('',#22668,#22667,#1832,.T.);
#28608=EDGE_CURVE('',#21003,#22668,#4354,.T.);
#28609=EDGE_CURVE('',#22669,#22668,#1833,.T.);
#28610=EDGE_CURVE('',#21004,#22669,#4355,.T.);
#28611=EDGE_CURVE('',#22670,#22669,#1834,.T.);
#28612=EDGE_CURVE('',#21005,#22670,#4356,.T.);
#28613=EDGE_CURVE('',#22671,#22670,#1835,.T.);
#28614=EDGE_CURVE('',#21006,#22671,#4357,.T.);
#28615=EDGE_CURVE('',#22004,#22671,#4358,.T.);
#28616=EDGE_CURVE('',#22672,#21826,#19703,.T.);
#28617=EDGE_CURVE('',#22672,#22673,#1836,.T.);
#28618=EDGE_CURVE('',#22673,#22674,#4359,.T.);
#28619=EDGE_CURVE('',#22674,#22675,#1837,.T.);
#28620=EDGE_CURVE('',#22675,#22676,#1838,.T.);
#28621=EDGE_CURVE('',#22676,#22677,#1839,.T.);
#28622=EDGE_CURVE('',#22677,#22678,#1840,.T.);
#28623=EDGE_CURVE('',#22678,#22679,#1841,.T.);
#28624=EDGE_CURVE('',#22679,#22680,#4360,.T.);
#28625=EDGE_CURVE('',#22680,#22681,#1842,.T.);
#28626=EDGE_CURVE('',#22681,#22682,#1843,.T.);
#28627=EDGE_CURVE('',#22682,#22683,#1844,.T.);
#28628=EDGE_CURVE('',#22683,#22684,#1845,.T.);
#28629=EDGE_CURVE('',#22684,#22685,#1846,.T.);
#28630=EDGE_CURVE('',#22685,#20977,#4361,.T.);
#28631=EDGE_CURVE('',#20945,#22685,#4362,.T.);
#28632=EDGE_CURVE('',#20946,#22684,#4363,.T.);
#28633=EDGE_CURVE('',#20947,#22683,#4364,.T.);
#28634=EDGE_CURVE('',#20948,#22682,#4365,.T.);
#28635=EDGE_CURVE('',#20949,#22681,#4366,.T.);
#28636=EDGE_CURVE('',#20950,#22680,#4367,.T.);
#28637=EDGE_CURVE('',#20951,#22679,#4368,.T.);
#28638=EDGE_CURVE('',#20952,#22678,#4369,.T.);
#28639=EDGE_CURVE('',#20953,#22677,#4370,.T.);
#28640=EDGE_CURVE('',#20954,#22676,#4371,.T.);
#28641=EDGE_CURVE('',#20955,#22675,#4372,.T.);
#28642=EDGE_CURVE('',#20956,#22674,#4373,.T.);
#28643=EDGE_CURVE('',#20957,#22673,#4374,.T.);
#28644=EDGE_CURVE('',#22108,#22672,#19117,.T.);
#28645=EDGE_CURVE('',#22686,#21823,#4375,.T.);
#28646=EDGE_CURVE('',#20961,#22686,#4376,.T.);
#28647=EDGE_CURVE('',#22687,#22686,#1847,.T.);
#28648=EDGE_CURVE('',#20962,#22687,#4377,.T.);
#28649=EDGE_CURVE('',#22688,#22687,#1848,.T.);
#28650=EDGE_CURVE('',#20963,#22688,#4378,.T.);
#28651=EDGE_CURVE('',#22689,#22688,#1849,.T.);
#28652=EDGE_CURVE('',#20964,#22689,#4379,.T.);
#28653=EDGE_CURVE('',#22690,#22689,#1850,.T.);
#28654=EDGE_CURVE('',#20965,#22690,#4380,.T.);
#28655=EDGE_CURVE('',#22691,#22690,#1851,.T.);
#28656=EDGE_CURVE('',#20966,#22691,#4381,.T.);
#28657=EDGE_CURVE('',#22692,#22691,#4382,.T.);
#28658=EDGE_CURVE('',#20967,#22692,#4383,.T.);
#28659=EDGE_CURVE('',#22693,#22692,#1852,.T.);
#28660=EDGE_CURVE('',#20968,#22693,#4384,.T.);
#28661=EDGE_CURVE('',#22694,#22693,#1853,.T.);
#28662=EDGE_CURVE('',#20969,#22694,#4385,.T.);
#28663=EDGE_CURVE('',#22695,#22694,#1854,.T.);
#28664=EDGE_CURVE('',#20970,#22695,#4386,.T.);
#28665=EDGE_CURVE('',#22696,#22695,#1855,.T.);
#28666=EDGE_CURVE('',#20971,#22696,#4387,.T.);
#28667=EDGE_CURVE('',#22697,#22696,#1856,.T.);
#28668=EDGE_CURVE('',#20972,#22697,#4388,.T.);
#28669=EDGE_CURVE('',#22007,#22697,#4389,.T.);
#28670=EDGE_CURVE('',#22698,#21822,#19704,.T.);
#28671=EDGE_CURVE('',#22698,#22699,#1857,.T.);
#28672=EDGE_CURVE('',#22699,#22700,#4390,.T.);
#28673=EDGE_CURVE('',#22700,#22701,#1858,.T.);
#28674=EDGE_CURVE('',#22701,#22702,#1859,.T.);
#28675=EDGE_CURVE('',#22702,#22703,#1860,.T.);
#28676=EDGE_CURVE('',#22703,#22704,#1861,.T.);
#28677=EDGE_CURVE('',#22704,#22705,#1862,.T.);
#28678=EDGE_CURVE('',#22705,#22706,#4391,.T.);
#28679=EDGE_CURVE('',#22706,#22707,#1863,.T.);
#28680=EDGE_CURVE('',#22707,#22708,#1864,.T.);
#28681=EDGE_CURVE('',#22708,#22709,#1865,.T.);
#28682=EDGE_CURVE('',#22709,#22710,#1866,.T.);
#28683=EDGE_CURVE('',#22710,#22711,#1867,.T.);
#28684=EDGE_CURVE('',#22711,#20943,#4392,.T.);
#28685=EDGE_CURVE('',#20911,#22711,#4393,.T.);
#28686=EDGE_CURVE('',#20912,#22710,#4394,.T.);
#28687=EDGE_CURVE('',#20913,#22709,#4395,.T.);
#28688=EDGE_CURVE('',#20914,#22708,#4396,.T.);
#28689=EDGE_CURVE('',#20915,#22707,#4397,.T.);
#28690=EDGE_CURVE('',#20916,#22706,#4398,.T.);
#28691=EDGE_CURVE('',#20917,#22705,#4399,.T.);
#28692=EDGE_CURVE('',#20918,#22704,#4400,.T.);
#28693=EDGE_CURVE('',#20919,#22703,#4401,.T.);
#28694=EDGE_CURVE('',#20920,#22702,#4402,.T.);
#28695=EDGE_CURVE('',#20921,#22701,#4403,.T.);
#28696=EDGE_CURVE('',#20922,#22700,#4404,.T.);
#28697=EDGE_CURVE('',#20923,#22699,#4405,.T.);
#28698=EDGE_CURVE('',#22109,#22698,#19118,.T.);
#28699=EDGE_CURVE('',#22712,#21819,#4406,.T.);
#28700=EDGE_CURVE('',#20927,#22712,#4407,.T.);
#28701=EDGE_CURVE('',#22713,#22712,#1868,.T.);
#28702=EDGE_CURVE('',#20928,#22713,#4408,.T.);
#28703=EDGE_CURVE('',#22714,#22713,#1869,.T.);
#28704=EDGE_CURVE('',#20929,#22714,#4409,.T.);
#28705=EDGE_CURVE('',#22715,#22714,#1870,.T.);
#28706=EDGE_CURVE('',#20930,#22715,#4410,.T.);
#28707=EDGE_CURVE('',#22716,#22715,#1871,.T.);
#28708=EDGE_CURVE('',#20931,#22716,#4411,.T.);
#28709=EDGE_CURVE('',#22717,#22716,#1872,.T.);
#28710=EDGE_CURVE('',#20932,#22717,#4412,.T.);
#28711=EDGE_CURVE('',#22718,#22717,#4413,.T.);
#28712=EDGE_CURVE('',#20933,#22718,#4414,.T.);
#28713=EDGE_CURVE('',#22719,#22718,#1873,.T.);
#28714=EDGE_CURVE('',#20934,#22719,#4415,.T.);
#28715=EDGE_CURVE('',#22720,#22719,#1874,.T.);
#28716=EDGE_CURVE('',#20935,#22720,#4416,.T.);
#28717=EDGE_CURVE('',#22721,#22720,#1875,.T.);
#28718=EDGE_CURVE('',#20936,#22721,#4417,.T.);
#28719=EDGE_CURVE('',#22722,#22721,#1876,.T.);
#28720=EDGE_CURVE('',#20937,#22722,#4418,.T.);
#28721=EDGE_CURVE('',#22723,#22722,#1877,.T.);
#28722=EDGE_CURVE('',#20938,#22723,#4419,.T.);
#28723=EDGE_CURVE('',#22010,#22723,#4420,.T.);
#28724=EDGE_CURVE('',#22724,#21818,#19705,.T.);
#28725=EDGE_CURVE('',#22724,#22725,#1878,.T.);
#28726=EDGE_CURVE('',#22725,#22726,#4421,.T.);
#28727=EDGE_CURVE('',#22726,#22727,#1879,.T.);
#28728=EDGE_CURVE('',#22727,#22728,#1880,.T.);
#28729=EDGE_CURVE('',#22728,#22729,#1881,.T.);
#28730=EDGE_CURVE('',#22729,#22730,#1882,.T.);
#28731=EDGE_CURVE('',#22730,#22731,#1883,.T.);
#28732=EDGE_CURVE('',#22731,#22732,#4422,.T.);
#28733=EDGE_CURVE('',#22732,#22733,#1884,.T.);
#28734=EDGE_CURVE('',#22733,#22734,#1885,.T.);
#28735=EDGE_CURVE('',#22734,#22735,#1886,.T.);
#28736=EDGE_CURVE('',#22735,#22736,#1887,.T.);
#28737=EDGE_CURVE('',#22736,#22737,#1888,.T.);
#28738=EDGE_CURVE('',#22737,#20909,#4423,.T.);
#28739=EDGE_CURVE('',#20877,#22737,#4424,.T.);
#28740=EDGE_CURVE('',#20878,#22736,#4425,.T.);
#28741=EDGE_CURVE('',#20879,#22735,#4426,.T.);
#28742=EDGE_CURVE('',#20880,#22734,#4427,.T.);
#28743=EDGE_CURVE('',#20881,#22733,#4428,.T.);
#28744=EDGE_CURVE('',#20882,#22732,#4429,.T.);
#28745=EDGE_CURVE('',#20883,#22731,#4430,.T.);
#28746=EDGE_CURVE('',#20884,#22730,#4431,.T.);
#28747=EDGE_CURVE('',#20885,#22729,#4432,.T.);
#28748=EDGE_CURVE('',#20886,#22728,#4433,.T.);
#28749=EDGE_CURVE('',#20887,#22727,#4434,.T.);
#28750=EDGE_CURVE('',#20888,#22726,#4435,.T.);
#28751=EDGE_CURVE('',#20889,#22725,#4436,.T.);
#28752=EDGE_CURVE('',#22110,#22724,#19119,.T.);
#28753=EDGE_CURVE('',#22738,#21815,#4437,.T.);
#28754=EDGE_CURVE('',#20893,#22738,#4438,.T.);
#28755=EDGE_CURVE('',#22739,#22738,#1889,.T.);
#28756=EDGE_CURVE('',#20894,#22739,#4439,.T.);
#28757=EDGE_CURVE('',#22740,#22739,#1890,.T.);
#28758=EDGE_CURVE('',#20895,#22740,#4440,.T.);
#28759=EDGE_CURVE('',#22741,#22740,#1891,.T.);
#28760=EDGE_CURVE('',#20896,#22741,#4441,.T.);
#28761=EDGE_CURVE('',#22742,#22741,#1892,.T.);
#28762=EDGE_CURVE('',#20897,#22742,#4442,.T.);
#28763=EDGE_CURVE('',#22743,#22742,#1893,.T.);
#28764=EDGE_CURVE('',#20898,#22743,#4443,.T.);
#28765=EDGE_CURVE('',#22744,#22743,#4444,.T.);
#28766=EDGE_CURVE('',#20899,#22744,#4445,.T.);
#28767=EDGE_CURVE('',#22745,#22744,#1894,.T.);
#28768=EDGE_CURVE('',#20900,#22745,#4446,.T.);
#28769=EDGE_CURVE('',#22746,#22745,#1895,.T.);
#28770=EDGE_CURVE('',#20901,#22746,#4447,.T.);
#28771=EDGE_CURVE('',#22747,#22746,#1896,.T.);
#28772=EDGE_CURVE('',#20902,#22747,#4448,.T.);
#28773=EDGE_CURVE('',#22748,#22747,#1897,.T.);
#28774=EDGE_CURVE('',#20903,#22748,#4449,.T.);
#28775=EDGE_CURVE('',#22749,#22748,#1898,.T.);
#28776=EDGE_CURVE('',#20904,#22749,#4450,.T.);
#28777=EDGE_CURVE('',#22013,#22749,#4451,.T.);
#28778=EDGE_CURVE('',#22750,#21814,#19706,.T.);
#28779=EDGE_CURVE('',#22750,#22751,#1899,.T.);
#28780=EDGE_CURVE('',#22751,#22752,#4452,.T.);
#28781=EDGE_CURVE('',#22752,#22753,#1900,.T.);
#28782=EDGE_CURVE('',#22753,#22754,#1901,.T.);
#28783=EDGE_CURVE('',#22754,#22755,#1902,.T.);
#28784=EDGE_CURVE('',#22755,#22756,#1903,.T.);
#28785=EDGE_CURVE('',#22756,#22757,#1904,.T.);
#28786=EDGE_CURVE('',#22757,#22758,#4453,.T.);
#28787=EDGE_CURVE('',#22758,#22759,#1905,.T.);
#28788=EDGE_CURVE('',#22759,#22760,#1906,.T.);
#28789=EDGE_CURVE('',#22760,#22761,#1907,.T.);
#28790=EDGE_CURVE('',#22761,#22762,#1908,.T.);
#28791=EDGE_CURVE('',#22762,#22763,#1909,.T.);
#28792=EDGE_CURVE('',#22763,#20875,#4454,.T.);
#28793=EDGE_CURVE('',#20843,#22763,#4455,.T.);
#28794=EDGE_CURVE('',#20844,#22762,#4456,.T.);
#28795=EDGE_CURVE('',#20845,#22761,#4457,.T.);
#28796=EDGE_CURVE('',#20846,#22760,#4458,.T.);
#28797=EDGE_CURVE('',#20847,#22759,#4459,.T.);
#28798=EDGE_CURVE('',#20848,#22758,#4460,.T.);
#28799=EDGE_CURVE('',#20849,#22757,#4461,.T.);
#28800=EDGE_CURVE('',#20850,#22756,#4462,.T.);
#28801=EDGE_CURVE('',#20851,#22755,#4463,.T.);
#28802=EDGE_CURVE('',#20852,#22754,#4464,.T.);
#28803=EDGE_CURVE('',#20853,#22753,#4465,.T.);
#28804=EDGE_CURVE('',#20854,#22752,#4466,.T.);
#28805=EDGE_CURVE('',#20855,#22751,#4467,.T.);
#28806=EDGE_CURVE('',#22111,#22750,#19120,.T.);
#28807=EDGE_CURVE('',#22764,#21811,#4468,.T.);
#28808=EDGE_CURVE('',#20859,#22764,#4469,.T.);
#28809=EDGE_CURVE('',#22765,#22764,#1910,.T.);
#28810=EDGE_CURVE('',#20860,#22765,#4470,.T.);
#28811=EDGE_CURVE('',#22766,#22765,#1911,.T.);
#28812=EDGE_CURVE('',#20861,#22766,#4471,.T.);
#28813=EDGE_CURVE('',#22767,#22766,#1912,.T.);
#28814=EDGE_CURVE('',#20862,#22767,#4472,.T.);
#28815=EDGE_CURVE('',#22768,#22767,#1913,.T.);
#28816=EDGE_CURVE('',#20863,#22768,#4473,.T.);
#28817=EDGE_CURVE('',#22769,#22768,#1914,.T.);
#28818=EDGE_CURVE('',#20864,#22769,#4474,.T.);
#28819=EDGE_CURVE('',#22770,#22769,#4475,.T.);
#28820=EDGE_CURVE('',#20865,#22770,#4476,.T.);
#28821=EDGE_CURVE('',#22771,#22770,#1915,.T.);
#28822=EDGE_CURVE('',#20866,#22771,#4477,.T.);
#28823=EDGE_CURVE('',#22772,#22771,#1916,.T.);
#28824=EDGE_CURVE('',#20867,#22772,#4478,.T.);
#28825=EDGE_CURVE('',#22773,#22772,#1917,.T.);
#28826=EDGE_CURVE('',#20868,#22773,#4479,.T.);
#28827=EDGE_CURVE('',#22774,#22773,#1918,.T.);
#28828=EDGE_CURVE('',#20869,#22774,#4480,.T.);
#28829=EDGE_CURVE('',#22775,#22774,#1919,.T.);
#28830=EDGE_CURVE('',#20870,#22775,#4481,.T.);
#28831=EDGE_CURVE('',#22016,#22775,#4482,.T.);
#28832=EDGE_CURVE('',#22776,#21810,#19707,.T.);
#28833=EDGE_CURVE('',#22776,#22777,#1920,.T.);
#28834=EDGE_CURVE('',#22777,#22778,#4483,.T.);
#28835=EDGE_CURVE('',#22778,#22779,#1921,.T.);
#28836=EDGE_CURVE('',#22779,#22780,#1922,.T.);
#28837=EDGE_CURVE('',#22780,#22781,#1923,.T.);
#28838=EDGE_CURVE('',#22781,#22782,#1924,.T.);
#28839=EDGE_CURVE('',#22782,#22783,#1925,.T.);
#28840=EDGE_CURVE('',#22783,#22784,#4484,.T.);
#28841=EDGE_CURVE('',#22784,#22785,#1926,.T.);
#28842=EDGE_CURVE('',#22785,#22786,#1927,.T.);
#28843=EDGE_CURVE('',#22786,#22787,#1928,.T.);
#28844=EDGE_CURVE('',#22787,#22788,#1929,.T.);
#28845=EDGE_CURVE('',#22788,#22789,#1930,.T.);
#28846=EDGE_CURVE('',#22789,#20841,#4485,.T.);
#28847=EDGE_CURVE('',#20809,#22789,#4486,.T.);
#28848=EDGE_CURVE('',#20810,#22788,#4487,.T.);
#28849=EDGE_CURVE('',#20811,#22787,#4488,.T.);
#28850=EDGE_CURVE('',#20812,#22786,#4489,.T.);
#28851=EDGE_CURVE('',#20813,#22785,#4490,.T.);
#28852=EDGE_CURVE('',#20814,#22784,#4491,.T.);
#28853=EDGE_CURVE('',#20815,#22783,#4492,.T.);
#28854=EDGE_CURVE('',#20816,#22782,#4493,.T.);
#28855=EDGE_CURVE('',#20817,#22781,#4494,.T.);
#28856=EDGE_CURVE('',#20818,#22780,#4495,.T.);
#28857=EDGE_CURVE('',#20819,#22779,#4496,.T.);
#28858=EDGE_CURVE('',#20820,#22778,#4497,.T.);
#28859=EDGE_CURVE('',#20821,#22777,#4498,.T.);
#28860=EDGE_CURVE('',#22112,#22776,#19121,.T.);
#28861=EDGE_CURVE('',#22790,#21807,#4499,.T.);
#28862=EDGE_CURVE('',#20825,#22790,#4500,.T.);
#28863=EDGE_CURVE('',#22791,#22790,#1931,.T.);
#28864=EDGE_CURVE('',#20826,#22791,#4501,.T.);
#28865=EDGE_CURVE('',#22792,#22791,#1932,.T.);
#28866=EDGE_CURVE('',#20827,#22792,#4502,.T.);
#28867=EDGE_CURVE('',#22793,#22792,#1933,.T.);
#28868=EDGE_CURVE('',#20828,#22793,#4503,.T.);
#28869=EDGE_CURVE('',#22794,#22793,#1934,.T.);
#28870=EDGE_CURVE('',#20829,#22794,#4504,.T.);
#28871=EDGE_CURVE('',#22795,#22794,#1935,.T.);
#28872=EDGE_CURVE('',#20830,#22795,#4505,.T.);
#28873=EDGE_CURVE('',#22796,#22795,#4506,.T.);
#28874=EDGE_CURVE('',#20831,#22796,#4507,.T.);
#28875=EDGE_CURVE('',#22797,#22796,#1936,.T.);
#28876=EDGE_CURVE('',#20832,#22797,#4508,.T.);
#28877=EDGE_CURVE('',#22798,#22797,#1937,.T.);
#28878=EDGE_CURVE('',#20833,#22798,#4509,.T.);
#28879=EDGE_CURVE('',#22799,#22798,#1938,.T.);
#28880=EDGE_CURVE('',#20834,#22799,#4510,.T.);
#28881=EDGE_CURVE('',#22800,#22799,#1939,.T.);
#28882=EDGE_CURVE('',#20835,#22800,#4511,.T.);
#28883=EDGE_CURVE('',#22801,#22800,#1940,.T.);
#28884=EDGE_CURVE('',#20836,#22801,#4512,.T.);
#28885=EDGE_CURVE('',#22019,#22801,#4513,.T.);
#28886=EDGE_CURVE('',#22802,#21806,#19708,.T.);
#28887=EDGE_CURVE('',#22802,#22803,#1941,.T.);
#28888=EDGE_CURVE('',#22803,#22804,#4514,.T.);
#28889=EDGE_CURVE('',#22804,#22805,#1942,.T.);
#28890=EDGE_CURVE('',#22805,#22806,#1943,.T.);
#28891=EDGE_CURVE('',#22806,#22807,#1944,.T.);
#28892=EDGE_CURVE('',#22807,#22808,#1945,.T.);
#28893=EDGE_CURVE('',#22808,#22809,#1946,.T.);
#28894=EDGE_CURVE('',#22809,#22810,#4515,.T.);
#28895=EDGE_CURVE('',#22810,#22811,#1947,.T.);
#28896=EDGE_CURVE('',#22811,#22812,#1948,.T.);
#28897=EDGE_CURVE('',#22812,#22813,#1949,.T.);
#28898=EDGE_CURVE('',#22813,#22814,#1950,.T.);
#28899=EDGE_CURVE('',#22814,#22815,#1951,.T.);
#28900=EDGE_CURVE('',#22815,#20807,#4516,.T.);
#28901=EDGE_CURVE('',#20775,#22815,#4517,.T.);
#28902=EDGE_CURVE('',#20776,#22814,#4518,.T.);
#28903=EDGE_CURVE('',#20777,#22813,#4519,.T.);
#28904=EDGE_CURVE('',#20778,#22812,#4520,.T.);
#28905=EDGE_CURVE('',#20779,#22811,#4521,.T.);
#28906=EDGE_CURVE('',#20780,#22810,#4522,.T.);
#28907=EDGE_CURVE('',#20781,#22809,#4523,.T.);
#28908=EDGE_CURVE('',#20782,#22808,#4524,.T.);
#28909=EDGE_CURVE('',#20783,#22807,#4525,.T.);
#28910=EDGE_CURVE('',#20784,#22806,#4526,.T.);
#28911=EDGE_CURVE('',#20785,#22805,#4527,.T.);
#28912=EDGE_CURVE('',#20786,#22804,#4528,.T.);
#28913=EDGE_CURVE('',#20787,#22803,#4529,.T.);
#28914=EDGE_CURVE('',#22113,#22802,#19122,.T.);
#28915=EDGE_CURVE('',#22816,#21803,#4530,.T.);
#28916=EDGE_CURVE('',#20791,#22816,#4531,.T.);
#28917=EDGE_CURVE('',#22817,#22816,#1952,.T.);
#28918=EDGE_CURVE('',#20792,#22817,#4532,.T.);
#28919=EDGE_CURVE('',#22818,#22817,#1953,.T.);
#28920=EDGE_CURVE('',#20793,#22818,#4533,.T.);
#28921=EDGE_CURVE('',#22819,#22818,#1954,.T.);
#28922=EDGE_CURVE('',#20794,#22819,#4534,.T.);
#28923=EDGE_CURVE('',#22820,#22819,#1955,.T.);
#28924=EDGE_CURVE('',#20795,#22820,#4535,.T.);
#28925=EDGE_CURVE('',#22821,#22820,#1956,.T.);
#28926=EDGE_CURVE('',#20796,#22821,#4536,.T.);
#28927=EDGE_CURVE('',#22822,#22821,#4537,.T.);
#28928=EDGE_CURVE('',#20797,#22822,#4538,.T.);
#28929=EDGE_CURVE('',#22823,#22822,#1957,.T.);
#28930=EDGE_CURVE('',#20798,#22823,#4539,.T.);
#28931=EDGE_CURVE('',#22824,#22823,#1958,.T.);
#28932=EDGE_CURVE('',#20799,#22824,#4540,.T.);
#28933=EDGE_CURVE('',#22825,#22824,#1959,.T.);
#28934=EDGE_CURVE('',#20800,#22825,#4541,.T.);
#28935=EDGE_CURVE('',#22826,#22825,#1960,.T.);
#28936=EDGE_CURVE('',#20801,#22826,#4542,.T.);
#28937=EDGE_CURVE('',#22827,#22826,#1961,.T.);
#28938=EDGE_CURVE('',#20802,#22827,#4543,.T.);
#28939=EDGE_CURVE('',#22022,#22827,#4544,.T.);
#28940=EDGE_CURVE('',#22828,#21802,#19709,.T.);
#28941=EDGE_CURVE('',#22828,#22829,#1962,.T.);
#28942=EDGE_CURVE('',#22829,#22830,#4545,.T.);
#28943=EDGE_CURVE('',#22830,#22831,#1963,.T.);
#28944=EDGE_CURVE('',#22831,#22832,#1964,.T.);
#28945=EDGE_CURVE('',#22832,#22833,#1965,.T.);
#28946=EDGE_CURVE('',#22833,#22834,#1966,.T.);
#28947=EDGE_CURVE('',#22834,#22835,#1967,.T.);
#28948=EDGE_CURVE('',#22835,#22836,#4546,.T.);
#28949=EDGE_CURVE('',#22836,#22837,#1968,.T.);
#28950=EDGE_CURVE('',#22837,#22838,#1969,.T.);
#28951=EDGE_CURVE('',#22838,#22839,#1970,.T.);
#28952=EDGE_CURVE('',#22839,#22840,#1971,.T.);
#28953=EDGE_CURVE('',#22840,#22841,#1972,.T.);
#28954=EDGE_CURVE('',#22841,#20773,#4547,.T.);
#28955=EDGE_CURVE('',#20741,#22841,#4548,.T.);
#28956=EDGE_CURVE('',#20742,#22840,#4549,.T.);
#28957=EDGE_CURVE('',#20743,#22839,#4550,.T.);
#28958=EDGE_CURVE('',#20744,#22838,#4551,.T.);
#28959=EDGE_CURVE('',#20745,#22837,#4552,.T.);
#28960=EDGE_CURVE('',#20746,#22836,#4553,.T.);
#28961=EDGE_CURVE('',#20747,#22835,#4554,.T.);
#28962=EDGE_CURVE('',#20748,#22834,#4555,.T.);
#28963=EDGE_CURVE('',#20749,#22833,#4556,.T.);
#28964=EDGE_CURVE('',#20750,#22832,#4557,.T.);
#28965=EDGE_CURVE('',#20751,#22831,#4558,.T.);
#28966=EDGE_CURVE('',#20752,#22830,#4559,.T.);
#28967=EDGE_CURVE('',#20753,#22829,#4560,.T.);
#28968=EDGE_CURVE('',#22114,#22828,#19123,.T.);
#28969=EDGE_CURVE('',#22842,#21799,#4561,.T.);
#28970=EDGE_CURVE('',#20757,#22842,#4562,.T.);
#28971=EDGE_CURVE('',#22843,#22842,#1973,.T.);
#28972=EDGE_CURVE('',#20758,#22843,#4563,.T.);
#28973=EDGE_CURVE('',#22844,#22843,#1974,.T.);
#28974=EDGE_CURVE('',#20759,#22844,#4564,.T.);
#28975=EDGE_CURVE('',#22845,#22844,#1975,.T.);
#28976=EDGE_CURVE('',#20760,#22845,#4565,.T.);
#28977=EDGE_CURVE('',#22846,#22845,#1976,.T.);
#28978=EDGE_CURVE('',#20761,#22846,#4566,.T.);
#28979=EDGE_CURVE('',#22847,#22846,#1977,.T.);
#28980=EDGE_CURVE('',#20762,#22847,#4567,.T.);
#28981=EDGE_CURVE('',#22848,#22847,#4568,.T.);
#28982=EDGE_CURVE('',#20763,#22848,#4569,.T.);
#28983=EDGE_CURVE('',#22849,#22848,#1978,.T.);
#28984=EDGE_CURVE('',#20764,#22849,#4570,.T.);
#28985=EDGE_CURVE('',#22850,#22849,#1979,.T.);
#28986=EDGE_CURVE('',#20765,#22850,#4571,.T.);
#28987=EDGE_CURVE('',#22851,#22850,#1980,.T.);
#28988=EDGE_CURVE('',#20766,#22851,#4572,.T.);
#28989=EDGE_CURVE('',#22852,#22851,#1981,.T.);
#28990=EDGE_CURVE('',#20767,#22852,#4573,.T.);
#28991=EDGE_CURVE('',#22853,#22852,#1982,.T.);
#28992=EDGE_CURVE('',#20768,#22853,#4574,.T.);
#28993=EDGE_CURVE('',#22025,#22853,#4575,.T.);
#28994=EDGE_CURVE('',#22854,#21798,#19710,.T.);
#28995=EDGE_CURVE('',#22854,#22855,#1983,.T.);
#28996=EDGE_CURVE('',#22855,#22856,#4576,.T.);
#28997=EDGE_CURVE('',#22856,#22857,#1984,.T.);
#28998=EDGE_CURVE('',#22857,#22858,#1985,.T.);
#28999=EDGE_CURVE('',#22858,#22859,#1986,.T.);
#29000=EDGE_CURVE('',#22859,#22860,#1987,.T.);
#29001=EDGE_CURVE('',#22860,#22861,#1988,.T.);
#29002=EDGE_CURVE('',#22861,#22862,#4577,.T.);
#29003=EDGE_CURVE('',#22862,#22863,#1989,.T.);
#29004=EDGE_CURVE('',#22863,#22864,#1990,.T.);
#29005=EDGE_CURVE('',#22864,#22865,#1991,.T.);
#29006=EDGE_CURVE('',#22865,#22866,#1992,.T.);
#29007=EDGE_CURVE('',#22866,#22867,#1993,.T.);
#29008=EDGE_CURVE('',#22867,#20739,#4578,.T.);
#29009=EDGE_CURVE('',#20707,#22867,#4579,.T.);
#29010=EDGE_CURVE('',#20708,#22866,#4580,.T.);
#29011=EDGE_CURVE('',#20709,#22865,#4581,.T.);
#29012=EDGE_CURVE('',#20710,#22864,#4582,.T.);
#29013=EDGE_CURVE('',#20711,#22863,#4583,.T.);
#29014=EDGE_CURVE('',#20712,#22862,#4584,.T.);
#29015=EDGE_CURVE('',#20713,#22861,#4585,.T.);
#29016=EDGE_CURVE('',#20714,#22860,#4586,.T.);
#29017=EDGE_CURVE('',#20715,#22859,#4587,.T.);
#29018=EDGE_CURVE('',#20716,#22858,#4588,.T.);
#29019=EDGE_CURVE('',#20717,#22857,#4589,.T.);
#29020=EDGE_CURVE('',#20718,#22856,#4590,.T.);
#29021=EDGE_CURVE('',#20719,#22855,#4591,.T.);
#29022=EDGE_CURVE('',#22115,#22854,#19124,.T.);
#29023=EDGE_CURVE('',#22868,#21795,#4592,.T.);
#29024=EDGE_CURVE('',#20723,#22868,#4593,.T.);
#29025=EDGE_CURVE('',#22869,#22868,#1994,.T.);
#29026=EDGE_CURVE('',#20724,#22869,#4594,.T.);
#29027=EDGE_CURVE('',#22870,#22869,#1995,.T.);
#29028=EDGE_CURVE('',#20725,#22870,#4595,.T.);
#29029=EDGE_CURVE('',#22871,#22870,#1996,.T.);
#29030=EDGE_CURVE('',#20726,#22871,#4596,.T.);
#29031=EDGE_CURVE('',#22872,#22871,#1997,.T.);
#29032=EDGE_CURVE('',#20727,#22872,#4597,.T.);
#29033=EDGE_CURVE('',#22873,#22872,#1998,.T.);
#29034=EDGE_CURVE('',#20728,#22873,#4598,.T.);
#29035=EDGE_CURVE('',#22874,#22873,#4599,.T.);
#29036=EDGE_CURVE('',#20729,#22874,#4600,.T.);
#29037=EDGE_CURVE('',#22875,#22874,#1999,.T.);
#29038=EDGE_CURVE('',#20730,#22875,#4601,.T.);
#29039=EDGE_CURVE('',#22876,#22875,#2000,.T.);
#29040=EDGE_CURVE('',#20731,#22876,#4602,.T.);
#29041=EDGE_CURVE('',#22877,#22876,#2001,.T.);
#29042=EDGE_CURVE('',#20732,#22877,#4603,.T.);
#29043=EDGE_CURVE('',#22878,#22877,#2002,.T.);
#29044=EDGE_CURVE('',#20733,#22878,#4604,.T.);
#29045=EDGE_CURVE('',#22879,#22878,#2003,.T.);
#29046=EDGE_CURVE('',#20734,#22879,#4605,.T.);
#29047=EDGE_CURVE('',#22028,#22879,#4606,.T.);
#29048=EDGE_CURVE('',#22880,#21794,#19711,.T.);
#29049=EDGE_CURVE('',#22880,#22881,#2004,.T.);
#29050=EDGE_CURVE('',#22881,#22882,#4607,.T.);
#29051=EDGE_CURVE('',#22882,#22883,#2005,.T.);
#29052=EDGE_CURVE('',#22883,#22884,#2006,.T.);
#29053=EDGE_CURVE('',#22884,#22885,#2007,.T.);
#29054=EDGE_CURVE('',#22885,#22886,#2008,.T.);
#29055=EDGE_CURVE('',#22886,#22887,#2009,.T.);
#29056=EDGE_CURVE('',#22887,#22888,#4608,.T.);
#29057=EDGE_CURVE('',#22888,#22889,#2010,.T.);
#29058=EDGE_CURVE('',#22889,#22890,#2011,.T.);
#29059=EDGE_CURVE('',#22890,#22891,#2012,.T.);
#29060=EDGE_CURVE('',#22891,#22892,#2013,.T.);
#29061=EDGE_CURVE('',#22892,#22893,#2014,.T.);
#29062=EDGE_CURVE('',#22893,#20705,#4609,.T.);
#29063=EDGE_CURVE('',#20673,#22893,#4610,.T.);
#29064=EDGE_CURVE('',#20674,#22892,#4611,.T.);
#29065=EDGE_CURVE('',#20675,#22891,#4612,.T.);
#29066=EDGE_CURVE('',#20676,#22890,#4613,.T.);
#29067=EDGE_CURVE('',#20677,#22889,#4614,.T.);
#29068=EDGE_CURVE('',#20678,#22888,#4615,.T.);
#29069=EDGE_CURVE('',#20679,#22887,#4616,.T.);
#29070=EDGE_CURVE('',#20680,#22886,#4617,.T.);
#29071=EDGE_CURVE('',#20681,#22885,#4618,.T.);
#29072=EDGE_CURVE('',#20682,#22884,#4619,.T.);
#29073=EDGE_CURVE('',#20683,#22883,#4620,.T.);
#29074=EDGE_CURVE('',#20684,#22882,#4621,.T.);
#29075=EDGE_CURVE('',#20685,#22881,#4622,.T.);
#29076=EDGE_CURVE('',#22116,#22880,#19125,.T.);
#29077=EDGE_CURVE('',#22894,#21791,#4623,.T.);
#29078=EDGE_CURVE('',#20689,#22894,#4624,.T.);
#29079=EDGE_CURVE('',#22895,#22894,#2015,.T.);
#29080=EDGE_CURVE('',#20690,#22895,#4625,.T.);
#29081=EDGE_CURVE('',#22896,#22895,#2016,.T.);
#29082=EDGE_CURVE('',#20691,#22896,#4626,.T.);
#29083=EDGE_CURVE('',#22897,#22896,#2017,.T.);
#29084=EDGE_CURVE('',#20692,#22897,#4627,.T.);
#29085=EDGE_CURVE('',#22898,#22897,#2018,.T.);
#29086=EDGE_CURVE('',#20693,#22898,#4628,.T.);
#29087=EDGE_CURVE('',#22899,#22898,#2019,.T.);
#29088=EDGE_CURVE('',#20694,#22899,#4629,.T.);
#29089=EDGE_CURVE('',#22900,#22899,#4630,.T.);
#29090=EDGE_CURVE('',#20695,#22900,#4631,.T.);
#29091=EDGE_CURVE('',#22901,#22900,#2020,.T.);
#29092=EDGE_CURVE('',#20696,#22901,#4632,.T.);
#29093=EDGE_CURVE('',#22902,#22901,#2021,.T.);
#29094=EDGE_CURVE('',#20697,#22902,#4633,.T.);
#29095=EDGE_CURVE('',#22903,#22902,#2022,.T.);
#29096=EDGE_CURVE('',#20698,#22903,#4634,.T.);
#29097=EDGE_CURVE('',#22904,#22903,#2023,.T.);
#29098=EDGE_CURVE('',#20699,#22904,#4635,.T.);
#29099=EDGE_CURVE('',#22905,#22904,#2024,.T.);
#29100=EDGE_CURVE('',#20700,#22905,#4636,.T.);
#29101=EDGE_CURVE('',#22031,#22905,#4637,.T.);
#29102=EDGE_CURVE('',#22906,#21790,#19712,.T.);
#29103=EDGE_CURVE('',#22906,#22907,#2025,.T.);
#29104=EDGE_CURVE('',#22907,#22908,#4638,.T.);
#29105=EDGE_CURVE('',#22908,#22909,#2026,.T.);
#29106=EDGE_CURVE('',#22909,#22910,#2027,.T.);
#29107=EDGE_CURVE('',#22910,#22911,#2028,.T.);
#29108=EDGE_CURVE('',#22911,#22912,#2029,.T.);
#29109=EDGE_CURVE('',#22912,#22913,#2030,.T.);
#29110=EDGE_CURVE('',#22913,#22914,#4639,.T.);
#29111=EDGE_CURVE('',#22914,#22915,#2031,.T.);
#29112=EDGE_CURVE('',#22915,#22916,#2032,.T.);
#29113=EDGE_CURVE('',#22916,#22917,#2033,.T.);
#29114=EDGE_CURVE('',#22917,#22918,#2034,.T.);
#29115=EDGE_CURVE('',#22918,#22919,#2035,.T.);
#29116=EDGE_CURVE('',#22919,#20671,#4640,.T.);
#29117=EDGE_CURVE('',#20639,#22919,#4641,.T.);
#29118=EDGE_CURVE('',#20640,#22918,#4642,.T.);
#29119=EDGE_CURVE('',#20641,#22917,#4643,.T.);
#29120=EDGE_CURVE('',#20642,#22916,#4644,.T.);
#29121=EDGE_CURVE('',#20643,#22915,#4645,.T.);
#29122=EDGE_CURVE('',#20644,#22914,#4646,.T.);
#29123=EDGE_CURVE('',#20645,#22913,#4647,.T.);
#29124=EDGE_CURVE('',#20646,#22912,#4648,.T.);
#29125=EDGE_CURVE('',#20647,#22911,#4649,.T.);
#29126=EDGE_CURVE('',#20648,#22910,#4650,.T.);
#29127=EDGE_CURVE('',#20649,#22909,#4651,.T.);
#29128=EDGE_CURVE('',#20650,#22908,#4652,.T.);
#29129=EDGE_CURVE('',#20651,#22907,#4653,.T.);
#29130=EDGE_CURVE('',#22117,#22906,#19126,.T.);
#29131=EDGE_CURVE('',#22920,#21787,#4654,.T.);
#29132=EDGE_CURVE('',#20655,#22920,#4655,.T.);
#29133=EDGE_CURVE('',#22921,#22920,#2036,.T.);
#29134=EDGE_CURVE('',#20656,#22921,#4656,.T.);
#29135=EDGE_CURVE('',#22922,#22921,#2037,.T.);
#29136=EDGE_CURVE('',#20657,#22922,#4657,.T.);
#29137=EDGE_CURVE('',#22923,#22922,#2038,.T.);
#29138=EDGE_CURVE('',#20658,#22923,#4658,.T.);
#29139=EDGE_CURVE('',#22924,#22923,#2039,.T.);
#29140=EDGE_CURVE('',#20659,#22924,#4659,.T.);
#29141=EDGE_CURVE('',#22925,#22924,#2040,.T.);
#29142=EDGE_CURVE('',#20660,#22925,#4660,.T.);
#29143=EDGE_CURVE('',#22926,#22925,#4661,.T.);
#29144=EDGE_CURVE('',#20661,#22926,#4662,.T.);
#29145=EDGE_CURVE('',#22927,#22926,#2041,.T.);
#29146=EDGE_CURVE('',#20662,#22927,#4663,.T.);
#29147=EDGE_CURVE('',#22928,#22927,#2042,.T.);
#29148=EDGE_CURVE('',#20663,#22928,#4664,.T.);
#29149=EDGE_CURVE('',#22929,#22928,#2043,.T.);
#29150=EDGE_CURVE('',#20664,#22929,#4665,.T.);
#29151=EDGE_CURVE('',#22930,#22929,#2044,.T.);
#29152=EDGE_CURVE('',#20665,#22930,#4666,.T.);
#29153=EDGE_CURVE('',#22931,#22930,#2045,.T.);
#29154=EDGE_CURVE('',#20666,#22931,#4667,.T.);
#29155=EDGE_CURVE('',#22034,#22931,#4668,.T.);
#29156=EDGE_CURVE('',#22932,#21786,#19713,.T.);
#29157=EDGE_CURVE('',#22932,#22933,#2046,.T.);
#29158=EDGE_CURVE('',#22933,#22934,#4669,.T.);
#29159=EDGE_CURVE('',#22934,#22935,#2047,.T.);
#29160=EDGE_CURVE('',#22935,#22936,#2048,.T.);
#29161=EDGE_CURVE('',#22936,#22937,#2049,.T.);
#29162=EDGE_CURVE('',#22937,#22938,#2050,.T.);
#29163=EDGE_CURVE('',#22938,#22939,#2051,.T.);
#29164=EDGE_CURVE('',#22939,#22940,#4670,.T.);
#29165=EDGE_CURVE('',#22940,#22941,#2052,.T.);
#29166=EDGE_CURVE('',#22941,#22942,#2053,.T.);
#29167=EDGE_CURVE('',#22942,#22943,#2054,.T.);
#29168=EDGE_CURVE('',#22943,#22944,#2055,.T.);
#29169=EDGE_CURVE('',#22944,#22945,#2056,.T.);
#29170=EDGE_CURVE('',#22945,#20637,#4671,.T.);
#29171=EDGE_CURVE('',#20605,#22945,#4672,.T.);
#29172=EDGE_CURVE('',#20606,#22944,#4673,.T.);
#29173=EDGE_CURVE('',#20607,#22943,#4674,.T.);
#29174=EDGE_CURVE('',#20608,#22942,#4675,.T.);
#29175=EDGE_CURVE('',#20609,#22941,#4676,.T.);
#29176=EDGE_CURVE('',#20610,#22940,#4677,.T.);
#29177=EDGE_CURVE('',#20611,#22939,#4678,.T.);
#29178=EDGE_CURVE('',#20612,#22938,#4679,.T.);
#29179=EDGE_CURVE('',#20613,#22937,#4680,.T.);
#29180=EDGE_CURVE('',#20614,#22936,#4681,.T.);
#29181=EDGE_CURVE('',#20615,#22935,#4682,.T.);
#29182=EDGE_CURVE('',#20616,#22934,#4683,.T.);
#29183=EDGE_CURVE('',#20617,#22933,#4684,.T.);
#29184=EDGE_CURVE('',#22118,#22932,#19127,.T.);
#29185=EDGE_CURVE('',#22946,#21783,#4685,.T.);
#29186=EDGE_CURVE('',#20621,#22946,#4686,.T.);
#29187=EDGE_CURVE('',#22947,#22946,#2057,.T.);
#29188=EDGE_CURVE('',#20622,#22947,#4687,.T.);
#29189=EDGE_CURVE('',#22948,#22947,#2058,.T.);
#29190=EDGE_CURVE('',#20623,#22948,#4688,.T.);
#29191=EDGE_CURVE('',#22949,#22948,#2059,.T.);
#29192=EDGE_CURVE('',#20624,#22949,#4689,.T.);
#29193=EDGE_CURVE('',#22950,#22949,#2060,.T.);
#29194=EDGE_CURVE('',#20625,#22950,#4690,.T.);
#29195=EDGE_CURVE('',#22951,#22950,#2061,.T.);
#29196=EDGE_CURVE('',#20626,#22951,#4691,.T.);
#29197=EDGE_CURVE('',#22952,#22951,#4692,.T.);
#29198=EDGE_CURVE('',#20627,#22952,#4693,.T.);
#29199=EDGE_CURVE('',#22953,#22952,#2062,.T.);
#29200=EDGE_CURVE('',#20628,#22953,#4694,.T.);
#29201=EDGE_CURVE('',#22954,#22953,#2063,.T.);
#29202=EDGE_CURVE('',#20629,#22954,#4695,.T.);
#29203=EDGE_CURVE('',#22955,#22954,#2064,.T.);
#29204=EDGE_CURVE('',#20630,#22955,#4696,.T.);
#29205=EDGE_CURVE('',#22956,#22955,#2065,.T.);
#29206=EDGE_CURVE('',#20631,#22956,#4697,.T.);
#29207=EDGE_CURVE('',#22957,#22956,#2066,.T.);
#29208=EDGE_CURVE('',#20632,#22957,#4698,.T.);
#29209=EDGE_CURVE('',#22037,#22957,#4699,.T.);
#29210=EDGE_CURVE('',#22958,#21782,#19714,.T.);
#29211=EDGE_CURVE('',#22958,#22959,#2067,.T.);
#29212=EDGE_CURVE('',#22959,#22960,#4700,.T.);
#29213=EDGE_CURVE('',#22960,#22961,#2068,.T.);
#29214=EDGE_CURVE('',#22961,#22962,#2069,.T.);
#29215=EDGE_CURVE('',#22962,#22963,#2070,.T.);
#29216=EDGE_CURVE('',#22963,#22964,#2071,.T.);
#29217=EDGE_CURVE('',#22964,#22965,#2072,.T.);
#29218=EDGE_CURVE('',#22965,#22966,#4701,.T.);
#29219=EDGE_CURVE('',#22966,#22967,#2073,.T.);
#29220=EDGE_CURVE('',#22967,#22968,#2074,.T.);
#29221=EDGE_CURVE('',#22968,#22969,#2075,.T.);
#29222=EDGE_CURVE('',#22969,#22970,#2076,.T.);
#29223=EDGE_CURVE('',#22970,#22971,#2077,.T.);
#29224=EDGE_CURVE('',#22971,#20603,#4702,.T.);
#29225=EDGE_CURVE('',#20571,#22971,#4703,.T.);
#29226=EDGE_CURVE('',#20572,#22970,#4704,.T.);
#29227=EDGE_CURVE('',#20573,#22969,#4705,.T.);
#29228=EDGE_CURVE('',#20574,#22968,#4706,.T.);
#29229=EDGE_CURVE('',#20575,#22967,#4707,.T.);
#29230=EDGE_CURVE('',#20576,#22966,#4708,.T.);
#29231=EDGE_CURVE('',#20577,#22965,#4709,.T.);
#29232=EDGE_CURVE('',#20578,#22964,#4710,.T.);
#29233=EDGE_CURVE('',#20579,#22963,#4711,.T.);
#29234=EDGE_CURVE('',#20580,#22962,#4712,.T.);
#29235=EDGE_CURVE('',#20581,#22961,#4713,.T.);
#29236=EDGE_CURVE('',#20582,#22960,#4714,.T.);
#29237=EDGE_CURVE('',#20583,#22959,#4715,.T.);
#29238=EDGE_CURVE('',#22119,#22958,#19128,.T.);
#29239=EDGE_CURVE('',#22972,#21779,#4716,.T.);
#29240=EDGE_CURVE('',#20587,#22972,#4717,.T.);
#29241=EDGE_CURVE('',#22973,#22972,#2078,.T.);
#29242=EDGE_CURVE('',#20588,#22973,#4718,.T.);
#29243=EDGE_CURVE('',#22974,#22973,#2079,.T.);
#29244=EDGE_CURVE('',#20589,#22974,#4719,.T.);
#29245=EDGE_CURVE('',#22975,#22974,#2080,.T.);
#29246=EDGE_CURVE('',#20590,#22975,#4720,.T.);
#29247=EDGE_CURVE('',#22976,#22975,#2081,.T.);
#29248=EDGE_CURVE('',#20591,#22976,#4721,.T.);
#29249=EDGE_CURVE('',#22977,#22976,#2082,.T.);
#29250=EDGE_CURVE('',#20592,#22977,#4722,.T.);
#29251=EDGE_CURVE('',#22978,#22977,#4723,.T.);
#29252=EDGE_CURVE('',#20593,#22978,#4724,.T.);
#29253=EDGE_CURVE('',#22979,#22978,#2083,.T.);
#29254=EDGE_CURVE('',#20594,#22979,#4725,.T.);
#29255=EDGE_CURVE('',#22980,#22979,#2084,.T.);
#29256=EDGE_CURVE('',#20595,#22980,#4726,.T.);
#29257=EDGE_CURVE('',#22981,#22980,#2085,.T.);
#29258=EDGE_CURVE('',#20596,#22981,#4727,.T.);
#29259=EDGE_CURVE('',#22982,#22981,#2086,.T.);
#29260=EDGE_CURVE('',#20597,#22982,#4728,.T.);
#29261=EDGE_CURVE('',#22983,#22982,#2087,.T.);
#29262=EDGE_CURVE('',#20598,#22983,#4729,.T.);
#29263=EDGE_CURVE('',#22040,#22983,#4730,.T.);
#29264=EDGE_CURVE('',#22984,#21778,#19715,.T.);
#29265=EDGE_CURVE('',#22984,#22985,#2088,.T.);
#29266=EDGE_CURVE('',#22985,#22986,#4731,.T.);
#29267=EDGE_CURVE('',#22986,#22987,#2089,.T.);
#29268=EDGE_CURVE('',#22987,#22988,#2090,.T.);
#29269=EDGE_CURVE('',#22988,#22989,#2091,.T.);
#29270=EDGE_CURVE('',#22989,#22990,#2092,.T.);
#29271=EDGE_CURVE('',#22990,#22991,#2093,.T.);
#29272=EDGE_CURVE('',#22991,#22992,#4732,.T.);
#29273=EDGE_CURVE('',#22992,#22993,#2094,.T.);
#29274=EDGE_CURVE('',#22993,#22994,#2095,.T.);
#29275=EDGE_CURVE('',#22994,#22995,#2096,.T.);
#29276=EDGE_CURVE('',#22995,#22996,#2097,.T.);
#29277=EDGE_CURVE('',#22996,#22997,#2098,.T.);
#29278=EDGE_CURVE('',#22997,#20569,#4733,.T.);
#29279=EDGE_CURVE('',#20537,#22997,#4734,.T.);
#29280=EDGE_CURVE('',#20538,#22996,#4735,.T.);
#29281=EDGE_CURVE('',#20539,#22995,#4736,.T.);
#29282=EDGE_CURVE('',#20540,#22994,#4737,.T.);
#29283=EDGE_CURVE('',#20541,#22993,#4738,.T.);
#29284=EDGE_CURVE('',#20542,#22992,#4739,.T.);
#29285=EDGE_CURVE('',#20543,#22991,#4740,.T.);
#29286=EDGE_CURVE('',#20544,#22990,#4741,.T.);
#29287=EDGE_CURVE('',#20545,#22989,#4742,.T.);
#29288=EDGE_CURVE('',#20546,#22988,#4743,.T.);
#29289=EDGE_CURVE('',#20547,#22987,#4744,.T.);
#29290=EDGE_CURVE('',#20548,#22986,#4745,.T.);
#29291=EDGE_CURVE('',#20549,#22985,#4746,.T.);
#29292=EDGE_CURVE('',#22120,#22984,#19129,.T.);
#29293=EDGE_CURVE('',#22998,#21775,#4747,.T.);
#29294=EDGE_CURVE('',#20553,#22998,#4748,.T.);
#29295=EDGE_CURVE('',#22999,#22998,#2099,.T.);
#29296=EDGE_CURVE('',#20554,#22999,#4749,.T.);
#29297=EDGE_CURVE('',#23000,#22999,#2100,.T.);
#29298=EDGE_CURVE('',#20555,#23000,#4750,.T.);
#29299=EDGE_CURVE('',#23001,#23000,#2101,.T.);
#29300=EDGE_CURVE('',#20556,#23001,#4751,.T.);
#29301=EDGE_CURVE('',#23002,#23001,#2102,.T.);
#29302=EDGE_CURVE('',#20557,#23002,#4752,.T.);
#29303=EDGE_CURVE('',#23003,#23002,#2103,.T.);
#29304=EDGE_CURVE('',#20558,#23003,#4753,.T.);
#29305=EDGE_CURVE('',#23004,#23003,#4754,.T.);
#29306=EDGE_CURVE('',#20559,#23004,#4755,.T.);
#29307=EDGE_CURVE('',#23005,#23004,#2104,.T.);
#29308=EDGE_CURVE('',#20560,#23005,#4756,.T.);
#29309=EDGE_CURVE('',#23006,#23005,#2105,.T.);
#29310=EDGE_CURVE('',#20561,#23006,#4757,.T.);
#29311=EDGE_CURVE('',#23007,#23006,#2106,.T.);
#29312=EDGE_CURVE('',#20562,#23007,#4758,.T.);
#29313=EDGE_CURVE('',#23008,#23007,#2107,.T.);
#29314=EDGE_CURVE('',#20563,#23008,#4759,.T.);
#29315=EDGE_CURVE('',#23009,#23008,#2108,.T.);
#29316=EDGE_CURVE('',#20564,#23009,#4760,.T.);
#29317=EDGE_CURVE('',#22043,#23009,#4761,.T.);
#29318=EDGE_CURVE('',#23010,#21774,#19716,.T.);
#29319=EDGE_CURVE('',#23010,#23011,#2109,.T.);
#29320=EDGE_CURVE('',#23011,#23012,#4762,.T.);
#29321=EDGE_CURVE('',#23012,#23013,#2110,.T.);
#29322=EDGE_CURVE('',#23013,#23014,#2111,.T.);
#29323=EDGE_CURVE('',#23014,#23015,#2112,.T.);
#29324=EDGE_CURVE('',#23015,#23016,#2113,.T.);
#29325=EDGE_CURVE('',#23016,#23017,#2114,.T.);
#29326=EDGE_CURVE('',#23017,#23018,#4763,.T.);
#29327=EDGE_CURVE('',#23018,#23019,#2115,.T.);
#29328=EDGE_CURVE('',#23019,#23020,#2116,.T.);
#29329=EDGE_CURVE('',#23020,#23021,#2117,.T.);
#29330=EDGE_CURVE('',#23021,#23022,#2118,.T.);
#29331=EDGE_CURVE('',#23022,#23023,#2119,.T.);
#29332=EDGE_CURVE('',#23023,#20535,#4764,.T.);
#29333=EDGE_CURVE('',#20503,#23023,#4765,.T.);
#29334=EDGE_CURVE('',#20504,#23022,#4766,.T.);
#29335=EDGE_CURVE('',#20505,#23021,#4767,.T.);
#29336=EDGE_CURVE('',#20506,#23020,#4768,.T.);
#29337=EDGE_CURVE('',#20507,#23019,#4769,.T.);
#29338=EDGE_CURVE('',#20508,#23018,#4770,.T.);
#29339=EDGE_CURVE('',#20509,#23017,#4771,.T.);
#29340=EDGE_CURVE('',#20510,#23016,#4772,.T.);
#29341=EDGE_CURVE('',#20511,#23015,#4773,.T.);
#29342=EDGE_CURVE('',#20512,#23014,#4774,.T.);
#29343=EDGE_CURVE('',#20513,#23013,#4775,.T.);
#29344=EDGE_CURVE('',#20514,#23012,#4776,.T.);
#29345=EDGE_CURVE('',#20515,#23011,#4777,.T.);
#29346=EDGE_CURVE('',#22121,#23010,#19130,.T.);
#29347=EDGE_CURVE('',#23024,#21771,#4778,.T.);
#29348=EDGE_CURVE('',#20519,#23024,#4779,.T.);
#29349=EDGE_CURVE('',#23025,#23024,#2120,.T.);
#29350=EDGE_CURVE('',#20520,#23025,#4780,.T.);
#29351=EDGE_CURVE('',#23026,#23025,#2121,.T.);
#29352=EDGE_CURVE('',#20521,#23026,#4781,.T.);
#29353=EDGE_CURVE('',#23027,#23026,#2122,.T.);
#29354=EDGE_CURVE('',#20522,#23027,#4782,.T.);
#29355=EDGE_CURVE('',#23028,#23027,#2123,.T.);
#29356=EDGE_CURVE('',#20523,#23028,#4783,.T.);
#29357=EDGE_CURVE('',#23029,#23028,#2124,.T.);
#29358=EDGE_CURVE('',#20524,#23029,#4784,.T.);
#29359=EDGE_CURVE('',#23030,#23029,#4785,.T.);
#29360=EDGE_CURVE('',#20525,#23030,#4786,.T.);
#29361=EDGE_CURVE('',#23031,#23030,#2125,.T.);
#29362=EDGE_CURVE('',#20526,#23031,#4787,.T.);
#29363=EDGE_CURVE('',#23032,#23031,#2126,.T.);
#29364=EDGE_CURVE('',#20527,#23032,#4788,.T.);
#29365=EDGE_CURVE('',#23033,#23032,#2127,.T.);
#29366=EDGE_CURVE('',#20528,#23033,#4789,.T.);
#29367=EDGE_CURVE('',#23034,#23033,#2128,.T.);
#29368=EDGE_CURVE('',#20529,#23034,#4790,.T.);
#29369=EDGE_CURVE('',#23035,#23034,#2129,.T.);
#29370=EDGE_CURVE('',#20530,#23035,#4791,.T.);
#29371=EDGE_CURVE('',#22046,#23035,#4792,.T.);
#29372=EDGE_CURVE('',#23036,#21770,#19717,.T.);
#29373=EDGE_CURVE('',#23036,#23037,#2130,.T.);
#29374=EDGE_CURVE('',#23037,#23038,#4793,.T.);
#29375=EDGE_CURVE('',#23038,#23039,#2131,.T.);
#29376=EDGE_CURVE('',#23039,#23040,#2132,.T.);
#29377=EDGE_CURVE('',#23040,#23041,#2133,.T.);
#29378=EDGE_CURVE('',#23041,#23042,#2134,.T.);
#29379=EDGE_CURVE('',#23042,#23043,#2135,.T.);
#29380=EDGE_CURVE('',#23043,#23044,#4794,.T.);
#29381=EDGE_CURVE('',#23044,#23045,#2136,.T.);
#29382=EDGE_CURVE('',#23045,#23046,#2137,.T.);
#29383=EDGE_CURVE('',#23046,#23047,#2138,.T.);
#29384=EDGE_CURVE('',#23047,#23048,#2139,.T.);
#29385=EDGE_CURVE('',#23048,#23049,#2140,.T.);
#29386=EDGE_CURVE('',#23049,#20501,#4795,.T.);
#29387=EDGE_CURVE('',#23050,#21767,#4796,.T.);
#29388=EDGE_CURVE('',#20485,#23050,#4797,.T.);
#29389=EDGE_CURVE('',#23051,#23050,#2141,.T.);
#29390=EDGE_CURVE('',#20486,#23051,#4798,.T.);
#29391=EDGE_CURVE('',#23052,#23051,#2142,.T.);
#29392=EDGE_CURVE('',#20487,#23052,#4799,.T.);
#29393=EDGE_CURVE('',#23053,#23052,#2143,.T.);
#29394=EDGE_CURVE('',#20488,#23053,#4800,.T.);
#29395=EDGE_CURVE('',#23054,#23053,#2144,.T.);
#29396=EDGE_CURVE('',#20489,#23054,#4801,.T.);
#29397=EDGE_CURVE('',#23055,#23054,#2145,.T.);
#29398=EDGE_CURVE('',#20490,#23055,#4802,.T.);
#29399=EDGE_CURVE('',#23056,#23055,#4803,.T.);
#29400=EDGE_CURVE('',#20491,#23056,#4804,.T.);
#29401=EDGE_CURVE('',#23057,#23056,#2146,.T.);
#29402=EDGE_CURVE('',#20492,#23057,#4805,.T.);
#29403=EDGE_CURVE('',#23058,#23057,#2147,.T.);
#29404=EDGE_CURVE('',#20493,#23058,#4806,.T.);
#29405=EDGE_CURVE('',#23059,#23058,#2148,.T.);
#29406=EDGE_CURVE('',#20494,#23059,#4807,.T.);
#29407=EDGE_CURVE('',#23060,#23059,#2149,.T.);
#29408=EDGE_CURVE('',#20495,#23060,#4808,.T.);
#29409=EDGE_CURVE('',#23061,#23060,#2150,.T.);
#29410=EDGE_CURVE('',#20496,#23061,#4809,.T.);
#29411=EDGE_CURVE('',#23062,#23061,#4810,.T.);
#29412=EDGE_CURVE('',#20497,#23062,#4811,.T.);
#29413=EDGE_CURVE('',#22151,#23062,#2151,.T.);
#29414=EDGE_CURVE('',#20469,#23049,#4812,.T.);
#29415=EDGE_CURVE('',#20470,#23048,#4813,.T.);
#29416=EDGE_CURVE('',#20471,#23047,#4814,.T.);
#29417=EDGE_CURVE('',#20472,#23046,#4815,.T.);
#29418=EDGE_CURVE('',#20473,#23045,#4816,.T.);
#29419=EDGE_CURVE('',#20474,#23044,#4817,.T.);
#29420=EDGE_CURVE('',#20475,#23043,#4818,.T.);
#29421=EDGE_CURVE('',#20476,#23042,#4819,.T.);
#29422=EDGE_CURVE('',#20477,#23041,#4820,.T.);
#29423=EDGE_CURVE('',#20478,#23040,#4821,.T.);
#29424=EDGE_CURVE('',#20479,#23039,#4822,.T.);
#29425=EDGE_CURVE('',#20480,#23038,#4823,.T.);
#29426=EDGE_CURVE('',#20481,#23037,#4824,.T.);
#29427=EDGE_CURVE('',#22122,#23036,#19131,.T.);
#29428=EDGE_CURVE('',#22136,#21766,#19718,.T.);
#29429=EDGE_CURVE('',#22104,#23063,#4825,.T.);
#29430=EDGE_CURVE('',#23063,#23063,#19719,.T.);
#29431=EDGE_CURVE('',#23064,#23064,#19720,.T.);
#29432=EDGE_CURVE('',#23064,#23065,#4826,.T.);
#29433=EDGE_CURVE('',#23065,#23066,#19721,.T.);
#29434=EDGE_CURVE('',#23066,#23065,#19722,.T.);
#29435=EDGE_CURVE('',#23066,#23067,#4827,.T.);
#29436=EDGE_CURVE('',#23068,#23067,#19723,.T.);
#29437=EDGE_CURVE('',#23067,#23068,#19724,.T.);
#29438=EDGE_CURVE('',#23068,#23069,#19725,.T.);
#29439=EDGE_CURVE('',#23069,#23070,#19726,.T.);
#29440=EDGE_CURVE('',#23070,#23069,#19727,.T.);
#29441=EDGE_CURVE('',#23070,#23071,#4828,.T.);
#29442=EDGE_CURVE('',#23071,#23071,#19728,.T.);
#29443=EDGE_CURVE('',#23072,#23073,#19729,.T.);
#29444=EDGE_CURVE('',#23073,#23074,#19730,.T.);
#29445=EDGE_CURVE('',#23074,#23074,#19731,.T.);
#29446=EDGE_CURVE('',#23073,#23072,#19732,.T.);
#29447=EDGE_CURVE('',#23072,#23075,#4829,.T.);
#29448=EDGE_CURVE('',#23076,#23075,#19733,.T.);
#29449=EDGE_CURVE('',#23075,#23076,#19734,.T.);
#29450=EDGE_CURVE('',#23077,#23077,#19735,.T.);
#29451=EDGE_CURVE('',#23078,#23078,#19736,.T.);
#29452=EDGE_CURVE('',#23078,#23076,#19737,.T.);
#29453=EDGE_CURVE('',#23079,#23079,#19738,.T.);
#29454=EDGE_CURVE('',#23080,#23080,#19739,.T.);
#29455=EDGE_CURVE('',#23081,#23081,#19740,.T.);
#29456=EDGE_CURVE('',#23081,#23080,#4830,.T.);
#29457=EDGE_CURVE('',#23082,#23082,#19741,.T.);
#29458=EDGE_CURVE('',#23082,#23081,#4831,.T.);
#29459=EDGE_CURVE('',#23079,#23082,#4832,.T.);
#29460=EDGE_CURVE('',#23083,#23083,#19742,.T.);
#29461=EDGE_CURVE('',#23083,#23077,#4833,.T.);
#29462=EDGE_CURVE('',#23071,#23083,#4834,.T.);
#32919=ORIENTED_EDGE('',*,*,#25321,.F.);
#32920=ORIENTED_EDGE('',*,*,#25322,.F.);
#32921=ORIENTED_EDGE('',*,*,#25323,.F.);
#32922=ORIENTED_EDGE('',*,*,#25324,.F.);
#32923=ORIENTED_EDGE('',*,*,#25325,.F.);
#32924=ORIENTED_EDGE('',*,*,#25326,.F.);
#32925=ORIENTED_EDGE('',*,*,#25327,.F.);
#32926=ORIENTED_EDGE('',*,*,#25328,.F.);
#32927=ORIENTED_EDGE('',*,*,#25329,.F.);
#32928=ORIENTED_EDGE('',*,*,#25330,.F.);
#32929=ORIENTED_EDGE('',*,*,#25331,.F.);
#32930=ORIENTED_EDGE('',*,*,#25332,.F.);
#32931=ORIENTED_EDGE('',*,*,#25333,.F.);
#32932=ORIENTED_EDGE('',*,*,#25334,.F.);
#32933=ORIENTED_EDGE('',*,*,#25335,.F.);
#32934=ORIENTED_EDGE('',*,*,#25336,.F.);
#32935=ORIENTED_EDGE('',*,*,#25337,.F.);
#32936=ORIENTED_EDGE('',*,*,#25338,.F.);
#32937=ORIENTED_EDGE('',*,*,#25339,.F.);
#32938=ORIENTED_EDGE('',*,*,#25340,.F.);
#32939=ORIENTED_EDGE('',*,*,#25341,.F.);
#32940=ORIENTED_EDGE('',*,*,#25342,.F.);
#32941=ORIENTED_EDGE('',*,*,#25343,.F.);
#32942=ORIENTED_EDGE('',*,*,#25344,.F.);
#32943=ORIENTED_EDGE('',*,*,#25345,.F.);
#32944=ORIENTED_EDGE('',*,*,#25346,.F.);
#32945=ORIENTED_EDGE('',*,*,#25347,.F.);
#32946=ORIENTED_EDGE('',*,*,#25348,.F.);
#32947=ORIENTED_EDGE('',*,*,#25349,.F.);
#32948=ORIENTED_EDGE('',*,*,#25350,.F.);
#32949=ORIENTED_EDGE('',*,*,#25351,.F.);
#32950=ORIENTED_EDGE('',*,*,#25352,.F.);
#32951=ORIENTED_EDGE('',*,*,#25353,.F.);
#32952=ORIENTED_EDGE('',*,*,#25354,.F.);
#32953=ORIENTED_EDGE('',*,*,#25355,.F.);
#32954=ORIENTED_EDGE('',*,*,#25356,.F.);
#32955=ORIENTED_EDGE('',*,*,#25357,.F.);
#32956=ORIENTED_EDGE('',*,*,#25358,.F.);
#32957=ORIENTED_EDGE('',*,*,#25359,.F.);
#32958=ORIENTED_EDGE('',*,*,#25360,.F.);
#32959=ORIENTED_EDGE('',*,*,#25361,.F.);
#32960=ORIENTED_EDGE('',*,*,#25362,.F.);
#32961=ORIENTED_EDGE('',*,*,#25363,.F.);
#32962=ORIENTED_EDGE('',*,*,#25364,.F.);
#32963=ORIENTED_EDGE('',*,*,#25365,.F.);
#32964=ORIENTED_EDGE('',*,*,#25366,.F.);
#32965=ORIENTED_EDGE('',*,*,#25367,.F.);
#32966=ORIENTED_EDGE('',*,*,#25368,.F.);
#32967=ORIENTED_EDGE('',*,*,#25369,.F.);
#32968=ORIENTED_EDGE('',*,*,#25370,.F.);
#32969=ORIENTED_EDGE('',*,*,#25371,.F.);
#32970=ORIENTED_EDGE('',*,*,#25372,.F.);
#32971=ORIENTED_EDGE('',*,*,#25373,.F.);
#32972=ORIENTED_EDGE('',*,*,#25374,.F.);
#32973=ORIENTED_EDGE('',*,*,#25375,.F.);
#32974=ORIENTED_EDGE('',*,*,#25376,.F.);
#32975=ORIENTED_EDGE('',*,*,#25377,.F.);
#32976=ORIENTED_EDGE('',*,*,#25378,.F.);
#32977=ORIENTED_EDGE('',*,*,#25379,.F.);
#32978=ORIENTED_EDGE('',*,*,#25380,.F.);
#32979=ORIENTED_EDGE('',*,*,#25381,.F.);
#32980=ORIENTED_EDGE('',*,*,#25382,.F.);
#32981=ORIENTED_EDGE('',*,*,#25383,.F.);
#32982=ORIENTED_EDGE('',*,*,#25384,.F.);
#32983=ORIENTED_EDGE('',*,*,#25385,.F.);
#32984=ORIENTED_EDGE('',*,*,#25386,.F.);
#32985=ORIENTED_EDGE('',*,*,#25387,.F.);
#32986=ORIENTED_EDGE('',*,*,#25388,.F.);
#32987=ORIENTED_EDGE('',*,*,#25389,.F.);
#32988=ORIENTED_EDGE('',*,*,#25390,.F.);
#32989=ORIENTED_EDGE('',*,*,#25391,.F.);
#32990=ORIENTED_EDGE('',*,*,#25392,.F.);
#32991=ORIENTED_EDGE('',*,*,#25393,.F.);
#32992=ORIENTED_EDGE('',*,*,#25394,.F.);
#32993=ORIENTED_EDGE('',*,*,#25395,.F.);
#32994=ORIENTED_EDGE('',*,*,#25396,.F.);
#32995=ORIENTED_EDGE('',*,*,#25397,.F.);
#32996=ORIENTED_EDGE('',*,*,#25398,.F.);
#32997=ORIENTED_EDGE('',*,*,#25399,.F.);
#32998=ORIENTED_EDGE('',*,*,#25400,.F.);
#32999=ORIENTED_EDGE('',*,*,#25401,.F.);
#33000=ORIENTED_EDGE('',*,*,#25402,.F.);
#33001=ORIENTED_EDGE('',*,*,#25403,.F.);
#33002=ORIENTED_EDGE('',*,*,#25404,.F.);
#33003=ORIENTED_EDGE('',*,*,#25405,.F.);
#33004=ORIENTED_EDGE('',*,*,#25406,.F.);
#33005=ORIENTED_EDGE('',*,*,#25407,.F.);
#33006=ORIENTED_EDGE('',*,*,#25408,.F.);
#33007=ORIENTED_EDGE('',*,*,#25409,.F.);
#33008=ORIENTED_EDGE('',*,*,#25410,.F.);
#33009=ORIENTED_EDGE('',*,*,#25411,.F.);
#33010=ORIENTED_EDGE('',*,*,#25412,.F.);
#33011=ORIENTED_EDGE('',*,*,#25413,.F.);
#33012=ORIENTED_EDGE('',*,*,#25414,.F.);
#33013=ORIENTED_EDGE('',*,*,#25415,.F.);
#33014=ORIENTED_EDGE('',*,*,#25416,.F.);
#33015=ORIENTED_EDGE('',*,*,#25417,.F.);
#33016=ORIENTED_EDGE('',*,*,#25418,.F.);
#33017=ORIENTED_EDGE('',*,*,#25419,.F.);
#33018=ORIENTED_EDGE('',*,*,#25420,.F.);
#33019=ORIENTED_EDGE('',*,*,#25421,.F.);
#33020=ORIENTED_EDGE('',*,*,#25422,.F.);
#33021=ORIENTED_EDGE('',*,*,#25423,.F.);
#33022=ORIENTED_EDGE('',*,*,#25424,.F.);
#33023=ORIENTED_EDGE('',*,*,#25425,.F.);
#33024=ORIENTED_EDGE('',*,*,#25426,.F.);
#33025=ORIENTED_EDGE('',*,*,#25427,.F.);
#33026=ORIENTED_EDGE('',*,*,#25428,.F.);
#33027=ORIENTED_EDGE('',*,*,#25429,.F.);
#33028=ORIENTED_EDGE('',*,*,#25430,.F.);
#33029=ORIENTED_EDGE('',*,*,#25431,.F.);
#33030=ORIENTED_EDGE('',*,*,#25432,.F.);
#33031=ORIENTED_EDGE('',*,*,#25433,.F.);
#33032=ORIENTED_EDGE('',*,*,#25434,.F.);
#33033=ORIENTED_EDGE('',*,*,#25435,.F.);
#33034=ORIENTED_EDGE('',*,*,#25436,.F.);
#33035=ORIENTED_EDGE('',*,*,#25437,.F.);
#33036=ORIENTED_EDGE('',*,*,#25438,.F.);
#33037=ORIENTED_EDGE('',*,*,#25439,.F.);
#33038=ORIENTED_EDGE('',*,*,#25440,.F.);
#33039=ORIENTED_EDGE('',*,*,#25441,.F.);
#33040=ORIENTED_EDGE('',*,*,#25442,.F.);
#33041=ORIENTED_EDGE('',*,*,#25443,.F.);
#33042=ORIENTED_EDGE('',*,*,#25444,.F.);
#33043=ORIENTED_EDGE('',*,*,#25445,.F.);
#33044=ORIENTED_EDGE('',*,*,#25446,.F.);
#33045=ORIENTED_EDGE('',*,*,#25447,.F.);
#33046=ORIENTED_EDGE('',*,*,#25448,.F.);
#33047=ORIENTED_EDGE('',*,*,#25449,.F.);
#33048=ORIENTED_EDGE('',*,*,#25450,.F.);
#33049=ORIENTED_EDGE('',*,*,#25451,.F.);
#33050=ORIENTED_EDGE('',*,*,#25452,.F.);
#33051=ORIENTED_EDGE('',*,*,#25453,.F.);
#33052=ORIENTED_EDGE('',*,*,#25454,.F.);
#33053=ORIENTED_EDGE('',*,*,#25455,.F.);
#33054=ORIENTED_EDGE('',*,*,#25456,.F.);
#33055=ORIENTED_EDGE('',*,*,#25457,.F.);
#33056=ORIENTED_EDGE('',*,*,#25458,.F.);
#33057=ORIENTED_EDGE('',*,*,#25459,.F.);
#33058=ORIENTED_EDGE('',*,*,#25460,.F.);
#33059=ORIENTED_EDGE('',*,*,#25461,.F.);
#33060=ORIENTED_EDGE('',*,*,#25462,.F.);
#33061=ORIENTED_EDGE('',*,*,#25463,.F.);
#33062=ORIENTED_EDGE('',*,*,#25464,.F.);
#33063=ORIENTED_EDGE('',*,*,#25463,.T.);
#33064=ORIENTED_EDGE('',*,*,#25465,.F.);
#33065=ORIENTED_EDGE('',*,*,#25466,.F.);
#33066=ORIENTED_EDGE('',*,*,#25467,.F.);
#33067=ORIENTED_EDGE('',*,*,#25468,.F.);
#33068=ORIENTED_EDGE('',*,*,#25469,.F.);
#33069=ORIENTED_EDGE('',*,*,#25470,.F.);
#33070=ORIENTED_EDGE('',*,*,#25471,.F.);
#33071=ORIENTED_EDGE('',*,*,#25472,.F.);
#33072=ORIENTED_EDGE('',*,*,#25473,.F.);
#33073=ORIENTED_EDGE('',*,*,#25474,.F.);
#33074=ORIENTED_EDGE('',*,*,#25475,.F.);
#33075=ORIENTED_EDGE('',*,*,#25476,.F.);
#33076=ORIENTED_EDGE('',*,*,#25477,.F.);
#33077=ORIENTED_EDGE('',*,*,#25478,.F.);
#33078=ORIENTED_EDGE('',*,*,#25479,.F.);
#33079=ORIENTED_EDGE('',*,*,#25480,.T.);
#33080=ORIENTED_EDGE('',*,*,#25481,.F.);
#33081=ORIENTED_EDGE('',*,*,#25482,.F.);
#33082=ORIENTED_EDGE('',*,*,#25483,.F.);
#33083=ORIENTED_EDGE('',*,*,#25484,.F.);
#33084=ORIENTED_EDGE('',*,*,#25485,.F.);
#33085=ORIENTED_EDGE('',*,*,#25486,.F.);
#33086=ORIENTED_EDGE('',*,*,#25487,.F.);
#33087=ORIENTED_EDGE('',*,*,#25488,.F.);
#33088=ORIENTED_EDGE('',*,*,#25489,.F.);
#33089=ORIENTED_EDGE('',*,*,#25490,.F.);
#33090=ORIENTED_EDGE('',*,*,#25491,.F.);
#33091=ORIENTED_EDGE('',*,*,#25492,.F.);
#33092=ORIENTED_EDGE('',*,*,#25493,.F.);
#33093=ORIENTED_EDGE('',*,*,#25494,.F.);
#33094=ORIENTED_EDGE('',*,*,#25495,.F.);
#33095=ORIENTED_EDGE('',*,*,#25462,.T.);
#33096=ORIENTED_EDGE('',*,*,#25496,.T.);
#33097=ORIENTED_EDGE('',*,*,#25497,.T.);
#33098=ORIENTED_EDGE('',*,*,#25498,.F.);
#33099=ORIENTED_EDGE('',*,*,#25499,.F.);
#33100=ORIENTED_EDGE('',*,*,#25500,.F.);
#33101=ORIENTED_EDGE('',*,*,#25465,.T.);
#33102=ORIENTED_EDGE('',*,*,#25459,.T.);
#33103=ORIENTED_EDGE('',*,*,#25501,.F.);
#33104=ORIENTED_EDGE('',*,*,#25502,.F.);
#33105=ORIENTED_EDGE('',*,*,#25503,.F.);
#33106=ORIENTED_EDGE('',*,*,#25504,.F.);
#33107=ORIENTED_EDGE('',*,*,#25505,.F.);
#33108=ORIENTED_EDGE('',*,*,#25506,.F.);
#33109=ORIENTED_EDGE('',*,*,#25507,.F.);
#33110=ORIENTED_EDGE('',*,*,#25508,.F.);
#33111=ORIENTED_EDGE('',*,*,#25509,.F.);
#33112=ORIENTED_EDGE('',*,*,#25510,.F.);
#33113=ORIENTED_EDGE('',*,*,#25511,.F.);
#33114=ORIENTED_EDGE('',*,*,#25512,.F.);
#33115=ORIENTED_EDGE('',*,*,#25513,.F.);
#33116=ORIENTED_EDGE('',*,*,#25514,.F.);
#33117=ORIENTED_EDGE('',*,*,#25515,.F.);
#33118=ORIENTED_EDGE('',*,*,#25516,.T.);
#33119=ORIENTED_EDGE('',*,*,#25517,.F.);
#33120=ORIENTED_EDGE('',*,*,#25518,.F.);
#33121=ORIENTED_EDGE('',*,*,#25519,.F.);
#33122=ORIENTED_EDGE('',*,*,#25520,.F.);
#33123=ORIENTED_EDGE('',*,*,#25521,.F.);
#33124=ORIENTED_EDGE('',*,*,#25522,.F.);
#33125=ORIENTED_EDGE('',*,*,#25523,.F.);
#33126=ORIENTED_EDGE('',*,*,#25524,.F.);
#33127=ORIENTED_EDGE('',*,*,#25525,.F.);
#33128=ORIENTED_EDGE('',*,*,#25526,.F.);
#33129=ORIENTED_EDGE('',*,*,#25527,.F.);
#33130=ORIENTED_EDGE('',*,*,#25528,.F.);
#33131=ORIENTED_EDGE('',*,*,#25529,.F.);
#33132=ORIENTED_EDGE('',*,*,#25530,.F.);
#33133=ORIENTED_EDGE('',*,*,#25531,.F.);
#33134=ORIENTED_EDGE('',*,*,#25458,.T.);
#33135=ORIENTED_EDGE('',*,*,#25532,.T.);
#33136=ORIENTED_EDGE('',*,*,#25533,.T.);
#33137=ORIENTED_EDGE('',*,*,#25534,.F.);
#33138=ORIENTED_EDGE('',*,*,#25535,.F.);
#33139=ORIENTED_EDGE('',*,*,#25536,.F.);
#33140=ORIENTED_EDGE('',*,*,#25501,.T.);
#33141=ORIENTED_EDGE('',*,*,#25455,.T.);
#33142=ORIENTED_EDGE('',*,*,#25537,.F.);
#33143=ORIENTED_EDGE('',*,*,#25538,.F.);
#33144=ORIENTED_EDGE('',*,*,#25539,.F.);
#33145=ORIENTED_EDGE('',*,*,#25540,.F.);
#33146=ORIENTED_EDGE('',*,*,#25541,.F.);
#33147=ORIENTED_EDGE('',*,*,#25542,.F.);
#33148=ORIENTED_EDGE('',*,*,#25543,.F.);
#33149=ORIENTED_EDGE('',*,*,#25544,.F.);
#33150=ORIENTED_EDGE('',*,*,#25545,.F.);
#33151=ORIENTED_EDGE('',*,*,#25546,.F.);
#33152=ORIENTED_EDGE('',*,*,#25547,.F.);
#33153=ORIENTED_EDGE('',*,*,#25548,.F.);
#33154=ORIENTED_EDGE('',*,*,#25549,.F.);
#33155=ORIENTED_EDGE('',*,*,#25550,.F.);
#33156=ORIENTED_EDGE('',*,*,#25551,.F.);
#33157=ORIENTED_EDGE('',*,*,#25552,.T.);
#33158=ORIENTED_EDGE('',*,*,#25553,.F.);
#33159=ORIENTED_EDGE('',*,*,#25554,.F.);
#33160=ORIENTED_EDGE('',*,*,#25555,.F.);
#33161=ORIENTED_EDGE('',*,*,#25556,.F.);
#33162=ORIENTED_EDGE('',*,*,#25557,.F.);
#33163=ORIENTED_EDGE('',*,*,#25558,.F.);
#33164=ORIENTED_EDGE('',*,*,#25559,.F.);
#33165=ORIENTED_EDGE('',*,*,#25560,.F.);
#33166=ORIENTED_EDGE('',*,*,#25561,.F.);
#33167=ORIENTED_EDGE('',*,*,#25562,.F.);
#33168=ORIENTED_EDGE('',*,*,#25563,.F.);
#33169=ORIENTED_EDGE('',*,*,#25564,.F.);
#33170=ORIENTED_EDGE('',*,*,#25565,.F.);
#33171=ORIENTED_EDGE('',*,*,#25566,.F.);
#33172=ORIENTED_EDGE('',*,*,#25567,.F.);
#33173=ORIENTED_EDGE('',*,*,#25454,.T.);
#33174=ORIENTED_EDGE('',*,*,#25568,.T.);
#33175=ORIENTED_EDGE('',*,*,#25569,.T.);
#33176=ORIENTED_EDGE('',*,*,#25570,.F.);
#33177=ORIENTED_EDGE('',*,*,#25571,.F.);
#33178=ORIENTED_EDGE('',*,*,#25572,.F.);
#33179=ORIENTED_EDGE('',*,*,#25537,.T.);
#33180=ORIENTED_EDGE('',*,*,#25451,.T.);
#33181=ORIENTED_EDGE('',*,*,#25573,.F.);
#33182=ORIENTED_EDGE('',*,*,#25574,.F.);
#33183=ORIENTED_EDGE('',*,*,#25575,.F.);
#33184=ORIENTED_EDGE('',*,*,#25576,.F.);
#33185=ORIENTED_EDGE('',*,*,#25577,.F.);
#33186=ORIENTED_EDGE('',*,*,#25578,.F.);
#33187=ORIENTED_EDGE('',*,*,#25579,.F.);
#33188=ORIENTED_EDGE('',*,*,#25580,.F.);
#33189=ORIENTED_EDGE('',*,*,#25581,.F.);
#33190=ORIENTED_EDGE('',*,*,#25582,.F.);
#33191=ORIENTED_EDGE('',*,*,#25583,.F.);
#33192=ORIENTED_EDGE('',*,*,#25584,.F.);
#33193=ORIENTED_EDGE('',*,*,#25585,.F.);
#33194=ORIENTED_EDGE('',*,*,#25586,.F.);
#33195=ORIENTED_EDGE('',*,*,#25587,.F.);
#33196=ORIENTED_EDGE('',*,*,#25588,.T.);
#33197=ORIENTED_EDGE('',*,*,#25589,.F.);
#33198=ORIENTED_EDGE('',*,*,#25590,.F.);
#33199=ORIENTED_EDGE('',*,*,#25591,.F.);
#33200=ORIENTED_EDGE('',*,*,#25592,.F.);
#33201=ORIENTED_EDGE('',*,*,#25593,.F.);
#33202=ORIENTED_EDGE('',*,*,#25594,.F.);
#33203=ORIENTED_EDGE('',*,*,#25595,.F.);
#33204=ORIENTED_EDGE('',*,*,#25596,.F.);
#33205=ORIENTED_EDGE('',*,*,#25597,.F.);
#33206=ORIENTED_EDGE('',*,*,#25598,.F.);
#33207=ORIENTED_EDGE('',*,*,#25599,.F.);
#33208=ORIENTED_EDGE('',*,*,#25600,.F.);
#33209=ORIENTED_EDGE('',*,*,#25601,.F.);
#33210=ORIENTED_EDGE('',*,*,#25602,.F.);
#33211=ORIENTED_EDGE('',*,*,#25603,.F.);
#33212=ORIENTED_EDGE('',*,*,#25450,.T.);
#33213=ORIENTED_EDGE('',*,*,#25604,.T.);
#33214=ORIENTED_EDGE('',*,*,#25605,.T.);
#33215=ORIENTED_EDGE('',*,*,#25606,.F.);
#33216=ORIENTED_EDGE('',*,*,#25607,.F.);
#33217=ORIENTED_EDGE('',*,*,#25608,.F.);
#33218=ORIENTED_EDGE('',*,*,#25573,.T.);
#33219=ORIENTED_EDGE('',*,*,#25447,.T.);
#33220=ORIENTED_EDGE('',*,*,#25609,.F.);
#33221=ORIENTED_EDGE('',*,*,#25610,.F.);
#33222=ORIENTED_EDGE('',*,*,#25611,.F.);
#33223=ORIENTED_EDGE('',*,*,#25612,.F.);
#33224=ORIENTED_EDGE('',*,*,#25613,.F.);
#33225=ORIENTED_EDGE('',*,*,#25614,.F.);
#33226=ORIENTED_EDGE('',*,*,#25615,.F.);
#33227=ORIENTED_EDGE('',*,*,#25616,.F.);
#33228=ORIENTED_EDGE('',*,*,#25617,.F.);
#33229=ORIENTED_EDGE('',*,*,#25618,.F.);
#33230=ORIENTED_EDGE('',*,*,#25619,.F.);
#33231=ORIENTED_EDGE('',*,*,#25620,.F.);
#33232=ORIENTED_EDGE('',*,*,#25621,.F.);
#33233=ORIENTED_EDGE('',*,*,#25622,.F.);
#33234=ORIENTED_EDGE('',*,*,#25623,.F.);
#33235=ORIENTED_EDGE('',*,*,#25624,.T.);
#33236=ORIENTED_EDGE('',*,*,#25625,.F.);
#33237=ORIENTED_EDGE('',*,*,#25626,.F.);
#33238=ORIENTED_EDGE('',*,*,#25627,.F.);
#33239=ORIENTED_EDGE('',*,*,#25628,.F.);
#33240=ORIENTED_EDGE('',*,*,#25629,.F.);
#33241=ORIENTED_EDGE('',*,*,#25630,.F.);
#33242=ORIENTED_EDGE('',*,*,#25631,.F.);
#33243=ORIENTED_EDGE('',*,*,#25632,.F.);
#33244=ORIENTED_EDGE('',*,*,#25633,.F.);
#33245=ORIENTED_EDGE('',*,*,#25634,.F.);
#33246=ORIENTED_EDGE('',*,*,#25635,.F.);
#33247=ORIENTED_EDGE('',*,*,#25636,.F.);
#33248=ORIENTED_EDGE('',*,*,#25637,.F.);
#33249=ORIENTED_EDGE('',*,*,#25638,.F.);
#33250=ORIENTED_EDGE('',*,*,#25639,.F.);
#33251=ORIENTED_EDGE('',*,*,#25446,.T.);
#33252=ORIENTED_EDGE('',*,*,#25640,.T.);
#33253=ORIENTED_EDGE('',*,*,#25641,.T.);
#33254=ORIENTED_EDGE('',*,*,#25642,.F.);
#33255=ORIENTED_EDGE('',*,*,#25643,.F.);
#33256=ORIENTED_EDGE('',*,*,#25644,.F.);
#33257=ORIENTED_EDGE('',*,*,#25609,.T.);
#33258=ORIENTED_EDGE('',*,*,#25443,.T.);
#33259=ORIENTED_EDGE('',*,*,#25645,.F.);
#33260=ORIENTED_EDGE('',*,*,#25646,.F.);
#33261=ORIENTED_EDGE('',*,*,#25647,.F.);
#33262=ORIENTED_EDGE('',*,*,#25648,.F.);
#33263=ORIENTED_EDGE('',*,*,#25649,.F.);
#33264=ORIENTED_EDGE('',*,*,#25650,.F.);
#33265=ORIENTED_EDGE('',*,*,#25651,.F.);
#33266=ORIENTED_EDGE('',*,*,#25652,.F.);
#33267=ORIENTED_EDGE('',*,*,#25653,.F.);
#33268=ORIENTED_EDGE('',*,*,#25654,.F.);
#33269=ORIENTED_EDGE('',*,*,#25655,.F.);
#33270=ORIENTED_EDGE('',*,*,#25656,.F.);
#33271=ORIENTED_EDGE('',*,*,#25657,.F.);
#33272=ORIENTED_EDGE('',*,*,#25658,.F.);
#33273=ORIENTED_EDGE('',*,*,#25659,.F.);
#33274=ORIENTED_EDGE('',*,*,#25660,.T.);
#33275=ORIENTED_EDGE('',*,*,#25661,.F.);
#33276=ORIENTED_EDGE('',*,*,#25662,.F.);
#33277=ORIENTED_EDGE('',*,*,#25663,.F.);
#33278=ORIENTED_EDGE('',*,*,#25664,.F.);
#33279=ORIENTED_EDGE('',*,*,#25665,.F.);
#33280=ORIENTED_EDGE('',*,*,#25666,.F.);
#33281=ORIENTED_EDGE('',*,*,#25667,.F.);
#33282=ORIENTED_EDGE('',*,*,#25668,.F.);
#33283=ORIENTED_EDGE('',*,*,#25669,.F.);
#33284=ORIENTED_EDGE('',*,*,#25670,.F.);
#33285=ORIENTED_EDGE('',*,*,#25671,.F.);
#33286=ORIENTED_EDGE('',*,*,#25672,.F.);
#33287=ORIENTED_EDGE('',*,*,#25673,.F.);
#33288=ORIENTED_EDGE('',*,*,#25674,.F.);
#33289=ORIENTED_EDGE('',*,*,#25675,.F.);
#33290=ORIENTED_EDGE('',*,*,#25442,.T.);
#33291=ORIENTED_EDGE('',*,*,#25676,.T.);
#33292=ORIENTED_EDGE('',*,*,#25677,.T.);
#33293=ORIENTED_EDGE('',*,*,#25678,.F.);
#33294=ORIENTED_EDGE('',*,*,#25679,.F.);
#33295=ORIENTED_EDGE('',*,*,#25680,.F.);
#33296=ORIENTED_EDGE('',*,*,#25645,.T.);
#33297=ORIENTED_EDGE('',*,*,#25439,.T.);
#33298=ORIENTED_EDGE('',*,*,#25681,.F.);
#33299=ORIENTED_EDGE('',*,*,#25682,.F.);
#33300=ORIENTED_EDGE('',*,*,#25683,.F.);
#33301=ORIENTED_EDGE('',*,*,#25684,.F.);
#33302=ORIENTED_EDGE('',*,*,#25685,.F.);
#33303=ORIENTED_EDGE('',*,*,#25686,.F.);
#33304=ORIENTED_EDGE('',*,*,#25687,.F.);
#33305=ORIENTED_EDGE('',*,*,#25688,.F.);
#33306=ORIENTED_EDGE('',*,*,#25689,.F.);
#33307=ORIENTED_EDGE('',*,*,#25690,.F.);
#33308=ORIENTED_EDGE('',*,*,#25691,.F.);
#33309=ORIENTED_EDGE('',*,*,#25692,.F.);
#33310=ORIENTED_EDGE('',*,*,#25693,.F.);
#33311=ORIENTED_EDGE('',*,*,#25694,.F.);
#33312=ORIENTED_EDGE('',*,*,#25695,.F.);
#33313=ORIENTED_EDGE('',*,*,#25696,.T.);
#33314=ORIENTED_EDGE('',*,*,#25697,.F.);
#33315=ORIENTED_EDGE('',*,*,#25698,.F.);
#33316=ORIENTED_EDGE('',*,*,#25699,.F.);
#33317=ORIENTED_EDGE('',*,*,#25700,.F.);
#33318=ORIENTED_EDGE('',*,*,#25701,.F.);
#33319=ORIENTED_EDGE('',*,*,#25702,.F.);
#33320=ORIENTED_EDGE('',*,*,#25703,.F.);
#33321=ORIENTED_EDGE('',*,*,#25704,.F.);
#33322=ORIENTED_EDGE('',*,*,#25705,.F.);
#33323=ORIENTED_EDGE('',*,*,#25706,.F.);
#33324=ORIENTED_EDGE('',*,*,#25707,.F.);
#33325=ORIENTED_EDGE('',*,*,#25708,.F.);
#33326=ORIENTED_EDGE('',*,*,#25709,.F.);
#33327=ORIENTED_EDGE('',*,*,#25710,.F.);
#33328=ORIENTED_EDGE('',*,*,#25711,.F.);
#33329=ORIENTED_EDGE('',*,*,#25438,.T.);
#33330=ORIENTED_EDGE('',*,*,#25712,.T.);
#33331=ORIENTED_EDGE('',*,*,#25713,.T.);
#33332=ORIENTED_EDGE('',*,*,#25714,.F.);
#33333=ORIENTED_EDGE('',*,*,#25715,.F.);
#33334=ORIENTED_EDGE('',*,*,#25716,.F.);
#33335=ORIENTED_EDGE('',*,*,#25681,.T.);
#33336=ORIENTED_EDGE('',*,*,#25435,.T.);
#33337=ORIENTED_EDGE('',*,*,#25717,.F.);
#33338=ORIENTED_EDGE('',*,*,#25718,.F.);
#33339=ORIENTED_EDGE('',*,*,#25719,.F.);
#33340=ORIENTED_EDGE('',*,*,#25720,.F.);
#33341=ORIENTED_EDGE('',*,*,#25721,.F.);
#33342=ORIENTED_EDGE('',*,*,#25722,.F.);
#33343=ORIENTED_EDGE('',*,*,#25723,.F.);
#33344=ORIENTED_EDGE('',*,*,#25724,.F.);
#33345=ORIENTED_EDGE('',*,*,#25725,.F.);
#33346=ORIENTED_EDGE('',*,*,#25726,.F.);
#33347=ORIENTED_EDGE('',*,*,#25727,.F.);
#33348=ORIENTED_EDGE('',*,*,#25728,.F.);
#33349=ORIENTED_EDGE('',*,*,#25729,.F.);
#33350=ORIENTED_EDGE('',*,*,#25730,.F.);
#33351=ORIENTED_EDGE('',*,*,#25731,.F.);
#33352=ORIENTED_EDGE('',*,*,#25732,.T.);
#33353=ORIENTED_EDGE('',*,*,#25733,.F.);
#33354=ORIENTED_EDGE('',*,*,#25734,.F.);
#33355=ORIENTED_EDGE('',*,*,#25735,.F.);
#33356=ORIENTED_EDGE('',*,*,#25736,.F.);
#33357=ORIENTED_EDGE('',*,*,#25737,.F.);
#33358=ORIENTED_EDGE('',*,*,#25738,.F.);
#33359=ORIENTED_EDGE('',*,*,#25739,.F.);
#33360=ORIENTED_EDGE('',*,*,#25740,.F.);
#33361=ORIENTED_EDGE('',*,*,#25741,.F.);
#33362=ORIENTED_EDGE('',*,*,#25742,.F.);
#33363=ORIENTED_EDGE('',*,*,#25743,.F.);
#33364=ORIENTED_EDGE('',*,*,#25744,.F.);
#33365=ORIENTED_EDGE('',*,*,#25745,.F.);
#33366=ORIENTED_EDGE('',*,*,#25746,.F.);
#33367=ORIENTED_EDGE('',*,*,#25747,.F.);
#33368=ORIENTED_EDGE('',*,*,#25434,.T.);
#33369=ORIENTED_EDGE('',*,*,#25748,.T.);
#33370=ORIENTED_EDGE('',*,*,#25749,.T.);
#33371=ORIENTED_EDGE('',*,*,#25750,.F.);
#33372=ORIENTED_EDGE('',*,*,#25751,.F.);
#33373=ORIENTED_EDGE('',*,*,#25752,.F.);
#33374=ORIENTED_EDGE('',*,*,#25717,.T.);
#33375=ORIENTED_EDGE('',*,*,#25431,.T.);
#33376=ORIENTED_EDGE('',*,*,#25753,.F.);
#33377=ORIENTED_EDGE('',*,*,#25754,.F.);
#33378=ORIENTED_EDGE('',*,*,#25755,.F.);
#33379=ORIENTED_EDGE('',*,*,#25756,.F.);
#33380=ORIENTED_EDGE('',*,*,#25757,.F.);
#33381=ORIENTED_EDGE('',*,*,#25758,.F.);
#33382=ORIENTED_EDGE('',*,*,#25759,.F.);
#33383=ORIENTED_EDGE('',*,*,#25760,.F.);
#33384=ORIENTED_EDGE('',*,*,#25761,.F.);
#33385=ORIENTED_EDGE('',*,*,#25762,.F.);
#33386=ORIENTED_EDGE('',*,*,#25763,.F.);
#33387=ORIENTED_EDGE('',*,*,#25764,.F.);
#33388=ORIENTED_EDGE('',*,*,#25765,.F.);
#33389=ORIENTED_EDGE('',*,*,#25766,.F.);
#33390=ORIENTED_EDGE('',*,*,#25767,.F.);
#33391=ORIENTED_EDGE('',*,*,#25768,.T.);
#33392=ORIENTED_EDGE('',*,*,#25769,.F.);
#33393=ORIENTED_EDGE('',*,*,#25770,.F.);
#33394=ORIENTED_EDGE('',*,*,#25771,.F.);
#33395=ORIENTED_EDGE('',*,*,#25772,.F.);
#33396=ORIENTED_EDGE('',*,*,#25773,.F.);
#33397=ORIENTED_EDGE('',*,*,#25774,.F.);
#33398=ORIENTED_EDGE('',*,*,#25775,.F.);
#33399=ORIENTED_EDGE('',*,*,#25776,.F.);
#33400=ORIENTED_EDGE('',*,*,#25777,.F.);
#33401=ORIENTED_EDGE('',*,*,#25778,.F.);
#33402=ORIENTED_EDGE('',*,*,#25779,.F.);
#33403=ORIENTED_EDGE('',*,*,#25780,.F.);
#33404=ORIENTED_EDGE('',*,*,#25781,.F.);
#33405=ORIENTED_EDGE('',*,*,#25782,.F.);
#33406=ORIENTED_EDGE('',*,*,#25783,.F.);
#33407=ORIENTED_EDGE('',*,*,#25430,.T.);
#33408=ORIENTED_EDGE('',*,*,#25784,.T.);
#33409=ORIENTED_EDGE('',*,*,#25785,.T.);
#33410=ORIENTED_EDGE('',*,*,#25786,.F.);
#33411=ORIENTED_EDGE('',*,*,#25787,.F.);
#33412=ORIENTED_EDGE('',*,*,#25788,.F.);
#33413=ORIENTED_EDGE('',*,*,#25753,.T.);
#33414=ORIENTED_EDGE('',*,*,#25427,.T.);
#33415=ORIENTED_EDGE('',*,*,#25789,.F.);
#33416=ORIENTED_EDGE('',*,*,#25790,.F.);
#33417=ORIENTED_EDGE('',*,*,#25791,.F.);
#33418=ORIENTED_EDGE('',*,*,#25792,.F.);
#33419=ORIENTED_EDGE('',*,*,#25793,.F.);
#33420=ORIENTED_EDGE('',*,*,#25794,.F.);
#33421=ORIENTED_EDGE('',*,*,#25795,.F.);
#33422=ORIENTED_EDGE('',*,*,#25796,.F.);
#33423=ORIENTED_EDGE('',*,*,#25797,.F.);
#33424=ORIENTED_EDGE('',*,*,#25798,.F.);
#33425=ORIENTED_EDGE('',*,*,#25799,.F.);
#33426=ORIENTED_EDGE('',*,*,#25800,.F.);
#33427=ORIENTED_EDGE('',*,*,#25801,.F.);
#33428=ORIENTED_EDGE('',*,*,#25802,.F.);
#33429=ORIENTED_EDGE('',*,*,#25803,.F.);
#33430=ORIENTED_EDGE('',*,*,#25804,.T.);
#33431=ORIENTED_EDGE('',*,*,#25805,.F.);
#33432=ORIENTED_EDGE('',*,*,#25806,.F.);
#33433=ORIENTED_EDGE('',*,*,#25807,.F.);
#33434=ORIENTED_EDGE('',*,*,#25808,.F.);
#33435=ORIENTED_EDGE('',*,*,#25809,.F.);
#33436=ORIENTED_EDGE('',*,*,#25810,.F.);
#33437=ORIENTED_EDGE('',*,*,#25811,.F.);
#33438=ORIENTED_EDGE('',*,*,#25812,.F.);
#33439=ORIENTED_EDGE('',*,*,#25813,.F.);
#33440=ORIENTED_EDGE('',*,*,#25814,.F.);
#33441=ORIENTED_EDGE('',*,*,#25815,.F.);
#33442=ORIENTED_EDGE('',*,*,#25816,.F.);
#33443=ORIENTED_EDGE('',*,*,#25817,.F.);
#33444=ORIENTED_EDGE('',*,*,#25818,.F.);
#33445=ORIENTED_EDGE('',*,*,#25819,.F.);
#33446=ORIENTED_EDGE('',*,*,#25426,.T.);
#33447=ORIENTED_EDGE('',*,*,#25820,.T.);
#33448=ORIENTED_EDGE('',*,*,#25821,.T.);
#33449=ORIENTED_EDGE('',*,*,#25822,.F.);
#33450=ORIENTED_EDGE('',*,*,#25823,.F.);
#33451=ORIENTED_EDGE('',*,*,#25824,.F.);
#33452=ORIENTED_EDGE('',*,*,#25789,.T.);
#33453=ORIENTED_EDGE('',*,*,#25423,.T.);
#33454=ORIENTED_EDGE('',*,*,#25825,.F.);
#33455=ORIENTED_EDGE('',*,*,#25826,.F.);
#33456=ORIENTED_EDGE('',*,*,#25827,.F.);
#33457=ORIENTED_EDGE('',*,*,#25828,.F.);
#33458=ORIENTED_EDGE('',*,*,#25829,.F.);
#33459=ORIENTED_EDGE('',*,*,#25830,.F.);
#33460=ORIENTED_EDGE('',*,*,#25831,.F.);
#33461=ORIENTED_EDGE('',*,*,#25832,.F.);
#33462=ORIENTED_EDGE('',*,*,#25833,.F.);
#33463=ORIENTED_EDGE('',*,*,#25834,.F.);
#33464=ORIENTED_EDGE('',*,*,#25835,.F.);
#33465=ORIENTED_EDGE('',*,*,#25836,.F.);
#33466=ORIENTED_EDGE('',*,*,#25837,.F.);
#33467=ORIENTED_EDGE('',*,*,#25838,.F.);
#33468=ORIENTED_EDGE('',*,*,#25839,.F.);
#33469=ORIENTED_EDGE('',*,*,#25840,.T.);
#33470=ORIENTED_EDGE('',*,*,#25841,.F.);
#33471=ORIENTED_EDGE('',*,*,#25842,.F.);
#33472=ORIENTED_EDGE('',*,*,#25843,.F.);
#33473=ORIENTED_EDGE('',*,*,#25844,.F.);
#33474=ORIENTED_EDGE('',*,*,#25845,.F.);
#33475=ORIENTED_EDGE('',*,*,#25846,.F.);
#33476=ORIENTED_EDGE('',*,*,#25847,.F.);
#33477=ORIENTED_EDGE('',*,*,#25848,.F.);
#33478=ORIENTED_EDGE('',*,*,#25849,.F.);
#33479=ORIENTED_EDGE('',*,*,#25850,.F.);
#33480=ORIENTED_EDGE('',*,*,#25851,.F.);
#33481=ORIENTED_EDGE('',*,*,#25852,.F.);
#33482=ORIENTED_EDGE('',*,*,#25853,.F.);
#33483=ORIENTED_EDGE('',*,*,#25854,.F.);
#33484=ORIENTED_EDGE('',*,*,#25855,.F.);
#33485=ORIENTED_EDGE('',*,*,#25422,.T.);
#33486=ORIENTED_EDGE('',*,*,#25856,.T.);
#33487=ORIENTED_EDGE('',*,*,#25857,.T.);
#33488=ORIENTED_EDGE('',*,*,#25858,.F.);
#33489=ORIENTED_EDGE('',*,*,#25859,.F.);
#33490=ORIENTED_EDGE('',*,*,#25860,.F.);
#33491=ORIENTED_EDGE('',*,*,#25825,.T.);
#33492=ORIENTED_EDGE('',*,*,#25419,.T.);
#33493=ORIENTED_EDGE('',*,*,#25861,.F.);
#33494=ORIENTED_EDGE('',*,*,#25862,.F.);
#33495=ORIENTED_EDGE('',*,*,#25863,.F.);
#33496=ORIENTED_EDGE('',*,*,#25864,.F.);
#33497=ORIENTED_EDGE('',*,*,#25865,.F.);
#33498=ORIENTED_EDGE('',*,*,#25866,.F.);
#33499=ORIENTED_EDGE('',*,*,#25867,.F.);
#33500=ORIENTED_EDGE('',*,*,#25868,.F.);
#33501=ORIENTED_EDGE('',*,*,#25869,.F.);
#33502=ORIENTED_EDGE('',*,*,#25870,.F.);
#33503=ORIENTED_EDGE('',*,*,#25871,.F.);
#33504=ORIENTED_EDGE('',*,*,#25872,.F.);
#33505=ORIENTED_EDGE('',*,*,#25873,.F.);
#33506=ORIENTED_EDGE('',*,*,#25874,.F.);
#33507=ORIENTED_EDGE('',*,*,#25875,.F.);
#33508=ORIENTED_EDGE('',*,*,#25876,.T.);
#33509=ORIENTED_EDGE('',*,*,#25877,.F.);
#33510=ORIENTED_EDGE('',*,*,#25878,.F.);
#33511=ORIENTED_EDGE('',*,*,#25879,.F.);
#33512=ORIENTED_EDGE('',*,*,#25880,.F.);
#33513=ORIENTED_EDGE('',*,*,#25881,.F.);
#33514=ORIENTED_EDGE('',*,*,#25882,.F.);
#33515=ORIENTED_EDGE('',*,*,#25883,.F.);
#33516=ORIENTED_EDGE('',*,*,#25884,.F.);
#33517=ORIENTED_EDGE('',*,*,#25885,.F.);
#33518=ORIENTED_EDGE('',*,*,#25886,.F.);
#33519=ORIENTED_EDGE('',*,*,#25887,.F.);
#33520=ORIENTED_EDGE('',*,*,#25888,.F.);
#33521=ORIENTED_EDGE('',*,*,#25889,.F.);
#33522=ORIENTED_EDGE('',*,*,#25890,.F.);
#33523=ORIENTED_EDGE('',*,*,#25891,.F.);
#33524=ORIENTED_EDGE('',*,*,#25418,.T.);
#33525=ORIENTED_EDGE('',*,*,#25892,.T.);
#33526=ORIENTED_EDGE('',*,*,#25893,.T.);
#33527=ORIENTED_EDGE('',*,*,#25894,.F.);
#33528=ORIENTED_EDGE('',*,*,#25895,.F.);
#33529=ORIENTED_EDGE('',*,*,#25896,.F.);
#33530=ORIENTED_EDGE('',*,*,#25861,.T.);
#33531=ORIENTED_EDGE('',*,*,#25415,.T.);
#33532=ORIENTED_EDGE('',*,*,#25897,.F.);
#33533=ORIENTED_EDGE('',*,*,#25898,.F.);
#33534=ORIENTED_EDGE('',*,*,#25899,.F.);
#33535=ORIENTED_EDGE('',*,*,#25900,.F.);
#33536=ORIENTED_EDGE('',*,*,#25901,.F.);
#33537=ORIENTED_EDGE('',*,*,#25902,.F.);
#33538=ORIENTED_EDGE('',*,*,#25903,.F.);
#33539=ORIENTED_EDGE('',*,*,#25904,.F.);
#33540=ORIENTED_EDGE('',*,*,#25905,.F.);
#33541=ORIENTED_EDGE('',*,*,#25906,.F.);
#33542=ORIENTED_EDGE('',*,*,#25907,.F.);
#33543=ORIENTED_EDGE('',*,*,#25908,.F.);
#33544=ORIENTED_EDGE('',*,*,#25909,.F.);
#33545=ORIENTED_EDGE('',*,*,#25910,.F.);
#33546=ORIENTED_EDGE('',*,*,#25911,.F.);
#33547=ORIENTED_EDGE('',*,*,#25912,.T.);
#33548=ORIENTED_EDGE('',*,*,#25913,.F.);
#33549=ORIENTED_EDGE('',*,*,#25914,.F.);
#33550=ORIENTED_EDGE('',*,*,#25915,.F.);
#33551=ORIENTED_EDGE('',*,*,#25916,.F.);
#33552=ORIENTED_EDGE('',*,*,#25917,.F.);
#33553=ORIENTED_EDGE('',*,*,#25918,.F.);
#33554=ORIENTED_EDGE('',*,*,#25919,.F.);
#33555=ORIENTED_EDGE('',*,*,#25920,.F.);
#33556=ORIENTED_EDGE('',*,*,#25921,.F.);
#33557=ORIENTED_EDGE('',*,*,#25922,.F.);
#33558=ORIENTED_EDGE('',*,*,#25923,.F.);
#33559=ORIENTED_EDGE('',*,*,#25924,.F.);
#33560=ORIENTED_EDGE('',*,*,#25925,.F.);
#33561=ORIENTED_EDGE('',*,*,#25926,.F.);
#33562=ORIENTED_EDGE('',*,*,#25927,.F.);
#33563=ORIENTED_EDGE('',*,*,#25414,.T.);
#33564=ORIENTED_EDGE('',*,*,#25928,.T.);
#33565=ORIENTED_EDGE('',*,*,#25929,.T.);
#33566=ORIENTED_EDGE('',*,*,#25930,.F.);
#33567=ORIENTED_EDGE('',*,*,#25931,.F.);
#33568=ORIENTED_EDGE('',*,*,#25932,.F.);
#33569=ORIENTED_EDGE('',*,*,#25897,.T.);
#33570=ORIENTED_EDGE('',*,*,#25411,.T.);
#33571=ORIENTED_EDGE('',*,*,#25933,.F.);
#33572=ORIENTED_EDGE('',*,*,#25934,.F.);
#33573=ORIENTED_EDGE('',*,*,#25935,.F.);
#33574=ORIENTED_EDGE('',*,*,#25936,.F.);
#33575=ORIENTED_EDGE('',*,*,#25937,.F.);
#33576=ORIENTED_EDGE('',*,*,#25938,.F.);
#33577=ORIENTED_EDGE('',*,*,#25939,.F.);
#33578=ORIENTED_EDGE('',*,*,#25940,.F.);
#33579=ORIENTED_EDGE('',*,*,#25941,.F.);
#33580=ORIENTED_EDGE('',*,*,#25942,.F.);
#33581=ORIENTED_EDGE('',*,*,#25943,.F.);
#33582=ORIENTED_EDGE('',*,*,#25944,.F.);
#33583=ORIENTED_EDGE('',*,*,#25945,.F.);
#33584=ORIENTED_EDGE('',*,*,#25946,.F.);
#33585=ORIENTED_EDGE('',*,*,#25947,.F.);
#33586=ORIENTED_EDGE('',*,*,#25948,.T.);
#33587=ORIENTED_EDGE('',*,*,#25949,.F.);
#33588=ORIENTED_EDGE('',*,*,#25950,.F.);
#33589=ORIENTED_EDGE('',*,*,#25951,.F.);
#33590=ORIENTED_EDGE('',*,*,#25952,.F.);
#33591=ORIENTED_EDGE('',*,*,#25953,.F.);
#33592=ORIENTED_EDGE('',*,*,#25954,.F.);
#33593=ORIENTED_EDGE('',*,*,#25955,.F.);
#33594=ORIENTED_EDGE('',*,*,#25956,.F.);
#33595=ORIENTED_EDGE('',*,*,#25957,.F.);
#33596=ORIENTED_EDGE('',*,*,#25958,.F.);
#33597=ORIENTED_EDGE('',*,*,#25959,.F.);
#33598=ORIENTED_EDGE('',*,*,#25960,.F.);
#33599=ORIENTED_EDGE('',*,*,#25961,.F.);
#33600=ORIENTED_EDGE('',*,*,#25962,.F.);
#33601=ORIENTED_EDGE('',*,*,#25963,.F.);
#33602=ORIENTED_EDGE('',*,*,#25410,.T.);
#33603=ORIENTED_EDGE('',*,*,#25964,.T.);
#33604=ORIENTED_EDGE('',*,*,#25965,.T.);
#33605=ORIENTED_EDGE('',*,*,#25966,.F.);
#33606=ORIENTED_EDGE('',*,*,#25967,.F.);
#33607=ORIENTED_EDGE('',*,*,#25968,.F.);
#33608=ORIENTED_EDGE('',*,*,#25933,.T.);
#33609=ORIENTED_EDGE('',*,*,#25407,.T.);
#33610=ORIENTED_EDGE('',*,*,#25969,.F.);
#33611=ORIENTED_EDGE('',*,*,#25970,.F.);
#33612=ORIENTED_EDGE('',*,*,#25971,.F.);
#33613=ORIENTED_EDGE('',*,*,#25972,.F.);
#33614=ORIENTED_EDGE('',*,*,#25973,.F.);
#33615=ORIENTED_EDGE('',*,*,#25974,.F.);
#33616=ORIENTED_EDGE('',*,*,#25975,.F.);
#33617=ORIENTED_EDGE('',*,*,#25976,.F.);
#33618=ORIENTED_EDGE('',*,*,#25977,.F.);
#33619=ORIENTED_EDGE('',*,*,#25978,.F.);
#33620=ORIENTED_EDGE('',*,*,#25979,.F.);
#33621=ORIENTED_EDGE('',*,*,#25980,.F.);
#33622=ORIENTED_EDGE('',*,*,#25981,.F.);
#33623=ORIENTED_EDGE('',*,*,#25982,.F.);
#33624=ORIENTED_EDGE('',*,*,#25983,.F.);
#33625=ORIENTED_EDGE('',*,*,#25984,.T.);
#33626=ORIENTED_EDGE('',*,*,#25985,.F.);
#33627=ORIENTED_EDGE('',*,*,#25986,.F.);
#33628=ORIENTED_EDGE('',*,*,#25987,.F.);
#33629=ORIENTED_EDGE('',*,*,#25988,.F.);
#33630=ORIENTED_EDGE('',*,*,#25989,.F.);
#33631=ORIENTED_EDGE('',*,*,#25990,.F.);
#33632=ORIENTED_EDGE('',*,*,#25991,.F.);
#33633=ORIENTED_EDGE('',*,*,#25992,.F.);
#33634=ORIENTED_EDGE('',*,*,#25993,.F.);
#33635=ORIENTED_EDGE('',*,*,#25994,.F.);
#33636=ORIENTED_EDGE('',*,*,#25995,.F.);
#33637=ORIENTED_EDGE('',*,*,#25996,.F.);
#33638=ORIENTED_EDGE('',*,*,#25997,.F.);
#33639=ORIENTED_EDGE('',*,*,#25998,.F.);
#33640=ORIENTED_EDGE('',*,*,#25999,.F.);
#33641=ORIENTED_EDGE('',*,*,#25406,.T.);
#33642=ORIENTED_EDGE('',*,*,#26000,.T.);
#33643=ORIENTED_EDGE('',*,*,#26001,.T.);
#33644=ORIENTED_EDGE('',*,*,#26002,.F.);
#33645=ORIENTED_EDGE('',*,*,#26003,.F.);
#33646=ORIENTED_EDGE('',*,*,#26004,.F.);
#33647=ORIENTED_EDGE('',*,*,#25969,.T.);
#33648=ORIENTED_EDGE('',*,*,#25403,.T.);
#33649=ORIENTED_EDGE('',*,*,#26005,.F.);
#33650=ORIENTED_EDGE('',*,*,#26006,.F.);
#33651=ORIENTED_EDGE('',*,*,#26007,.F.);
#33652=ORIENTED_EDGE('',*,*,#26008,.F.);
#33653=ORIENTED_EDGE('',*,*,#26009,.F.);
#33654=ORIENTED_EDGE('',*,*,#26010,.F.);
#33655=ORIENTED_EDGE('',*,*,#26011,.F.);
#33656=ORIENTED_EDGE('',*,*,#26012,.F.);
#33657=ORIENTED_EDGE('',*,*,#26013,.F.);
#33658=ORIENTED_EDGE('',*,*,#26014,.F.);
#33659=ORIENTED_EDGE('',*,*,#26015,.F.);
#33660=ORIENTED_EDGE('',*,*,#26016,.F.);
#33661=ORIENTED_EDGE('',*,*,#26017,.F.);
#33662=ORIENTED_EDGE('',*,*,#26018,.F.);
#33663=ORIENTED_EDGE('',*,*,#26019,.F.);
#33664=ORIENTED_EDGE('',*,*,#26020,.T.);
#33665=ORIENTED_EDGE('',*,*,#26021,.F.);
#33666=ORIENTED_EDGE('',*,*,#26022,.F.);
#33667=ORIENTED_EDGE('',*,*,#26023,.F.);
#33668=ORIENTED_EDGE('',*,*,#26024,.F.);
#33669=ORIENTED_EDGE('',*,*,#26025,.F.);
#33670=ORIENTED_EDGE('',*,*,#26026,.F.);
#33671=ORIENTED_EDGE('',*,*,#26027,.F.);
#33672=ORIENTED_EDGE('',*,*,#26028,.F.);
#33673=ORIENTED_EDGE('',*,*,#26029,.F.);
#33674=ORIENTED_EDGE('',*,*,#26030,.F.);
#33675=ORIENTED_EDGE('',*,*,#26031,.F.);
#33676=ORIENTED_EDGE('',*,*,#26032,.F.);
#33677=ORIENTED_EDGE('',*,*,#26033,.F.);
#33678=ORIENTED_EDGE('',*,*,#26034,.F.);
#33679=ORIENTED_EDGE('',*,*,#26035,.F.);
#33680=ORIENTED_EDGE('',*,*,#25402,.T.);
#33681=ORIENTED_EDGE('',*,*,#26036,.T.);
#33682=ORIENTED_EDGE('',*,*,#26037,.T.);
#33683=ORIENTED_EDGE('',*,*,#26038,.F.);
#33684=ORIENTED_EDGE('',*,*,#26039,.F.);
#33685=ORIENTED_EDGE('',*,*,#26040,.F.);
#33686=ORIENTED_EDGE('',*,*,#26005,.T.);
#33687=ORIENTED_EDGE('',*,*,#25399,.T.);
#33688=ORIENTED_EDGE('',*,*,#26041,.F.);
#33689=ORIENTED_EDGE('',*,*,#26042,.F.);
#33690=ORIENTED_EDGE('',*,*,#26043,.F.);
#33691=ORIENTED_EDGE('',*,*,#26044,.F.);
#33692=ORIENTED_EDGE('',*,*,#26045,.F.);
#33693=ORIENTED_EDGE('',*,*,#26046,.F.);
#33694=ORIENTED_EDGE('',*,*,#26047,.F.);
#33695=ORIENTED_EDGE('',*,*,#26048,.F.);
#33696=ORIENTED_EDGE('',*,*,#26049,.F.);
#33697=ORIENTED_EDGE('',*,*,#26050,.F.);
#33698=ORIENTED_EDGE('',*,*,#26051,.F.);
#33699=ORIENTED_EDGE('',*,*,#26052,.F.);
#33700=ORIENTED_EDGE('',*,*,#26053,.F.);
#33701=ORIENTED_EDGE('',*,*,#26054,.F.);
#33702=ORIENTED_EDGE('',*,*,#26055,.F.);
#33703=ORIENTED_EDGE('',*,*,#26056,.T.);
#33704=ORIENTED_EDGE('',*,*,#26057,.F.);
#33705=ORIENTED_EDGE('',*,*,#26058,.F.);
#33706=ORIENTED_EDGE('',*,*,#26059,.F.);
#33707=ORIENTED_EDGE('',*,*,#26060,.F.);
#33708=ORIENTED_EDGE('',*,*,#26061,.F.);
#33709=ORIENTED_EDGE('',*,*,#26062,.F.);
#33710=ORIENTED_EDGE('',*,*,#26063,.F.);
#33711=ORIENTED_EDGE('',*,*,#26064,.F.);
#33712=ORIENTED_EDGE('',*,*,#26065,.F.);
#33713=ORIENTED_EDGE('',*,*,#26066,.F.);
#33714=ORIENTED_EDGE('',*,*,#26067,.F.);
#33715=ORIENTED_EDGE('',*,*,#26068,.F.);
#33716=ORIENTED_EDGE('',*,*,#26069,.F.);
#33717=ORIENTED_EDGE('',*,*,#26070,.F.);
#33718=ORIENTED_EDGE('',*,*,#26071,.F.);
#33719=ORIENTED_EDGE('',*,*,#25398,.T.);
#33720=ORIENTED_EDGE('',*,*,#26072,.T.);
#33721=ORIENTED_EDGE('',*,*,#26073,.T.);
#33722=ORIENTED_EDGE('',*,*,#26074,.F.);
#33723=ORIENTED_EDGE('',*,*,#26075,.F.);
#33724=ORIENTED_EDGE('',*,*,#26076,.F.);
#33725=ORIENTED_EDGE('',*,*,#26041,.T.);
#33726=ORIENTED_EDGE('',*,*,#25395,.T.);
#33727=ORIENTED_EDGE('',*,*,#26077,.F.);
#33728=ORIENTED_EDGE('',*,*,#26078,.F.);
#33729=ORIENTED_EDGE('',*,*,#26079,.F.);
#33730=ORIENTED_EDGE('',*,*,#26080,.F.);
#33731=ORIENTED_EDGE('',*,*,#26081,.F.);
#33732=ORIENTED_EDGE('',*,*,#26082,.F.);
#33733=ORIENTED_EDGE('',*,*,#26083,.F.);
#33734=ORIENTED_EDGE('',*,*,#26084,.F.);
#33735=ORIENTED_EDGE('',*,*,#26085,.F.);
#33736=ORIENTED_EDGE('',*,*,#26086,.F.);
#33737=ORIENTED_EDGE('',*,*,#26087,.F.);
#33738=ORIENTED_EDGE('',*,*,#26088,.F.);
#33739=ORIENTED_EDGE('',*,*,#26089,.F.);
#33740=ORIENTED_EDGE('',*,*,#26090,.F.);
#33741=ORIENTED_EDGE('',*,*,#26091,.F.);
#33742=ORIENTED_EDGE('',*,*,#26092,.T.);
#33743=ORIENTED_EDGE('',*,*,#26093,.F.);
#33744=ORIENTED_EDGE('',*,*,#26094,.F.);
#33745=ORIENTED_EDGE('',*,*,#26095,.F.);
#33746=ORIENTED_EDGE('',*,*,#26096,.F.);
#33747=ORIENTED_EDGE('',*,*,#26097,.F.);
#33748=ORIENTED_EDGE('',*,*,#26098,.F.);
#33749=ORIENTED_EDGE('',*,*,#26099,.F.);
#33750=ORIENTED_EDGE('',*,*,#26100,.F.);
#33751=ORIENTED_EDGE('',*,*,#26101,.F.);
#33752=ORIENTED_EDGE('',*,*,#26102,.F.);
#33753=ORIENTED_EDGE('',*,*,#26103,.F.);
#33754=ORIENTED_EDGE('',*,*,#26104,.F.);
#33755=ORIENTED_EDGE('',*,*,#26105,.F.);
#33756=ORIENTED_EDGE('',*,*,#26106,.F.);
#33757=ORIENTED_EDGE('',*,*,#26107,.F.);
#33758=ORIENTED_EDGE('',*,*,#25394,.T.);
#33759=ORIENTED_EDGE('',*,*,#26108,.T.);
#33760=ORIENTED_EDGE('',*,*,#26109,.T.);
#33761=ORIENTED_EDGE('',*,*,#26110,.F.);
#33762=ORIENTED_EDGE('',*,*,#26111,.F.);
#33763=ORIENTED_EDGE('',*,*,#26112,.F.);
#33764=ORIENTED_EDGE('',*,*,#26077,.T.);
#33765=ORIENTED_EDGE('',*,*,#25391,.T.);
#33766=ORIENTED_EDGE('',*,*,#26113,.F.);
#33767=ORIENTED_EDGE('',*,*,#26114,.F.);
#33768=ORIENTED_EDGE('',*,*,#26115,.F.);
#33769=ORIENTED_EDGE('',*,*,#26116,.F.);
#33770=ORIENTED_EDGE('',*,*,#26117,.F.);
#33771=ORIENTED_EDGE('',*,*,#26118,.F.);
#33772=ORIENTED_EDGE('',*,*,#26119,.F.);
#33773=ORIENTED_EDGE('',*,*,#26120,.F.);
#33774=ORIENTED_EDGE('',*,*,#26121,.F.);
#33775=ORIENTED_EDGE('',*,*,#26122,.F.);
#33776=ORIENTED_EDGE('',*,*,#26123,.F.);
#33777=ORIENTED_EDGE('',*,*,#26124,.F.);
#33778=ORIENTED_EDGE('',*,*,#26125,.F.);
#33779=ORIENTED_EDGE('',*,*,#26126,.F.);
#33780=ORIENTED_EDGE('',*,*,#26127,.F.);
#33781=ORIENTED_EDGE('',*,*,#26128,.T.);
#33782=ORIENTED_EDGE('',*,*,#26129,.F.);
#33783=ORIENTED_EDGE('',*,*,#26130,.F.);
#33784=ORIENTED_EDGE('',*,*,#26131,.F.);
#33785=ORIENTED_EDGE('',*,*,#26132,.F.);
#33786=ORIENTED_EDGE('',*,*,#26133,.F.);
#33787=ORIENTED_EDGE('',*,*,#26134,.F.);
#33788=ORIENTED_EDGE('',*,*,#26135,.F.);
#33789=ORIENTED_EDGE('',*,*,#26136,.F.);
#33790=ORIENTED_EDGE('',*,*,#26137,.F.);
#33791=ORIENTED_EDGE('',*,*,#26138,.F.);
#33792=ORIENTED_EDGE('',*,*,#26139,.F.);
#33793=ORIENTED_EDGE('',*,*,#26140,.F.);
#33794=ORIENTED_EDGE('',*,*,#26141,.F.);
#33795=ORIENTED_EDGE('',*,*,#26142,.F.);
#33796=ORIENTED_EDGE('',*,*,#26143,.F.);
#33797=ORIENTED_EDGE('',*,*,#25390,.T.);
#33798=ORIENTED_EDGE('',*,*,#26144,.T.);
#33799=ORIENTED_EDGE('',*,*,#26145,.T.);
#33800=ORIENTED_EDGE('',*,*,#26146,.F.);
#33801=ORIENTED_EDGE('',*,*,#26147,.F.);
#33802=ORIENTED_EDGE('',*,*,#26148,.F.);
#33803=ORIENTED_EDGE('',*,*,#26113,.T.);
#33804=ORIENTED_EDGE('',*,*,#25387,.T.);
#33805=ORIENTED_EDGE('',*,*,#26149,.F.);
#33806=ORIENTED_EDGE('',*,*,#26150,.F.);
#33807=ORIENTED_EDGE('',*,*,#26151,.F.);
#33808=ORIENTED_EDGE('',*,*,#26152,.F.);
#33809=ORIENTED_EDGE('',*,*,#26153,.F.);
#33810=ORIENTED_EDGE('',*,*,#26154,.F.);
#33811=ORIENTED_EDGE('',*,*,#26155,.F.);
#33812=ORIENTED_EDGE('',*,*,#26156,.F.);
#33813=ORIENTED_EDGE('',*,*,#26157,.F.);
#33814=ORIENTED_EDGE('',*,*,#26158,.F.);
#33815=ORIENTED_EDGE('',*,*,#26159,.F.);
#33816=ORIENTED_EDGE('',*,*,#26160,.F.);
#33817=ORIENTED_EDGE('',*,*,#26161,.F.);
#33818=ORIENTED_EDGE('',*,*,#26162,.F.);
#33819=ORIENTED_EDGE('',*,*,#26163,.F.);
#33820=ORIENTED_EDGE('',*,*,#26164,.T.);
#33821=ORIENTED_EDGE('',*,*,#26165,.F.);
#33822=ORIENTED_EDGE('',*,*,#26166,.F.);
#33823=ORIENTED_EDGE('',*,*,#26167,.F.);
#33824=ORIENTED_EDGE('',*,*,#26168,.F.);
#33825=ORIENTED_EDGE('',*,*,#26169,.F.);
#33826=ORIENTED_EDGE('',*,*,#26170,.F.);
#33827=ORIENTED_EDGE('',*,*,#26171,.F.);
#33828=ORIENTED_EDGE('',*,*,#26172,.F.);
#33829=ORIENTED_EDGE('',*,*,#26173,.F.);
#33830=ORIENTED_EDGE('',*,*,#26174,.F.);
#33831=ORIENTED_EDGE('',*,*,#26175,.F.);
#33832=ORIENTED_EDGE('',*,*,#26176,.F.);
#33833=ORIENTED_EDGE('',*,*,#26177,.F.);
#33834=ORIENTED_EDGE('',*,*,#26178,.F.);
#33835=ORIENTED_EDGE('',*,*,#26179,.F.);
#33836=ORIENTED_EDGE('',*,*,#25386,.T.);
#33837=ORIENTED_EDGE('',*,*,#26180,.T.);
#33838=ORIENTED_EDGE('',*,*,#26181,.T.);
#33839=ORIENTED_EDGE('',*,*,#26182,.F.);
#33840=ORIENTED_EDGE('',*,*,#26183,.F.);
#33841=ORIENTED_EDGE('',*,*,#26184,.F.);
#33842=ORIENTED_EDGE('',*,*,#26149,.T.);
#33843=ORIENTED_EDGE('',*,*,#25383,.T.);
#33844=ORIENTED_EDGE('',*,*,#26185,.F.);
#33845=ORIENTED_EDGE('',*,*,#26186,.F.);
#33846=ORIENTED_EDGE('',*,*,#26187,.F.);
#33847=ORIENTED_EDGE('',*,*,#26188,.F.);
#33848=ORIENTED_EDGE('',*,*,#26189,.F.);
#33849=ORIENTED_EDGE('',*,*,#26190,.F.);
#33850=ORIENTED_EDGE('',*,*,#26191,.F.);
#33851=ORIENTED_EDGE('',*,*,#26192,.F.);
#33852=ORIENTED_EDGE('',*,*,#26193,.F.);
#33853=ORIENTED_EDGE('',*,*,#26194,.F.);
#33854=ORIENTED_EDGE('',*,*,#26195,.F.);
#33855=ORIENTED_EDGE('',*,*,#26196,.F.);
#33856=ORIENTED_EDGE('',*,*,#26197,.F.);
#33857=ORIENTED_EDGE('',*,*,#26198,.F.);
#33858=ORIENTED_EDGE('',*,*,#26199,.F.);
#33859=ORIENTED_EDGE('',*,*,#26200,.T.);
#33860=ORIENTED_EDGE('',*,*,#26201,.F.);
#33861=ORIENTED_EDGE('',*,*,#26202,.F.);
#33862=ORIENTED_EDGE('',*,*,#26203,.F.);
#33863=ORIENTED_EDGE('',*,*,#26204,.F.);
#33864=ORIENTED_EDGE('',*,*,#26205,.F.);
#33865=ORIENTED_EDGE('',*,*,#26206,.F.);
#33866=ORIENTED_EDGE('',*,*,#26207,.F.);
#33867=ORIENTED_EDGE('',*,*,#26208,.F.);
#33868=ORIENTED_EDGE('',*,*,#26209,.F.);
#33869=ORIENTED_EDGE('',*,*,#26210,.F.);
#33870=ORIENTED_EDGE('',*,*,#26211,.F.);
#33871=ORIENTED_EDGE('',*,*,#26212,.F.);
#33872=ORIENTED_EDGE('',*,*,#26213,.F.);
#33873=ORIENTED_EDGE('',*,*,#26214,.F.);
#33874=ORIENTED_EDGE('',*,*,#26215,.F.);
#33875=ORIENTED_EDGE('',*,*,#25382,.T.);
#33876=ORIENTED_EDGE('',*,*,#26216,.T.);
#33877=ORIENTED_EDGE('',*,*,#26217,.T.);
#33878=ORIENTED_EDGE('',*,*,#26218,.F.);
#33879=ORIENTED_EDGE('',*,*,#26219,.F.);
#33880=ORIENTED_EDGE('',*,*,#26220,.F.);
#33881=ORIENTED_EDGE('',*,*,#26185,.T.);
#33882=ORIENTED_EDGE('',*,*,#25379,.T.);
#33883=ORIENTED_EDGE('',*,*,#26221,.F.);
#33884=ORIENTED_EDGE('',*,*,#26222,.F.);
#33885=ORIENTED_EDGE('',*,*,#26223,.F.);
#33886=ORIENTED_EDGE('',*,*,#26224,.F.);
#33887=ORIENTED_EDGE('',*,*,#26225,.F.);
#33888=ORIENTED_EDGE('',*,*,#26226,.F.);
#33889=ORIENTED_EDGE('',*,*,#26227,.F.);
#33890=ORIENTED_EDGE('',*,*,#26228,.F.);
#33891=ORIENTED_EDGE('',*,*,#26229,.F.);
#33892=ORIENTED_EDGE('',*,*,#26230,.F.);
#33893=ORIENTED_EDGE('',*,*,#26231,.F.);
#33894=ORIENTED_EDGE('',*,*,#26232,.F.);
#33895=ORIENTED_EDGE('',*,*,#26233,.F.);
#33896=ORIENTED_EDGE('',*,*,#26234,.F.);
#33897=ORIENTED_EDGE('',*,*,#26235,.F.);
#33898=ORIENTED_EDGE('',*,*,#26236,.T.);
#33899=ORIENTED_EDGE('',*,*,#26237,.F.);
#33900=ORIENTED_EDGE('',*,*,#26238,.F.);
#33901=ORIENTED_EDGE('',*,*,#26239,.F.);
#33902=ORIENTED_EDGE('',*,*,#26240,.F.);
#33903=ORIENTED_EDGE('',*,*,#26241,.F.);
#33904=ORIENTED_EDGE('',*,*,#26242,.F.);
#33905=ORIENTED_EDGE('',*,*,#26243,.F.);
#33906=ORIENTED_EDGE('',*,*,#26244,.F.);
#33907=ORIENTED_EDGE('',*,*,#26245,.F.);
#33908=ORIENTED_EDGE('',*,*,#26246,.F.);
#33909=ORIENTED_EDGE('',*,*,#26247,.F.);
#33910=ORIENTED_EDGE('',*,*,#26248,.F.);
#33911=ORIENTED_EDGE('',*,*,#26249,.F.);
#33912=ORIENTED_EDGE('',*,*,#26250,.F.);
#33913=ORIENTED_EDGE('',*,*,#26251,.F.);
#33914=ORIENTED_EDGE('',*,*,#25378,.T.);
#33915=ORIENTED_EDGE('',*,*,#26252,.T.);
#33916=ORIENTED_EDGE('',*,*,#26253,.T.);
#33917=ORIENTED_EDGE('',*,*,#26254,.F.);
#33918=ORIENTED_EDGE('',*,*,#26255,.F.);
#33919=ORIENTED_EDGE('',*,*,#26256,.F.);
#33920=ORIENTED_EDGE('',*,*,#26221,.T.);
#33921=ORIENTED_EDGE('',*,*,#25375,.T.);
#33922=ORIENTED_EDGE('',*,*,#26257,.F.);
#33923=ORIENTED_EDGE('',*,*,#26258,.F.);
#33924=ORIENTED_EDGE('',*,*,#26259,.F.);
#33925=ORIENTED_EDGE('',*,*,#26260,.F.);
#33926=ORIENTED_EDGE('',*,*,#26261,.F.);
#33927=ORIENTED_EDGE('',*,*,#26262,.F.);
#33928=ORIENTED_EDGE('',*,*,#26263,.F.);
#33929=ORIENTED_EDGE('',*,*,#26264,.F.);
#33930=ORIENTED_EDGE('',*,*,#26265,.F.);
#33931=ORIENTED_EDGE('',*,*,#26266,.F.);
#33932=ORIENTED_EDGE('',*,*,#26267,.F.);
#33933=ORIENTED_EDGE('',*,*,#26268,.F.);
#33934=ORIENTED_EDGE('',*,*,#26269,.F.);
#33935=ORIENTED_EDGE('',*,*,#26270,.F.);
#33936=ORIENTED_EDGE('',*,*,#26271,.F.);
#33937=ORIENTED_EDGE('',*,*,#26272,.T.);
#33938=ORIENTED_EDGE('',*,*,#26273,.F.);
#33939=ORIENTED_EDGE('',*,*,#26274,.F.);
#33940=ORIENTED_EDGE('',*,*,#26275,.F.);
#33941=ORIENTED_EDGE('',*,*,#26276,.F.);
#33942=ORIENTED_EDGE('',*,*,#26277,.F.);
#33943=ORIENTED_EDGE('',*,*,#26278,.F.);
#33944=ORIENTED_EDGE('',*,*,#26279,.F.);
#33945=ORIENTED_EDGE('',*,*,#26280,.F.);
#33946=ORIENTED_EDGE('',*,*,#26281,.F.);
#33947=ORIENTED_EDGE('',*,*,#26282,.F.);
#33948=ORIENTED_EDGE('',*,*,#26283,.F.);
#33949=ORIENTED_EDGE('',*,*,#26284,.F.);
#33950=ORIENTED_EDGE('',*,*,#26285,.F.);
#33951=ORIENTED_EDGE('',*,*,#26286,.F.);
#33952=ORIENTED_EDGE('',*,*,#26287,.F.);
#33953=ORIENTED_EDGE('',*,*,#25374,.T.);
#33954=ORIENTED_EDGE('',*,*,#26288,.T.);
#33955=ORIENTED_EDGE('',*,*,#26289,.T.);
#33956=ORIENTED_EDGE('',*,*,#26290,.F.);
#33957=ORIENTED_EDGE('',*,*,#26291,.F.);
#33958=ORIENTED_EDGE('',*,*,#26292,.F.);
#33959=ORIENTED_EDGE('',*,*,#26257,.T.);
#33960=ORIENTED_EDGE('',*,*,#25371,.T.);
#33961=ORIENTED_EDGE('',*,*,#26293,.F.);
#33962=ORIENTED_EDGE('',*,*,#26294,.F.);
#33963=ORIENTED_EDGE('',*,*,#26295,.F.);
#33964=ORIENTED_EDGE('',*,*,#26296,.F.);
#33965=ORIENTED_EDGE('',*,*,#26297,.F.);
#33966=ORIENTED_EDGE('',*,*,#26298,.F.);
#33967=ORIENTED_EDGE('',*,*,#26299,.F.);
#33968=ORIENTED_EDGE('',*,*,#26300,.F.);
#33969=ORIENTED_EDGE('',*,*,#26301,.F.);
#33970=ORIENTED_EDGE('',*,*,#26302,.F.);
#33971=ORIENTED_EDGE('',*,*,#26303,.F.);
#33972=ORIENTED_EDGE('',*,*,#26304,.F.);
#33973=ORIENTED_EDGE('',*,*,#26305,.F.);
#33974=ORIENTED_EDGE('',*,*,#26306,.F.);
#33975=ORIENTED_EDGE('',*,*,#26307,.F.);
#33976=ORIENTED_EDGE('',*,*,#26308,.T.);
#33977=ORIENTED_EDGE('',*,*,#26309,.F.);
#33978=ORIENTED_EDGE('',*,*,#26310,.F.);
#33979=ORIENTED_EDGE('',*,*,#26311,.F.);
#33980=ORIENTED_EDGE('',*,*,#26312,.F.);
#33981=ORIENTED_EDGE('',*,*,#26313,.F.);
#33982=ORIENTED_EDGE('',*,*,#26314,.F.);
#33983=ORIENTED_EDGE('',*,*,#26315,.F.);
#33984=ORIENTED_EDGE('',*,*,#26316,.F.);
#33985=ORIENTED_EDGE('',*,*,#26317,.F.);
#33986=ORIENTED_EDGE('',*,*,#26318,.F.);
#33987=ORIENTED_EDGE('',*,*,#26319,.F.);
#33988=ORIENTED_EDGE('',*,*,#26320,.F.);
#33989=ORIENTED_EDGE('',*,*,#26321,.F.);
#33990=ORIENTED_EDGE('',*,*,#26322,.F.);
#33991=ORIENTED_EDGE('',*,*,#26323,.F.);
#33992=ORIENTED_EDGE('',*,*,#25370,.T.);
#33993=ORIENTED_EDGE('',*,*,#26324,.T.);
#33994=ORIENTED_EDGE('',*,*,#26325,.T.);
#33995=ORIENTED_EDGE('',*,*,#26326,.F.);
#33996=ORIENTED_EDGE('',*,*,#26327,.F.);
#33997=ORIENTED_EDGE('',*,*,#26328,.F.);
#33998=ORIENTED_EDGE('',*,*,#26293,.T.);
#33999=ORIENTED_EDGE('',*,*,#25367,.T.);
#34000=ORIENTED_EDGE('',*,*,#26329,.F.);
#34001=ORIENTED_EDGE('',*,*,#26330,.F.);
#34002=ORIENTED_EDGE('',*,*,#26331,.F.);
#34003=ORIENTED_EDGE('',*,*,#26332,.F.);
#34004=ORIENTED_EDGE('',*,*,#26333,.F.);
#34005=ORIENTED_EDGE('',*,*,#26334,.F.);
#34006=ORIENTED_EDGE('',*,*,#26335,.F.);
#34007=ORIENTED_EDGE('',*,*,#26336,.F.);
#34008=ORIENTED_EDGE('',*,*,#26337,.F.);
#34009=ORIENTED_EDGE('',*,*,#26338,.F.);
#34010=ORIENTED_EDGE('',*,*,#26339,.F.);
#34011=ORIENTED_EDGE('',*,*,#26340,.F.);
#34012=ORIENTED_EDGE('',*,*,#26341,.F.);
#34013=ORIENTED_EDGE('',*,*,#26342,.F.);
#34014=ORIENTED_EDGE('',*,*,#26343,.F.);
#34015=ORIENTED_EDGE('',*,*,#26344,.T.);
#34016=ORIENTED_EDGE('',*,*,#26345,.F.);
#34017=ORIENTED_EDGE('',*,*,#26346,.F.);
#34018=ORIENTED_EDGE('',*,*,#26347,.F.);
#34019=ORIENTED_EDGE('',*,*,#26348,.F.);
#34020=ORIENTED_EDGE('',*,*,#26349,.F.);
#34021=ORIENTED_EDGE('',*,*,#26350,.F.);
#34022=ORIENTED_EDGE('',*,*,#26351,.F.);
#34023=ORIENTED_EDGE('',*,*,#26352,.F.);
#34024=ORIENTED_EDGE('',*,*,#26353,.F.);
#34025=ORIENTED_EDGE('',*,*,#26354,.F.);
#34026=ORIENTED_EDGE('',*,*,#26355,.F.);
#34027=ORIENTED_EDGE('',*,*,#26356,.F.);
#34028=ORIENTED_EDGE('',*,*,#26357,.F.);
#34029=ORIENTED_EDGE('',*,*,#26358,.F.);
#34030=ORIENTED_EDGE('',*,*,#26359,.F.);
#34031=ORIENTED_EDGE('',*,*,#25366,.T.);
#34032=ORIENTED_EDGE('',*,*,#26360,.T.);
#34033=ORIENTED_EDGE('',*,*,#26361,.T.);
#34034=ORIENTED_EDGE('',*,*,#26362,.F.);
#34035=ORIENTED_EDGE('',*,*,#26363,.F.);
#34036=ORIENTED_EDGE('',*,*,#26364,.F.);
#34037=ORIENTED_EDGE('',*,*,#26329,.T.);
#34038=ORIENTED_EDGE('',*,*,#25363,.T.);
#34039=ORIENTED_EDGE('',*,*,#26365,.F.);
#34040=ORIENTED_EDGE('',*,*,#26366,.F.);
#34041=ORIENTED_EDGE('',*,*,#26367,.F.);
#34042=ORIENTED_EDGE('',*,*,#26368,.F.);
#34043=ORIENTED_EDGE('',*,*,#26369,.F.);
#34044=ORIENTED_EDGE('',*,*,#26370,.F.);
#34045=ORIENTED_EDGE('',*,*,#26371,.F.);
#34046=ORIENTED_EDGE('',*,*,#26372,.F.);
#34047=ORIENTED_EDGE('',*,*,#26373,.F.);
#34048=ORIENTED_EDGE('',*,*,#26374,.F.);
#34049=ORIENTED_EDGE('',*,*,#26375,.F.);
#34050=ORIENTED_EDGE('',*,*,#26376,.F.);
#34051=ORIENTED_EDGE('',*,*,#26377,.F.);
#34052=ORIENTED_EDGE('',*,*,#26378,.F.);
#34053=ORIENTED_EDGE('',*,*,#26379,.F.);
#34054=ORIENTED_EDGE('',*,*,#26380,.T.);
#34055=ORIENTED_EDGE('',*,*,#26381,.F.);
#34056=ORIENTED_EDGE('',*,*,#26382,.F.);
#34057=ORIENTED_EDGE('',*,*,#26383,.F.);
#34058=ORIENTED_EDGE('',*,*,#26384,.F.);
#34059=ORIENTED_EDGE('',*,*,#26385,.F.);
#34060=ORIENTED_EDGE('',*,*,#26386,.F.);
#34061=ORIENTED_EDGE('',*,*,#26387,.F.);
#34062=ORIENTED_EDGE('',*,*,#26388,.F.);
#34063=ORIENTED_EDGE('',*,*,#26389,.F.);
#34064=ORIENTED_EDGE('',*,*,#26390,.F.);
#34065=ORIENTED_EDGE('',*,*,#26391,.F.);
#34066=ORIENTED_EDGE('',*,*,#26392,.F.);
#34067=ORIENTED_EDGE('',*,*,#26393,.F.);
#34068=ORIENTED_EDGE('',*,*,#26394,.F.);
#34069=ORIENTED_EDGE('',*,*,#26395,.F.);
#34070=ORIENTED_EDGE('',*,*,#25362,.T.);
#34071=ORIENTED_EDGE('',*,*,#26396,.T.);
#34072=ORIENTED_EDGE('',*,*,#26397,.T.);
#34073=ORIENTED_EDGE('',*,*,#26398,.F.);
#34074=ORIENTED_EDGE('',*,*,#26399,.F.);
#34075=ORIENTED_EDGE('',*,*,#26400,.F.);
#34076=ORIENTED_EDGE('',*,*,#26365,.T.);
#34077=ORIENTED_EDGE('',*,*,#25359,.T.);
#34078=ORIENTED_EDGE('',*,*,#26401,.F.);
#34079=ORIENTED_EDGE('',*,*,#26402,.F.);
#34080=ORIENTED_EDGE('',*,*,#26403,.F.);
#34081=ORIENTED_EDGE('',*,*,#26404,.F.);
#34082=ORIENTED_EDGE('',*,*,#26405,.F.);
#34083=ORIENTED_EDGE('',*,*,#26406,.F.);
#34084=ORIENTED_EDGE('',*,*,#26407,.F.);
#34085=ORIENTED_EDGE('',*,*,#26408,.F.);
#34086=ORIENTED_EDGE('',*,*,#26409,.F.);
#34087=ORIENTED_EDGE('',*,*,#26410,.F.);
#34088=ORIENTED_EDGE('',*,*,#26411,.F.);
#34089=ORIENTED_EDGE('',*,*,#26412,.F.);
#34090=ORIENTED_EDGE('',*,*,#26413,.F.);
#34091=ORIENTED_EDGE('',*,*,#26414,.F.);
#34092=ORIENTED_EDGE('',*,*,#26415,.F.);
#34093=ORIENTED_EDGE('',*,*,#26416,.T.);
#34094=ORIENTED_EDGE('',*,*,#26417,.F.);
#34095=ORIENTED_EDGE('',*,*,#26418,.F.);
#34096=ORIENTED_EDGE('',*,*,#26419,.F.);
#34097=ORIENTED_EDGE('',*,*,#26420,.F.);
#34098=ORIENTED_EDGE('',*,*,#26421,.F.);
#34099=ORIENTED_EDGE('',*,*,#26422,.F.);
#34100=ORIENTED_EDGE('',*,*,#26423,.F.);
#34101=ORIENTED_EDGE('',*,*,#26424,.F.);
#34102=ORIENTED_EDGE('',*,*,#26425,.F.);
#34103=ORIENTED_EDGE('',*,*,#26426,.F.);
#34104=ORIENTED_EDGE('',*,*,#26427,.F.);
#34105=ORIENTED_EDGE('',*,*,#26428,.F.);
#34106=ORIENTED_EDGE('',*,*,#26429,.F.);
#34107=ORIENTED_EDGE('',*,*,#26430,.F.);
#34108=ORIENTED_EDGE('',*,*,#26431,.F.);
#34109=ORIENTED_EDGE('',*,*,#25358,.T.);
#34110=ORIENTED_EDGE('',*,*,#26432,.T.);
#34111=ORIENTED_EDGE('',*,*,#26433,.T.);
#34112=ORIENTED_EDGE('',*,*,#26434,.F.);
#34113=ORIENTED_EDGE('',*,*,#26435,.F.);
#34114=ORIENTED_EDGE('',*,*,#26436,.F.);
#34115=ORIENTED_EDGE('',*,*,#26401,.T.);
#34116=ORIENTED_EDGE('',*,*,#25355,.T.);
#34117=ORIENTED_EDGE('',*,*,#26437,.F.);
#34118=ORIENTED_EDGE('',*,*,#26438,.F.);
#34119=ORIENTED_EDGE('',*,*,#26439,.F.);
#34120=ORIENTED_EDGE('',*,*,#26440,.F.);
#34121=ORIENTED_EDGE('',*,*,#26441,.F.);
#34122=ORIENTED_EDGE('',*,*,#26442,.F.);
#34123=ORIENTED_EDGE('',*,*,#26443,.F.);
#34124=ORIENTED_EDGE('',*,*,#26444,.F.);
#34125=ORIENTED_EDGE('',*,*,#26445,.F.);
#34126=ORIENTED_EDGE('',*,*,#26446,.F.);
#34127=ORIENTED_EDGE('',*,*,#26447,.F.);
#34128=ORIENTED_EDGE('',*,*,#26448,.F.);
#34129=ORIENTED_EDGE('',*,*,#26449,.F.);
#34130=ORIENTED_EDGE('',*,*,#26450,.F.);
#34131=ORIENTED_EDGE('',*,*,#26451,.F.);
#34132=ORIENTED_EDGE('',*,*,#26452,.T.);
#34133=ORIENTED_EDGE('',*,*,#26453,.F.);
#34134=ORIENTED_EDGE('',*,*,#26454,.F.);
#34135=ORIENTED_EDGE('',*,*,#26455,.F.);
#34136=ORIENTED_EDGE('',*,*,#26456,.F.);
#34137=ORIENTED_EDGE('',*,*,#26457,.F.);
#34138=ORIENTED_EDGE('',*,*,#26458,.F.);
#34139=ORIENTED_EDGE('',*,*,#26459,.F.);
#34140=ORIENTED_EDGE('',*,*,#26460,.F.);
#34141=ORIENTED_EDGE('',*,*,#26461,.F.);
#34142=ORIENTED_EDGE('',*,*,#26462,.F.);
#34143=ORIENTED_EDGE('',*,*,#26463,.F.);
#34144=ORIENTED_EDGE('',*,*,#26464,.F.);
#34145=ORIENTED_EDGE('',*,*,#26465,.F.);
#34146=ORIENTED_EDGE('',*,*,#26466,.F.);
#34147=ORIENTED_EDGE('',*,*,#26467,.F.);
#34148=ORIENTED_EDGE('',*,*,#25354,.T.);
#34149=ORIENTED_EDGE('',*,*,#26468,.T.);
#34150=ORIENTED_EDGE('',*,*,#26469,.T.);
#34151=ORIENTED_EDGE('',*,*,#26470,.F.);
#34152=ORIENTED_EDGE('',*,*,#26471,.F.);
#34153=ORIENTED_EDGE('',*,*,#26472,.F.);
#34154=ORIENTED_EDGE('',*,*,#26437,.T.);
#34155=ORIENTED_EDGE('',*,*,#25351,.T.);
#34156=ORIENTED_EDGE('',*,*,#26473,.F.);
#34157=ORIENTED_EDGE('',*,*,#26474,.F.);
#34158=ORIENTED_EDGE('',*,*,#26475,.F.);
#34159=ORIENTED_EDGE('',*,*,#26476,.F.);
#34160=ORIENTED_EDGE('',*,*,#26477,.F.);
#34161=ORIENTED_EDGE('',*,*,#26478,.F.);
#34162=ORIENTED_EDGE('',*,*,#26479,.F.);
#34163=ORIENTED_EDGE('',*,*,#26480,.F.);
#34164=ORIENTED_EDGE('',*,*,#26481,.F.);
#34165=ORIENTED_EDGE('',*,*,#26482,.F.);
#34166=ORIENTED_EDGE('',*,*,#26483,.F.);
#34167=ORIENTED_EDGE('',*,*,#26484,.F.);
#34168=ORIENTED_EDGE('',*,*,#26485,.F.);
#34169=ORIENTED_EDGE('',*,*,#26486,.F.);
#34170=ORIENTED_EDGE('',*,*,#26487,.F.);
#34171=ORIENTED_EDGE('',*,*,#26488,.T.);
#34172=ORIENTED_EDGE('',*,*,#26489,.F.);
#34173=ORIENTED_EDGE('',*,*,#26490,.F.);
#34174=ORIENTED_EDGE('',*,*,#26491,.F.);
#34175=ORIENTED_EDGE('',*,*,#26492,.F.);
#34176=ORIENTED_EDGE('',*,*,#26493,.F.);
#34177=ORIENTED_EDGE('',*,*,#26494,.F.);
#34178=ORIENTED_EDGE('',*,*,#26495,.F.);
#34179=ORIENTED_EDGE('',*,*,#26496,.F.);
#34180=ORIENTED_EDGE('',*,*,#26497,.F.);
#34181=ORIENTED_EDGE('',*,*,#26498,.F.);
#34182=ORIENTED_EDGE('',*,*,#26499,.F.);
#34183=ORIENTED_EDGE('',*,*,#26500,.F.);
#34184=ORIENTED_EDGE('',*,*,#26501,.F.);
#34185=ORIENTED_EDGE('',*,*,#26502,.F.);
#34186=ORIENTED_EDGE('',*,*,#26503,.F.);
#34187=ORIENTED_EDGE('',*,*,#25350,.T.);
#34188=ORIENTED_EDGE('',*,*,#26504,.T.);
#34189=ORIENTED_EDGE('',*,*,#26505,.T.);
#34190=ORIENTED_EDGE('',*,*,#26506,.F.);
#34191=ORIENTED_EDGE('',*,*,#26507,.F.);
#34192=ORIENTED_EDGE('',*,*,#26508,.F.);
#34193=ORIENTED_EDGE('',*,*,#26473,.T.);
#34194=ORIENTED_EDGE('',*,*,#25347,.T.);
#34195=ORIENTED_EDGE('',*,*,#26509,.F.);
#34196=ORIENTED_EDGE('',*,*,#26510,.F.);
#34197=ORIENTED_EDGE('',*,*,#26511,.F.);
#34198=ORIENTED_EDGE('',*,*,#26512,.F.);
#34199=ORIENTED_EDGE('',*,*,#26513,.F.);
#34200=ORIENTED_EDGE('',*,*,#26514,.F.);
#34201=ORIENTED_EDGE('',*,*,#26515,.F.);
#34202=ORIENTED_EDGE('',*,*,#26516,.F.);
#34203=ORIENTED_EDGE('',*,*,#26517,.F.);
#34204=ORIENTED_EDGE('',*,*,#26518,.F.);
#34205=ORIENTED_EDGE('',*,*,#26519,.F.);
#34206=ORIENTED_EDGE('',*,*,#26520,.F.);
#34207=ORIENTED_EDGE('',*,*,#26521,.F.);
#34208=ORIENTED_EDGE('',*,*,#26522,.F.);
#34209=ORIENTED_EDGE('',*,*,#26523,.F.);
#34210=ORIENTED_EDGE('',*,*,#26524,.T.);
#34211=ORIENTED_EDGE('',*,*,#26525,.F.);
#34212=ORIENTED_EDGE('',*,*,#26526,.F.);
#34213=ORIENTED_EDGE('',*,*,#26527,.F.);
#34214=ORIENTED_EDGE('',*,*,#26528,.F.);
#34215=ORIENTED_EDGE('',*,*,#26529,.F.);
#34216=ORIENTED_EDGE('',*,*,#26530,.F.);
#34217=ORIENTED_EDGE('',*,*,#26531,.F.);
#34218=ORIENTED_EDGE('',*,*,#26532,.F.);
#34219=ORIENTED_EDGE('',*,*,#26533,.F.);
#34220=ORIENTED_EDGE('',*,*,#26534,.F.);
#34221=ORIENTED_EDGE('',*,*,#26535,.F.);
#34222=ORIENTED_EDGE('',*,*,#26536,.F.);
#34223=ORIENTED_EDGE('',*,*,#26537,.F.);
#34224=ORIENTED_EDGE('',*,*,#26538,.F.);
#34225=ORIENTED_EDGE('',*,*,#26539,.F.);
#34226=ORIENTED_EDGE('',*,*,#25346,.T.);
#34227=ORIENTED_EDGE('',*,*,#26540,.T.);
#34228=ORIENTED_EDGE('',*,*,#26541,.T.);
#34229=ORIENTED_EDGE('',*,*,#26542,.F.);
#34230=ORIENTED_EDGE('',*,*,#26543,.F.);
#34231=ORIENTED_EDGE('',*,*,#26544,.F.);
#34232=ORIENTED_EDGE('',*,*,#26509,.T.);
#34233=ORIENTED_EDGE('',*,*,#25343,.T.);
#34234=ORIENTED_EDGE('',*,*,#26545,.F.);
#34235=ORIENTED_EDGE('',*,*,#26546,.F.);
#34236=ORIENTED_EDGE('',*,*,#26547,.F.);
#34237=ORIENTED_EDGE('',*,*,#26548,.F.);
#34238=ORIENTED_EDGE('',*,*,#26549,.F.);
#34239=ORIENTED_EDGE('',*,*,#26550,.F.);
#34240=ORIENTED_EDGE('',*,*,#26551,.F.);
#34241=ORIENTED_EDGE('',*,*,#26552,.F.);
#34242=ORIENTED_EDGE('',*,*,#26553,.F.);
#34243=ORIENTED_EDGE('',*,*,#26554,.F.);
#34244=ORIENTED_EDGE('',*,*,#26555,.F.);
#34245=ORIENTED_EDGE('',*,*,#26556,.F.);
#34246=ORIENTED_EDGE('',*,*,#26557,.F.);
#34247=ORIENTED_EDGE('',*,*,#26558,.F.);
#34248=ORIENTED_EDGE('',*,*,#26559,.F.);
#34249=ORIENTED_EDGE('',*,*,#26560,.T.);
#34250=ORIENTED_EDGE('',*,*,#26561,.F.);
#34251=ORIENTED_EDGE('',*,*,#26562,.F.);
#34252=ORIENTED_EDGE('',*,*,#26563,.F.);
#34253=ORIENTED_EDGE('',*,*,#26564,.F.);
#34254=ORIENTED_EDGE('',*,*,#26565,.F.);
#34255=ORIENTED_EDGE('',*,*,#26566,.F.);
#34256=ORIENTED_EDGE('',*,*,#26567,.F.);
#34257=ORIENTED_EDGE('',*,*,#26568,.F.);
#34258=ORIENTED_EDGE('',*,*,#26569,.F.);
#34259=ORIENTED_EDGE('',*,*,#26570,.F.);
#34260=ORIENTED_EDGE('',*,*,#26571,.F.);
#34261=ORIENTED_EDGE('',*,*,#26572,.F.);
#34262=ORIENTED_EDGE('',*,*,#26573,.F.);
#34263=ORIENTED_EDGE('',*,*,#26574,.F.);
#34264=ORIENTED_EDGE('',*,*,#26575,.F.);
#34265=ORIENTED_EDGE('',*,*,#25342,.T.);
#34266=ORIENTED_EDGE('',*,*,#26576,.T.);
#34267=ORIENTED_EDGE('',*,*,#26577,.T.);
#34268=ORIENTED_EDGE('',*,*,#26578,.F.);
#34269=ORIENTED_EDGE('',*,*,#26579,.F.);
#34270=ORIENTED_EDGE('',*,*,#26580,.F.);
#34271=ORIENTED_EDGE('',*,*,#26545,.T.);
#34272=ORIENTED_EDGE('',*,*,#25339,.T.);
#34273=ORIENTED_EDGE('',*,*,#26581,.F.);
#34274=ORIENTED_EDGE('',*,*,#26582,.F.);
#34275=ORIENTED_EDGE('',*,*,#26583,.F.);
#34276=ORIENTED_EDGE('',*,*,#26584,.F.);
#34277=ORIENTED_EDGE('',*,*,#26585,.F.);
#34278=ORIENTED_EDGE('',*,*,#26586,.F.);
#34279=ORIENTED_EDGE('',*,*,#26587,.F.);
#34280=ORIENTED_EDGE('',*,*,#26588,.F.);
#34281=ORIENTED_EDGE('',*,*,#26589,.F.);
#34282=ORIENTED_EDGE('',*,*,#26590,.F.);
#34283=ORIENTED_EDGE('',*,*,#26591,.F.);
#34284=ORIENTED_EDGE('',*,*,#26592,.F.);
#34285=ORIENTED_EDGE('',*,*,#26593,.F.);
#34286=ORIENTED_EDGE('',*,*,#26594,.F.);
#34287=ORIENTED_EDGE('',*,*,#26595,.F.);
#34288=ORIENTED_EDGE('',*,*,#26596,.T.);
#34289=ORIENTED_EDGE('',*,*,#26597,.F.);
#34290=ORIENTED_EDGE('',*,*,#26598,.F.);
#34291=ORIENTED_EDGE('',*,*,#26599,.F.);
#34292=ORIENTED_EDGE('',*,*,#26600,.F.);
#34293=ORIENTED_EDGE('',*,*,#26601,.F.);
#34294=ORIENTED_EDGE('',*,*,#26602,.F.);
#34295=ORIENTED_EDGE('',*,*,#26603,.F.);
#34296=ORIENTED_EDGE('',*,*,#26604,.F.);
#34297=ORIENTED_EDGE('',*,*,#26605,.F.);
#34298=ORIENTED_EDGE('',*,*,#26606,.F.);
#34299=ORIENTED_EDGE('',*,*,#26607,.F.);
#34300=ORIENTED_EDGE('',*,*,#26608,.F.);
#34301=ORIENTED_EDGE('',*,*,#26609,.F.);
#34302=ORIENTED_EDGE('',*,*,#26610,.F.);
#34303=ORIENTED_EDGE('',*,*,#26611,.F.);
#34304=ORIENTED_EDGE('',*,*,#25338,.T.);
#34305=ORIENTED_EDGE('',*,*,#26612,.T.);
#34306=ORIENTED_EDGE('',*,*,#26613,.T.);
#34307=ORIENTED_EDGE('',*,*,#26614,.F.);
#34308=ORIENTED_EDGE('',*,*,#26615,.F.);
#34309=ORIENTED_EDGE('',*,*,#26616,.F.);
#34310=ORIENTED_EDGE('',*,*,#26581,.T.);
#34311=ORIENTED_EDGE('',*,*,#25335,.T.);
#34312=ORIENTED_EDGE('',*,*,#26617,.F.);
#34313=ORIENTED_EDGE('',*,*,#26618,.F.);
#34314=ORIENTED_EDGE('',*,*,#26619,.F.);
#34315=ORIENTED_EDGE('',*,*,#26620,.F.);
#34316=ORIENTED_EDGE('',*,*,#26621,.F.);
#34317=ORIENTED_EDGE('',*,*,#26622,.F.);
#34318=ORIENTED_EDGE('',*,*,#26623,.F.);
#34319=ORIENTED_EDGE('',*,*,#26624,.F.);
#34320=ORIENTED_EDGE('',*,*,#26625,.F.);
#34321=ORIENTED_EDGE('',*,*,#26626,.F.);
#34322=ORIENTED_EDGE('',*,*,#26627,.F.);
#34323=ORIENTED_EDGE('',*,*,#26628,.F.);
#34324=ORIENTED_EDGE('',*,*,#26629,.F.);
#34325=ORIENTED_EDGE('',*,*,#26630,.F.);
#34326=ORIENTED_EDGE('',*,*,#26631,.F.);
#34327=ORIENTED_EDGE('',*,*,#26632,.T.);
#34328=ORIENTED_EDGE('',*,*,#26633,.F.);
#34329=ORIENTED_EDGE('',*,*,#26634,.F.);
#34330=ORIENTED_EDGE('',*,*,#26635,.F.);
#34331=ORIENTED_EDGE('',*,*,#26636,.F.);
#34332=ORIENTED_EDGE('',*,*,#26637,.F.);
#34333=ORIENTED_EDGE('',*,*,#26638,.F.);
#34334=ORIENTED_EDGE('',*,*,#26639,.F.);
#34335=ORIENTED_EDGE('',*,*,#26640,.F.);
#34336=ORIENTED_EDGE('',*,*,#26641,.F.);
#34337=ORIENTED_EDGE('',*,*,#26642,.F.);
#34338=ORIENTED_EDGE('',*,*,#26643,.F.);
#34339=ORIENTED_EDGE('',*,*,#26644,.F.);
#34340=ORIENTED_EDGE('',*,*,#26645,.F.);
#34341=ORIENTED_EDGE('',*,*,#26646,.F.);
#34342=ORIENTED_EDGE('',*,*,#26647,.F.);
#34343=ORIENTED_EDGE('',*,*,#25334,.T.);
#34344=ORIENTED_EDGE('',*,*,#26648,.T.);
#34345=ORIENTED_EDGE('',*,*,#26649,.T.);
#34346=ORIENTED_EDGE('',*,*,#26650,.F.);
#34347=ORIENTED_EDGE('',*,*,#26651,.F.);
#34348=ORIENTED_EDGE('',*,*,#26652,.F.);
#34349=ORIENTED_EDGE('',*,*,#26617,.T.);
#34350=ORIENTED_EDGE('',*,*,#25331,.T.);
#34351=ORIENTED_EDGE('',*,*,#26653,.F.);
#34352=ORIENTED_EDGE('',*,*,#26654,.F.);
#34353=ORIENTED_EDGE('',*,*,#26655,.F.);
#34354=ORIENTED_EDGE('',*,*,#26656,.F.);
#34355=ORIENTED_EDGE('',*,*,#26657,.F.);
#34356=ORIENTED_EDGE('',*,*,#26658,.F.);
#34357=ORIENTED_EDGE('',*,*,#26659,.F.);
#34358=ORIENTED_EDGE('',*,*,#26660,.F.);
#34359=ORIENTED_EDGE('',*,*,#26661,.F.);
#34360=ORIENTED_EDGE('',*,*,#26662,.F.);
#34361=ORIENTED_EDGE('',*,*,#26663,.F.);
#34362=ORIENTED_EDGE('',*,*,#26664,.F.);
#34363=ORIENTED_EDGE('',*,*,#26665,.F.);
#34364=ORIENTED_EDGE('',*,*,#26666,.F.);
#34365=ORIENTED_EDGE('',*,*,#26667,.F.);
#34366=ORIENTED_EDGE('',*,*,#26668,.T.);
#34367=ORIENTED_EDGE('',*,*,#26669,.F.);
#34368=ORIENTED_EDGE('',*,*,#26670,.F.);
#34369=ORIENTED_EDGE('',*,*,#26671,.F.);
#34370=ORIENTED_EDGE('',*,*,#26672,.F.);
#34371=ORIENTED_EDGE('',*,*,#26673,.F.);
#34372=ORIENTED_EDGE('',*,*,#26674,.F.);
#34373=ORIENTED_EDGE('',*,*,#26675,.F.);
#34374=ORIENTED_EDGE('',*,*,#26676,.F.);
#34375=ORIENTED_EDGE('',*,*,#26677,.F.);
#34376=ORIENTED_EDGE('',*,*,#26678,.F.);
#34377=ORIENTED_EDGE('',*,*,#26679,.F.);
#34378=ORIENTED_EDGE('',*,*,#26680,.F.);
#34379=ORIENTED_EDGE('',*,*,#26681,.F.);
#34380=ORIENTED_EDGE('',*,*,#26682,.F.);
#34381=ORIENTED_EDGE('',*,*,#26683,.F.);
#34382=ORIENTED_EDGE('',*,*,#25330,.T.);
#34383=ORIENTED_EDGE('',*,*,#26684,.T.);
#34384=ORIENTED_EDGE('',*,*,#26685,.T.);
#34385=ORIENTED_EDGE('',*,*,#26686,.F.);
#34386=ORIENTED_EDGE('',*,*,#26687,.F.);
#34387=ORIENTED_EDGE('',*,*,#26688,.F.);
#34388=ORIENTED_EDGE('',*,*,#26653,.T.);
#34389=ORIENTED_EDGE('',*,*,#25327,.T.);
#34390=ORIENTED_EDGE('',*,*,#26689,.F.);
#34391=ORIENTED_EDGE('',*,*,#26690,.F.);
#34392=ORIENTED_EDGE('',*,*,#26691,.F.);
#34393=ORIENTED_EDGE('',*,*,#26692,.F.);
#34394=ORIENTED_EDGE('',*,*,#26693,.F.);
#34395=ORIENTED_EDGE('',*,*,#26694,.F.);
#34396=ORIENTED_EDGE('',*,*,#26695,.F.);
#34397=ORIENTED_EDGE('',*,*,#26696,.F.);
#34398=ORIENTED_EDGE('',*,*,#26697,.F.);
#34399=ORIENTED_EDGE('',*,*,#26698,.F.);
#34400=ORIENTED_EDGE('',*,*,#26699,.F.);
#34401=ORIENTED_EDGE('',*,*,#26700,.F.);
#34402=ORIENTED_EDGE('',*,*,#26701,.F.);
#34403=ORIENTED_EDGE('',*,*,#26702,.F.);
#34404=ORIENTED_EDGE('',*,*,#26703,.F.);
#34405=ORIENTED_EDGE('',*,*,#26704,.T.);
#34406=ORIENTED_EDGE('',*,*,#26705,.F.);
#34407=ORIENTED_EDGE('',*,*,#26706,.F.);
#34408=ORIENTED_EDGE('',*,*,#26707,.F.);
#34409=ORIENTED_EDGE('',*,*,#26708,.F.);
#34410=ORIENTED_EDGE('',*,*,#26709,.F.);
#34411=ORIENTED_EDGE('',*,*,#26710,.F.);
#34412=ORIENTED_EDGE('',*,*,#26711,.F.);
#34413=ORIENTED_EDGE('',*,*,#26712,.F.);
#34414=ORIENTED_EDGE('',*,*,#26713,.F.);
#34415=ORIENTED_EDGE('',*,*,#26714,.F.);
#34416=ORIENTED_EDGE('',*,*,#26715,.F.);
#34417=ORIENTED_EDGE('',*,*,#26716,.F.);
#34418=ORIENTED_EDGE('',*,*,#26717,.F.);
#34419=ORIENTED_EDGE('',*,*,#26718,.F.);
#34420=ORIENTED_EDGE('',*,*,#26719,.F.);
#34421=ORIENTED_EDGE('',*,*,#25326,.T.);
#34422=ORIENTED_EDGE('',*,*,#26720,.T.);
#34423=ORIENTED_EDGE('',*,*,#26721,.T.);
#34424=ORIENTED_EDGE('',*,*,#26722,.F.);
#34425=ORIENTED_EDGE('',*,*,#26723,.F.);
#34426=ORIENTED_EDGE('',*,*,#26724,.F.);
#34427=ORIENTED_EDGE('',*,*,#26689,.T.);
#34428=ORIENTED_EDGE('',*,*,#25323,.T.);
#34429=ORIENTED_EDGE('',*,*,#26725,.F.);
#34430=ORIENTED_EDGE('',*,*,#26726,.F.);
#34431=ORIENTED_EDGE('',*,*,#26727,.F.);
#34432=ORIENTED_EDGE('',*,*,#26728,.F.);
#34433=ORIENTED_EDGE('',*,*,#26729,.F.);
#34434=ORIENTED_EDGE('',*,*,#26730,.F.);
#34435=ORIENTED_EDGE('',*,*,#26731,.F.);
#34436=ORIENTED_EDGE('',*,*,#26732,.F.);
#34437=ORIENTED_EDGE('',*,*,#26733,.F.);
#34438=ORIENTED_EDGE('',*,*,#26734,.F.);
#34439=ORIENTED_EDGE('',*,*,#26735,.F.);
#34440=ORIENTED_EDGE('',*,*,#26736,.F.);
#34441=ORIENTED_EDGE('',*,*,#26737,.F.);
#34442=ORIENTED_EDGE('',*,*,#26738,.F.);
#34443=ORIENTED_EDGE('',*,*,#26739,.F.);
#34444=ORIENTED_EDGE('',*,*,#26740,.T.);
#34445=ORIENTED_EDGE('',*,*,#26741,.F.);
#34446=ORIENTED_EDGE('',*,*,#26742,.F.);
#34447=ORIENTED_EDGE('',*,*,#26743,.F.);
#34448=ORIENTED_EDGE('',*,*,#26744,.F.);
#34449=ORIENTED_EDGE('',*,*,#26745,.F.);
#34450=ORIENTED_EDGE('',*,*,#26746,.F.);
#34451=ORIENTED_EDGE('',*,*,#26747,.F.);
#34452=ORIENTED_EDGE('',*,*,#26748,.F.);
#34453=ORIENTED_EDGE('',*,*,#26749,.F.);
#34454=ORIENTED_EDGE('',*,*,#26750,.F.);
#34455=ORIENTED_EDGE('',*,*,#26751,.F.);
#34456=ORIENTED_EDGE('',*,*,#26752,.F.);
#34457=ORIENTED_EDGE('',*,*,#26753,.F.);
#34458=ORIENTED_EDGE('',*,*,#26754,.F.);
#34459=ORIENTED_EDGE('',*,*,#26755,.F.);
#34460=ORIENTED_EDGE('',*,*,#25322,.T.);
#34461=ORIENTED_EDGE('',*,*,#26756,.T.);
#34462=ORIENTED_EDGE('',*,*,#26757,.T.);
#34463=ORIENTED_EDGE('',*,*,#26758,.F.);
#34464=ORIENTED_EDGE('',*,*,#26759,.F.);
#34465=ORIENTED_EDGE('',*,*,#26760,.F.);
#34466=ORIENTED_EDGE('',*,*,#26725,.T.);
#34467=ORIENTED_EDGE('',*,*,#26761,.F.);
#34468=ORIENTED_EDGE('',*,*,#26762,.F.);
#34469=ORIENTED_EDGE('',*,*,#26740,.F.);
#34470=ORIENTED_EDGE('',*,*,#26763,.F.);
#34471=ORIENTED_EDGE('',*,*,#26764,.F.);
#34472=ORIENTED_EDGE('',*,*,#26765,.F.);
#34473=ORIENTED_EDGE('',*,*,#26704,.F.);
#34474=ORIENTED_EDGE('',*,*,#26766,.F.);
#34475=ORIENTED_EDGE('',*,*,#26767,.F.);
#34476=ORIENTED_EDGE('',*,*,#26768,.F.);
#34477=ORIENTED_EDGE('',*,*,#26668,.F.);
#34478=ORIENTED_EDGE('',*,*,#26769,.F.);
#34479=ORIENTED_EDGE('',*,*,#26770,.F.);
#34480=ORIENTED_EDGE('',*,*,#26771,.F.);
#34481=ORIENTED_EDGE('',*,*,#26632,.F.);
#34482=ORIENTED_EDGE('',*,*,#26772,.F.);
#34483=ORIENTED_EDGE('',*,*,#26773,.F.);
#34484=ORIENTED_EDGE('',*,*,#26774,.F.);
#34485=ORIENTED_EDGE('',*,*,#26596,.F.);
#34486=ORIENTED_EDGE('',*,*,#26775,.F.);
#34487=ORIENTED_EDGE('',*,*,#26776,.F.);
#34488=ORIENTED_EDGE('',*,*,#26777,.F.);
#34489=ORIENTED_EDGE('',*,*,#26560,.F.);
#34490=ORIENTED_EDGE('',*,*,#26778,.F.);
#34491=ORIENTED_EDGE('',*,*,#26779,.F.);
#34492=ORIENTED_EDGE('',*,*,#26780,.F.);
#34493=ORIENTED_EDGE('',*,*,#26524,.F.);
#34494=ORIENTED_EDGE('',*,*,#26781,.F.);
#34495=ORIENTED_EDGE('',*,*,#26782,.F.);
#34496=ORIENTED_EDGE('',*,*,#26783,.F.);
#34497=ORIENTED_EDGE('',*,*,#26488,.F.);
#34498=ORIENTED_EDGE('',*,*,#26784,.F.);
#34499=ORIENTED_EDGE('',*,*,#26785,.F.);
#34500=ORIENTED_EDGE('',*,*,#26786,.F.);
#34501=ORIENTED_EDGE('',*,*,#26452,.F.);
#34502=ORIENTED_EDGE('',*,*,#26787,.F.);
#34503=ORIENTED_EDGE('',*,*,#26788,.F.);
#34504=ORIENTED_EDGE('',*,*,#26789,.F.);
#34505=ORIENTED_EDGE('',*,*,#26416,.F.);
#34506=ORIENTED_EDGE('',*,*,#26790,.F.);
#34507=ORIENTED_EDGE('',*,*,#26791,.F.);
#34508=ORIENTED_EDGE('',*,*,#26792,.F.);
#34509=ORIENTED_EDGE('',*,*,#26380,.F.);
#34510=ORIENTED_EDGE('',*,*,#26793,.F.);
#34511=ORIENTED_EDGE('',*,*,#26794,.F.);
#34512=ORIENTED_EDGE('',*,*,#26795,.F.);
#34513=ORIENTED_EDGE('',*,*,#26344,.F.);
#34514=ORIENTED_EDGE('',*,*,#26796,.F.);
#34515=ORIENTED_EDGE('',*,*,#26797,.F.);
#34516=ORIENTED_EDGE('',*,*,#26798,.F.);
#34517=ORIENTED_EDGE('',*,*,#26308,.F.);
#34518=ORIENTED_EDGE('',*,*,#26799,.F.);
#34519=ORIENTED_EDGE('',*,*,#26800,.F.);
#34520=ORIENTED_EDGE('',*,*,#26801,.F.);
#34521=ORIENTED_EDGE('',*,*,#26272,.F.);
#34522=ORIENTED_EDGE('',*,*,#26802,.F.);
#34523=ORIENTED_EDGE('',*,*,#26803,.F.);
#34524=ORIENTED_EDGE('',*,*,#26804,.F.);
#34525=ORIENTED_EDGE('',*,*,#26236,.F.);
#34526=ORIENTED_EDGE('',*,*,#26805,.F.);
#34527=ORIENTED_EDGE('',*,*,#26806,.F.);
#34528=ORIENTED_EDGE('',*,*,#26807,.F.);
#34529=ORIENTED_EDGE('',*,*,#26200,.F.);
#34530=ORIENTED_EDGE('',*,*,#26808,.F.);
#34531=ORIENTED_EDGE('',*,*,#26809,.F.);
#34532=ORIENTED_EDGE('',*,*,#26810,.F.);
#34533=ORIENTED_EDGE('',*,*,#26164,.F.);
#34534=ORIENTED_EDGE('',*,*,#26811,.F.);
#34535=ORIENTED_EDGE('',*,*,#26812,.F.);
#34536=ORIENTED_EDGE('',*,*,#26813,.F.);
#34537=ORIENTED_EDGE('',*,*,#26128,.F.);
#34538=ORIENTED_EDGE('',*,*,#26814,.F.);
#34539=ORIENTED_EDGE('',*,*,#26815,.F.);
#34540=ORIENTED_EDGE('',*,*,#26816,.F.);
#34541=ORIENTED_EDGE('',*,*,#26092,.F.);
#34542=ORIENTED_EDGE('',*,*,#26817,.F.);
#34543=ORIENTED_EDGE('',*,*,#26818,.F.);
#34544=ORIENTED_EDGE('',*,*,#26819,.F.);
#34545=ORIENTED_EDGE('',*,*,#26056,.F.);
#34546=ORIENTED_EDGE('',*,*,#26820,.F.);
#34547=ORIENTED_EDGE('',*,*,#26821,.F.);
#34548=ORIENTED_EDGE('',*,*,#26822,.F.);
#34549=ORIENTED_EDGE('',*,*,#26020,.F.);
#34550=ORIENTED_EDGE('',*,*,#26823,.F.);
#34551=ORIENTED_EDGE('',*,*,#26824,.F.);
#34552=ORIENTED_EDGE('',*,*,#26825,.F.);
#34553=ORIENTED_EDGE('',*,*,#25984,.F.);
#34554=ORIENTED_EDGE('',*,*,#26826,.F.);
#34555=ORIENTED_EDGE('',*,*,#26827,.F.);
#34556=ORIENTED_EDGE('',*,*,#26828,.F.);
#34557=ORIENTED_EDGE('',*,*,#25948,.F.);
#34558=ORIENTED_EDGE('',*,*,#26829,.F.);
#34559=ORIENTED_EDGE('',*,*,#26830,.F.);
#34560=ORIENTED_EDGE('',*,*,#26831,.F.);
#34561=ORIENTED_EDGE('',*,*,#25912,.F.);
#34562=ORIENTED_EDGE('',*,*,#26832,.F.);
#34563=ORIENTED_EDGE('',*,*,#26833,.F.);
#34564=ORIENTED_EDGE('',*,*,#26834,.F.);
#34565=ORIENTED_EDGE('',*,*,#25876,.F.);
#34566=ORIENTED_EDGE('',*,*,#26835,.F.);
#34567=ORIENTED_EDGE('',*,*,#26836,.F.);
#34568=ORIENTED_EDGE('',*,*,#26837,.F.);
#34569=ORIENTED_EDGE('',*,*,#25840,.F.);
#34570=ORIENTED_EDGE('',*,*,#26838,.F.);
#34571=ORIENTED_EDGE('',*,*,#26839,.F.);
#34572=ORIENTED_EDGE('',*,*,#26840,.F.);
#34573=ORIENTED_EDGE('',*,*,#25804,.F.);
#34574=ORIENTED_EDGE('',*,*,#26841,.F.);
#34575=ORIENTED_EDGE('',*,*,#26842,.F.);
#34576=ORIENTED_EDGE('',*,*,#26843,.F.);
#34577=ORIENTED_EDGE('',*,*,#25768,.F.);
#34578=ORIENTED_EDGE('',*,*,#26844,.F.);
#34579=ORIENTED_EDGE('',*,*,#26845,.F.);
#34580=ORIENTED_EDGE('',*,*,#26846,.F.);
#34581=ORIENTED_EDGE('',*,*,#25732,.F.);
#34582=ORIENTED_EDGE('',*,*,#26847,.F.);
#34583=ORIENTED_EDGE('',*,*,#26848,.F.);
#34584=ORIENTED_EDGE('',*,*,#26849,.F.);
#34585=ORIENTED_EDGE('',*,*,#25696,.F.);
#34586=ORIENTED_EDGE('',*,*,#26850,.F.);
#34587=ORIENTED_EDGE('',*,*,#26851,.F.);
#34588=ORIENTED_EDGE('',*,*,#26852,.F.);
#34589=ORIENTED_EDGE('',*,*,#25660,.F.);
#34590=ORIENTED_EDGE('',*,*,#26853,.F.);
#34591=ORIENTED_EDGE('',*,*,#26854,.F.);
#34592=ORIENTED_EDGE('',*,*,#26855,.F.);
#34593=ORIENTED_EDGE('',*,*,#25624,.F.);
#34594=ORIENTED_EDGE('',*,*,#26856,.F.);
#34595=ORIENTED_EDGE('',*,*,#26857,.F.);
#34596=ORIENTED_EDGE('',*,*,#26858,.F.);
#34597=ORIENTED_EDGE('',*,*,#25588,.F.);
#34598=ORIENTED_EDGE('',*,*,#26859,.F.);
#34599=ORIENTED_EDGE('',*,*,#26860,.F.);
#34600=ORIENTED_EDGE('',*,*,#26861,.F.);
#34601=ORIENTED_EDGE('',*,*,#25552,.F.);
#34602=ORIENTED_EDGE('',*,*,#26862,.F.);
#34603=ORIENTED_EDGE('',*,*,#26863,.F.);
#34604=ORIENTED_EDGE('',*,*,#26864,.F.);
#34605=ORIENTED_EDGE('',*,*,#25516,.F.);
#34606=ORIENTED_EDGE('',*,*,#26865,.F.);
#34607=ORIENTED_EDGE('',*,*,#26866,.F.);
#34608=ORIENTED_EDGE('',*,*,#26867,.F.);
#34609=ORIENTED_EDGE('',*,*,#25480,.F.);
#34610=ORIENTED_EDGE('',*,*,#26868,.F.);
#34611=ORIENTED_EDGE('',*,*,#26867,.T.);
#34612=ORIENTED_EDGE('',*,*,#26869,.T.);
#34613=ORIENTED_EDGE('',*,*,#26870,.T.);
#34614=ORIENTED_EDGE('',*,*,#26871,.F.);
#34615=ORIENTED_EDGE('',*,*,#26872,.F.);
#34616=ORIENTED_EDGE('',*,*,#26873,.F.);
#34617=ORIENTED_EDGE('',*,*,#25481,.T.);
#34618=ORIENTED_EDGE('',*,*,#26864,.T.);
#34619=ORIENTED_EDGE('',*,*,#26874,.T.);
#34620=ORIENTED_EDGE('',*,*,#26875,.T.);
#34621=ORIENTED_EDGE('',*,*,#26876,.F.);
#34622=ORIENTED_EDGE('',*,*,#26877,.F.);
#34623=ORIENTED_EDGE('',*,*,#26878,.F.);
#34624=ORIENTED_EDGE('',*,*,#25517,.T.);
#34625=ORIENTED_EDGE('',*,*,#26861,.T.);
#34626=ORIENTED_EDGE('',*,*,#26879,.T.);
#34627=ORIENTED_EDGE('',*,*,#26880,.T.);
#34628=ORIENTED_EDGE('',*,*,#26881,.F.);
#34629=ORIENTED_EDGE('',*,*,#26882,.F.);
#34630=ORIENTED_EDGE('',*,*,#26883,.F.);
#34631=ORIENTED_EDGE('',*,*,#25553,.T.);
#34632=ORIENTED_EDGE('',*,*,#26858,.T.);
#34633=ORIENTED_EDGE('',*,*,#26884,.T.);
#34634=ORIENTED_EDGE('',*,*,#26885,.T.);
#34635=ORIENTED_EDGE('',*,*,#26886,.F.);
#34636=ORIENTED_EDGE('',*,*,#26887,.F.);
#34637=ORIENTED_EDGE('',*,*,#26888,.F.);
#34638=ORIENTED_EDGE('',*,*,#25589,.T.);
#34639=ORIENTED_EDGE('',*,*,#26855,.T.);
#34640=ORIENTED_EDGE('',*,*,#26889,.T.);
#34641=ORIENTED_EDGE('',*,*,#26890,.T.);
#34642=ORIENTED_EDGE('',*,*,#26891,.F.);
#34643=ORIENTED_EDGE('',*,*,#26892,.F.);
#34644=ORIENTED_EDGE('',*,*,#26893,.F.);
#34645=ORIENTED_EDGE('',*,*,#25625,.T.);
#34646=ORIENTED_EDGE('',*,*,#26852,.T.);
#34647=ORIENTED_EDGE('',*,*,#26894,.T.);
#34648=ORIENTED_EDGE('',*,*,#26895,.T.);
#34649=ORIENTED_EDGE('',*,*,#26896,.F.);
#34650=ORIENTED_EDGE('',*,*,#26897,.F.);
#34651=ORIENTED_EDGE('',*,*,#26898,.F.);
#34652=ORIENTED_EDGE('',*,*,#25661,.T.);
#34653=ORIENTED_EDGE('',*,*,#26849,.T.);
#34654=ORIENTED_EDGE('',*,*,#26899,.T.);
#34655=ORIENTED_EDGE('',*,*,#26900,.T.);
#34656=ORIENTED_EDGE('',*,*,#26901,.F.);
#34657=ORIENTED_EDGE('',*,*,#26902,.F.);
#34658=ORIENTED_EDGE('',*,*,#26903,.F.);
#34659=ORIENTED_EDGE('',*,*,#25697,.T.);
#34660=ORIENTED_EDGE('',*,*,#26846,.T.);
#34661=ORIENTED_EDGE('',*,*,#26904,.T.);
#34662=ORIENTED_EDGE('',*,*,#26905,.T.);
#34663=ORIENTED_EDGE('',*,*,#26906,.F.);
#34664=ORIENTED_EDGE('',*,*,#26907,.F.);
#34665=ORIENTED_EDGE('',*,*,#26908,.F.);
#34666=ORIENTED_EDGE('',*,*,#25733,.T.);
#34667=ORIENTED_EDGE('',*,*,#26843,.T.);
#34668=ORIENTED_EDGE('',*,*,#26909,.T.);
#34669=ORIENTED_EDGE('',*,*,#26910,.T.);
#34670=ORIENTED_EDGE('',*,*,#26911,.F.);
#34671=ORIENTED_EDGE('',*,*,#26912,.F.);
#34672=ORIENTED_EDGE('',*,*,#26913,.F.);
#34673=ORIENTED_EDGE('',*,*,#25769,.T.);
#34674=ORIENTED_EDGE('',*,*,#26840,.T.);
#34675=ORIENTED_EDGE('',*,*,#26914,.T.);
#34676=ORIENTED_EDGE('',*,*,#26915,.T.);
#34677=ORIENTED_EDGE('',*,*,#26916,.F.);
#34678=ORIENTED_EDGE('',*,*,#26917,.F.);
#34679=ORIENTED_EDGE('',*,*,#26918,.F.);
#34680=ORIENTED_EDGE('',*,*,#25805,.T.);
#34681=ORIENTED_EDGE('',*,*,#26837,.T.);
#34682=ORIENTED_EDGE('',*,*,#26919,.T.);
#34683=ORIENTED_EDGE('',*,*,#26920,.T.);
#34684=ORIENTED_EDGE('',*,*,#26921,.F.);
#34685=ORIENTED_EDGE('',*,*,#26922,.F.);
#34686=ORIENTED_EDGE('',*,*,#26923,.F.);
#34687=ORIENTED_EDGE('',*,*,#25841,.T.);
#34688=ORIENTED_EDGE('',*,*,#26834,.T.);
#34689=ORIENTED_EDGE('',*,*,#26924,.T.);
#34690=ORIENTED_EDGE('',*,*,#26925,.T.);
#34691=ORIENTED_EDGE('',*,*,#26926,.F.);
#34692=ORIENTED_EDGE('',*,*,#26927,.F.);
#34693=ORIENTED_EDGE('',*,*,#26928,.F.);
#34694=ORIENTED_EDGE('',*,*,#25877,.T.);
#34695=ORIENTED_EDGE('',*,*,#26831,.T.);
#34696=ORIENTED_EDGE('',*,*,#26929,.T.);
#34697=ORIENTED_EDGE('',*,*,#26930,.T.);
#34698=ORIENTED_EDGE('',*,*,#26931,.F.);
#34699=ORIENTED_EDGE('',*,*,#26932,.F.);
#34700=ORIENTED_EDGE('',*,*,#26933,.F.);
#34701=ORIENTED_EDGE('',*,*,#25913,.T.);
#34702=ORIENTED_EDGE('',*,*,#26828,.T.);
#34703=ORIENTED_EDGE('',*,*,#26934,.T.);
#34704=ORIENTED_EDGE('',*,*,#26935,.T.);
#34705=ORIENTED_EDGE('',*,*,#26936,.F.);
#34706=ORIENTED_EDGE('',*,*,#26937,.F.);
#34707=ORIENTED_EDGE('',*,*,#26938,.F.);
#34708=ORIENTED_EDGE('',*,*,#25949,.T.);
#34709=ORIENTED_EDGE('',*,*,#26825,.T.);
#34710=ORIENTED_EDGE('',*,*,#26939,.T.);
#34711=ORIENTED_EDGE('',*,*,#26940,.T.);
#34712=ORIENTED_EDGE('',*,*,#26941,.F.);
#34713=ORIENTED_EDGE('',*,*,#26942,.F.);
#34714=ORIENTED_EDGE('',*,*,#26943,.F.);
#34715=ORIENTED_EDGE('',*,*,#25985,.T.);
#34716=ORIENTED_EDGE('',*,*,#26822,.T.);
#34717=ORIENTED_EDGE('',*,*,#26944,.T.);
#34718=ORIENTED_EDGE('',*,*,#26945,.T.);
#34719=ORIENTED_EDGE('',*,*,#26946,.F.);
#34720=ORIENTED_EDGE('',*,*,#26947,.F.);
#34721=ORIENTED_EDGE('',*,*,#26948,.F.);
#34722=ORIENTED_EDGE('',*,*,#26021,.T.);
#34723=ORIENTED_EDGE('',*,*,#26819,.T.);
#34724=ORIENTED_EDGE('',*,*,#26949,.T.);
#34725=ORIENTED_EDGE('',*,*,#26950,.T.);
#34726=ORIENTED_EDGE('',*,*,#26951,.F.);
#34727=ORIENTED_EDGE('',*,*,#26952,.F.);
#34728=ORIENTED_EDGE('',*,*,#26953,.F.);
#34729=ORIENTED_EDGE('',*,*,#26057,.T.);
#34730=ORIENTED_EDGE('',*,*,#26816,.T.);
#34731=ORIENTED_EDGE('',*,*,#26954,.T.);
#34732=ORIENTED_EDGE('',*,*,#26955,.T.);
#34733=ORIENTED_EDGE('',*,*,#26956,.F.);
#34734=ORIENTED_EDGE('',*,*,#26957,.F.);
#34735=ORIENTED_EDGE('',*,*,#26958,.F.);
#34736=ORIENTED_EDGE('',*,*,#26093,.T.);
#34737=ORIENTED_EDGE('',*,*,#26813,.T.);
#34738=ORIENTED_EDGE('',*,*,#26959,.T.);
#34739=ORIENTED_EDGE('',*,*,#26960,.T.);
#34740=ORIENTED_EDGE('',*,*,#26961,.F.);
#34741=ORIENTED_EDGE('',*,*,#26962,.F.);
#34742=ORIENTED_EDGE('',*,*,#26963,.F.);
#34743=ORIENTED_EDGE('',*,*,#26129,.T.);
#34744=ORIENTED_EDGE('',*,*,#26810,.T.);
#34745=ORIENTED_EDGE('',*,*,#26964,.T.);
#34746=ORIENTED_EDGE('',*,*,#26965,.T.);
#34747=ORIENTED_EDGE('',*,*,#26966,.F.);
#34748=ORIENTED_EDGE('',*,*,#26967,.F.);
#34749=ORIENTED_EDGE('',*,*,#26968,.F.);
#34750=ORIENTED_EDGE('',*,*,#26165,.T.);
#34751=ORIENTED_EDGE('',*,*,#26807,.T.);
#34752=ORIENTED_EDGE('',*,*,#26969,.T.);
#34753=ORIENTED_EDGE('',*,*,#26970,.T.);
#34754=ORIENTED_EDGE('',*,*,#26971,.F.);
#34755=ORIENTED_EDGE('',*,*,#26972,.F.);
#34756=ORIENTED_EDGE('',*,*,#26973,.F.);
#34757=ORIENTED_EDGE('',*,*,#26201,.T.);
#34758=ORIENTED_EDGE('',*,*,#26804,.T.);
#34759=ORIENTED_EDGE('',*,*,#26974,.T.);
#34760=ORIENTED_EDGE('',*,*,#26975,.T.);
#34761=ORIENTED_EDGE('',*,*,#26976,.F.);
#34762=ORIENTED_EDGE('',*,*,#26977,.F.);
#34763=ORIENTED_EDGE('',*,*,#26978,.F.);
#34764=ORIENTED_EDGE('',*,*,#26237,.T.);
#34765=ORIENTED_EDGE('',*,*,#26801,.T.);
#34766=ORIENTED_EDGE('',*,*,#26979,.T.);
#34767=ORIENTED_EDGE('',*,*,#26980,.T.);
#34768=ORIENTED_EDGE('',*,*,#26981,.F.);
#34769=ORIENTED_EDGE('',*,*,#26982,.F.);
#34770=ORIENTED_EDGE('',*,*,#26983,.F.);
#34771=ORIENTED_EDGE('',*,*,#26273,.T.);
#34772=ORIENTED_EDGE('',*,*,#26798,.T.);
#34773=ORIENTED_EDGE('',*,*,#26984,.T.);
#34774=ORIENTED_EDGE('',*,*,#26985,.T.);
#34775=ORIENTED_EDGE('',*,*,#26986,.F.);
#34776=ORIENTED_EDGE('',*,*,#26987,.F.);
#34777=ORIENTED_EDGE('',*,*,#26988,.F.);
#34778=ORIENTED_EDGE('',*,*,#26309,.T.);
#34779=ORIENTED_EDGE('',*,*,#26795,.T.);
#34780=ORIENTED_EDGE('',*,*,#26989,.T.);
#34781=ORIENTED_EDGE('',*,*,#26990,.T.);
#34782=ORIENTED_EDGE('',*,*,#26991,.F.);
#34783=ORIENTED_EDGE('',*,*,#26992,.F.);
#34784=ORIENTED_EDGE('',*,*,#26993,.F.);
#34785=ORIENTED_EDGE('',*,*,#26345,.T.);
#34786=ORIENTED_EDGE('',*,*,#26792,.T.);
#34787=ORIENTED_EDGE('',*,*,#26994,.T.);
#34788=ORIENTED_EDGE('',*,*,#26995,.T.);
#34789=ORIENTED_EDGE('',*,*,#26996,.F.);
#34790=ORIENTED_EDGE('',*,*,#26997,.F.);
#34791=ORIENTED_EDGE('',*,*,#26998,.F.);
#34792=ORIENTED_EDGE('',*,*,#26381,.T.);
#34793=ORIENTED_EDGE('',*,*,#26789,.T.);
#34794=ORIENTED_EDGE('',*,*,#26999,.T.);
#34795=ORIENTED_EDGE('',*,*,#27000,.T.);
#34796=ORIENTED_EDGE('',*,*,#27001,.F.);
#34797=ORIENTED_EDGE('',*,*,#27002,.F.);
#34798=ORIENTED_EDGE('',*,*,#27003,.F.);
#34799=ORIENTED_EDGE('',*,*,#26417,.T.);
#34800=ORIENTED_EDGE('',*,*,#26786,.T.);
#34801=ORIENTED_EDGE('',*,*,#27004,.T.);
#34802=ORIENTED_EDGE('',*,*,#27005,.T.);
#34803=ORIENTED_EDGE('',*,*,#27006,.F.);
#34804=ORIENTED_EDGE('',*,*,#27007,.F.);
#34805=ORIENTED_EDGE('',*,*,#27008,.F.);
#34806=ORIENTED_EDGE('',*,*,#26453,.T.);
#34807=ORIENTED_EDGE('',*,*,#26783,.T.);
#34808=ORIENTED_EDGE('',*,*,#27009,.T.);
#34809=ORIENTED_EDGE('',*,*,#27010,.T.);
#34810=ORIENTED_EDGE('',*,*,#27011,.F.);
#34811=ORIENTED_EDGE('',*,*,#27012,.F.);
#34812=ORIENTED_EDGE('',*,*,#27013,.F.);
#34813=ORIENTED_EDGE('',*,*,#26489,.T.);
#34814=ORIENTED_EDGE('',*,*,#26780,.T.);
#34815=ORIENTED_EDGE('',*,*,#27014,.T.);
#34816=ORIENTED_EDGE('',*,*,#27015,.T.);
#34817=ORIENTED_EDGE('',*,*,#27016,.F.);
#34818=ORIENTED_EDGE('',*,*,#27017,.F.);
#34819=ORIENTED_EDGE('',*,*,#27018,.F.);
#34820=ORIENTED_EDGE('',*,*,#26525,.T.);
#34821=ORIENTED_EDGE('',*,*,#26777,.T.);
#34822=ORIENTED_EDGE('',*,*,#27019,.T.);
#34823=ORIENTED_EDGE('',*,*,#27020,.T.);
#34824=ORIENTED_EDGE('',*,*,#27021,.F.);
#34825=ORIENTED_EDGE('',*,*,#27022,.F.);
#34826=ORIENTED_EDGE('',*,*,#27023,.F.);
#34827=ORIENTED_EDGE('',*,*,#26561,.T.);
#34828=ORIENTED_EDGE('',*,*,#26774,.T.);
#34829=ORIENTED_EDGE('',*,*,#27024,.T.);
#34830=ORIENTED_EDGE('',*,*,#27025,.T.);
#34831=ORIENTED_EDGE('',*,*,#27026,.F.);
#34832=ORIENTED_EDGE('',*,*,#27027,.F.);
#34833=ORIENTED_EDGE('',*,*,#27028,.F.);
#34834=ORIENTED_EDGE('',*,*,#26597,.T.);
#34835=ORIENTED_EDGE('',*,*,#26771,.T.);
#34836=ORIENTED_EDGE('',*,*,#27029,.T.);
#34837=ORIENTED_EDGE('',*,*,#27030,.T.);
#34838=ORIENTED_EDGE('',*,*,#27031,.F.);
#34839=ORIENTED_EDGE('',*,*,#27032,.F.);
#34840=ORIENTED_EDGE('',*,*,#27033,.F.);
#34841=ORIENTED_EDGE('',*,*,#26633,.T.);
#34842=ORIENTED_EDGE('',*,*,#26768,.T.);
#34843=ORIENTED_EDGE('',*,*,#27034,.T.);
#34844=ORIENTED_EDGE('',*,*,#27035,.T.);
#34845=ORIENTED_EDGE('',*,*,#27036,.F.);
#34846=ORIENTED_EDGE('',*,*,#27037,.F.);
#34847=ORIENTED_EDGE('',*,*,#27038,.F.);
#34848=ORIENTED_EDGE('',*,*,#26669,.T.);
#34849=ORIENTED_EDGE('',*,*,#26765,.T.);
#34850=ORIENTED_EDGE('',*,*,#27039,.T.);
#34851=ORIENTED_EDGE('',*,*,#27040,.T.);
#34852=ORIENTED_EDGE('',*,*,#27041,.F.);
#34853=ORIENTED_EDGE('',*,*,#27042,.F.);
#34854=ORIENTED_EDGE('',*,*,#27043,.F.);
#34855=ORIENTED_EDGE('',*,*,#26705,.T.);
#34856=ORIENTED_EDGE('',*,*,#26762,.T.);
#34857=ORIENTED_EDGE('',*,*,#27044,.T.);
#34858=ORIENTED_EDGE('',*,*,#27045,.T.);
#34859=ORIENTED_EDGE('',*,*,#27046,.F.);
#34860=ORIENTED_EDGE('',*,*,#27047,.F.);
#34861=ORIENTED_EDGE('',*,*,#27048,.F.);
#34862=ORIENTED_EDGE('',*,*,#26741,.T.);
#34863=ORIENTED_EDGE('',*,*,#25461,.T.);
#34864=ORIENTED_EDGE('',*,*,#27049,.F.);
#34865=ORIENTED_EDGE('',*,*,#27050,.F.);
#34866=ORIENTED_EDGE('',*,*,#25496,.F.);
#34867=ORIENTED_EDGE('',*,*,#25457,.T.);
#34868=ORIENTED_EDGE('',*,*,#27051,.F.);
#34869=ORIENTED_EDGE('',*,*,#27052,.F.);
#34870=ORIENTED_EDGE('',*,*,#25532,.F.);
#34871=ORIENTED_EDGE('',*,*,#25453,.T.);
#34872=ORIENTED_EDGE('',*,*,#27053,.F.);
#34873=ORIENTED_EDGE('',*,*,#27054,.F.);
#34874=ORIENTED_EDGE('',*,*,#25568,.F.);
#34875=ORIENTED_EDGE('',*,*,#25449,.T.);
#34876=ORIENTED_EDGE('',*,*,#27055,.F.);
#34877=ORIENTED_EDGE('',*,*,#27056,.F.);
#34878=ORIENTED_EDGE('',*,*,#25604,.F.);
#34879=ORIENTED_EDGE('',*,*,#25445,.T.);
#34880=ORIENTED_EDGE('',*,*,#27057,.F.);
#34881=ORIENTED_EDGE('',*,*,#27058,.F.);
#34882=ORIENTED_EDGE('',*,*,#25640,.F.);
#34883=ORIENTED_EDGE('',*,*,#25441,.T.);
#34884=ORIENTED_EDGE('',*,*,#27059,.F.);
#34885=ORIENTED_EDGE('',*,*,#27060,.F.);
#34886=ORIENTED_EDGE('',*,*,#25676,.F.);
#34887=ORIENTED_EDGE('',*,*,#25437,.T.);
#34888=ORIENTED_EDGE('',*,*,#27061,.F.);
#34889=ORIENTED_EDGE('',*,*,#27062,.F.);
#34890=ORIENTED_EDGE('',*,*,#25712,.F.);
#34891=ORIENTED_EDGE('',*,*,#25433,.T.);
#34892=ORIENTED_EDGE('',*,*,#27063,.F.);
#34893=ORIENTED_EDGE('',*,*,#27064,.F.);
#34894=ORIENTED_EDGE('',*,*,#25748,.F.);
#34895=ORIENTED_EDGE('',*,*,#25429,.T.);
#34896=ORIENTED_EDGE('',*,*,#27065,.F.);
#34897=ORIENTED_EDGE('',*,*,#27066,.F.);
#34898=ORIENTED_EDGE('',*,*,#25784,.F.);
#34899=ORIENTED_EDGE('',*,*,#25425,.T.);
#34900=ORIENTED_EDGE('',*,*,#27067,.F.);
#34901=ORIENTED_EDGE('',*,*,#27068,.F.);
#34902=ORIENTED_EDGE('',*,*,#25820,.F.);
#34903=ORIENTED_EDGE('',*,*,#25421,.T.);
#34904=ORIENTED_EDGE('',*,*,#27069,.F.);
#34905=ORIENTED_EDGE('',*,*,#27070,.F.);
#34906=ORIENTED_EDGE('',*,*,#25856,.F.);
#34907=ORIENTED_EDGE('',*,*,#25417,.T.);
#34908=ORIENTED_EDGE('',*,*,#27071,.F.);
#34909=ORIENTED_EDGE('',*,*,#27072,.F.);
#34910=ORIENTED_EDGE('',*,*,#25892,.F.);
#34911=ORIENTED_EDGE('',*,*,#25413,.T.);
#34912=ORIENTED_EDGE('',*,*,#27073,.F.);
#34913=ORIENTED_EDGE('',*,*,#27074,.F.);
#34914=ORIENTED_EDGE('',*,*,#25928,.F.);
#34915=ORIENTED_EDGE('',*,*,#25409,.T.);
#34916=ORIENTED_EDGE('',*,*,#27075,.F.);
#34917=ORIENTED_EDGE('',*,*,#27076,.F.);
#34918=ORIENTED_EDGE('',*,*,#25964,.F.);
#34919=ORIENTED_EDGE('',*,*,#25405,.T.);
#34920=ORIENTED_EDGE('',*,*,#27077,.F.);
#34921=ORIENTED_EDGE('',*,*,#27078,.F.);
#34922=ORIENTED_EDGE('',*,*,#26000,.F.);
#34923=ORIENTED_EDGE('',*,*,#25401,.T.);
#34924=ORIENTED_EDGE('',*,*,#27079,.F.);
#34925=ORIENTED_EDGE('',*,*,#27080,.F.);
#34926=ORIENTED_EDGE('',*,*,#26036,.F.);
#34927=ORIENTED_EDGE('',*,*,#25397,.T.);
#34928=ORIENTED_EDGE('',*,*,#27081,.F.);
#34929=ORIENTED_EDGE('',*,*,#27082,.F.);
#34930=ORIENTED_EDGE('',*,*,#26072,.F.);
#34931=ORIENTED_EDGE('',*,*,#25393,.T.);
#34932=ORIENTED_EDGE('',*,*,#27083,.F.);
#34933=ORIENTED_EDGE('',*,*,#27084,.F.);
#34934=ORIENTED_EDGE('',*,*,#26108,.F.);
#34935=ORIENTED_EDGE('',*,*,#25389,.T.);
#34936=ORIENTED_EDGE('',*,*,#27085,.F.);
#34937=ORIENTED_EDGE('',*,*,#27086,.F.);
#34938=ORIENTED_EDGE('',*,*,#26144,.F.);
#34939=ORIENTED_EDGE('',*,*,#25385,.T.);
#34940=ORIENTED_EDGE('',*,*,#27087,.F.);
#34941=ORIENTED_EDGE('',*,*,#27088,.F.);
#34942=ORIENTED_EDGE('',*,*,#26180,.F.);
#34943=ORIENTED_EDGE('',*,*,#25381,.T.);
#34944=ORIENTED_EDGE('',*,*,#27089,.F.);
#34945=ORIENTED_EDGE('',*,*,#27090,.F.);
#34946=ORIENTED_EDGE('',*,*,#26216,.F.);
#34947=ORIENTED_EDGE('',*,*,#25377,.T.);
#34948=ORIENTED_EDGE('',*,*,#27091,.F.);
#34949=ORIENTED_EDGE('',*,*,#27092,.F.);
#34950=ORIENTED_EDGE('',*,*,#26252,.F.);
#34951=ORIENTED_EDGE('',*,*,#25373,.T.);
#34952=ORIENTED_EDGE('',*,*,#27093,.F.);
#34953=ORIENTED_EDGE('',*,*,#27094,.F.);
#34954=ORIENTED_EDGE('',*,*,#26288,.F.);
#34955=ORIENTED_EDGE('',*,*,#25369,.T.);
#34956=ORIENTED_EDGE('',*,*,#27095,.F.);
#34957=ORIENTED_EDGE('',*,*,#27096,.F.);
#34958=ORIENTED_EDGE('',*,*,#26324,.F.);
#34959=ORIENTED_EDGE('',*,*,#25365,.T.);
#34960=ORIENTED_EDGE('',*,*,#27097,.F.);
#34961=ORIENTED_EDGE('',*,*,#27098,.F.);
#34962=ORIENTED_EDGE('',*,*,#26360,.F.);
#34963=ORIENTED_EDGE('',*,*,#25361,.T.);
#34964=ORIENTED_EDGE('',*,*,#27099,.F.);
#34965=ORIENTED_EDGE('',*,*,#27100,.F.);
#34966=ORIENTED_EDGE('',*,*,#26396,.F.);
#34967=ORIENTED_EDGE('',*,*,#25357,.T.);
#34968=ORIENTED_EDGE('',*,*,#27101,.F.);
#34969=ORIENTED_EDGE('',*,*,#27102,.F.);
#34970=ORIENTED_EDGE('',*,*,#26432,.F.);
#34971=ORIENTED_EDGE('',*,*,#25353,.T.);
#34972=ORIENTED_EDGE('',*,*,#27103,.F.);
#34973=ORIENTED_EDGE('',*,*,#27104,.F.);
#34974=ORIENTED_EDGE('',*,*,#26468,.F.);
#34975=ORIENTED_EDGE('',*,*,#25349,.T.);
#34976=ORIENTED_EDGE('',*,*,#27105,.F.);
#34977=ORIENTED_EDGE('',*,*,#27106,.F.);
#34978=ORIENTED_EDGE('',*,*,#26504,.F.);
#34979=ORIENTED_EDGE('',*,*,#25345,.T.);
#34980=ORIENTED_EDGE('',*,*,#27107,.F.);
#34981=ORIENTED_EDGE('',*,*,#27108,.F.);
#34982=ORIENTED_EDGE('',*,*,#26540,.F.);
#34983=ORIENTED_EDGE('',*,*,#25341,.T.);
#34984=ORIENTED_EDGE('',*,*,#27109,.F.);
#34985=ORIENTED_EDGE('',*,*,#27110,.F.);
#34986=ORIENTED_EDGE('',*,*,#26576,.F.);
#34987=ORIENTED_EDGE('',*,*,#25337,.T.);
#34988=ORIENTED_EDGE('',*,*,#27111,.F.);
#34989=ORIENTED_EDGE('',*,*,#27112,.F.);
#34990=ORIENTED_EDGE('',*,*,#26612,.F.);
#34991=ORIENTED_EDGE('',*,*,#25333,.T.);
#34992=ORIENTED_EDGE('',*,*,#27113,.F.);
#34993=ORIENTED_EDGE('',*,*,#27114,.F.);
#34994=ORIENTED_EDGE('',*,*,#26648,.F.);
#34995=ORIENTED_EDGE('',*,*,#25329,.T.);
#34996=ORIENTED_EDGE('',*,*,#27115,.F.);
#34997=ORIENTED_EDGE('',*,*,#27116,.F.);
#34998=ORIENTED_EDGE('',*,*,#26684,.F.);
#34999=ORIENTED_EDGE('',*,*,#25325,.T.);
#35000=ORIENTED_EDGE('',*,*,#27117,.F.);
#35001=ORIENTED_EDGE('',*,*,#27118,.F.);
#35002=ORIENTED_EDGE('',*,*,#26720,.F.);
#35003=ORIENTED_EDGE('',*,*,#25321,.T.);
#35004=ORIENTED_EDGE('',*,*,#27119,.F.);
#35005=ORIENTED_EDGE('',*,*,#27120,.F.);
#35006=ORIENTED_EDGE('',*,*,#26756,.F.);
#35007=ORIENTED_EDGE('',*,*,#25324,.T.);
#35008=ORIENTED_EDGE('',*,*,#26755,.T.);
#35009=ORIENTED_EDGE('',*,*,#27121,.T.);
#35010=ORIENTED_EDGE('',*,*,#27122,.F.);
#35011=ORIENTED_EDGE('',*,*,#27123,.F.);
#35012=ORIENTED_EDGE('',*,*,#27124,.T.);
#35013=ORIENTED_EDGE('',*,*,#27119,.T.);
#35014=ORIENTED_EDGE('',*,*,#25328,.T.);
#35015=ORIENTED_EDGE('',*,*,#26719,.T.);
#35016=ORIENTED_EDGE('',*,*,#27125,.T.);
#35017=ORIENTED_EDGE('',*,*,#27126,.F.);
#35018=ORIENTED_EDGE('',*,*,#27127,.F.);
#35019=ORIENTED_EDGE('',*,*,#27128,.T.);
#35020=ORIENTED_EDGE('',*,*,#27117,.T.);
#35021=ORIENTED_EDGE('',*,*,#25332,.T.);
#35022=ORIENTED_EDGE('',*,*,#26683,.T.);
#35023=ORIENTED_EDGE('',*,*,#27129,.T.);
#35024=ORIENTED_EDGE('',*,*,#27130,.F.);
#35025=ORIENTED_EDGE('',*,*,#27131,.F.);
#35026=ORIENTED_EDGE('',*,*,#27132,.T.);
#35027=ORIENTED_EDGE('',*,*,#27115,.T.);
#35028=ORIENTED_EDGE('',*,*,#25336,.T.);
#35029=ORIENTED_EDGE('',*,*,#26647,.T.);
#35030=ORIENTED_EDGE('',*,*,#27133,.T.);
#35031=ORIENTED_EDGE('',*,*,#27134,.F.);
#35032=ORIENTED_EDGE('',*,*,#27135,.F.);
#35033=ORIENTED_EDGE('',*,*,#27136,.T.);
#35034=ORIENTED_EDGE('',*,*,#27113,.T.);
#35035=ORIENTED_EDGE('',*,*,#25340,.T.);
#35036=ORIENTED_EDGE('',*,*,#26611,.T.);
#35037=ORIENTED_EDGE('',*,*,#27137,.T.);
#35038=ORIENTED_EDGE('',*,*,#27138,.F.);
#35039=ORIENTED_EDGE('',*,*,#27139,.F.);
#35040=ORIENTED_EDGE('',*,*,#27140,.T.);
#35041=ORIENTED_EDGE('',*,*,#27111,.T.);
#35042=ORIENTED_EDGE('',*,*,#25344,.T.);
#35043=ORIENTED_EDGE('',*,*,#26575,.T.);
#35044=ORIENTED_EDGE('',*,*,#27141,.T.);
#35045=ORIENTED_EDGE('',*,*,#27142,.F.);
#35046=ORIENTED_EDGE('',*,*,#27143,.F.);
#35047=ORIENTED_EDGE('',*,*,#27144,.T.);
#35048=ORIENTED_EDGE('',*,*,#27109,.T.);
#35049=ORIENTED_EDGE('',*,*,#25348,.T.);
#35050=ORIENTED_EDGE('',*,*,#26539,.T.);
#35051=ORIENTED_EDGE('',*,*,#27145,.T.);
#35052=ORIENTED_EDGE('',*,*,#27146,.F.);
#35053=ORIENTED_EDGE('',*,*,#27147,.F.);
#35054=ORIENTED_EDGE('',*,*,#27148,.T.);
#35055=ORIENTED_EDGE('',*,*,#27107,.T.);
#35056=ORIENTED_EDGE('',*,*,#25352,.T.);
#35057=ORIENTED_EDGE('',*,*,#26503,.T.);
#35058=ORIENTED_EDGE('',*,*,#27149,.T.);
#35059=ORIENTED_EDGE('',*,*,#27150,.F.);
#35060=ORIENTED_EDGE('',*,*,#27151,.F.);
#35061=ORIENTED_EDGE('',*,*,#27152,.T.);
#35062=ORIENTED_EDGE('',*,*,#27105,.T.);
#35063=ORIENTED_EDGE('',*,*,#25356,.T.);
#35064=ORIENTED_EDGE('',*,*,#26467,.T.);
#35065=ORIENTED_EDGE('',*,*,#27153,.T.);
#35066=ORIENTED_EDGE('',*,*,#27154,.F.);
#35067=ORIENTED_EDGE('',*,*,#27155,.F.);
#35068=ORIENTED_EDGE('',*,*,#27156,.T.);
#35069=ORIENTED_EDGE('',*,*,#27103,.T.);
#35070=ORIENTED_EDGE('',*,*,#25360,.T.);
#35071=ORIENTED_EDGE('',*,*,#26431,.T.);
#35072=ORIENTED_EDGE('',*,*,#27157,.T.);
#35073=ORIENTED_EDGE('',*,*,#27158,.F.);
#35074=ORIENTED_EDGE('',*,*,#27159,.F.);
#35075=ORIENTED_EDGE('',*,*,#27160,.T.);
#35076=ORIENTED_EDGE('',*,*,#27101,.T.);
#35077=ORIENTED_EDGE('',*,*,#25364,.T.);
#35078=ORIENTED_EDGE('',*,*,#26395,.T.);
#35079=ORIENTED_EDGE('',*,*,#27161,.T.);
#35080=ORIENTED_EDGE('',*,*,#27162,.F.);
#35081=ORIENTED_EDGE('',*,*,#27163,.F.);
#35082=ORIENTED_EDGE('',*,*,#27164,.T.);
#35083=ORIENTED_EDGE('',*,*,#27099,.T.);
#35084=ORIENTED_EDGE('',*,*,#25368,.T.);
#35085=ORIENTED_EDGE('',*,*,#26359,.T.);
#35086=ORIENTED_EDGE('',*,*,#27165,.T.);
#35087=ORIENTED_EDGE('',*,*,#27166,.F.);
#35088=ORIENTED_EDGE('',*,*,#27167,.F.);
#35089=ORIENTED_EDGE('',*,*,#27168,.T.);
#35090=ORIENTED_EDGE('',*,*,#27097,.T.);
#35091=ORIENTED_EDGE('',*,*,#25372,.T.);
#35092=ORIENTED_EDGE('',*,*,#26323,.T.);
#35093=ORIENTED_EDGE('',*,*,#27169,.T.);
#35094=ORIENTED_EDGE('',*,*,#27170,.F.);
#35095=ORIENTED_EDGE('',*,*,#27171,.F.);
#35096=ORIENTED_EDGE('',*,*,#27172,.T.);
#35097=ORIENTED_EDGE('',*,*,#27095,.T.);
#35098=ORIENTED_EDGE('',*,*,#25376,.T.);
#35099=ORIENTED_EDGE('',*,*,#26287,.T.);
#35100=ORIENTED_EDGE('',*,*,#27173,.T.);
#35101=ORIENTED_EDGE('',*,*,#27174,.F.);
#35102=ORIENTED_EDGE('',*,*,#27175,.F.);
#35103=ORIENTED_EDGE('',*,*,#27176,.T.);
#35104=ORIENTED_EDGE('',*,*,#27093,.T.);
#35105=ORIENTED_EDGE('',*,*,#25380,.T.);
#35106=ORIENTED_EDGE('',*,*,#26251,.T.);
#35107=ORIENTED_EDGE('',*,*,#27177,.T.);
#35108=ORIENTED_EDGE('',*,*,#27178,.F.);
#35109=ORIENTED_EDGE('',*,*,#27179,.F.);
#35110=ORIENTED_EDGE('',*,*,#27180,.T.);
#35111=ORIENTED_EDGE('',*,*,#27091,.T.);
#35112=ORIENTED_EDGE('',*,*,#25384,.T.);
#35113=ORIENTED_EDGE('',*,*,#26215,.T.);
#35114=ORIENTED_EDGE('',*,*,#27181,.T.);
#35115=ORIENTED_EDGE('',*,*,#27182,.F.);
#35116=ORIENTED_EDGE('',*,*,#27183,.F.);
#35117=ORIENTED_EDGE('',*,*,#27184,.T.);
#35118=ORIENTED_EDGE('',*,*,#27089,.T.);
#35119=ORIENTED_EDGE('',*,*,#25388,.T.);
#35120=ORIENTED_EDGE('',*,*,#26179,.T.);
#35121=ORIENTED_EDGE('',*,*,#27185,.T.);
#35122=ORIENTED_EDGE('',*,*,#27186,.F.);
#35123=ORIENTED_EDGE('',*,*,#27187,.F.);
#35124=ORIENTED_EDGE('',*,*,#27188,.T.);
#35125=ORIENTED_EDGE('',*,*,#27087,.T.);
#35126=ORIENTED_EDGE('',*,*,#25392,.T.);
#35127=ORIENTED_EDGE('',*,*,#26143,.T.);
#35128=ORIENTED_EDGE('',*,*,#27189,.T.);
#35129=ORIENTED_EDGE('',*,*,#27190,.F.);
#35130=ORIENTED_EDGE('',*,*,#27191,.F.);
#35131=ORIENTED_EDGE('',*,*,#27192,.T.);
#35132=ORIENTED_EDGE('',*,*,#27085,.T.);
#35133=ORIENTED_EDGE('',*,*,#25396,.T.);
#35134=ORIENTED_EDGE('',*,*,#26107,.T.);
#35135=ORIENTED_EDGE('',*,*,#27193,.T.);
#35136=ORIENTED_EDGE('',*,*,#27194,.F.);
#35137=ORIENTED_EDGE('',*,*,#27195,.F.);
#35138=ORIENTED_EDGE('',*,*,#27196,.T.);
#35139=ORIENTED_EDGE('',*,*,#27083,.T.);
#35140=ORIENTED_EDGE('',*,*,#25400,.T.);
#35141=ORIENTED_EDGE('',*,*,#26071,.T.);
#35142=ORIENTED_EDGE('',*,*,#27197,.T.);
#35143=ORIENTED_EDGE('',*,*,#27198,.F.);
#35144=ORIENTED_EDGE('',*,*,#27199,.F.);
#35145=ORIENTED_EDGE('',*,*,#27200,.T.);
#35146=ORIENTED_EDGE('',*,*,#27081,.T.);
#35147=ORIENTED_EDGE('',*,*,#25404,.T.);
#35148=ORIENTED_EDGE('',*,*,#26035,.T.);
#35149=ORIENTED_EDGE('',*,*,#27201,.T.);
#35150=ORIENTED_EDGE('',*,*,#27202,.F.);
#35151=ORIENTED_EDGE('',*,*,#27203,.F.);
#35152=ORIENTED_EDGE('',*,*,#27204,.T.);
#35153=ORIENTED_EDGE('',*,*,#27079,.T.);
#35154=ORIENTED_EDGE('',*,*,#25408,.T.);
#35155=ORIENTED_EDGE('',*,*,#25999,.T.);
#35156=ORIENTED_EDGE('',*,*,#27205,.T.);
#35157=ORIENTED_EDGE('',*,*,#27206,.F.);
#35158=ORIENTED_EDGE('',*,*,#27207,.F.);
#35159=ORIENTED_EDGE('',*,*,#27208,.T.);
#35160=ORIENTED_EDGE('',*,*,#27077,.T.);
#35161=ORIENTED_EDGE('',*,*,#25412,.T.);
#35162=ORIENTED_EDGE('',*,*,#25963,.T.);
#35163=ORIENTED_EDGE('',*,*,#27209,.T.);
#35164=ORIENTED_EDGE('',*,*,#27210,.F.);
#35165=ORIENTED_EDGE('',*,*,#27211,.F.);
#35166=ORIENTED_EDGE('',*,*,#27212,.T.);
#35167=ORIENTED_EDGE('',*,*,#27075,.T.);
#35168=ORIENTED_EDGE('',*,*,#25416,.T.);
#35169=ORIENTED_EDGE('',*,*,#25927,.T.);
#35170=ORIENTED_EDGE('',*,*,#27213,.T.);
#35171=ORIENTED_EDGE('',*,*,#27214,.F.);
#35172=ORIENTED_EDGE('',*,*,#27215,.F.);
#35173=ORIENTED_EDGE('',*,*,#27216,.T.);
#35174=ORIENTED_EDGE('',*,*,#27073,.T.);
#35175=ORIENTED_EDGE('',*,*,#25420,.T.);
#35176=ORIENTED_EDGE('',*,*,#25891,.T.);
#35177=ORIENTED_EDGE('',*,*,#27217,.T.);
#35178=ORIENTED_EDGE('',*,*,#27218,.F.);
#35179=ORIENTED_EDGE('',*,*,#27219,.F.);
#35180=ORIENTED_EDGE('',*,*,#27220,.T.);
#35181=ORIENTED_EDGE('',*,*,#27071,.T.);
#35182=ORIENTED_EDGE('',*,*,#25424,.T.);
#35183=ORIENTED_EDGE('',*,*,#25855,.T.);
#35184=ORIENTED_EDGE('',*,*,#27221,.T.);
#35185=ORIENTED_EDGE('',*,*,#27222,.F.);
#35186=ORIENTED_EDGE('',*,*,#27223,.F.);
#35187=ORIENTED_EDGE('',*,*,#27224,.T.);
#35188=ORIENTED_EDGE('',*,*,#27069,.T.);
#35189=ORIENTED_EDGE('',*,*,#25428,.T.);
#35190=ORIENTED_EDGE('',*,*,#25819,.T.);
#35191=ORIENTED_EDGE('',*,*,#27225,.T.);
#35192=ORIENTED_EDGE('',*,*,#27226,.F.);
#35193=ORIENTED_EDGE('',*,*,#27227,.F.);
#35194=ORIENTED_EDGE('',*,*,#27228,.T.);
#35195=ORIENTED_EDGE('',*,*,#27067,.T.);
#35196=ORIENTED_EDGE('',*,*,#25432,.T.);
#35197=ORIENTED_EDGE('',*,*,#25783,.T.);
#35198=ORIENTED_EDGE('',*,*,#27229,.T.);
#35199=ORIENTED_EDGE('',*,*,#27230,.F.);
#35200=ORIENTED_EDGE('',*,*,#27231,.F.);
#35201=ORIENTED_EDGE('',*,*,#27232,.T.);
#35202=ORIENTED_EDGE('',*,*,#27065,.T.);
#35203=ORIENTED_EDGE('',*,*,#25436,.T.);
#35204=ORIENTED_EDGE('',*,*,#25747,.T.);
#35205=ORIENTED_EDGE('',*,*,#27233,.T.);
#35206=ORIENTED_EDGE('',*,*,#27234,.F.);
#35207=ORIENTED_EDGE('',*,*,#27235,.F.);
#35208=ORIENTED_EDGE('',*,*,#27236,.T.);
#35209=ORIENTED_EDGE('',*,*,#27063,.T.);
#35210=ORIENTED_EDGE('',*,*,#25440,.T.);
#35211=ORIENTED_EDGE('',*,*,#25711,.T.);
#35212=ORIENTED_EDGE('',*,*,#27237,.T.);
#35213=ORIENTED_EDGE('',*,*,#27238,.F.);
#35214=ORIENTED_EDGE('',*,*,#27239,.F.);
#35215=ORIENTED_EDGE('',*,*,#27240,.T.);
#35216=ORIENTED_EDGE('',*,*,#27061,.T.);
#35217=ORIENTED_EDGE('',*,*,#25444,.T.);
#35218=ORIENTED_EDGE('',*,*,#25675,.T.);
#35219=ORIENTED_EDGE('',*,*,#27241,.T.);
#35220=ORIENTED_EDGE('',*,*,#27242,.F.);
#35221=ORIENTED_EDGE('',*,*,#27243,.F.);
#35222=ORIENTED_EDGE('',*,*,#27244,.T.);
#35223=ORIENTED_EDGE('',*,*,#27059,.T.);
#35224=ORIENTED_EDGE('',*,*,#25448,.T.);
#35225=ORIENTED_EDGE('',*,*,#25639,.T.);
#35226=ORIENTED_EDGE('',*,*,#27245,.T.);
#35227=ORIENTED_EDGE('',*,*,#27246,.F.);
#35228=ORIENTED_EDGE('',*,*,#27247,.F.);
#35229=ORIENTED_EDGE('',*,*,#27248,.T.);
#35230=ORIENTED_EDGE('',*,*,#27057,.T.);
#35231=ORIENTED_EDGE('',*,*,#25452,.T.);
#35232=ORIENTED_EDGE('',*,*,#25603,.T.);
#35233=ORIENTED_EDGE('',*,*,#27249,.T.);
#35234=ORIENTED_EDGE('',*,*,#27250,.F.);
#35235=ORIENTED_EDGE('',*,*,#27251,.F.);
#35236=ORIENTED_EDGE('',*,*,#27252,.T.);
#35237=ORIENTED_EDGE('',*,*,#27055,.T.);
#35238=ORIENTED_EDGE('',*,*,#25456,.T.);
#35239=ORIENTED_EDGE('',*,*,#25567,.T.);
#35240=ORIENTED_EDGE('',*,*,#27253,.T.);
#35241=ORIENTED_EDGE('',*,*,#27254,.F.);
#35242=ORIENTED_EDGE('',*,*,#27255,.F.);
#35243=ORIENTED_EDGE('',*,*,#27256,.T.);
#35244=ORIENTED_EDGE('',*,*,#27053,.T.);
#35245=ORIENTED_EDGE('',*,*,#25460,.T.);
#35246=ORIENTED_EDGE('',*,*,#25531,.T.);
#35247=ORIENTED_EDGE('',*,*,#27257,.T.);
#35248=ORIENTED_EDGE('',*,*,#27258,.F.);
#35249=ORIENTED_EDGE('',*,*,#27259,.F.);
#35250=ORIENTED_EDGE('',*,*,#27260,.T.);
#35251=ORIENTED_EDGE('',*,*,#27051,.T.);
#35252=ORIENTED_EDGE('',*,*,#27050,.T.);
#35253=ORIENTED_EDGE('',*,*,#27261,.F.);
#35254=ORIENTED_EDGE('',*,*,#27262,.F.);
#35255=ORIENTED_EDGE('',*,*,#25497,.F.);
#35256=ORIENTED_EDGE('',*,*,#26866,.T.);
#35257=ORIENTED_EDGE('',*,*,#27263,.F.);
#35258=ORIENTED_EDGE('',*,*,#27264,.F.);
#35259=ORIENTED_EDGE('',*,*,#26869,.F.);
#35260=ORIENTED_EDGE('',*,*,#26863,.T.);
#35261=ORIENTED_EDGE('',*,*,#27265,.F.);
#35262=ORIENTED_EDGE('',*,*,#27266,.F.);
#35263=ORIENTED_EDGE('',*,*,#26874,.F.);
#35264=ORIENTED_EDGE('',*,*,#26860,.T.);
#35265=ORIENTED_EDGE('',*,*,#27267,.F.);
#35266=ORIENTED_EDGE('',*,*,#27268,.F.);
#35267=ORIENTED_EDGE('',*,*,#26879,.F.);
#35268=ORIENTED_EDGE('',*,*,#26857,.T.);
#35269=ORIENTED_EDGE('',*,*,#27269,.F.);
#35270=ORIENTED_EDGE('',*,*,#27270,.F.);
#35271=ORIENTED_EDGE('',*,*,#26884,.F.);
#35272=ORIENTED_EDGE('',*,*,#26854,.T.);
#35273=ORIENTED_EDGE('',*,*,#27271,.F.);
#35274=ORIENTED_EDGE('',*,*,#27272,.F.);
#35275=ORIENTED_EDGE('',*,*,#26889,.F.);
#35276=ORIENTED_EDGE('',*,*,#26851,.T.);
#35277=ORIENTED_EDGE('',*,*,#27273,.F.);
#35278=ORIENTED_EDGE('',*,*,#27274,.F.);
#35279=ORIENTED_EDGE('',*,*,#26894,.F.);
#35280=ORIENTED_EDGE('',*,*,#26848,.T.);
#35281=ORIENTED_EDGE('',*,*,#27275,.F.);
#35282=ORIENTED_EDGE('',*,*,#27276,.F.);
#35283=ORIENTED_EDGE('',*,*,#26899,.F.);
#35284=ORIENTED_EDGE('',*,*,#26845,.T.);
#35285=ORIENTED_EDGE('',*,*,#27277,.F.);
#35286=ORIENTED_EDGE('',*,*,#27278,.F.);
#35287=ORIENTED_EDGE('',*,*,#26904,.F.);
#35288=ORIENTED_EDGE('',*,*,#26842,.T.);
#35289=ORIENTED_EDGE('',*,*,#27279,.F.);
#35290=ORIENTED_EDGE('',*,*,#27280,.F.);
#35291=ORIENTED_EDGE('',*,*,#26909,.F.);
#35292=ORIENTED_EDGE('',*,*,#26839,.T.);
#35293=ORIENTED_EDGE('',*,*,#27281,.F.);
#35294=ORIENTED_EDGE('',*,*,#27282,.F.);
#35295=ORIENTED_EDGE('',*,*,#26914,.F.);
#35296=ORIENTED_EDGE('',*,*,#26836,.T.);
#35297=ORIENTED_EDGE('',*,*,#27283,.F.);
#35298=ORIENTED_EDGE('',*,*,#27284,.F.);
#35299=ORIENTED_EDGE('',*,*,#26919,.F.);
#35300=ORIENTED_EDGE('',*,*,#26833,.T.);
#35301=ORIENTED_EDGE('',*,*,#27285,.F.);
#35302=ORIENTED_EDGE('',*,*,#27286,.F.);
#35303=ORIENTED_EDGE('',*,*,#26924,.F.);
#35304=ORIENTED_EDGE('',*,*,#26830,.T.);
#35305=ORIENTED_EDGE('',*,*,#27287,.F.);
#35306=ORIENTED_EDGE('',*,*,#27288,.F.);
#35307=ORIENTED_EDGE('',*,*,#26929,.F.);
#35308=ORIENTED_EDGE('',*,*,#26827,.T.);
#35309=ORIENTED_EDGE('',*,*,#27289,.F.);
#35310=ORIENTED_EDGE('',*,*,#27290,.F.);
#35311=ORIENTED_EDGE('',*,*,#26934,.F.);
#35312=ORIENTED_EDGE('',*,*,#26824,.T.);
#35313=ORIENTED_EDGE('',*,*,#27291,.F.);
#35314=ORIENTED_EDGE('',*,*,#27292,.F.);
#35315=ORIENTED_EDGE('',*,*,#26939,.F.);
#35316=ORIENTED_EDGE('',*,*,#26821,.T.);
#35317=ORIENTED_EDGE('',*,*,#27293,.F.);
#35318=ORIENTED_EDGE('',*,*,#27294,.F.);
#35319=ORIENTED_EDGE('',*,*,#26944,.F.);
#35320=ORIENTED_EDGE('',*,*,#26818,.T.);
#35321=ORIENTED_EDGE('',*,*,#27295,.F.);
#35322=ORIENTED_EDGE('',*,*,#27296,.F.);
#35323=ORIENTED_EDGE('',*,*,#26949,.F.);
#35324=ORIENTED_EDGE('',*,*,#26815,.T.);
#35325=ORIENTED_EDGE('',*,*,#27297,.F.);
#35326=ORIENTED_EDGE('',*,*,#27298,.F.);
#35327=ORIENTED_EDGE('',*,*,#26954,.F.);
#35328=ORIENTED_EDGE('',*,*,#26812,.T.);
#35329=ORIENTED_EDGE('',*,*,#27299,.F.);
#35330=ORIENTED_EDGE('',*,*,#27300,.F.);
#35331=ORIENTED_EDGE('',*,*,#26959,.F.);
#35332=ORIENTED_EDGE('',*,*,#26809,.T.);
#35333=ORIENTED_EDGE('',*,*,#27301,.F.);
#35334=ORIENTED_EDGE('',*,*,#27302,.F.);
#35335=ORIENTED_EDGE('',*,*,#26964,.F.);
#35336=ORIENTED_EDGE('',*,*,#26806,.T.);
#35337=ORIENTED_EDGE('',*,*,#27303,.F.);
#35338=ORIENTED_EDGE('',*,*,#27304,.F.);
#35339=ORIENTED_EDGE('',*,*,#26969,.F.);
#35340=ORIENTED_EDGE('',*,*,#26803,.T.);
#35341=ORIENTED_EDGE('',*,*,#27305,.F.);
#35342=ORIENTED_EDGE('',*,*,#27306,.F.);
#35343=ORIENTED_EDGE('',*,*,#26974,.F.);
#35344=ORIENTED_EDGE('',*,*,#26800,.T.);
#35345=ORIENTED_EDGE('',*,*,#27307,.F.);
#35346=ORIENTED_EDGE('',*,*,#27308,.F.);
#35347=ORIENTED_EDGE('',*,*,#26979,.F.);
#35348=ORIENTED_EDGE('',*,*,#26797,.T.);
#35349=ORIENTED_EDGE('',*,*,#27309,.F.);
#35350=ORIENTED_EDGE('',*,*,#27310,.F.);
#35351=ORIENTED_EDGE('',*,*,#26984,.F.);
#35352=ORIENTED_EDGE('',*,*,#26794,.T.);
#35353=ORIENTED_EDGE('',*,*,#27311,.F.);
#35354=ORIENTED_EDGE('',*,*,#27312,.F.);
#35355=ORIENTED_EDGE('',*,*,#26989,.F.);
#35356=ORIENTED_EDGE('',*,*,#26791,.T.);
#35357=ORIENTED_EDGE('',*,*,#27313,.F.);
#35358=ORIENTED_EDGE('',*,*,#27314,.F.);
#35359=ORIENTED_EDGE('',*,*,#26994,.F.);
#35360=ORIENTED_EDGE('',*,*,#26788,.T.);
#35361=ORIENTED_EDGE('',*,*,#27315,.F.);
#35362=ORIENTED_EDGE('',*,*,#27316,.F.);
#35363=ORIENTED_EDGE('',*,*,#26999,.F.);
#35364=ORIENTED_EDGE('',*,*,#26785,.T.);
#35365=ORIENTED_EDGE('',*,*,#27317,.F.);
#35366=ORIENTED_EDGE('',*,*,#27318,.F.);
#35367=ORIENTED_EDGE('',*,*,#27004,.F.);
#35368=ORIENTED_EDGE('',*,*,#26782,.T.);
#35369=ORIENTED_EDGE('',*,*,#27319,.F.);
#35370=ORIENTED_EDGE('',*,*,#27320,.F.);
#35371=ORIENTED_EDGE('',*,*,#27009,.F.);
#35372=ORIENTED_EDGE('',*,*,#26779,.T.);
#35373=ORIENTED_EDGE('',*,*,#27321,.F.);
#35374=ORIENTED_EDGE('',*,*,#27322,.F.);
#35375=ORIENTED_EDGE('',*,*,#27014,.F.);
#35376=ORIENTED_EDGE('',*,*,#26776,.T.);
#35377=ORIENTED_EDGE('',*,*,#27323,.F.);
#35378=ORIENTED_EDGE('',*,*,#27324,.F.);
#35379=ORIENTED_EDGE('',*,*,#27019,.F.);
#35380=ORIENTED_EDGE('',*,*,#26773,.T.);
#35381=ORIENTED_EDGE('',*,*,#27325,.F.);
#35382=ORIENTED_EDGE('',*,*,#27326,.F.);
#35383=ORIENTED_EDGE('',*,*,#27024,.F.);
#35384=ORIENTED_EDGE('',*,*,#26770,.T.);
#35385=ORIENTED_EDGE('',*,*,#27327,.F.);
#35386=ORIENTED_EDGE('',*,*,#27328,.F.);
#35387=ORIENTED_EDGE('',*,*,#27029,.F.);
#35388=ORIENTED_EDGE('',*,*,#26767,.T.);
#35389=ORIENTED_EDGE('',*,*,#27329,.F.);
#35390=ORIENTED_EDGE('',*,*,#27330,.F.);
#35391=ORIENTED_EDGE('',*,*,#27034,.F.);
#35392=ORIENTED_EDGE('',*,*,#26764,.T.);
#35393=ORIENTED_EDGE('',*,*,#27331,.F.);
#35394=ORIENTED_EDGE('',*,*,#27332,.F.);
#35395=ORIENTED_EDGE('',*,*,#27039,.F.);
#35396=ORIENTED_EDGE('',*,*,#26761,.T.);
#35397=ORIENTED_EDGE('',*,*,#27333,.F.);
#35398=ORIENTED_EDGE('',*,*,#27334,.F.);
#35399=ORIENTED_EDGE('',*,*,#27044,.F.);
#35400=ORIENTED_EDGE('',*,*,#27334,.T.);
#35401=ORIENTED_EDGE('',*,*,#27335,.F.);
#35402=ORIENTED_EDGE('',*,*,#27336,.F.);
#35403=ORIENTED_EDGE('',*,*,#27045,.F.);
#35404=ORIENTED_EDGE('',*,*,#27332,.T.);
#35405=ORIENTED_EDGE('',*,*,#27337,.F.);
#35406=ORIENTED_EDGE('',*,*,#27338,.F.);
#35407=ORIENTED_EDGE('',*,*,#27040,.F.);
#35408=ORIENTED_EDGE('',*,*,#27330,.T.);
#35409=ORIENTED_EDGE('',*,*,#27339,.F.);
#35410=ORIENTED_EDGE('',*,*,#27340,.F.);
#35411=ORIENTED_EDGE('',*,*,#27035,.F.);
#35412=ORIENTED_EDGE('',*,*,#27328,.T.);
#35413=ORIENTED_EDGE('',*,*,#27341,.F.);
#35414=ORIENTED_EDGE('',*,*,#27342,.F.);
#35415=ORIENTED_EDGE('',*,*,#27030,.F.);
#35416=ORIENTED_EDGE('',*,*,#27326,.T.);
#35417=ORIENTED_EDGE('',*,*,#27343,.F.);
#35418=ORIENTED_EDGE('',*,*,#27344,.F.);
#35419=ORIENTED_EDGE('',*,*,#27025,.F.);
#35420=ORIENTED_EDGE('',*,*,#27324,.T.);
#35421=ORIENTED_EDGE('',*,*,#27345,.F.);
#35422=ORIENTED_EDGE('',*,*,#27346,.F.);
#35423=ORIENTED_EDGE('',*,*,#27020,.F.);
#35424=ORIENTED_EDGE('',*,*,#27322,.T.);
#35425=ORIENTED_EDGE('',*,*,#27347,.F.);
#35426=ORIENTED_EDGE('',*,*,#27348,.F.);
#35427=ORIENTED_EDGE('',*,*,#27015,.F.);
#35428=ORIENTED_EDGE('',*,*,#27320,.T.);
#35429=ORIENTED_EDGE('',*,*,#27349,.F.);
#35430=ORIENTED_EDGE('',*,*,#27350,.F.);
#35431=ORIENTED_EDGE('',*,*,#27010,.F.);
#35432=ORIENTED_EDGE('',*,*,#27318,.T.);
#35433=ORIENTED_EDGE('',*,*,#27351,.F.);
#35434=ORIENTED_EDGE('',*,*,#27352,.F.);
#35435=ORIENTED_EDGE('',*,*,#27005,.F.);
#35436=ORIENTED_EDGE('',*,*,#27316,.T.);
#35437=ORIENTED_EDGE('',*,*,#27353,.F.);
#35438=ORIENTED_EDGE('',*,*,#27354,.F.);
#35439=ORIENTED_EDGE('',*,*,#27000,.F.);
#35440=ORIENTED_EDGE('',*,*,#27314,.T.);
#35441=ORIENTED_EDGE('',*,*,#27355,.F.);
#35442=ORIENTED_EDGE('',*,*,#27356,.F.);
#35443=ORIENTED_EDGE('',*,*,#26995,.F.);
#35444=ORIENTED_EDGE('',*,*,#27312,.T.);
#35445=ORIENTED_EDGE('',*,*,#27357,.F.);
#35446=ORIENTED_EDGE('',*,*,#27358,.F.);
#35447=ORIENTED_EDGE('',*,*,#26990,.F.);
#35448=ORIENTED_EDGE('',*,*,#27310,.T.);
#35449=ORIENTED_EDGE('',*,*,#27359,.F.);
#35450=ORIENTED_EDGE('',*,*,#27360,.F.);
#35451=ORIENTED_EDGE('',*,*,#26985,.F.);
#35452=ORIENTED_EDGE('',*,*,#27308,.T.);
#35453=ORIENTED_EDGE('',*,*,#27361,.F.);
#35454=ORIENTED_EDGE('',*,*,#27362,.F.);
#35455=ORIENTED_EDGE('',*,*,#26980,.F.);
#35456=ORIENTED_EDGE('',*,*,#27306,.T.);
#35457=ORIENTED_EDGE('',*,*,#27363,.F.);
#35458=ORIENTED_EDGE('',*,*,#27364,.F.);
#35459=ORIENTED_EDGE('',*,*,#26975,.F.);
#35460=ORIENTED_EDGE('',*,*,#27304,.T.);
#35461=ORIENTED_EDGE('',*,*,#27365,.F.);
#35462=ORIENTED_EDGE('',*,*,#27366,.F.);
#35463=ORIENTED_EDGE('',*,*,#26970,.F.);
#35464=ORIENTED_EDGE('',*,*,#27302,.T.);
#35465=ORIENTED_EDGE('',*,*,#27367,.F.);
#35466=ORIENTED_EDGE('',*,*,#27368,.F.);
#35467=ORIENTED_EDGE('',*,*,#26965,.F.);
#35468=ORIENTED_EDGE('',*,*,#27300,.T.);
#35469=ORIENTED_EDGE('',*,*,#27369,.F.);
#35470=ORIENTED_EDGE('',*,*,#27370,.F.);
#35471=ORIENTED_EDGE('',*,*,#27371,.F.);
#35472=ORIENTED_EDGE('',*,*,#26960,.F.);
#35473=ORIENTED_EDGE('',*,*,#27298,.T.);
#35474=ORIENTED_EDGE('',*,*,#27372,.F.);
#35475=ORIENTED_EDGE('',*,*,#27373,.F.);
#35476=ORIENTED_EDGE('',*,*,#26955,.F.);
#35477=ORIENTED_EDGE('',*,*,#27296,.T.);
#35478=ORIENTED_EDGE('',*,*,#27374,.F.);
#35479=ORIENTED_EDGE('',*,*,#27375,.F.);
#35480=ORIENTED_EDGE('',*,*,#26950,.F.);
#35481=ORIENTED_EDGE('',*,*,#27294,.T.);
#35482=ORIENTED_EDGE('',*,*,#27376,.F.);
#35483=ORIENTED_EDGE('',*,*,#27377,.F.);
#35484=ORIENTED_EDGE('',*,*,#26945,.F.);
#35485=ORIENTED_EDGE('',*,*,#27292,.T.);
#35486=ORIENTED_EDGE('',*,*,#27378,.F.);
#35487=ORIENTED_EDGE('',*,*,#27379,.F.);
#35488=ORIENTED_EDGE('',*,*,#26940,.F.);
#35489=ORIENTED_EDGE('',*,*,#27290,.T.);
#35490=ORIENTED_EDGE('',*,*,#27380,.F.);
#35491=ORIENTED_EDGE('',*,*,#27381,.F.);
#35492=ORIENTED_EDGE('',*,*,#26935,.F.);
#35493=ORIENTED_EDGE('',*,*,#27288,.T.);
#35494=ORIENTED_EDGE('',*,*,#27382,.F.);
#35495=ORIENTED_EDGE('',*,*,#27383,.F.);
#35496=ORIENTED_EDGE('',*,*,#26930,.F.);
#35497=ORIENTED_EDGE('',*,*,#27286,.T.);
#35498=ORIENTED_EDGE('',*,*,#27384,.F.);
#35499=ORIENTED_EDGE('',*,*,#27385,.F.);
#35500=ORIENTED_EDGE('',*,*,#26925,.F.);
#35501=ORIENTED_EDGE('',*,*,#27284,.T.);
#35502=ORIENTED_EDGE('',*,*,#27386,.F.);
#35503=ORIENTED_EDGE('',*,*,#27387,.F.);
#35504=ORIENTED_EDGE('',*,*,#26920,.F.);
#35505=ORIENTED_EDGE('',*,*,#27282,.T.);
#35506=ORIENTED_EDGE('',*,*,#27388,.F.);
#35507=ORIENTED_EDGE('',*,*,#27389,.F.);
#35508=ORIENTED_EDGE('',*,*,#26915,.F.);
#35509=ORIENTED_EDGE('',*,*,#27280,.T.);
#35510=ORIENTED_EDGE('',*,*,#27390,.F.);
#35511=ORIENTED_EDGE('',*,*,#27391,.F.);
#35512=ORIENTED_EDGE('',*,*,#26910,.F.);
#35513=ORIENTED_EDGE('',*,*,#27278,.T.);
#35514=ORIENTED_EDGE('',*,*,#27392,.F.);
#35515=ORIENTED_EDGE('',*,*,#27393,.F.);
#35516=ORIENTED_EDGE('',*,*,#26905,.F.);
#35517=ORIENTED_EDGE('',*,*,#27276,.T.);
#35518=ORIENTED_EDGE('',*,*,#27394,.F.);
#35519=ORIENTED_EDGE('',*,*,#27395,.F.);
#35520=ORIENTED_EDGE('',*,*,#26900,.F.);
#35521=ORIENTED_EDGE('',*,*,#27274,.T.);
#35522=ORIENTED_EDGE('',*,*,#27396,.F.);
#35523=ORIENTED_EDGE('',*,*,#27397,.F.);
#35524=ORIENTED_EDGE('',*,*,#26895,.F.);
#35525=ORIENTED_EDGE('',*,*,#27272,.T.);
#35526=ORIENTED_EDGE('',*,*,#27398,.F.);
#35527=ORIENTED_EDGE('',*,*,#27399,.F.);
#35528=ORIENTED_EDGE('',*,*,#26890,.F.);
#35529=ORIENTED_EDGE('',*,*,#27270,.T.);
#35530=ORIENTED_EDGE('',*,*,#27400,.F.);
#35531=ORIENTED_EDGE('',*,*,#27401,.F.);
#35532=ORIENTED_EDGE('',*,*,#26885,.F.);
#35533=ORIENTED_EDGE('',*,*,#27268,.T.);
#35534=ORIENTED_EDGE('',*,*,#27402,.F.);
#35535=ORIENTED_EDGE('',*,*,#27403,.F.);
#35536=ORIENTED_EDGE('',*,*,#26880,.F.);
#35537=ORIENTED_EDGE('',*,*,#27266,.T.);
#35538=ORIENTED_EDGE('',*,*,#27404,.F.);
#35539=ORIENTED_EDGE('',*,*,#27405,.F.);
#35540=ORIENTED_EDGE('',*,*,#26875,.F.);
#35541=ORIENTED_EDGE('',*,*,#27264,.T.);
#35542=ORIENTED_EDGE('',*,*,#27406,.F.);
#35543=ORIENTED_EDGE('',*,*,#27407,.F.);
#35544=ORIENTED_EDGE('',*,*,#26870,.F.);
#35545=ORIENTED_EDGE('',*,*,#27408,.F.);
#35546=ORIENTED_EDGE('',*,*,#27409,.F.);
#35547=ORIENTED_EDGE('',*,*,#26726,.T.);
#35548=ORIENTED_EDGE('',*,*,#26760,.T.);
#35549=ORIENTED_EDGE('',*,*,#27410,.F.);
#35550=ORIENTED_EDGE('',*,*,#27411,.F.);
#35551=ORIENTED_EDGE('',*,*,#26727,.T.);
#35552=ORIENTED_EDGE('',*,*,#27409,.T.);
#35553=ORIENTED_EDGE('',*,*,#27412,.F.);
#35554=ORIENTED_EDGE('',*,*,#27413,.F.);
#35555=ORIENTED_EDGE('',*,*,#26728,.T.);
#35556=ORIENTED_EDGE('',*,*,#27411,.T.);
#35557=ORIENTED_EDGE('',*,*,#27414,.F.);
#35558=ORIENTED_EDGE('',*,*,#27415,.F.);
#35559=ORIENTED_EDGE('',*,*,#26729,.T.);
#35560=ORIENTED_EDGE('',*,*,#27413,.T.);
#35561=ORIENTED_EDGE('',*,*,#27416,.F.);
#35562=ORIENTED_EDGE('',*,*,#27417,.F.);
#35563=ORIENTED_EDGE('',*,*,#26730,.T.);
#35564=ORIENTED_EDGE('',*,*,#27415,.T.);
#35565=ORIENTED_EDGE('',*,*,#27418,.F.);
#35566=ORIENTED_EDGE('',*,*,#27419,.F.);
#35567=ORIENTED_EDGE('',*,*,#26731,.T.);
#35568=ORIENTED_EDGE('',*,*,#27417,.T.);
#35569=ORIENTED_EDGE('',*,*,#27420,.F.);
#35570=ORIENTED_EDGE('',*,*,#27421,.F.);
#35571=ORIENTED_EDGE('',*,*,#26732,.T.);
#35572=ORIENTED_EDGE('',*,*,#27419,.T.);
#35573=ORIENTED_EDGE('',*,*,#27422,.F.);
#35574=ORIENTED_EDGE('',*,*,#27423,.F.);
#35575=ORIENTED_EDGE('',*,*,#26733,.T.);
#35576=ORIENTED_EDGE('',*,*,#27421,.T.);
#35577=ORIENTED_EDGE('',*,*,#27424,.F.);
#35578=ORIENTED_EDGE('',*,*,#27425,.F.);
#35579=ORIENTED_EDGE('',*,*,#26734,.T.);
#35580=ORIENTED_EDGE('',*,*,#27423,.T.);
#35581=ORIENTED_EDGE('',*,*,#27426,.F.);
#35582=ORIENTED_EDGE('',*,*,#27427,.F.);
#35583=ORIENTED_EDGE('',*,*,#26735,.T.);
#35584=ORIENTED_EDGE('',*,*,#27425,.T.);
#35585=ORIENTED_EDGE('',*,*,#27428,.F.);
#35586=ORIENTED_EDGE('',*,*,#27429,.F.);
#35587=ORIENTED_EDGE('',*,*,#26736,.T.);
#35588=ORIENTED_EDGE('',*,*,#27427,.T.);
#35589=ORIENTED_EDGE('',*,*,#27430,.F.);
#35590=ORIENTED_EDGE('',*,*,#27431,.F.);
#35591=ORIENTED_EDGE('',*,*,#26737,.T.);
#35592=ORIENTED_EDGE('',*,*,#27429,.T.);
#35593=ORIENTED_EDGE('',*,*,#27432,.F.);
#35594=ORIENTED_EDGE('',*,*,#27433,.F.);
#35595=ORIENTED_EDGE('',*,*,#26738,.T.);
#35596=ORIENTED_EDGE('',*,*,#27431,.T.);
#35597=ORIENTED_EDGE('',*,*,#26763,.T.);
#35598=ORIENTED_EDGE('',*,*,#26739,.T.);
#35599=ORIENTED_EDGE('',*,*,#27433,.T.);
#35600=ORIENTED_EDGE('',*,*,#27434,.F.);
#35601=ORIENTED_EDGE('',*,*,#27435,.F.);
#35602=ORIENTED_EDGE('',*,*,#27335,.T.);
#35603=ORIENTED_EDGE('',*,*,#27333,.T.);
#35604=ORIENTED_EDGE('',*,*,#27436,.F.);
#35605=ORIENTED_EDGE('',*,*,#27437,.F.);
#35606=ORIENTED_EDGE('',*,*,#26742,.T.);
#35607=ORIENTED_EDGE('',*,*,#27048,.T.);
#35608=ORIENTED_EDGE('',*,*,#27438,.F.);
#35609=ORIENTED_EDGE('',*,*,#27439,.F.);
#35610=ORIENTED_EDGE('',*,*,#26743,.T.);
#35611=ORIENTED_EDGE('',*,*,#27437,.T.);
#35612=ORIENTED_EDGE('',*,*,#27440,.F.);
#35613=ORIENTED_EDGE('',*,*,#27441,.F.);
#35614=ORIENTED_EDGE('',*,*,#26744,.T.);
#35615=ORIENTED_EDGE('',*,*,#27439,.T.);
#35616=ORIENTED_EDGE('',*,*,#27442,.F.);
#35617=ORIENTED_EDGE('',*,*,#27443,.F.);
#35618=ORIENTED_EDGE('',*,*,#26745,.T.);
#35619=ORIENTED_EDGE('',*,*,#27441,.T.);
#35620=ORIENTED_EDGE('',*,*,#27444,.F.);
#35621=ORIENTED_EDGE('',*,*,#27445,.F.);
#35622=ORIENTED_EDGE('',*,*,#26746,.T.);
#35623=ORIENTED_EDGE('',*,*,#27443,.T.);
#35624=ORIENTED_EDGE('',*,*,#27446,.F.);
#35625=ORIENTED_EDGE('',*,*,#27447,.F.);
#35626=ORIENTED_EDGE('',*,*,#26747,.T.);
#35627=ORIENTED_EDGE('',*,*,#27445,.T.);
#35628=ORIENTED_EDGE('',*,*,#27448,.F.);
#35629=ORIENTED_EDGE('',*,*,#27449,.F.);
#35630=ORIENTED_EDGE('',*,*,#26748,.T.);
#35631=ORIENTED_EDGE('',*,*,#27447,.T.);
#35632=ORIENTED_EDGE('',*,*,#27450,.F.);
#35633=ORIENTED_EDGE('',*,*,#27451,.F.);
#35634=ORIENTED_EDGE('',*,*,#26749,.T.);
#35635=ORIENTED_EDGE('',*,*,#27449,.T.);
#35636=ORIENTED_EDGE('',*,*,#27452,.F.);
#35637=ORIENTED_EDGE('',*,*,#27453,.F.);
#35638=ORIENTED_EDGE('',*,*,#26750,.T.);
#35639=ORIENTED_EDGE('',*,*,#27451,.T.);
#35640=ORIENTED_EDGE('',*,*,#27454,.F.);
#35641=ORIENTED_EDGE('',*,*,#27455,.F.);
#35642=ORIENTED_EDGE('',*,*,#26751,.T.);
#35643=ORIENTED_EDGE('',*,*,#27453,.T.);
#35644=ORIENTED_EDGE('',*,*,#27456,.F.);
#35645=ORIENTED_EDGE('',*,*,#27457,.F.);
#35646=ORIENTED_EDGE('',*,*,#26752,.T.);
#35647=ORIENTED_EDGE('',*,*,#27455,.T.);
#35648=ORIENTED_EDGE('',*,*,#27458,.F.);
#35649=ORIENTED_EDGE('',*,*,#27459,.F.);
#35650=ORIENTED_EDGE('',*,*,#26753,.T.);
#35651=ORIENTED_EDGE('',*,*,#27457,.T.);
#35652=ORIENTED_EDGE('',*,*,#27460,.F.);
#35653=ORIENTED_EDGE('',*,*,#27121,.F.);
#35654=ORIENTED_EDGE('',*,*,#26754,.T.);
#35655=ORIENTED_EDGE('',*,*,#27459,.T.);
#35656=ORIENTED_EDGE('',*,*,#27120,.T.);
#35657=ORIENTED_EDGE('',*,*,#27124,.F.);
#35658=ORIENTED_EDGE('',*,*,#27461,.F.);
#35659=ORIENTED_EDGE('',*,*,#26757,.F.);
#35660=ORIENTED_EDGE('',*,*,#27462,.T.);
#35661=ORIENTED_EDGE('',*,*,#27463,.T.);
#35662=ORIENTED_EDGE('',*,*,#27464,.T.);
#35663=ORIENTED_EDGE('',*,*,#27191,.T.);
#35664=ORIENTED_EDGE('',*,*,#27465,.F.);
#35665=ORIENTED_EDGE('',*,*,#26110,.T.);
#35666=ORIENTED_EDGE('',*,*,#27466,.T.);
#35667=ORIENTED_EDGE('',*,*,#27195,.T.);
#35668=ORIENTED_EDGE('',*,*,#27467,.F.);
#35669=ORIENTED_EDGE('',*,*,#26074,.T.);
#35670=ORIENTED_EDGE('',*,*,#27468,.T.);
#35671=ORIENTED_EDGE('',*,*,#27199,.T.);
#35672=ORIENTED_EDGE('',*,*,#27469,.F.);
#35673=ORIENTED_EDGE('',*,*,#26038,.T.);
#35674=ORIENTED_EDGE('',*,*,#27470,.T.);
#35675=ORIENTED_EDGE('',*,*,#27203,.T.);
#35676=ORIENTED_EDGE('',*,*,#27471,.F.);
#35677=ORIENTED_EDGE('',*,*,#26002,.T.);
#35678=ORIENTED_EDGE('',*,*,#27472,.T.);
#35679=ORIENTED_EDGE('',*,*,#27207,.T.);
#35680=ORIENTED_EDGE('',*,*,#27473,.F.);
#35681=ORIENTED_EDGE('',*,*,#25966,.T.);
#35682=ORIENTED_EDGE('',*,*,#27474,.T.);
#35683=ORIENTED_EDGE('',*,*,#27211,.T.);
#35684=ORIENTED_EDGE('',*,*,#27475,.F.);
#35685=ORIENTED_EDGE('',*,*,#25930,.T.);
#35686=ORIENTED_EDGE('',*,*,#27476,.T.);
#35687=ORIENTED_EDGE('',*,*,#27215,.T.);
#35688=ORIENTED_EDGE('',*,*,#27477,.F.);
#35689=ORIENTED_EDGE('',*,*,#25894,.T.);
#35690=ORIENTED_EDGE('',*,*,#27478,.T.);
#35691=ORIENTED_EDGE('',*,*,#27219,.T.);
#35692=ORIENTED_EDGE('',*,*,#27479,.F.);
#35693=ORIENTED_EDGE('',*,*,#25858,.T.);
#35694=ORIENTED_EDGE('',*,*,#27480,.T.);
#35695=ORIENTED_EDGE('',*,*,#27223,.T.);
#35696=ORIENTED_EDGE('',*,*,#27481,.F.);
#35697=ORIENTED_EDGE('',*,*,#25822,.T.);
#35698=ORIENTED_EDGE('',*,*,#27482,.T.);
#35699=ORIENTED_EDGE('',*,*,#27227,.T.);
#35700=ORIENTED_EDGE('',*,*,#27483,.F.);
#35701=ORIENTED_EDGE('',*,*,#25786,.T.);
#35702=ORIENTED_EDGE('',*,*,#27484,.T.);
#35703=ORIENTED_EDGE('',*,*,#27231,.T.);
#35704=ORIENTED_EDGE('',*,*,#27485,.F.);
#35705=ORIENTED_EDGE('',*,*,#25750,.T.);
#35706=ORIENTED_EDGE('',*,*,#27486,.T.);
#35707=ORIENTED_EDGE('',*,*,#27235,.T.);
#35708=ORIENTED_EDGE('',*,*,#27487,.F.);
#35709=ORIENTED_EDGE('',*,*,#25714,.T.);
#35710=ORIENTED_EDGE('',*,*,#27488,.T.);
#35711=ORIENTED_EDGE('',*,*,#27239,.T.);
#35712=ORIENTED_EDGE('',*,*,#27489,.F.);
#35713=ORIENTED_EDGE('',*,*,#25678,.T.);
#35714=ORIENTED_EDGE('',*,*,#27490,.T.);
#35715=ORIENTED_EDGE('',*,*,#27243,.T.);
#35716=ORIENTED_EDGE('',*,*,#27491,.F.);
#35717=ORIENTED_EDGE('',*,*,#25642,.T.);
#35718=ORIENTED_EDGE('',*,*,#27492,.T.);
#35719=ORIENTED_EDGE('',*,*,#27247,.T.);
#35720=ORIENTED_EDGE('',*,*,#27493,.F.);
#35721=ORIENTED_EDGE('',*,*,#25606,.T.);
#35722=ORIENTED_EDGE('',*,*,#27494,.T.);
#35723=ORIENTED_EDGE('',*,*,#27251,.T.);
#35724=ORIENTED_EDGE('',*,*,#27495,.F.);
#35725=ORIENTED_EDGE('',*,*,#25570,.T.);
#35726=ORIENTED_EDGE('',*,*,#27496,.T.);
#35727=ORIENTED_EDGE('',*,*,#27255,.T.);
#35728=ORIENTED_EDGE('',*,*,#27497,.F.);
#35729=ORIENTED_EDGE('',*,*,#25534,.T.);
#35730=ORIENTED_EDGE('',*,*,#27498,.T.);
#35731=ORIENTED_EDGE('',*,*,#27259,.T.);
#35732=ORIENTED_EDGE('',*,*,#27499,.F.);
#35733=ORIENTED_EDGE('',*,*,#25498,.T.);
#35734=ORIENTED_EDGE('',*,*,#27262,.T.);
#35735=ORIENTED_EDGE('',*,*,#27500,.T.);
#35736=ORIENTED_EDGE('',*,*,#27501,.F.);
#35737=ORIENTED_EDGE('',*,*,#26758,.T.);
#35738=ORIENTED_EDGE('',*,*,#27461,.T.);
#35739=ORIENTED_EDGE('',*,*,#27123,.T.);
#35740=ORIENTED_EDGE('',*,*,#27502,.F.);
#35741=ORIENTED_EDGE('',*,*,#26722,.T.);
#35742=ORIENTED_EDGE('',*,*,#27503,.T.);
#35743=ORIENTED_EDGE('',*,*,#27127,.T.);
#35744=ORIENTED_EDGE('',*,*,#27504,.F.);
#35745=ORIENTED_EDGE('',*,*,#26686,.T.);
#35746=ORIENTED_EDGE('',*,*,#27505,.T.);
#35747=ORIENTED_EDGE('',*,*,#27131,.T.);
#35748=ORIENTED_EDGE('',*,*,#27506,.F.);
#35749=ORIENTED_EDGE('',*,*,#26650,.T.);
#35750=ORIENTED_EDGE('',*,*,#27507,.T.);
#35751=ORIENTED_EDGE('',*,*,#27135,.T.);
#35752=ORIENTED_EDGE('',*,*,#27508,.F.);
#35753=ORIENTED_EDGE('',*,*,#26614,.T.);
#35754=ORIENTED_EDGE('',*,*,#27509,.T.);
#35755=ORIENTED_EDGE('',*,*,#27139,.T.);
#35756=ORIENTED_EDGE('',*,*,#27510,.F.);
#35757=ORIENTED_EDGE('',*,*,#26578,.T.);
#35758=ORIENTED_EDGE('',*,*,#27511,.T.);
#35759=ORIENTED_EDGE('',*,*,#27143,.T.);
#35760=ORIENTED_EDGE('',*,*,#27512,.F.);
#35761=ORIENTED_EDGE('',*,*,#26542,.T.);
#35762=ORIENTED_EDGE('',*,*,#27513,.T.);
#35763=ORIENTED_EDGE('',*,*,#27147,.T.);
#35764=ORIENTED_EDGE('',*,*,#27514,.F.);
#35765=ORIENTED_EDGE('',*,*,#26506,.T.);
#35766=ORIENTED_EDGE('',*,*,#27515,.T.);
#35767=ORIENTED_EDGE('',*,*,#27151,.T.);
#35768=ORIENTED_EDGE('',*,*,#27516,.F.);
#35769=ORIENTED_EDGE('',*,*,#26470,.T.);
#35770=ORIENTED_EDGE('',*,*,#27517,.T.);
#35771=ORIENTED_EDGE('',*,*,#27155,.T.);
#35772=ORIENTED_EDGE('',*,*,#27518,.F.);
#35773=ORIENTED_EDGE('',*,*,#26434,.T.);
#35774=ORIENTED_EDGE('',*,*,#27519,.T.);
#35775=ORIENTED_EDGE('',*,*,#27159,.T.);
#35776=ORIENTED_EDGE('',*,*,#27520,.F.);
#35777=ORIENTED_EDGE('',*,*,#26398,.T.);
#35778=ORIENTED_EDGE('',*,*,#27521,.T.);
#35779=ORIENTED_EDGE('',*,*,#27163,.T.);
#35780=ORIENTED_EDGE('',*,*,#27522,.F.);
#35781=ORIENTED_EDGE('',*,*,#26362,.T.);
#35782=ORIENTED_EDGE('',*,*,#27523,.T.);
#35783=ORIENTED_EDGE('',*,*,#27167,.T.);
#35784=ORIENTED_EDGE('',*,*,#27524,.F.);
#35785=ORIENTED_EDGE('',*,*,#26326,.T.);
#35786=ORIENTED_EDGE('',*,*,#27525,.T.);
#35787=ORIENTED_EDGE('',*,*,#27171,.T.);
#35788=ORIENTED_EDGE('',*,*,#27526,.F.);
#35789=ORIENTED_EDGE('',*,*,#26290,.T.);
#35790=ORIENTED_EDGE('',*,*,#27527,.T.);
#35791=ORIENTED_EDGE('',*,*,#27175,.T.);
#35792=ORIENTED_EDGE('',*,*,#27528,.F.);
#35793=ORIENTED_EDGE('',*,*,#26254,.T.);
#35794=ORIENTED_EDGE('',*,*,#27529,.T.);
#35795=ORIENTED_EDGE('',*,*,#27179,.T.);
#35796=ORIENTED_EDGE('',*,*,#27530,.F.);
#35797=ORIENTED_EDGE('',*,*,#26218,.T.);
#35798=ORIENTED_EDGE('',*,*,#27531,.T.);
#35799=ORIENTED_EDGE('',*,*,#27183,.T.);
#35800=ORIENTED_EDGE('',*,*,#27532,.F.);
#35801=ORIENTED_EDGE('',*,*,#26182,.T.);
#35802=ORIENTED_EDGE('',*,*,#27533,.T.);
#35803=ORIENTED_EDGE('',*,*,#27187,.T.);
#35804=ORIENTED_EDGE('',*,*,#27534,.F.);
#35805=ORIENTED_EDGE('',*,*,#26146,.T.);
#35806=ORIENTED_EDGE('',*,*,#27535,.T.);
#35807=ORIENTED_EDGE('',*,*,#27463,.F.);
#35808=ORIENTED_EDGE('',*,*,#27122,.T.);
#35809=ORIENTED_EDGE('',*,*,#27460,.T.);
#35810=ORIENTED_EDGE('',*,*,#27458,.T.);
#35811=ORIENTED_EDGE('',*,*,#27456,.T.);
#35812=ORIENTED_EDGE('',*,*,#27454,.T.);
#35813=ORIENTED_EDGE('',*,*,#27452,.T.);
#35814=ORIENTED_EDGE('',*,*,#27450,.T.);
#35815=ORIENTED_EDGE('',*,*,#27448,.T.);
#35816=ORIENTED_EDGE('',*,*,#27446,.T.);
#35817=ORIENTED_EDGE('',*,*,#27444,.T.);
#35818=ORIENTED_EDGE('',*,*,#27442,.T.);
#35819=ORIENTED_EDGE('',*,*,#27440,.T.);
#35820=ORIENTED_EDGE('',*,*,#27438,.T.);
#35821=ORIENTED_EDGE('',*,*,#27436,.T.);
#35822=ORIENTED_EDGE('',*,*,#27047,.T.);
#35823=ORIENTED_EDGE('',*,*,#27536,.F.);
#35824=ORIENTED_EDGE('',*,*,#27537,.T.);
#35825=ORIENTED_EDGE('',*,*,#27538,.T.);
#35826=ORIENTED_EDGE('',*,*,#27539,.T.);
#35827=ORIENTED_EDGE('',*,*,#27540,.T.);
#35828=ORIENTED_EDGE('',*,*,#27541,.T.);
#35829=ORIENTED_EDGE('',*,*,#27542,.T.);
#35830=ORIENTED_EDGE('',*,*,#27543,.T.);
#35831=ORIENTED_EDGE('',*,*,#27544,.T.);
#35832=ORIENTED_EDGE('',*,*,#27545,.T.);
#35833=ORIENTED_EDGE('',*,*,#27546,.T.);
#35834=ORIENTED_EDGE('',*,*,#27547,.T.);
#35835=ORIENTED_EDGE('',*,*,#27548,.T.);
#35836=ORIENTED_EDGE('',*,*,#27549,.T.);
#35837=ORIENTED_EDGE('',*,*,#27550,.T.);
#35838=ORIENTED_EDGE('',*,*,#26723,.T.);
#35839=ORIENTED_EDGE('',*,*,#27502,.T.);
#35840=ORIENTED_EDGE('',*,*,#27550,.F.);
#35841=ORIENTED_EDGE('',*,*,#27551,.F.);
#35842=ORIENTED_EDGE('',*,*,#26690,.T.);
#35843=ORIENTED_EDGE('',*,*,#26724,.T.);
#35844=ORIENTED_EDGE('',*,*,#27549,.F.);
#35845=ORIENTED_EDGE('',*,*,#27552,.F.);
#35846=ORIENTED_EDGE('',*,*,#26691,.T.);
#35847=ORIENTED_EDGE('',*,*,#27551,.T.);
#35848=ORIENTED_EDGE('',*,*,#27548,.F.);
#35849=ORIENTED_EDGE('',*,*,#27553,.F.);
#35850=ORIENTED_EDGE('',*,*,#26692,.T.);
#35851=ORIENTED_EDGE('',*,*,#27552,.T.);
#35852=ORIENTED_EDGE('',*,*,#27547,.F.);
#35853=ORIENTED_EDGE('',*,*,#27554,.F.);
#35854=ORIENTED_EDGE('',*,*,#26693,.T.);
#35855=ORIENTED_EDGE('',*,*,#27553,.T.);
#35856=ORIENTED_EDGE('',*,*,#27546,.F.);
#35857=ORIENTED_EDGE('',*,*,#27555,.F.);
#35858=ORIENTED_EDGE('',*,*,#26694,.T.);
#35859=ORIENTED_EDGE('',*,*,#27554,.T.);
#35860=ORIENTED_EDGE('',*,*,#27545,.F.);
#35861=ORIENTED_EDGE('',*,*,#27556,.F.);
#35862=ORIENTED_EDGE('',*,*,#26695,.T.);
#35863=ORIENTED_EDGE('',*,*,#27555,.T.);
#35864=ORIENTED_EDGE('',*,*,#27544,.F.);
#35865=ORIENTED_EDGE('',*,*,#27557,.F.);
#35866=ORIENTED_EDGE('',*,*,#26696,.T.);
#35867=ORIENTED_EDGE('',*,*,#27556,.T.);
#35868=ORIENTED_EDGE('',*,*,#27543,.F.);
#35869=ORIENTED_EDGE('',*,*,#27558,.F.);
#35870=ORIENTED_EDGE('',*,*,#26697,.T.);
#35871=ORIENTED_EDGE('',*,*,#27557,.T.);
#35872=ORIENTED_EDGE('',*,*,#27542,.F.);
#35873=ORIENTED_EDGE('',*,*,#27559,.F.);
#35874=ORIENTED_EDGE('',*,*,#26698,.T.);
#35875=ORIENTED_EDGE('',*,*,#27558,.T.);
#35876=ORIENTED_EDGE('',*,*,#27541,.F.);
#35877=ORIENTED_EDGE('',*,*,#27560,.F.);
#35878=ORIENTED_EDGE('',*,*,#26699,.T.);
#35879=ORIENTED_EDGE('',*,*,#27559,.T.);
#35880=ORIENTED_EDGE('',*,*,#27540,.F.);
#35881=ORIENTED_EDGE('',*,*,#27561,.F.);
#35882=ORIENTED_EDGE('',*,*,#26700,.T.);
#35883=ORIENTED_EDGE('',*,*,#27560,.T.);
#35884=ORIENTED_EDGE('',*,*,#27539,.F.);
#35885=ORIENTED_EDGE('',*,*,#27562,.F.);
#35886=ORIENTED_EDGE('',*,*,#26701,.T.);
#35887=ORIENTED_EDGE('',*,*,#27561,.T.);
#35888=ORIENTED_EDGE('',*,*,#27538,.F.);
#35889=ORIENTED_EDGE('',*,*,#27563,.F.);
#35890=ORIENTED_EDGE('',*,*,#26702,.T.);
#35891=ORIENTED_EDGE('',*,*,#27562,.T.);
#35892=ORIENTED_EDGE('',*,*,#26766,.T.);
#35893=ORIENTED_EDGE('',*,*,#26703,.T.);
#35894=ORIENTED_EDGE('',*,*,#27563,.T.);
#35895=ORIENTED_EDGE('',*,*,#27537,.F.);
#35896=ORIENTED_EDGE('',*,*,#27564,.F.);
#35897=ORIENTED_EDGE('',*,*,#27337,.T.);
#35898=ORIENTED_EDGE('',*,*,#27331,.T.);
#35899=ORIENTED_EDGE('',*,*,#27565,.F.);
#35900=ORIENTED_EDGE('',*,*,#27566,.F.);
#35901=ORIENTED_EDGE('',*,*,#26706,.T.);
#35902=ORIENTED_EDGE('',*,*,#27043,.T.);
#35903=ORIENTED_EDGE('',*,*,#27567,.F.);
#35904=ORIENTED_EDGE('',*,*,#27568,.F.);
#35905=ORIENTED_EDGE('',*,*,#26707,.T.);
#35906=ORIENTED_EDGE('',*,*,#27566,.T.);
#35907=ORIENTED_EDGE('',*,*,#27569,.F.);
#35908=ORIENTED_EDGE('',*,*,#27570,.F.);
#35909=ORIENTED_EDGE('',*,*,#26708,.T.);
#35910=ORIENTED_EDGE('',*,*,#27568,.T.);
#35911=ORIENTED_EDGE('',*,*,#27571,.F.);
#35912=ORIENTED_EDGE('',*,*,#27572,.F.);
#35913=ORIENTED_EDGE('',*,*,#26709,.T.);
#35914=ORIENTED_EDGE('',*,*,#27570,.T.);
#35915=ORIENTED_EDGE('',*,*,#27573,.F.);
#35916=ORIENTED_EDGE('',*,*,#27574,.F.);
#35917=ORIENTED_EDGE('',*,*,#26710,.T.);
#35918=ORIENTED_EDGE('',*,*,#27572,.T.);
#35919=ORIENTED_EDGE('',*,*,#27575,.F.);
#35920=ORIENTED_EDGE('',*,*,#27576,.F.);
#35921=ORIENTED_EDGE('',*,*,#26711,.T.);
#35922=ORIENTED_EDGE('',*,*,#27574,.T.);
#35923=ORIENTED_EDGE('',*,*,#27577,.F.);
#35924=ORIENTED_EDGE('',*,*,#27578,.F.);
#35925=ORIENTED_EDGE('',*,*,#26712,.T.);
#35926=ORIENTED_EDGE('',*,*,#27576,.T.);
#35927=ORIENTED_EDGE('',*,*,#27579,.F.);
#35928=ORIENTED_EDGE('',*,*,#27580,.F.);
#35929=ORIENTED_EDGE('',*,*,#26713,.T.);
#35930=ORIENTED_EDGE('',*,*,#27578,.T.);
#35931=ORIENTED_EDGE('',*,*,#27581,.F.);
#35932=ORIENTED_EDGE('',*,*,#27582,.F.);
#35933=ORIENTED_EDGE('',*,*,#26714,.T.);
#35934=ORIENTED_EDGE('',*,*,#27580,.T.);
#35935=ORIENTED_EDGE('',*,*,#27583,.F.);
#35936=ORIENTED_EDGE('',*,*,#27584,.F.);
#35937=ORIENTED_EDGE('',*,*,#26715,.T.);
#35938=ORIENTED_EDGE('',*,*,#27582,.T.);
#35939=ORIENTED_EDGE('',*,*,#27585,.F.);
#35940=ORIENTED_EDGE('',*,*,#27586,.F.);
#35941=ORIENTED_EDGE('',*,*,#26716,.T.);
#35942=ORIENTED_EDGE('',*,*,#27584,.T.);
#35943=ORIENTED_EDGE('',*,*,#27587,.F.);
#35944=ORIENTED_EDGE('',*,*,#27588,.F.);
#35945=ORIENTED_EDGE('',*,*,#26717,.T.);
#35946=ORIENTED_EDGE('',*,*,#27586,.T.);
#35947=ORIENTED_EDGE('',*,*,#27589,.F.);
#35948=ORIENTED_EDGE('',*,*,#27125,.F.);
#35949=ORIENTED_EDGE('',*,*,#26718,.T.);
#35950=ORIENTED_EDGE('',*,*,#27588,.T.);
#35951=ORIENTED_EDGE('',*,*,#27118,.T.);
#35952=ORIENTED_EDGE('',*,*,#27128,.F.);
#35953=ORIENTED_EDGE('',*,*,#27503,.F.);
#35954=ORIENTED_EDGE('',*,*,#26721,.F.);
#35955=ORIENTED_EDGE('',*,*,#27126,.T.);
#35956=ORIENTED_EDGE('',*,*,#27589,.T.);
#35957=ORIENTED_EDGE('',*,*,#27587,.T.);
#35958=ORIENTED_EDGE('',*,*,#27585,.T.);
#35959=ORIENTED_EDGE('',*,*,#27583,.T.);
#35960=ORIENTED_EDGE('',*,*,#27581,.T.);
#35961=ORIENTED_EDGE('',*,*,#27579,.T.);
#35962=ORIENTED_EDGE('',*,*,#27577,.T.);
#35963=ORIENTED_EDGE('',*,*,#27575,.T.);
#35964=ORIENTED_EDGE('',*,*,#27573,.T.);
#35965=ORIENTED_EDGE('',*,*,#27571,.T.);
#35966=ORIENTED_EDGE('',*,*,#27569,.T.);
#35967=ORIENTED_EDGE('',*,*,#27567,.T.);
#35968=ORIENTED_EDGE('',*,*,#27565,.T.);
#35969=ORIENTED_EDGE('',*,*,#27042,.T.);
#35970=ORIENTED_EDGE('',*,*,#27590,.F.);
#35971=ORIENTED_EDGE('',*,*,#27591,.T.);
#35972=ORIENTED_EDGE('',*,*,#27592,.T.);
#35973=ORIENTED_EDGE('',*,*,#27593,.T.);
#35974=ORIENTED_EDGE('',*,*,#27594,.T.);
#35975=ORIENTED_EDGE('',*,*,#27595,.T.);
#35976=ORIENTED_EDGE('',*,*,#27596,.T.);
#35977=ORIENTED_EDGE('',*,*,#27597,.T.);
#35978=ORIENTED_EDGE('',*,*,#27598,.T.);
#35979=ORIENTED_EDGE('',*,*,#27599,.T.);
#35980=ORIENTED_EDGE('',*,*,#27600,.T.);
#35981=ORIENTED_EDGE('',*,*,#27601,.T.);
#35982=ORIENTED_EDGE('',*,*,#27602,.T.);
#35983=ORIENTED_EDGE('',*,*,#27603,.T.);
#35984=ORIENTED_EDGE('',*,*,#27604,.T.);
#35985=ORIENTED_EDGE('',*,*,#26687,.T.);
#35986=ORIENTED_EDGE('',*,*,#27504,.T.);
#35987=ORIENTED_EDGE('',*,*,#27604,.F.);
#35988=ORIENTED_EDGE('',*,*,#27605,.F.);
#35989=ORIENTED_EDGE('',*,*,#26654,.T.);
#35990=ORIENTED_EDGE('',*,*,#26688,.T.);
#35991=ORIENTED_EDGE('',*,*,#27603,.F.);
#35992=ORIENTED_EDGE('',*,*,#27606,.F.);
#35993=ORIENTED_EDGE('',*,*,#26655,.T.);
#35994=ORIENTED_EDGE('',*,*,#27605,.T.);
#35995=ORIENTED_EDGE('',*,*,#27602,.F.);
#35996=ORIENTED_EDGE('',*,*,#27607,.F.);
#35997=ORIENTED_EDGE('',*,*,#26656,.T.);
#35998=ORIENTED_EDGE('',*,*,#27606,.T.);
#35999=ORIENTED_EDGE('',*,*,#27601,.F.);
#36000=ORIENTED_EDGE('',*,*,#27608,.F.);
#36001=ORIENTED_EDGE('',*,*,#26657,.T.);
#36002=ORIENTED_EDGE('',*,*,#27607,.T.);
#36003=ORIENTED_EDGE('',*,*,#27600,.F.);
#36004=ORIENTED_EDGE('',*,*,#27609,.F.);
#36005=ORIENTED_EDGE('',*,*,#26658,.T.);
#36006=ORIENTED_EDGE('',*,*,#27608,.T.);
#36007=ORIENTED_EDGE('',*,*,#27599,.F.);
#36008=ORIENTED_EDGE('',*,*,#27610,.F.);
#36009=ORIENTED_EDGE('',*,*,#26659,.T.);
#36010=ORIENTED_EDGE('',*,*,#27609,.T.);
#36011=ORIENTED_EDGE('',*,*,#27598,.F.);
#36012=ORIENTED_EDGE('',*,*,#27611,.F.);
#36013=ORIENTED_EDGE('',*,*,#26660,.T.);
#36014=ORIENTED_EDGE('',*,*,#27610,.T.);
#36015=ORIENTED_EDGE('',*,*,#27597,.F.);
#36016=ORIENTED_EDGE('',*,*,#27612,.F.);
#36017=ORIENTED_EDGE('',*,*,#26661,.T.);
#36018=ORIENTED_EDGE('',*,*,#27611,.T.);
#36019=ORIENTED_EDGE('',*,*,#27596,.F.);
#36020=ORIENTED_EDGE('',*,*,#27613,.F.);
#36021=ORIENTED_EDGE('',*,*,#26662,.T.);
#36022=ORIENTED_EDGE('',*,*,#27612,.T.);
#36023=ORIENTED_EDGE('',*,*,#27595,.F.);
#36024=ORIENTED_EDGE('',*,*,#27614,.F.);
#36025=ORIENTED_EDGE('',*,*,#26663,.T.);
#36026=ORIENTED_EDGE('',*,*,#27613,.T.);
#36027=ORIENTED_EDGE('',*,*,#27594,.F.);
#36028=ORIENTED_EDGE('',*,*,#27615,.F.);
#36029=ORIENTED_EDGE('',*,*,#26664,.T.);
#36030=ORIENTED_EDGE('',*,*,#27614,.T.);
#36031=ORIENTED_EDGE('',*,*,#27593,.F.);
#36032=ORIENTED_EDGE('',*,*,#27616,.F.);
#36033=ORIENTED_EDGE('',*,*,#26665,.T.);
#36034=ORIENTED_EDGE('',*,*,#27615,.T.);
#36035=ORIENTED_EDGE('',*,*,#27592,.F.);
#36036=ORIENTED_EDGE('',*,*,#27617,.F.);
#36037=ORIENTED_EDGE('',*,*,#26666,.T.);
#36038=ORIENTED_EDGE('',*,*,#27616,.T.);
#36039=ORIENTED_EDGE('',*,*,#26769,.T.);
#36040=ORIENTED_EDGE('',*,*,#26667,.T.);
#36041=ORIENTED_EDGE('',*,*,#27617,.T.);
#36042=ORIENTED_EDGE('',*,*,#27591,.F.);
#36043=ORIENTED_EDGE('',*,*,#27618,.F.);
#36044=ORIENTED_EDGE('',*,*,#27339,.T.);
#36045=ORIENTED_EDGE('',*,*,#27329,.T.);
#36046=ORIENTED_EDGE('',*,*,#27619,.F.);
#36047=ORIENTED_EDGE('',*,*,#27620,.F.);
#36048=ORIENTED_EDGE('',*,*,#26670,.T.);
#36049=ORIENTED_EDGE('',*,*,#27038,.T.);
#36050=ORIENTED_EDGE('',*,*,#27621,.F.);
#36051=ORIENTED_EDGE('',*,*,#27622,.F.);
#36052=ORIENTED_EDGE('',*,*,#26671,.T.);
#36053=ORIENTED_EDGE('',*,*,#27620,.T.);
#36054=ORIENTED_EDGE('',*,*,#27623,.F.);
#36055=ORIENTED_EDGE('',*,*,#27624,.F.);
#36056=ORIENTED_EDGE('',*,*,#26672,.T.);
#36057=ORIENTED_EDGE('',*,*,#27622,.T.);
#36058=ORIENTED_EDGE('',*,*,#27625,.F.);
#36059=ORIENTED_EDGE('',*,*,#27626,.F.);
#36060=ORIENTED_EDGE('',*,*,#26673,.T.);
#36061=ORIENTED_EDGE('',*,*,#27624,.T.);
#36062=ORIENTED_EDGE('',*,*,#27627,.F.);
#36063=ORIENTED_EDGE('',*,*,#27628,.F.);
#36064=ORIENTED_EDGE('',*,*,#26674,.T.);
#36065=ORIENTED_EDGE('',*,*,#27626,.T.);
#36066=ORIENTED_EDGE('',*,*,#27629,.F.);
#36067=ORIENTED_EDGE('',*,*,#27630,.F.);
#36068=ORIENTED_EDGE('',*,*,#26675,.T.);
#36069=ORIENTED_EDGE('',*,*,#27628,.T.);
#36070=ORIENTED_EDGE('',*,*,#27631,.F.);
#36071=ORIENTED_EDGE('',*,*,#27632,.F.);
#36072=ORIENTED_EDGE('',*,*,#26676,.T.);
#36073=ORIENTED_EDGE('',*,*,#27630,.T.);
#36074=ORIENTED_EDGE('',*,*,#27633,.F.);
#36075=ORIENTED_EDGE('',*,*,#27634,.F.);
#36076=ORIENTED_EDGE('',*,*,#26677,.T.);
#36077=ORIENTED_EDGE('',*,*,#27632,.T.);
#36078=ORIENTED_EDGE('',*,*,#27635,.F.);
#36079=ORIENTED_EDGE('',*,*,#27636,.F.);
#36080=ORIENTED_EDGE('',*,*,#26678,.T.);
#36081=ORIENTED_EDGE('',*,*,#27634,.T.);
#36082=ORIENTED_EDGE('',*,*,#27637,.F.);
#36083=ORIENTED_EDGE('',*,*,#27638,.F.);
#36084=ORIENTED_EDGE('',*,*,#26679,.T.);
#36085=ORIENTED_EDGE('',*,*,#27636,.T.);
#36086=ORIENTED_EDGE('',*,*,#27639,.F.);
#36087=ORIENTED_EDGE('',*,*,#27640,.F.);
#36088=ORIENTED_EDGE('',*,*,#26680,.T.);
#36089=ORIENTED_EDGE('',*,*,#27638,.T.);
#36090=ORIENTED_EDGE('',*,*,#27641,.F.);
#36091=ORIENTED_EDGE('',*,*,#27642,.F.);
#36092=ORIENTED_EDGE('',*,*,#26681,.T.);
#36093=ORIENTED_EDGE('',*,*,#27640,.T.);
#36094=ORIENTED_EDGE('',*,*,#27643,.F.);
#36095=ORIENTED_EDGE('',*,*,#27129,.F.);
#36096=ORIENTED_EDGE('',*,*,#26682,.T.);
#36097=ORIENTED_EDGE('',*,*,#27642,.T.);
#36098=ORIENTED_EDGE('',*,*,#27116,.T.);
#36099=ORIENTED_EDGE('',*,*,#27132,.F.);
#36100=ORIENTED_EDGE('',*,*,#27505,.F.);
#36101=ORIENTED_EDGE('',*,*,#26685,.F.);
#36102=ORIENTED_EDGE('',*,*,#27130,.T.);
#36103=ORIENTED_EDGE('',*,*,#27643,.T.);
#36104=ORIENTED_EDGE('',*,*,#27641,.T.);
#36105=ORIENTED_EDGE('',*,*,#27639,.T.);
#36106=ORIENTED_EDGE('',*,*,#27637,.T.);
#36107=ORIENTED_EDGE('',*,*,#27635,.T.);
#36108=ORIENTED_EDGE('',*,*,#27633,.T.);
#36109=ORIENTED_EDGE('',*,*,#27631,.T.);
#36110=ORIENTED_EDGE('',*,*,#27629,.T.);
#36111=ORIENTED_EDGE('',*,*,#27627,.T.);
#36112=ORIENTED_EDGE('',*,*,#27625,.T.);
#36113=ORIENTED_EDGE('',*,*,#27623,.T.);
#36114=ORIENTED_EDGE('',*,*,#27621,.T.);
#36115=ORIENTED_EDGE('',*,*,#27619,.T.);
#36116=ORIENTED_EDGE('',*,*,#27037,.T.);
#36117=ORIENTED_EDGE('',*,*,#27644,.F.);
#36118=ORIENTED_EDGE('',*,*,#27645,.T.);
#36119=ORIENTED_EDGE('',*,*,#27646,.T.);
#36120=ORIENTED_EDGE('',*,*,#27647,.T.);
#36121=ORIENTED_EDGE('',*,*,#27648,.T.);
#36122=ORIENTED_EDGE('',*,*,#27649,.T.);
#36123=ORIENTED_EDGE('',*,*,#27650,.T.);
#36124=ORIENTED_EDGE('',*,*,#27651,.T.);
#36125=ORIENTED_EDGE('',*,*,#27652,.T.);
#36126=ORIENTED_EDGE('',*,*,#27653,.T.);
#36127=ORIENTED_EDGE('',*,*,#27654,.T.);
#36128=ORIENTED_EDGE('',*,*,#27655,.T.);
#36129=ORIENTED_EDGE('',*,*,#27656,.T.);
#36130=ORIENTED_EDGE('',*,*,#27657,.T.);
#36131=ORIENTED_EDGE('',*,*,#27658,.T.);
#36132=ORIENTED_EDGE('',*,*,#26651,.T.);
#36133=ORIENTED_EDGE('',*,*,#27506,.T.);
#36134=ORIENTED_EDGE('',*,*,#27658,.F.);
#36135=ORIENTED_EDGE('',*,*,#27659,.F.);
#36136=ORIENTED_EDGE('',*,*,#26618,.T.);
#36137=ORIENTED_EDGE('',*,*,#26652,.T.);
#36138=ORIENTED_EDGE('',*,*,#27657,.F.);
#36139=ORIENTED_EDGE('',*,*,#27660,.F.);
#36140=ORIENTED_EDGE('',*,*,#26619,.T.);
#36141=ORIENTED_EDGE('',*,*,#27659,.T.);
#36142=ORIENTED_EDGE('',*,*,#27656,.F.);
#36143=ORIENTED_EDGE('',*,*,#27661,.F.);
#36144=ORIENTED_EDGE('',*,*,#26620,.T.);
#36145=ORIENTED_EDGE('',*,*,#27660,.T.);
#36146=ORIENTED_EDGE('',*,*,#27655,.F.);
#36147=ORIENTED_EDGE('',*,*,#27662,.F.);
#36148=ORIENTED_EDGE('',*,*,#26621,.T.);
#36149=ORIENTED_EDGE('',*,*,#27661,.T.);
#36150=ORIENTED_EDGE('',*,*,#27654,.F.);
#36151=ORIENTED_EDGE('',*,*,#27663,.F.);
#36152=ORIENTED_EDGE('',*,*,#26622,.T.);
#36153=ORIENTED_EDGE('',*,*,#27662,.T.);
#36154=ORIENTED_EDGE('',*,*,#27653,.F.);
#36155=ORIENTED_EDGE('',*,*,#27664,.F.);
#36156=ORIENTED_EDGE('',*,*,#26623,.T.);
#36157=ORIENTED_EDGE('',*,*,#27663,.T.);
#36158=ORIENTED_EDGE('',*,*,#27652,.F.);
#36159=ORIENTED_EDGE('',*,*,#27665,.F.);
#36160=ORIENTED_EDGE('',*,*,#26624,.T.);
#36161=ORIENTED_EDGE('',*,*,#27664,.T.);
#36162=ORIENTED_EDGE('',*,*,#27651,.F.);
#36163=ORIENTED_EDGE('',*,*,#27666,.F.);
#36164=ORIENTED_EDGE('',*,*,#26625,.T.);
#36165=ORIENTED_EDGE('',*,*,#27665,.T.);
#36166=ORIENTED_EDGE('',*,*,#27650,.F.);
#36167=ORIENTED_EDGE('',*,*,#27667,.F.);
#36168=ORIENTED_EDGE('',*,*,#26626,.T.);
#36169=ORIENTED_EDGE('',*,*,#27666,.T.);
#36170=ORIENTED_EDGE('',*,*,#27649,.F.);
#36171=ORIENTED_EDGE('',*,*,#27668,.F.);
#36172=ORIENTED_EDGE('',*,*,#26627,.T.);
#36173=ORIENTED_EDGE('',*,*,#27667,.T.);
#36174=ORIENTED_EDGE('',*,*,#27648,.F.);
#36175=ORIENTED_EDGE('',*,*,#27669,.F.);
#36176=ORIENTED_EDGE('',*,*,#26628,.T.);
#36177=ORIENTED_EDGE('',*,*,#27668,.T.);
#36178=ORIENTED_EDGE('',*,*,#27647,.F.);
#36179=ORIENTED_EDGE('',*,*,#27670,.F.);
#36180=ORIENTED_EDGE('',*,*,#26629,.T.);
#36181=ORIENTED_EDGE('',*,*,#27669,.T.);
#36182=ORIENTED_EDGE('',*,*,#27646,.F.);
#36183=ORIENTED_EDGE('',*,*,#27671,.F.);
#36184=ORIENTED_EDGE('',*,*,#26630,.T.);
#36185=ORIENTED_EDGE('',*,*,#27670,.T.);
#36186=ORIENTED_EDGE('',*,*,#26772,.T.);
#36187=ORIENTED_EDGE('',*,*,#26631,.T.);
#36188=ORIENTED_EDGE('',*,*,#27671,.T.);
#36189=ORIENTED_EDGE('',*,*,#27645,.F.);
#36190=ORIENTED_EDGE('',*,*,#27672,.F.);
#36191=ORIENTED_EDGE('',*,*,#27341,.T.);
#36192=ORIENTED_EDGE('',*,*,#27327,.T.);
#36193=ORIENTED_EDGE('',*,*,#27673,.F.);
#36194=ORIENTED_EDGE('',*,*,#27674,.F.);
#36195=ORIENTED_EDGE('',*,*,#26634,.T.);
#36196=ORIENTED_EDGE('',*,*,#27033,.T.);
#36197=ORIENTED_EDGE('',*,*,#27675,.F.);
#36198=ORIENTED_EDGE('',*,*,#27676,.F.);
#36199=ORIENTED_EDGE('',*,*,#26635,.T.);
#36200=ORIENTED_EDGE('',*,*,#27674,.T.);
#36201=ORIENTED_EDGE('',*,*,#27677,.F.);
#36202=ORIENTED_EDGE('',*,*,#27678,.F.);
#36203=ORIENTED_EDGE('',*,*,#26636,.T.);
#36204=ORIENTED_EDGE('',*,*,#27676,.T.);
#36205=ORIENTED_EDGE('',*,*,#27679,.F.);
#36206=ORIENTED_EDGE('',*,*,#27680,.F.);
#36207=ORIENTED_EDGE('',*,*,#26637,.T.);
#36208=ORIENTED_EDGE('',*,*,#27678,.T.);
#36209=ORIENTED_EDGE('',*,*,#27681,.F.);
#36210=ORIENTED_EDGE('',*,*,#27682,.F.);
#36211=ORIENTED_EDGE('',*,*,#26638,.T.);
#36212=ORIENTED_EDGE('',*,*,#27680,.T.);
#36213=ORIENTED_EDGE('',*,*,#27683,.F.);
#36214=ORIENTED_EDGE('',*,*,#27684,.F.);
#36215=ORIENTED_EDGE('',*,*,#26639,.T.);
#36216=ORIENTED_EDGE('',*,*,#27682,.T.);
#36217=ORIENTED_EDGE('',*,*,#27685,.F.);
#36218=ORIENTED_EDGE('',*,*,#27686,.F.);
#36219=ORIENTED_EDGE('',*,*,#26640,.T.);
#36220=ORIENTED_EDGE('',*,*,#27684,.T.);
#36221=ORIENTED_EDGE('',*,*,#27687,.F.);
#36222=ORIENTED_EDGE('',*,*,#27688,.F.);
#36223=ORIENTED_EDGE('',*,*,#26641,.T.);
#36224=ORIENTED_EDGE('',*,*,#27686,.T.);
#36225=ORIENTED_EDGE('',*,*,#27689,.F.);
#36226=ORIENTED_EDGE('',*,*,#27690,.F.);
#36227=ORIENTED_EDGE('',*,*,#26642,.T.);
#36228=ORIENTED_EDGE('',*,*,#27688,.T.);
#36229=ORIENTED_EDGE('',*,*,#27691,.F.);
#36230=ORIENTED_EDGE('',*,*,#27692,.F.);
#36231=ORIENTED_EDGE('',*,*,#26643,.T.);
#36232=ORIENTED_EDGE('',*,*,#27690,.T.);
#36233=ORIENTED_EDGE('',*,*,#27693,.F.);
#36234=ORIENTED_EDGE('',*,*,#27694,.F.);
#36235=ORIENTED_EDGE('',*,*,#26644,.T.);
#36236=ORIENTED_EDGE('',*,*,#27692,.T.);
#36237=ORIENTED_EDGE('',*,*,#27695,.F.);
#36238=ORIENTED_EDGE('',*,*,#27696,.F.);
#36239=ORIENTED_EDGE('',*,*,#26645,.T.);
#36240=ORIENTED_EDGE('',*,*,#27694,.T.);
#36241=ORIENTED_EDGE('',*,*,#27697,.F.);
#36242=ORIENTED_EDGE('',*,*,#27133,.F.);
#36243=ORIENTED_EDGE('',*,*,#26646,.T.);
#36244=ORIENTED_EDGE('',*,*,#27696,.T.);
#36245=ORIENTED_EDGE('',*,*,#27114,.T.);
#36246=ORIENTED_EDGE('',*,*,#27136,.F.);
#36247=ORIENTED_EDGE('',*,*,#27507,.F.);
#36248=ORIENTED_EDGE('',*,*,#26649,.F.);
#36249=ORIENTED_EDGE('',*,*,#27134,.T.);
#36250=ORIENTED_EDGE('',*,*,#27697,.T.);
#36251=ORIENTED_EDGE('',*,*,#27695,.T.);
#36252=ORIENTED_EDGE('',*,*,#27693,.T.);
#36253=ORIENTED_EDGE('',*,*,#27691,.T.);
#36254=ORIENTED_EDGE('',*,*,#27689,.T.);
#36255=ORIENTED_EDGE('',*,*,#27687,.T.);
#36256=ORIENTED_EDGE('',*,*,#27685,.T.);
#36257=ORIENTED_EDGE('',*,*,#27683,.T.);
#36258=ORIENTED_EDGE('',*,*,#27681,.T.);
#36259=ORIENTED_EDGE('',*,*,#27679,.T.);
#36260=ORIENTED_EDGE('',*,*,#27677,.T.);
#36261=ORIENTED_EDGE('',*,*,#27675,.T.);
#36262=ORIENTED_EDGE('',*,*,#27673,.T.);
#36263=ORIENTED_EDGE('',*,*,#27032,.T.);
#36264=ORIENTED_EDGE('',*,*,#27698,.F.);
#36265=ORIENTED_EDGE('',*,*,#27699,.T.);
#36266=ORIENTED_EDGE('',*,*,#27700,.T.);
#36267=ORIENTED_EDGE('',*,*,#27701,.T.);
#36268=ORIENTED_EDGE('',*,*,#27702,.T.);
#36269=ORIENTED_EDGE('',*,*,#27703,.T.);
#36270=ORIENTED_EDGE('',*,*,#27704,.T.);
#36271=ORIENTED_EDGE('',*,*,#27705,.T.);
#36272=ORIENTED_EDGE('',*,*,#27706,.T.);
#36273=ORIENTED_EDGE('',*,*,#27707,.T.);
#36274=ORIENTED_EDGE('',*,*,#27708,.T.);
#36275=ORIENTED_EDGE('',*,*,#27709,.T.);
#36276=ORIENTED_EDGE('',*,*,#27710,.T.);
#36277=ORIENTED_EDGE('',*,*,#27711,.T.);
#36278=ORIENTED_EDGE('',*,*,#27712,.T.);
#36279=ORIENTED_EDGE('',*,*,#26615,.T.);
#36280=ORIENTED_EDGE('',*,*,#27508,.T.);
#36281=ORIENTED_EDGE('',*,*,#27712,.F.);
#36282=ORIENTED_EDGE('',*,*,#27713,.F.);
#36283=ORIENTED_EDGE('',*,*,#26582,.T.);
#36284=ORIENTED_EDGE('',*,*,#26616,.T.);
#36285=ORIENTED_EDGE('',*,*,#27711,.F.);
#36286=ORIENTED_EDGE('',*,*,#27714,.F.);
#36287=ORIENTED_EDGE('',*,*,#26583,.T.);
#36288=ORIENTED_EDGE('',*,*,#27713,.T.);
#36289=ORIENTED_EDGE('',*,*,#27710,.F.);
#36290=ORIENTED_EDGE('',*,*,#27715,.F.);
#36291=ORIENTED_EDGE('',*,*,#26584,.T.);
#36292=ORIENTED_EDGE('',*,*,#27714,.T.);
#36293=ORIENTED_EDGE('',*,*,#27709,.F.);
#36294=ORIENTED_EDGE('',*,*,#27716,.F.);
#36295=ORIENTED_EDGE('',*,*,#26585,.T.);
#36296=ORIENTED_EDGE('',*,*,#27715,.T.);
#36297=ORIENTED_EDGE('',*,*,#27708,.F.);
#36298=ORIENTED_EDGE('',*,*,#27717,.F.);
#36299=ORIENTED_EDGE('',*,*,#26586,.T.);
#36300=ORIENTED_EDGE('',*,*,#27716,.T.);
#36301=ORIENTED_EDGE('',*,*,#27707,.F.);
#36302=ORIENTED_EDGE('',*,*,#27718,.F.);
#36303=ORIENTED_EDGE('',*,*,#26587,.T.);
#36304=ORIENTED_EDGE('',*,*,#27717,.T.);
#36305=ORIENTED_EDGE('',*,*,#27706,.F.);
#36306=ORIENTED_EDGE('',*,*,#27719,.F.);
#36307=ORIENTED_EDGE('',*,*,#26588,.T.);
#36308=ORIENTED_EDGE('',*,*,#27718,.T.);
#36309=ORIENTED_EDGE('',*,*,#27705,.F.);
#36310=ORIENTED_EDGE('',*,*,#27720,.F.);
#36311=ORIENTED_EDGE('',*,*,#26589,.T.);
#36312=ORIENTED_EDGE('',*,*,#27719,.T.);
#36313=ORIENTED_EDGE('',*,*,#27704,.F.);
#36314=ORIENTED_EDGE('',*,*,#27721,.F.);
#36315=ORIENTED_EDGE('',*,*,#26590,.T.);
#36316=ORIENTED_EDGE('',*,*,#27720,.T.);
#36317=ORIENTED_EDGE('',*,*,#27703,.F.);
#36318=ORIENTED_EDGE('',*,*,#27722,.F.);
#36319=ORIENTED_EDGE('',*,*,#26591,.T.);
#36320=ORIENTED_EDGE('',*,*,#27721,.T.);
#36321=ORIENTED_EDGE('',*,*,#27702,.F.);
#36322=ORIENTED_EDGE('',*,*,#27723,.F.);
#36323=ORIENTED_EDGE('',*,*,#26592,.T.);
#36324=ORIENTED_EDGE('',*,*,#27722,.T.);
#36325=ORIENTED_EDGE('',*,*,#27701,.F.);
#36326=ORIENTED_EDGE('',*,*,#27724,.F.);
#36327=ORIENTED_EDGE('',*,*,#26593,.T.);
#36328=ORIENTED_EDGE('',*,*,#27723,.T.);
#36329=ORIENTED_EDGE('',*,*,#27700,.F.);
#36330=ORIENTED_EDGE('',*,*,#27725,.F.);
#36331=ORIENTED_EDGE('',*,*,#26594,.T.);
#36332=ORIENTED_EDGE('',*,*,#27724,.T.);
#36333=ORIENTED_EDGE('',*,*,#26775,.T.);
#36334=ORIENTED_EDGE('',*,*,#26595,.T.);
#36335=ORIENTED_EDGE('',*,*,#27725,.T.);
#36336=ORIENTED_EDGE('',*,*,#27699,.F.);
#36337=ORIENTED_EDGE('',*,*,#27726,.F.);
#36338=ORIENTED_EDGE('',*,*,#27343,.T.);
#36339=ORIENTED_EDGE('',*,*,#27325,.T.);
#36340=ORIENTED_EDGE('',*,*,#27727,.F.);
#36341=ORIENTED_EDGE('',*,*,#27728,.F.);
#36342=ORIENTED_EDGE('',*,*,#26598,.T.);
#36343=ORIENTED_EDGE('',*,*,#27028,.T.);
#36344=ORIENTED_EDGE('',*,*,#27729,.F.);
#36345=ORIENTED_EDGE('',*,*,#27730,.F.);
#36346=ORIENTED_EDGE('',*,*,#26599,.T.);
#36347=ORIENTED_EDGE('',*,*,#27728,.T.);
#36348=ORIENTED_EDGE('',*,*,#27731,.F.);
#36349=ORIENTED_EDGE('',*,*,#27732,.F.);
#36350=ORIENTED_EDGE('',*,*,#26600,.T.);
#36351=ORIENTED_EDGE('',*,*,#27730,.T.);
#36352=ORIENTED_EDGE('',*,*,#27733,.F.);
#36353=ORIENTED_EDGE('',*,*,#27734,.F.);
#36354=ORIENTED_EDGE('',*,*,#26601,.T.);
#36355=ORIENTED_EDGE('',*,*,#27732,.T.);
#36356=ORIENTED_EDGE('',*,*,#27735,.F.);
#36357=ORIENTED_EDGE('',*,*,#27736,.F.);
#36358=ORIENTED_EDGE('',*,*,#26602,.T.);
#36359=ORIENTED_EDGE('',*,*,#27734,.T.);
#36360=ORIENTED_EDGE('',*,*,#27737,.F.);
#36361=ORIENTED_EDGE('',*,*,#27738,.F.);
#36362=ORIENTED_EDGE('',*,*,#26603,.T.);
#36363=ORIENTED_EDGE('',*,*,#27736,.T.);
#36364=ORIENTED_EDGE('',*,*,#27739,.F.);
#36365=ORIENTED_EDGE('',*,*,#27740,.F.);
#36366=ORIENTED_EDGE('',*,*,#26604,.T.);
#36367=ORIENTED_EDGE('',*,*,#27738,.T.);
#36368=ORIENTED_EDGE('',*,*,#27741,.F.);
#36369=ORIENTED_EDGE('',*,*,#27742,.F.);
#36370=ORIENTED_EDGE('',*,*,#26605,.T.);
#36371=ORIENTED_EDGE('',*,*,#27740,.T.);
#36372=ORIENTED_EDGE('',*,*,#27743,.F.);
#36373=ORIENTED_EDGE('',*,*,#27744,.F.);
#36374=ORIENTED_EDGE('',*,*,#26606,.T.);
#36375=ORIENTED_EDGE('',*,*,#27742,.T.);
#36376=ORIENTED_EDGE('',*,*,#27745,.F.);
#36377=ORIENTED_EDGE('',*,*,#27746,.F.);
#36378=ORIENTED_EDGE('',*,*,#26607,.T.);
#36379=ORIENTED_EDGE('',*,*,#27744,.T.);
#36380=ORIENTED_EDGE('',*,*,#27747,.F.);
#36381=ORIENTED_EDGE('',*,*,#27748,.F.);
#36382=ORIENTED_EDGE('',*,*,#26608,.T.);
#36383=ORIENTED_EDGE('',*,*,#27746,.T.);
#36384=ORIENTED_EDGE('',*,*,#27749,.F.);
#36385=ORIENTED_EDGE('',*,*,#27750,.F.);
#36386=ORIENTED_EDGE('',*,*,#26609,.T.);
#36387=ORIENTED_EDGE('',*,*,#27748,.T.);
#36388=ORIENTED_EDGE('',*,*,#27751,.F.);
#36389=ORIENTED_EDGE('',*,*,#27137,.F.);
#36390=ORIENTED_EDGE('',*,*,#26610,.T.);
#36391=ORIENTED_EDGE('',*,*,#27750,.T.);
#36392=ORIENTED_EDGE('',*,*,#27112,.T.);
#36393=ORIENTED_EDGE('',*,*,#27140,.F.);
#36394=ORIENTED_EDGE('',*,*,#27509,.F.);
#36395=ORIENTED_EDGE('',*,*,#26613,.F.);
#36396=ORIENTED_EDGE('',*,*,#27138,.T.);
#36397=ORIENTED_EDGE('',*,*,#27751,.T.);
#36398=ORIENTED_EDGE('',*,*,#27749,.T.);
#36399=ORIENTED_EDGE('',*,*,#27747,.T.);
#36400=ORIENTED_EDGE('',*,*,#27745,.T.);
#36401=ORIENTED_EDGE('',*,*,#27743,.T.);
#36402=ORIENTED_EDGE('',*,*,#27741,.T.);
#36403=ORIENTED_EDGE('',*,*,#27739,.T.);
#36404=ORIENTED_EDGE('',*,*,#27737,.T.);
#36405=ORIENTED_EDGE('',*,*,#27735,.T.);
#36406=ORIENTED_EDGE('',*,*,#27733,.T.);
#36407=ORIENTED_EDGE('',*,*,#27731,.T.);
#36408=ORIENTED_EDGE('',*,*,#27729,.T.);
#36409=ORIENTED_EDGE('',*,*,#27727,.T.);
#36410=ORIENTED_EDGE('',*,*,#27027,.T.);
#36411=ORIENTED_EDGE('',*,*,#27752,.F.);
#36412=ORIENTED_EDGE('',*,*,#27753,.T.);
#36413=ORIENTED_EDGE('',*,*,#27754,.T.);
#36414=ORIENTED_EDGE('',*,*,#27755,.T.);
#36415=ORIENTED_EDGE('',*,*,#27756,.T.);
#36416=ORIENTED_EDGE('',*,*,#27757,.T.);
#36417=ORIENTED_EDGE('',*,*,#27758,.T.);
#36418=ORIENTED_EDGE('',*,*,#27759,.T.);
#36419=ORIENTED_EDGE('',*,*,#27760,.T.);
#36420=ORIENTED_EDGE('',*,*,#27761,.T.);
#36421=ORIENTED_EDGE('',*,*,#27762,.T.);
#36422=ORIENTED_EDGE('',*,*,#27763,.T.);
#36423=ORIENTED_EDGE('',*,*,#27764,.T.);
#36424=ORIENTED_EDGE('',*,*,#27765,.T.);
#36425=ORIENTED_EDGE('',*,*,#27766,.T.);
#36426=ORIENTED_EDGE('',*,*,#26579,.T.);
#36427=ORIENTED_EDGE('',*,*,#27510,.T.);
#36428=ORIENTED_EDGE('',*,*,#27766,.F.);
#36429=ORIENTED_EDGE('',*,*,#27767,.F.);
#36430=ORIENTED_EDGE('',*,*,#26546,.T.);
#36431=ORIENTED_EDGE('',*,*,#26580,.T.);
#36432=ORIENTED_EDGE('',*,*,#27765,.F.);
#36433=ORIENTED_EDGE('',*,*,#27768,.F.);
#36434=ORIENTED_EDGE('',*,*,#26547,.T.);
#36435=ORIENTED_EDGE('',*,*,#27767,.T.);
#36436=ORIENTED_EDGE('',*,*,#27764,.F.);
#36437=ORIENTED_EDGE('',*,*,#27769,.F.);
#36438=ORIENTED_EDGE('',*,*,#26548,.T.);
#36439=ORIENTED_EDGE('',*,*,#27768,.T.);
#36440=ORIENTED_EDGE('',*,*,#27763,.F.);
#36441=ORIENTED_EDGE('',*,*,#27770,.F.);
#36442=ORIENTED_EDGE('',*,*,#26549,.T.);
#36443=ORIENTED_EDGE('',*,*,#27769,.T.);
#36444=ORIENTED_EDGE('',*,*,#27762,.F.);
#36445=ORIENTED_EDGE('',*,*,#27771,.F.);
#36446=ORIENTED_EDGE('',*,*,#26550,.T.);
#36447=ORIENTED_EDGE('',*,*,#27770,.T.);
#36448=ORIENTED_EDGE('',*,*,#27761,.F.);
#36449=ORIENTED_EDGE('',*,*,#27772,.F.);
#36450=ORIENTED_EDGE('',*,*,#26551,.T.);
#36451=ORIENTED_EDGE('',*,*,#27771,.T.);
#36452=ORIENTED_EDGE('',*,*,#27760,.F.);
#36453=ORIENTED_EDGE('',*,*,#27773,.F.);
#36454=ORIENTED_EDGE('',*,*,#26552,.T.);
#36455=ORIENTED_EDGE('',*,*,#27772,.T.);
#36456=ORIENTED_EDGE('',*,*,#27759,.F.);
#36457=ORIENTED_EDGE('',*,*,#27774,.F.);
#36458=ORIENTED_EDGE('',*,*,#26553,.T.);
#36459=ORIENTED_EDGE('',*,*,#27773,.T.);
#36460=ORIENTED_EDGE('',*,*,#27758,.F.);
#36461=ORIENTED_EDGE('',*,*,#27775,.F.);
#36462=ORIENTED_EDGE('',*,*,#26554,.T.);
#36463=ORIENTED_EDGE('',*,*,#27774,.T.);
#36464=ORIENTED_EDGE('',*,*,#27757,.F.);
#36465=ORIENTED_EDGE('',*,*,#27776,.F.);
#36466=ORIENTED_EDGE('',*,*,#26555,.T.);
#36467=ORIENTED_EDGE('',*,*,#27775,.T.);
#36468=ORIENTED_EDGE('',*,*,#27756,.F.);
#36469=ORIENTED_EDGE('',*,*,#27777,.F.);
#36470=ORIENTED_EDGE('',*,*,#26556,.T.);
#36471=ORIENTED_EDGE('',*,*,#27776,.T.);
#36472=ORIENTED_EDGE('',*,*,#27755,.F.);
#36473=ORIENTED_EDGE('',*,*,#27778,.F.);
#36474=ORIENTED_EDGE('',*,*,#26557,.T.);
#36475=ORIENTED_EDGE('',*,*,#27777,.T.);
#36476=ORIENTED_EDGE('',*,*,#27754,.F.);
#36477=ORIENTED_EDGE('',*,*,#27779,.F.);
#36478=ORIENTED_EDGE('',*,*,#26558,.T.);
#36479=ORIENTED_EDGE('',*,*,#27778,.T.);
#36480=ORIENTED_EDGE('',*,*,#26778,.T.);
#36481=ORIENTED_EDGE('',*,*,#26559,.T.);
#36482=ORIENTED_EDGE('',*,*,#27779,.T.);
#36483=ORIENTED_EDGE('',*,*,#27753,.F.);
#36484=ORIENTED_EDGE('',*,*,#27780,.F.);
#36485=ORIENTED_EDGE('',*,*,#27345,.T.);
#36486=ORIENTED_EDGE('',*,*,#27323,.T.);
#36487=ORIENTED_EDGE('',*,*,#27781,.F.);
#36488=ORIENTED_EDGE('',*,*,#27782,.F.);
#36489=ORIENTED_EDGE('',*,*,#26562,.T.);
#36490=ORIENTED_EDGE('',*,*,#27023,.T.);
#36491=ORIENTED_EDGE('',*,*,#27783,.F.);
#36492=ORIENTED_EDGE('',*,*,#27784,.F.);
#36493=ORIENTED_EDGE('',*,*,#26563,.T.);
#36494=ORIENTED_EDGE('',*,*,#27782,.T.);
#36495=ORIENTED_EDGE('',*,*,#27785,.F.);
#36496=ORIENTED_EDGE('',*,*,#27786,.F.);
#36497=ORIENTED_EDGE('',*,*,#26564,.T.);
#36498=ORIENTED_EDGE('',*,*,#27784,.T.);
#36499=ORIENTED_EDGE('',*,*,#27787,.F.);
#36500=ORIENTED_EDGE('',*,*,#27788,.F.);
#36501=ORIENTED_EDGE('',*,*,#26565,.T.);
#36502=ORIENTED_EDGE('',*,*,#27786,.T.);
#36503=ORIENTED_EDGE('',*,*,#27789,.F.);
#36504=ORIENTED_EDGE('',*,*,#27790,.F.);
#36505=ORIENTED_EDGE('',*,*,#26566,.T.);
#36506=ORIENTED_EDGE('',*,*,#27788,.T.);
#36507=ORIENTED_EDGE('',*,*,#27791,.F.);
#36508=ORIENTED_EDGE('',*,*,#27792,.F.);
#36509=ORIENTED_EDGE('',*,*,#26567,.T.);
#36510=ORIENTED_EDGE('',*,*,#27790,.T.);
#36511=ORIENTED_EDGE('',*,*,#27793,.F.);
#36512=ORIENTED_EDGE('',*,*,#27794,.F.);
#36513=ORIENTED_EDGE('',*,*,#26568,.T.);
#36514=ORIENTED_EDGE('',*,*,#27792,.T.);
#36515=ORIENTED_EDGE('',*,*,#27795,.F.);
#36516=ORIENTED_EDGE('',*,*,#27796,.F.);
#36517=ORIENTED_EDGE('',*,*,#26569,.T.);
#36518=ORIENTED_EDGE('',*,*,#27794,.T.);
#36519=ORIENTED_EDGE('',*,*,#27797,.F.);
#36520=ORIENTED_EDGE('',*,*,#27798,.F.);
#36521=ORIENTED_EDGE('',*,*,#26570,.T.);
#36522=ORIENTED_EDGE('',*,*,#27796,.T.);
#36523=ORIENTED_EDGE('',*,*,#27799,.F.);
#36524=ORIENTED_EDGE('',*,*,#27800,.F.);
#36525=ORIENTED_EDGE('',*,*,#26571,.T.);
#36526=ORIENTED_EDGE('',*,*,#27798,.T.);
#36527=ORIENTED_EDGE('',*,*,#27801,.F.);
#36528=ORIENTED_EDGE('',*,*,#27802,.F.);
#36529=ORIENTED_EDGE('',*,*,#26572,.T.);
#36530=ORIENTED_EDGE('',*,*,#27800,.T.);
#36531=ORIENTED_EDGE('',*,*,#27803,.F.);
#36532=ORIENTED_EDGE('',*,*,#27804,.F.);
#36533=ORIENTED_EDGE('',*,*,#26573,.T.);
#36534=ORIENTED_EDGE('',*,*,#27802,.T.);
#36535=ORIENTED_EDGE('',*,*,#27805,.F.);
#36536=ORIENTED_EDGE('',*,*,#27141,.F.);
#36537=ORIENTED_EDGE('',*,*,#26574,.T.);
#36538=ORIENTED_EDGE('',*,*,#27804,.T.);
#36539=ORIENTED_EDGE('',*,*,#27110,.T.);
#36540=ORIENTED_EDGE('',*,*,#27144,.F.);
#36541=ORIENTED_EDGE('',*,*,#27511,.F.);
#36542=ORIENTED_EDGE('',*,*,#26577,.F.);
#36543=ORIENTED_EDGE('',*,*,#27142,.T.);
#36544=ORIENTED_EDGE('',*,*,#27805,.T.);
#36545=ORIENTED_EDGE('',*,*,#27803,.T.);
#36546=ORIENTED_EDGE('',*,*,#27801,.T.);
#36547=ORIENTED_EDGE('',*,*,#27799,.T.);
#36548=ORIENTED_EDGE('',*,*,#27797,.T.);
#36549=ORIENTED_EDGE('',*,*,#27795,.T.);
#36550=ORIENTED_EDGE('',*,*,#27793,.T.);
#36551=ORIENTED_EDGE('',*,*,#27791,.T.);
#36552=ORIENTED_EDGE('',*,*,#27789,.T.);
#36553=ORIENTED_EDGE('',*,*,#27787,.T.);
#36554=ORIENTED_EDGE('',*,*,#27785,.T.);
#36555=ORIENTED_EDGE('',*,*,#27783,.T.);
#36556=ORIENTED_EDGE('',*,*,#27781,.T.);
#36557=ORIENTED_EDGE('',*,*,#27022,.T.);
#36558=ORIENTED_EDGE('',*,*,#27806,.F.);
#36559=ORIENTED_EDGE('',*,*,#27807,.T.);
#36560=ORIENTED_EDGE('',*,*,#27808,.T.);
#36561=ORIENTED_EDGE('',*,*,#27809,.T.);
#36562=ORIENTED_EDGE('',*,*,#27810,.T.);
#36563=ORIENTED_EDGE('',*,*,#27811,.T.);
#36564=ORIENTED_EDGE('',*,*,#27812,.T.);
#36565=ORIENTED_EDGE('',*,*,#27813,.T.);
#36566=ORIENTED_EDGE('',*,*,#27814,.T.);
#36567=ORIENTED_EDGE('',*,*,#27815,.T.);
#36568=ORIENTED_EDGE('',*,*,#27816,.T.);
#36569=ORIENTED_EDGE('',*,*,#27817,.T.);
#36570=ORIENTED_EDGE('',*,*,#27818,.T.);
#36571=ORIENTED_EDGE('',*,*,#27819,.T.);
#36572=ORIENTED_EDGE('',*,*,#27820,.T.);
#36573=ORIENTED_EDGE('',*,*,#26543,.T.);
#36574=ORIENTED_EDGE('',*,*,#27512,.T.);
#36575=ORIENTED_EDGE('',*,*,#27820,.F.);
#36576=ORIENTED_EDGE('',*,*,#27821,.F.);
#36577=ORIENTED_EDGE('',*,*,#26510,.T.);
#36578=ORIENTED_EDGE('',*,*,#26544,.T.);
#36579=ORIENTED_EDGE('',*,*,#27819,.F.);
#36580=ORIENTED_EDGE('',*,*,#27822,.F.);
#36581=ORIENTED_EDGE('',*,*,#26511,.T.);
#36582=ORIENTED_EDGE('',*,*,#27821,.T.);
#36583=ORIENTED_EDGE('',*,*,#27818,.F.);
#36584=ORIENTED_EDGE('',*,*,#27823,.F.);
#36585=ORIENTED_EDGE('',*,*,#26512,.T.);
#36586=ORIENTED_EDGE('',*,*,#27822,.T.);
#36587=ORIENTED_EDGE('',*,*,#27817,.F.);
#36588=ORIENTED_EDGE('',*,*,#27824,.F.);
#36589=ORIENTED_EDGE('',*,*,#26513,.T.);
#36590=ORIENTED_EDGE('',*,*,#27823,.T.);
#36591=ORIENTED_EDGE('',*,*,#27816,.F.);
#36592=ORIENTED_EDGE('',*,*,#27825,.F.);
#36593=ORIENTED_EDGE('',*,*,#26514,.T.);
#36594=ORIENTED_EDGE('',*,*,#27824,.T.);
#36595=ORIENTED_EDGE('',*,*,#27815,.F.);
#36596=ORIENTED_EDGE('',*,*,#27826,.F.);
#36597=ORIENTED_EDGE('',*,*,#26515,.T.);
#36598=ORIENTED_EDGE('',*,*,#27825,.T.);
#36599=ORIENTED_EDGE('',*,*,#27814,.F.);
#36600=ORIENTED_EDGE('',*,*,#27827,.F.);
#36601=ORIENTED_EDGE('',*,*,#26516,.T.);
#36602=ORIENTED_EDGE('',*,*,#27826,.T.);
#36603=ORIENTED_EDGE('',*,*,#27813,.F.);
#36604=ORIENTED_EDGE('',*,*,#27828,.F.);
#36605=ORIENTED_EDGE('',*,*,#26517,.T.);
#36606=ORIENTED_EDGE('',*,*,#27827,.T.);
#36607=ORIENTED_EDGE('',*,*,#27812,.F.);
#36608=ORIENTED_EDGE('',*,*,#27829,.F.);
#36609=ORIENTED_EDGE('',*,*,#26518,.T.);
#36610=ORIENTED_EDGE('',*,*,#27828,.T.);
#36611=ORIENTED_EDGE('',*,*,#27811,.F.);
#36612=ORIENTED_EDGE('',*,*,#27830,.F.);
#36613=ORIENTED_EDGE('',*,*,#26519,.T.);
#36614=ORIENTED_EDGE('',*,*,#27829,.T.);
#36615=ORIENTED_EDGE('',*,*,#27810,.F.);
#36616=ORIENTED_EDGE('',*,*,#27831,.F.);
#36617=ORIENTED_EDGE('',*,*,#26520,.T.);
#36618=ORIENTED_EDGE('',*,*,#27830,.T.);
#36619=ORIENTED_EDGE('',*,*,#27809,.F.);
#36620=ORIENTED_EDGE('',*,*,#27832,.F.);
#36621=ORIENTED_EDGE('',*,*,#26521,.T.);
#36622=ORIENTED_EDGE('',*,*,#27831,.T.);
#36623=ORIENTED_EDGE('',*,*,#27808,.F.);
#36624=ORIENTED_EDGE('',*,*,#27833,.F.);
#36625=ORIENTED_EDGE('',*,*,#26522,.T.);
#36626=ORIENTED_EDGE('',*,*,#27832,.T.);
#36627=ORIENTED_EDGE('',*,*,#26781,.T.);
#36628=ORIENTED_EDGE('',*,*,#26523,.T.);
#36629=ORIENTED_EDGE('',*,*,#27833,.T.);
#36630=ORIENTED_EDGE('',*,*,#27807,.F.);
#36631=ORIENTED_EDGE('',*,*,#27834,.F.);
#36632=ORIENTED_EDGE('',*,*,#27347,.T.);
#36633=ORIENTED_EDGE('',*,*,#27321,.T.);
#36634=ORIENTED_EDGE('',*,*,#27835,.F.);
#36635=ORIENTED_EDGE('',*,*,#27836,.F.);
#36636=ORIENTED_EDGE('',*,*,#26526,.T.);
#36637=ORIENTED_EDGE('',*,*,#27018,.T.);
#36638=ORIENTED_EDGE('',*,*,#27837,.F.);
#36639=ORIENTED_EDGE('',*,*,#27838,.F.);
#36640=ORIENTED_EDGE('',*,*,#26527,.T.);
#36641=ORIENTED_EDGE('',*,*,#27836,.T.);
#36642=ORIENTED_EDGE('',*,*,#27839,.F.);
#36643=ORIENTED_EDGE('',*,*,#27840,.F.);
#36644=ORIENTED_EDGE('',*,*,#26528,.T.);
#36645=ORIENTED_EDGE('',*,*,#27838,.T.);
#36646=ORIENTED_EDGE('',*,*,#27841,.F.);
#36647=ORIENTED_EDGE('',*,*,#27842,.F.);
#36648=ORIENTED_EDGE('',*,*,#26529,.T.);
#36649=ORIENTED_EDGE('',*,*,#27840,.T.);
#36650=ORIENTED_EDGE('',*,*,#27843,.F.);
#36651=ORIENTED_EDGE('',*,*,#27844,.F.);
#36652=ORIENTED_EDGE('',*,*,#26530,.T.);
#36653=ORIENTED_EDGE('',*,*,#27842,.T.);
#36654=ORIENTED_EDGE('',*,*,#27845,.F.);
#36655=ORIENTED_EDGE('',*,*,#27846,.F.);
#36656=ORIENTED_EDGE('',*,*,#26531,.T.);
#36657=ORIENTED_EDGE('',*,*,#27844,.T.);
#36658=ORIENTED_EDGE('',*,*,#27847,.F.);
#36659=ORIENTED_EDGE('',*,*,#27848,.F.);
#36660=ORIENTED_EDGE('',*,*,#26532,.T.);
#36661=ORIENTED_EDGE('',*,*,#27846,.T.);
#36662=ORIENTED_EDGE('',*,*,#27849,.F.);
#36663=ORIENTED_EDGE('',*,*,#27850,.F.);
#36664=ORIENTED_EDGE('',*,*,#26533,.T.);
#36665=ORIENTED_EDGE('',*,*,#27848,.T.);
#36666=ORIENTED_EDGE('',*,*,#27851,.F.);
#36667=ORIENTED_EDGE('',*,*,#27852,.F.);
#36668=ORIENTED_EDGE('',*,*,#26534,.T.);
#36669=ORIENTED_EDGE('',*,*,#27850,.T.);
#36670=ORIENTED_EDGE('',*,*,#27853,.F.);
#36671=ORIENTED_EDGE('',*,*,#27854,.F.);
#36672=ORIENTED_EDGE('',*,*,#26535,.T.);
#36673=ORIENTED_EDGE('',*,*,#27852,.T.);
#36674=ORIENTED_EDGE('',*,*,#27855,.F.);
#36675=ORIENTED_EDGE('',*,*,#27856,.F.);
#36676=ORIENTED_EDGE('',*,*,#26536,.T.);
#36677=ORIENTED_EDGE('',*,*,#27854,.T.);
#36678=ORIENTED_EDGE('',*,*,#27857,.F.);
#36679=ORIENTED_EDGE('',*,*,#27858,.F.);
#36680=ORIENTED_EDGE('',*,*,#26537,.T.);
#36681=ORIENTED_EDGE('',*,*,#27856,.T.);
#36682=ORIENTED_EDGE('',*,*,#27859,.F.);
#36683=ORIENTED_EDGE('',*,*,#27145,.F.);
#36684=ORIENTED_EDGE('',*,*,#26538,.T.);
#36685=ORIENTED_EDGE('',*,*,#27858,.T.);
#36686=ORIENTED_EDGE('',*,*,#27108,.T.);
#36687=ORIENTED_EDGE('',*,*,#27148,.F.);
#36688=ORIENTED_EDGE('',*,*,#27513,.F.);
#36689=ORIENTED_EDGE('',*,*,#26541,.F.);
#36690=ORIENTED_EDGE('',*,*,#27146,.T.);
#36691=ORIENTED_EDGE('',*,*,#27859,.T.);
#36692=ORIENTED_EDGE('',*,*,#27857,.T.);
#36693=ORIENTED_EDGE('',*,*,#27855,.T.);
#36694=ORIENTED_EDGE('',*,*,#27853,.T.);
#36695=ORIENTED_EDGE('',*,*,#27851,.T.);
#36696=ORIENTED_EDGE('',*,*,#27849,.T.);
#36697=ORIENTED_EDGE('',*,*,#27847,.T.);
#36698=ORIENTED_EDGE('',*,*,#27845,.T.);
#36699=ORIENTED_EDGE('',*,*,#27843,.T.);
#36700=ORIENTED_EDGE('',*,*,#27841,.T.);
#36701=ORIENTED_EDGE('',*,*,#27839,.T.);
#36702=ORIENTED_EDGE('',*,*,#27837,.T.);
#36703=ORIENTED_EDGE('',*,*,#27835,.T.);
#36704=ORIENTED_EDGE('',*,*,#27017,.T.);
#36705=ORIENTED_EDGE('',*,*,#27860,.F.);
#36706=ORIENTED_EDGE('',*,*,#27861,.T.);
#36707=ORIENTED_EDGE('',*,*,#27862,.T.);
#36708=ORIENTED_EDGE('',*,*,#27863,.T.);
#36709=ORIENTED_EDGE('',*,*,#27864,.T.);
#36710=ORIENTED_EDGE('',*,*,#27865,.T.);
#36711=ORIENTED_EDGE('',*,*,#27866,.T.);
#36712=ORIENTED_EDGE('',*,*,#27867,.T.);
#36713=ORIENTED_EDGE('',*,*,#27868,.T.);
#36714=ORIENTED_EDGE('',*,*,#27869,.T.);
#36715=ORIENTED_EDGE('',*,*,#27870,.T.);
#36716=ORIENTED_EDGE('',*,*,#27871,.T.);
#36717=ORIENTED_EDGE('',*,*,#27872,.T.);
#36718=ORIENTED_EDGE('',*,*,#27873,.T.);
#36719=ORIENTED_EDGE('',*,*,#27874,.T.);
#36720=ORIENTED_EDGE('',*,*,#26507,.T.);
#36721=ORIENTED_EDGE('',*,*,#27514,.T.);
#36722=ORIENTED_EDGE('',*,*,#27874,.F.);
#36723=ORIENTED_EDGE('',*,*,#27875,.F.);
#36724=ORIENTED_EDGE('',*,*,#26474,.T.);
#36725=ORIENTED_EDGE('',*,*,#26508,.T.);
#36726=ORIENTED_EDGE('',*,*,#27873,.F.);
#36727=ORIENTED_EDGE('',*,*,#27876,.F.);
#36728=ORIENTED_EDGE('',*,*,#26475,.T.);
#36729=ORIENTED_EDGE('',*,*,#27875,.T.);
#36730=ORIENTED_EDGE('',*,*,#27872,.F.);
#36731=ORIENTED_EDGE('',*,*,#27877,.F.);
#36732=ORIENTED_EDGE('',*,*,#26476,.T.);
#36733=ORIENTED_EDGE('',*,*,#27876,.T.);
#36734=ORIENTED_EDGE('',*,*,#27871,.F.);
#36735=ORIENTED_EDGE('',*,*,#27878,.F.);
#36736=ORIENTED_EDGE('',*,*,#26477,.T.);
#36737=ORIENTED_EDGE('',*,*,#27877,.T.);
#36738=ORIENTED_EDGE('',*,*,#27870,.F.);
#36739=ORIENTED_EDGE('',*,*,#27879,.F.);
#36740=ORIENTED_EDGE('',*,*,#26478,.T.);
#36741=ORIENTED_EDGE('',*,*,#27878,.T.);
#36742=ORIENTED_EDGE('',*,*,#27869,.F.);
#36743=ORIENTED_EDGE('',*,*,#27880,.F.);
#36744=ORIENTED_EDGE('',*,*,#26479,.T.);
#36745=ORIENTED_EDGE('',*,*,#27879,.T.);
#36746=ORIENTED_EDGE('',*,*,#27868,.F.);
#36747=ORIENTED_EDGE('',*,*,#27881,.F.);
#36748=ORIENTED_EDGE('',*,*,#26480,.T.);
#36749=ORIENTED_EDGE('',*,*,#27880,.T.);
#36750=ORIENTED_EDGE('',*,*,#27867,.F.);
#36751=ORIENTED_EDGE('',*,*,#27882,.F.);
#36752=ORIENTED_EDGE('',*,*,#26481,.T.);
#36753=ORIENTED_EDGE('',*,*,#27881,.T.);
#36754=ORIENTED_EDGE('',*,*,#27866,.F.);
#36755=ORIENTED_EDGE('',*,*,#27883,.F.);
#36756=ORIENTED_EDGE('',*,*,#26482,.T.);
#36757=ORIENTED_EDGE('',*,*,#27882,.T.);
#36758=ORIENTED_EDGE('',*,*,#27865,.F.);
#36759=ORIENTED_EDGE('',*,*,#27884,.F.);
#36760=ORIENTED_EDGE('',*,*,#26483,.T.);
#36761=ORIENTED_EDGE('',*,*,#27883,.T.);
#36762=ORIENTED_EDGE('',*,*,#27864,.F.);
#36763=ORIENTED_EDGE('',*,*,#27885,.F.);
#36764=ORIENTED_EDGE('',*,*,#26484,.T.);
#36765=ORIENTED_EDGE('',*,*,#27884,.T.);
#36766=ORIENTED_EDGE('',*,*,#27863,.F.);
#36767=ORIENTED_EDGE('',*,*,#27886,.F.);
#36768=ORIENTED_EDGE('',*,*,#26485,.T.);
#36769=ORIENTED_EDGE('',*,*,#27885,.T.);
#36770=ORIENTED_EDGE('',*,*,#27862,.F.);
#36771=ORIENTED_EDGE('',*,*,#27887,.F.);
#36772=ORIENTED_EDGE('',*,*,#26486,.T.);
#36773=ORIENTED_EDGE('',*,*,#27886,.T.);
#36774=ORIENTED_EDGE('',*,*,#26784,.T.);
#36775=ORIENTED_EDGE('',*,*,#26487,.T.);
#36776=ORIENTED_EDGE('',*,*,#27887,.T.);
#36777=ORIENTED_EDGE('',*,*,#27861,.F.);
#36778=ORIENTED_EDGE('',*,*,#27888,.F.);
#36779=ORIENTED_EDGE('',*,*,#27349,.T.);
#36780=ORIENTED_EDGE('',*,*,#27319,.T.);
#36781=ORIENTED_EDGE('',*,*,#27889,.F.);
#36782=ORIENTED_EDGE('',*,*,#27890,.F.);
#36783=ORIENTED_EDGE('',*,*,#26490,.T.);
#36784=ORIENTED_EDGE('',*,*,#27013,.T.);
#36785=ORIENTED_EDGE('',*,*,#27891,.F.);
#36786=ORIENTED_EDGE('',*,*,#27892,.F.);
#36787=ORIENTED_EDGE('',*,*,#26491,.T.);
#36788=ORIENTED_EDGE('',*,*,#27890,.T.);
#36789=ORIENTED_EDGE('',*,*,#27893,.F.);
#36790=ORIENTED_EDGE('',*,*,#27894,.F.);
#36791=ORIENTED_EDGE('',*,*,#26492,.T.);
#36792=ORIENTED_EDGE('',*,*,#27892,.T.);
#36793=ORIENTED_EDGE('',*,*,#27895,.F.);
#36794=ORIENTED_EDGE('',*,*,#27896,.F.);
#36795=ORIENTED_EDGE('',*,*,#26493,.T.);
#36796=ORIENTED_EDGE('',*,*,#27894,.T.);
#36797=ORIENTED_EDGE('',*,*,#27897,.F.);
#36798=ORIENTED_EDGE('',*,*,#27898,.F.);
#36799=ORIENTED_EDGE('',*,*,#26494,.T.);
#36800=ORIENTED_EDGE('',*,*,#27896,.T.);
#36801=ORIENTED_EDGE('',*,*,#27899,.F.);
#36802=ORIENTED_EDGE('',*,*,#27900,.F.);
#36803=ORIENTED_EDGE('',*,*,#26495,.T.);
#36804=ORIENTED_EDGE('',*,*,#27898,.T.);
#36805=ORIENTED_EDGE('',*,*,#27901,.F.);
#36806=ORIENTED_EDGE('',*,*,#27902,.F.);
#36807=ORIENTED_EDGE('',*,*,#26496,.T.);
#36808=ORIENTED_EDGE('',*,*,#27900,.T.);
#36809=ORIENTED_EDGE('',*,*,#27903,.F.);
#36810=ORIENTED_EDGE('',*,*,#27904,.F.);
#36811=ORIENTED_EDGE('',*,*,#26497,.T.);
#36812=ORIENTED_EDGE('',*,*,#27902,.T.);
#36813=ORIENTED_EDGE('',*,*,#27905,.F.);
#36814=ORIENTED_EDGE('',*,*,#27906,.F.);
#36815=ORIENTED_EDGE('',*,*,#26498,.T.);
#36816=ORIENTED_EDGE('',*,*,#27904,.T.);
#36817=ORIENTED_EDGE('',*,*,#27907,.F.);
#36818=ORIENTED_EDGE('',*,*,#27908,.F.);
#36819=ORIENTED_EDGE('',*,*,#26499,.T.);
#36820=ORIENTED_EDGE('',*,*,#27906,.T.);
#36821=ORIENTED_EDGE('',*,*,#27909,.F.);
#36822=ORIENTED_EDGE('',*,*,#27910,.F.);
#36823=ORIENTED_EDGE('',*,*,#26500,.T.);
#36824=ORIENTED_EDGE('',*,*,#27908,.T.);
#36825=ORIENTED_EDGE('',*,*,#27911,.F.);
#36826=ORIENTED_EDGE('',*,*,#27912,.F.);
#36827=ORIENTED_EDGE('',*,*,#26501,.T.);
#36828=ORIENTED_EDGE('',*,*,#27910,.T.);
#36829=ORIENTED_EDGE('',*,*,#27913,.F.);
#36830=ORIENTED_EDGE('',*,*,#27149,.F.);
#36831=ORIENTED_EDGE('',*,*,#26502,.T.);
#36832=ORIENTED_EDGE('',*,*,#27912,.T.);
#36833=ORIENTED_EDGE('',*,*,#27106,.T.);
#36834=ORIENTED_EDGE('',*,*,#27152,.F.);
#36835=ORIENTED_EDGE('',*,*,#27515,.F.);
#36836=ORIENTED_EDGE('',*,*,#26505,.F.);
#36837=ORIENTED_EDGE('',*,*,#27150,.T.);
#36838=ORIENTED_EDGE('',*,*,#27913,.T.);
#36839=ORIENTED_EDGE('',*,*,#27911,.T.);
#36840=ORIENTED_EDGE('',*,*,#27909,.T.);
#36841=ORIENTED_EDGE('',*,*,#27907,.T.);
#36842=ORIENTED_EDGE('',*,*,#27905,.T.);
#36843=ORIENTED_EDGE('',*,*,#27903,.T.);
#36844=ORIENTED_EDGE('',*,*,#27901,.T.);
#36845=ORIENTED_EDGE('',*,*,#27899,.T.);
#36846=ORIENTED_EDGE('',*,*,#27897,.T.);
#36847=ORIENTED_EDGE('',*,*,#27895,.T.);
#36848=ORIENTED_EDGE('',*,*,#27893,.T.);
#36849=ORIENTED_EDGE('',*,*,#27891,.T.);
#36850=ORIENTED_EDGE('',*,*,#27889,.T.);
#36851=ORIENTED_EDGE('',*,*,#27012,.T.);
#36852=ORIENTED_EDGE('',*,*,#27914,.F.);
#36853=ORIENTED_EDGE('',*,*,#27915,.T.);
#36854=ORIENTED_EDGE('',*,*,#27916,.T.);
#36855=ORIENTED_EDGE('',*,*,#27917,.T.);
#36856=ORIENTED_EDGE('',*,*,#27918,.T.);
#36857=ORIENTED_EDGE('',*,*,#27919,.T.);
#36858=ORIENTED_EDGE('',*,*,#27920,.T.);
#36859=ORIENTED_EDGE('',*,*,#27921,.T.);
#36860=ORIENTED_EDGE('',*,*,#27922,.T.);
#36861=ORIENTED_EDGE('',*,*,#27923,.T.);
#36862=ORIENTED_EDGE('',*,*,#27924,.T.);
#36863=ORIENTED_EDGE('',*,*,#27925,.T.);
#36864=ORIENTED_EDGE('',*,*,#27926,.T.);
#36865=ORIENTED_EDGE('',*,*,#27927,.T.);
#36866=ORIENTED_EDGE('',*,*,#27928,.T.);
#36867=ORIENTED_EDGE('',*,*,#26471,.T.);
#36868=ORIENTED_EDGE('',*,*,#27516,.T.);
#36869=ORIENTED_EDGE('',*,*,#27928,.F.);
#36870=ORIENTED_EDGE('',*,*,#27929,.F.);
#36871=ORIENTED_EDGE('',*,*,#26438,.T.);
#36872=ORIENTED_EDGE('',*,*,#26472,.T.);
#36873=ORIENTED_EDGE('',*,*,#27927,.F.);
#36874=ORIENTED_EDGE('',*,*,#27930,.F.);
#36875=ORIENTED_EDGE('',*,*,#26439,.T.);
#36876=ORIENTED_EDGE('',*,*,#27929,.T.);
#36877=ORIENTED_EDGE('',*,*,#27926,.F.);
#36878=ORIENTED_EDGE('',*,*,#27931,.F.);
#36879=ORIENTED_EDGE('',*,*,#26440,.T.);
#36880=ORIENTED_EDGE('',*,*,#27930,.T.);
#36881=ORIENTED_EDGE('',*,*,#27925,.F.);
#36882=ORIENTED_EDGE('',*,*,#27932,.F.);
#36883=ORIENTED_EDGE('',*,*,#26441,.T.);
#36884=ORIENTED_EDGE('',*,*,#27931,.T.);
#36885=ORIENTED_EDGE('',*,*,#27924,.F.);
#36886=ORIENTED_EDGE('',*,*,#27933,.F.);
#36887=ORIENTED_EDGE('',*,*,#26442,.T.);
#36888=ORIENTED_EDGE('',*,*,#27932,.T.);
#36889=ORIENTED_EDGE('',*,*,#27923,.F.);
#36890=ORIENTED_EDGE('',*,*,#27934,.F.);
#36891=ORIENTED_EDGE('',*,*,#26443,.T.);
#36892=ORIENTED_EDGE('',*,*,#27933,.T.);
#36893=ORIENTED_EDGE('',*,*,#27922,.F.);
#36894=ORIENTED_EDGE('',*,*,#27935,.F.);
#36895=ORIENTED_EDGE('',*,*,#26444,.T.);
#36896=ORIENTED_EDGE('',*,*,#27934,.T.);
#36897=ORIENTED_EDGE('',*,*,#27921,.F.);
#36898=ORIENTED_EDGE('',*,*,#27936,.F.);
#36899=ORIENTED_EDGE('',*,*,#26445,.T.);
#36900=ORIENTED_EDGE('',*,*,#27935,.T.);
#36901=ORIENTED_EDGE('',*,*,#27920,.F.);
#36902=ORIENTED_EDGE('',*,*,#27937,.F.);
#36903=ORIENTED_EDGE('',*,*,#26446,.T.);
#36904=ORIENTED_EDGE('',*,*,#27936,.T.);
#36905=ORIENTED_EDGE('',*,*,#27919,.F.);
#36906=ORIENTED_EDGE('',*,*,#27938,.F.);
#36907=ORIENTED_EDGE('',*,*,#26447,.T.);
#36908=ORIENTED_EDGE('',*,*,#27937,.T.);
#36909=ORIENTED_EDGE('',*,*,#27918,.F.);
#36910=ORIENTED_EDGE('',*,*,#27939,.F.);
#36911=ORIENTED_EDGE('',*,*,#26448,.T.);
#36912=ORIENTED_EDGE('',*,*,#27938,.T.);
#36913=ORIENTED_EDGE('',*,*,#27917,.F.);
#36914=ORIENTED_EDGE('',*,*,#27940,.F.);
#36915=ORIENTED_EDGE('',*,*,#26449,.T.);
#36916=ORIENTED_EDGE('',*,*,#27939,.T.);
#36917=ORIENTED_EDGE('',*,*,#27916,.F.);
#36918=ORIENTED_EDGE('',*,*,#27941,.F.);
#36919=ORIENTED_EDGE('',*,*,#26450,.T.);
#36920=ORIENTED_EDGE('',*,*,#27940,.T.);
#36921=ORIENTED_EDGE('',*,*,#26787,.T.);
#36922=ORIENTED_EDGE('',*,*,#26451,.T.);
#36923=ORIENTED_EDGE('',*,*,#27941,.T.);
#36924=ORIENTED_EDGE('',*,*,#27915,.F.);
#36925=ORIENTED_EDGE('',*,*,#27942,.F.);
#36926=ORIENTED_EDGE('',*,*,#27351,.T.);
#36927=ORIENTED_EDGE('',*,*,#27317,.T.);
#36928=ORIENTED_EDGE('',*,*,#27943,.F.);
#36929=ORIENTED_EDGE('',*,*,#27944,.F.);
#36930=ORIENTED_EDGE('',*,*,#26454,.T.);
#36931=ORIENTED_EDGE('',*,*,#27008,.T.);
#36932=ORIENTED_EDGE('',*,*,#27945,.F.);
#36933=ORIENTED_EDGE('',*,*,#27946,.F.);
#36934=ORIENTED_EDGE('',*,*,#26455,.T.);
#36935=ORIENTED_EDGE('',*,*,#27944,.T.);
#36936=ORIENTED_EDGE('',*,*,#27947,.F.);
#36937=ORIENTED_EDGE('',*,*,#27948,.F.);
#36938=ORIENTED_EDGE('',*,*,#26456,.T.);
#36939=ORIENTED_EDGE('',*,*,#27946,.T.);
#36940=ORIENTED_EDGE('',*,*,#27949,.F.);
#36941=ORIENTED_EDGE('',*,*,#27950,.F.);
#36942=ORIENTED_EDGE('',*,*,#26457,.T.);
#36943=ORIENTED_EDGE('',*,*,#27948,.T.);
#36944=ORIENTED_EDGE('',*,*,#27951,.F.);
#36945=ORIENTED_EDGE('',*,*,#27952,.F.);
#36946=ORIENTED_EDGE('',*,*,#26458,.T.);
#36947=ORIENTED_EDGE('',*,*,#27950,.T.);
#36948=ORIENTED_EDGE('',*,*,#27953,.F.);
#36949=ORIENTED_EDGE('',*,*,#27954,.F.);
#36950=ORIENTED_EDGE('',*,*,#26459,.T.);
#36951=ORIENTED_EDGE('',*,*,#27952,.T.);
#36952=ORIENTED_EDGE('',*,*,#27955,.F.);
#36953=ORIENTED_EDGE('',*,*,#27956,.F.);
#36954=ORIENTED_EDGE('',*,*,#26460,.T.);
#36955=ORIENTED_EDGE('',*,*,#27954,.T.);
#36956=ORIENTED_EDGE('',*,*,#27957,.F.);
#36957=ORIENTED_EDGE('',*,*,#27958,.F.);
#36958=ORIENTED_EDGE('',*,*,#26461,.T.);
#36959=ORIENTED_EDGE('',*,*,#27956,.T.);
#36960=ORIENTED_EDGE('',*,*,#27959,.F.);
#36961=ORIENTED_EDGE('',*,*,#27960,.F.);
#36962=ORIENTED_EDGE('',*,*,#26462,.T.);
#36963=ORIENTED_EDGE('',*,*,#27958,.T.);
#36964=ORIENTED_EDGE('',*,*,#27961,.F.);
#36965=ORIENTED_EDGE('',*,*,#27962,.F.);
#36966=ORIENTED_EDGE('',*,*,#26463,.T.);
#36967=ORIENTED_EDGE('',*,*,#27960,.T.);
#36968=ORIENTED_EDGE('',*,*,#27963,.F.);
#36969=ORIENTED_EDGE('',*,*,#27964,.F.);
#36970=ORIENTED_EDGE('',*,*,#26464,.T.);
#36971=ORIENTED_EDGE('',*,*,#27962,.T.);
#36972=ORIENTED_EDGE('',*,*,#27965,.F.);
#36973=ORIENTED_EDGE('',*,*,#27966,.F.);
#36974=ORIENTED_EDGE('',*,*,#26465,.T.);
#36975=ORIENTED_EDGE('',*,*,#27964,.T.);
#36976=ORIENTED_EDGE('',*,*,#27967,.F.);
#36977=ORIENTED_EDGE('',*,*,#27153,.F.);
#36978=ORIENTED_EDGE('',*,*,#26466,.T.);
#36979=ORIENTED_EDGE('',*,*,#27966,.T.);
#36980=ORIENTED_EDGE('',*,*,#27104,.T.);
#36981=ORIENTED_EDGE('',*,*,#27156,.F.);
#36982=ORIENTED_EDGE('',*,*,#27517,.F.);
#36983=ORIENTED_EDGE('',*,*,#26469,.F.);
#36984=ORIENTED_EDGE('',*,*,#27154,.T.);
#36985=ORIENTED_EDGE('',*,*,#27967,.T.);
#36986=ORIENTED_EDGE('',*,*,#27965,.T.);
#36987=ORIENTED_EDGE('',*,*,#27963,.T.);
#36988=ORIENTED_EDGE('',*,*,#27961,.T.);
#36989=ORIENTED_EDGE('',*,*,#27959,.T.);
#36990=ORIENTED_EDGE('',*,*,#27957,.T.);
#36991=ORIENTED_EDGE('',*,*,#27955,.T.);
#36992=ORIENTED_EDGE('',*,*,#27953,.T.);
#36993=ORIENTED_EDGE('',*,*,#27951,.T.);
#36994=ORIENTED_EDGE('',*,*,#27949,.T.);
#36995=ORIENTED_EDGE('',*,*,#27947,.T.);
#36996=ORIENTED_EDGE('',*,*,#27945,.T.);
#36997=ORIENTED_EDGE('',*,*,#27943,.T.);
#36998=ORIENTED_EDGE('',*,*,#27007,.T.);
#36999=ORIENTED_EDGE('',*,*,#27968,.F.);
#37000=ORIENTED_EDGE('',*,*,#27969,.T.);
#37001=ORIENTED_EDGE('',*,*,#27970,.T.);
#37002=ORIENTED_EDGE('',*,*,#27971,.T.);
#37003=ORIENTED_EDGE('',*,*,#27972,.T.);
#37004=ORIENTED_EDGE('',*,*,#27973,.T.);
#37005=ORIENTED_EDGE('',*,*,#27974,.T.);
#37006=ORIENTED_EDGE('',*,*,#27975,.T.);
#37007=ORIENTED_EDGE('',*,*,#27976,.T.);
#37008=ORIENTED_EDGE('',*,*,#27977,.T.);
#37009=ORIENTED_EDGE('',*,*,#27978,.T.);
#37010=ORIENTED_EDGE('',*,*,#27979,.T.);
#37011=ORIENTED_EDGE('',*,*,#27980,.T.);
#37012=ORIENTED_EDGE('',*,*,#27981,.T.);
#37013=ORIENTED_EDGE('',*,*,#27982,.T.);
#37014=ORIENTED_EDGE('',*,*,#26435,.T.);
#37015=ORIENTED_EDGE('',*,*,#27518,.T.);
#37016=ORIENTED_EDGE('',*,*,#27982,.F.);
#37017=ORIENTED_EDGE('',*,*,#27983,.F.);
#37018=ORIENTED_EDGE('',*,*,#26402,.T.);
#37019=ORIENTED_EDGE('',*,*,#26436,.T.);
#37020=ORIENTED_EDGE('',*,*,#27981,.F.);
#37021=ORIENTED_EDGE('',*,*,#27984,.F.);
#37022=ORIENTED_EDGE('',*,*,#26403,.T.);
#37023=ORIENTED_EDGE('',*,*,#27983,.T.);
#37024=ORIENTED_EDGE('',*,*,#27980,.F.);
#37025=ORIENTED_EDGE('',*,*,#27985,.F.);
#37026=ORIENTED_EDGE('',*,*,#26404,.T.);
#37027=ORIENTED_EDGE('',*,*,#27984,.T.);
#37028=ORIENTED_EDGE('',*,*,#27979,.F.);
#37029=ORIENTED_EDGE('',*,*,#27986,.F.);
#37030=ORIENTED_EDGE('',*,*,#26405,.T.);
#37031=ORIENTED_EDGE('',*,*,#27985,.T.);
#37032=ORIENTED_EDGE('',*,*,#27978,.F.);
#37033=ORIENTED_EDGE('',*,*,#27987,.F.);
#37034=ORIENTED_EDGE('',*,*,#26406,.T.);
#37035=ORIENTED_EDGE('',*,*,#27986,.T.);
#37036=ORIENTED_EDGE('',*,*,#27977,.F.);
#37037=ORIENTED_EDGE('',*,*,#27988,.F.);
#37038=ORIENTED_EDGE('',*,*,#26407,.T.);
#37039=ORIENTED_EDGE('',*,*,#27987,.T.);
#37040=ORIENTED_EDGE('',*,*,#27976,.F.);
#37041=ORIENTED_EDGE('',*,*,#27989,.F.);
#37042=ORIENTED_EDGE('',*,*,#26408,.T.);
#37043=ORIENTED_EDGE('',*,*,#27988,.T.);
#37044=ORIENTED_EDGE('',*,*,#27975,.F.);
#37045=ORIENTED_EDGE('',*,*,#27990,.F.);
#37046=ORIENTED_EDGE('',*,*,#26409,.T.);
#37047=ORIENTED_EDGE('',*,*,#27989,.T.);
#37048=ORIENTED_EDGE('',*,*,#27974,.F.);
#37049=ORIENTED_EDGE('',*,*,#27991,.F.);
#37050=ORIENTED_EDGE('',*,*,#26410,.T.);
#37051=ORIENTED_EDGE('',*,*,#27990,.T.);
#37052=ORIENTED_EDGE('',*,*,#27973,.F.);
#37053=ORIENTED_EDGE('',*,*,#27992,.F.);
#37054=ORIENTED_EDGE('',*,*,#26411,.T.);
#37055=ORIENTED_EDGE('',*,*,#27991,.T.);
#37056=ORIENTED_EDGE('',*,*,#27972,.F.);
#37057=ORIENTED_EDGE('',*,*,#27993,.F.);
#37058=ORIENTED_EDGE('',*,*,#26412,.T.);
#37059=ORIENTED_EDGE('',*,*,#27992,.T.);
#37060=ORIENTED_EDGE('',*,*,#27971,.F.);
#37061=ORIENTED_EDGE('',*,*,#27994,.F.);
#37062=ORIENTED_EDGE('',*,*,#26413,.T.);
#37063=ORIENTED_EDGE('',*,*,#27993,.T.);
#37064=ORIENTED_EDGE('',*,*,#27970,.F.);
#37065=ORIENTED_EDGE('',*,*,#27995,.F.);
#37066=ORIENTED_EDGE('',*,*,#26414,.T.);
#37067=ORIENTED_EDGE('',*,*,#27994,.T.);
#37068=ORIENTED_EDGE('',*,*,#26790,.T.);
#37069=ORIENTED_EDGE('',*,*,#26415,.T.);
#37070=ORIENTED_EDGE('',*,*,#27995,.T.);
#37071=ORIENTED_EDGE('',*,*,#27969,.F.);
#37072=ORIENTED_EDGE('',*,*,#27996,.F.);
#37073=ORIENTED_EDGE('',*,*,#27353,.T.);
#37074=ORIENTED_EDGE('',*,*,#27315,.T.);
#37075=ORIENTED_EDGE('',*,*,#27997,.F.);
#37076=ORIENTED_EDGE('',*,*,#27998,.F.);
#37077=ORIENTED_EDGE('',*,*,#26418,.T.);
#37078=ORIENTED_EDGE('',*,*,#27003,.T.);
#37079=ORIENTED_EDGE('',*,*,#27999,.F.);
#37080=ORIENTED_EDGE('',*,*,#28000,.F.);
#37081=ORIENTED_EDGE('',*,*,#26419,.T.);
#37082=ORIENTED_EDGE('',*,*,#27998,.T.);
#37083=ORIENTED_EDGE('',*,*,#28001,.F.);
#37084=ORIENTED_EDGE('',*,*,#28002,.F.);
#37085=ORIENTED_EDGE('',*,*,#26420,.T.);
#37086=ORIENTED_EDGE('',*,*,#28000,.T.);
#37087=ORIENTED_EDGE('',*,*,#28003,.F.);
#37088=ORIENTED_EDGE('',*,*,#28004,.F.);
#37089=ORIENTED_EDGE('',*,*,#26421,.T.);
#37090=ORIENTED_EDGE('',*,*,#28002,.T.);
#37091=ORIENTED_EDGE('',*,*,#28005,.F.);
#37092=ORIENTED_EDGE('',*,*,#28006,.F.);
#37093=ORIENTED_EDGE('',*,*,#26422,.T.);
#37094=ORIENTED_EDGE('',*,*,#28004,.T.);
#37095=ORIENTED_EDGE('',*,*,#28007,.F.);
#37096=ORIENTED_EDGE('',*,*,#28008,.F.);
#37097=ORIENTED_EDGE('',*,*,#26423,.T.);
#37098=ORIENTED_EDGE('',*,*,#28006,.T.);
#37099=ORIENTED_EDGE('',*,*,#28009,.F.);
#37100=ORIENTED_EDGE('',*,*,#28010,.F.);
#37101=ORIENTED_EDGE('',*,*,#26424,.T.);
#37102=ORIENTED_EDGE('',*,*,#28008,.T.);
#37103=ORIENTED_EDGE('',*,*,#28011,.F.);
#37104=ORIENTED_EDGE('',*,*,#28012,.F.);
#37105=ORIENTED_EDGE('',*,*,#26425,.T.);
#37106=ORIENTED_EDGE('',*,*,#28010,.T.);
#37107=ORIENTED_EDGE('',*,*,#28013,.F.);
#37108=ORIENTED_EDGE('',*,*,#28014,.F.);
#37109=ORIENTED_EDGE('',*,*,#26426,.T.);
#37110=ORIENTED_EDGE('',*,*,#28012,.T.);
#37111=ORIENTED_EDGE('',*,*,#28015,.F.);
#37112=ORIENTED_EDGE('',*,*,#28016,.F.);
#37113=ORIENTED_EDGE('',*,*,#26427,.T.);
#37114=ORIENTED_EDGE('',*,*,#28014,.T.);
#37115=ORIENTED_EDGE('',*,*,#28017,.F.);
#37116=ORIENTED_EDGE('',*,*,#28018,.F.);
#37117=ORIENTED_EDGE('',*,*,#26428,.T.);
#37118=ORIENTED_EDGE('',*,*,#28016,.T.);
#37119=ORIENTED_EDGE('',*,*,#28019,.F.);
#37120=ORIENTED_EDGE('',*,*,#28020,.F.);
#37121=ORIENTED_EDGE('',*,*,#26429,.T.);
#37122=ORIENTED_EDGE('',*,*,#28018,.T.);
#37123=ORIENTED_EDGE('',*,*,#28021,.F.);
#37124=ORIENTED_EDGE('',*,*,#27157,.F.);
#37125=ORIENTED_EDGE('',*,*,#26430,.T.);
#37126=ORIENTED_EDGE('',*,*,#28020,.T.);
#37127=ORIENTED_EDGE('',*,*,#27102,.T.);
#37128=ORIENTED_EDGE('',*,*,#27160,.F.);
#37129=ORIENTED_EDGE('',*,*,#27519,.F.);
#37130=ORIENTED_EDGE('',*,*,#26433,.F.);
#37131=ORIENTED_EDGE('',*,*,#27158,.T.);
#37132=ORIENTED_EDGE('',*,*,#28021,.T.);
#37133=ORIENTED_EDGE('',*,*,#28019,.T.);
#37134=ORIENTED_EDGE('',*,*,#28017,.T.);
#37135=ORIENTED_EDGE('',*,*,#28015,.T.);
#37136=ORIENTED_EDGE('',*,*,#28013,.T.);
#37137=ORIENTED_EDGE('',*,*,#28011,.T.);
#37138=ORIENTED_EDGE('',*,*,#28009,.T.);
#37139=ORIENTED_EDGE('',*,*,#28007,.T.);
#37140=ORIENTED_EDGE('',*,*,#28005,.T.);
#37141=ORIENTED_EDGE('',*,*,#28003,.T.);
#37142=ORIENTED_EDGE('',*,*,#28001,.T.);
#37143=ORIENTED_EDGE('',*,*,#27999,.T.);
#37144=ORIENTED_EDGE('',*,*,#27997,.T.);
#37145=ORIENTED_EDGE('',*,*,#27002,.T.);
#37146=ORIENTED_EDGE('',*,*,#28022,.F.);
#37147=ORIENTED_EDGE('',*,*,#28023,.T.);
#37148=ORIENTED_EDGE('',*,*,#28024,.T.);
#37149=ORIENTED_EDGE('',*,*,#28025,.T.);
#37150=ORIENTED_EDGE('',*,*,#28026,.T.);
#37151=ORIENTED_EDGE('',*,*,#28027,.T.);
#37152=ORIENTED_EDGE('',*,*,#28028,.T.);
#37153=ORIENTED_EDGE('',*,*,#28029,.T.);
#37154=ORIENTED_EDGE('',*,*,#28030,.T.);
#37155=ORIENTED_EDGE('',*,*,#28031,.T.);
#37156=ORIENTED_EDGE('',*,*,#28032,.T.);
#37157=ORIENTED_EDGE('',*,*,#28033,.T.);
#37158=ORIENTED_EDGE('',*,*,#28034,.T.);
#37159=ORIENTED_EDGE('',*,*,#28035,.T.);
#37160=ORIENTED_EDGE('',*,*,#28036,.T.);
#37161=ORIENTED_EDGE('',*,*,#26399,.T.);
#37162=ORIENTED_EDGE('',*,*,#27520,.T.);
#37163=ORIENTED_EDGE('',*,*,#28036,.F.);
#37164=ORIENTED_EDGE('',*,*,#28037,.F.);
#37165=ORIENTED_EDGE('',*,*,#26366,.T.);
#37166=ORIENTED_EDGE('',*,*,#26400,.T.);
#37167=ORIENTED_EDGE('',*,*,#28035,.F.);
#37168=ORIENTED_EDGE('',*,*,#28038,.F.);
#37169=ORIENTED_EDGE('',*,*,#26367,.T.);
#37170=ORIENTED_EDGE('',*,*,#28037,.T.);
#37171=ORIENTED_EDGE('',*,*,#28034,.F.);
#37172=ORIENTED_EDGE('',*,*,#28039,.F.);
#37173=ORIENTED_EDGE('',*,*,#26368,.T.);
#37174=ORIENTED_EDGE('',*,*,#28038,.T.);
#37175=ORIENTED_EDGE('',*,*,#28033,.F.);
#37176=ORIENTED_EDGE('',*,*,#28040,.F.);
#37177=ORIENTED_EDGE('',*,*,#26369,.T.);
#37178=ORIENTED_EDGE('',*,*,#28039,.T.);
#37179=ORIENTED_EDGE('',*,*,#28032,.F.);
#37180=ORIENTED_EDGE('',*,*,#28041,.F.);
#37181=ORIENTED_EDGE('',*,*,#26370,.T.);
#37182=ORIENTED_EDGE('',*,*,#28040,.T.);
#37183=ORIENTED_EDGE('',*,*,#28031,.F.);
#37184=ORIENTED_EDGE('',*,*,#28042,.F.);
#37185=ORIENTED_EDGE('',*,*,#26371,.T.);
#37186=ORIENTED_EDGE('',*,*,#28041,.T.);
#37187=ORIENTED_EDGE('',*,*,#28030,.F.);
#37188=ORIENTED_EDGE('',*,*,#28043,.F.);
#37189=ORIENTED_EDGE('',*,*,#26372,.T.);
#37190=ORIENTED_EDGE('',*,*,#28042,.T.);
#37191=ORIENTED_EDGE('',*,*,#28029,.F.);
#37192=ORIENTED_EDGE('',*,*,#28044,.F.);
#37193=ORIENTED_EDGE('',*,*,#26373,.T.);
#37194=ORIENTED_EDGE('',*,*,#28043,.T.);
#37195=ORIENTED_EDGE('',*,*,#28028,.F.);
#37196=ORIENTED_EDGE('',*,*,#28045,.F.);
#37197=ORIENTED_EDGE('',*,*,#26374,.T.);
#37198=ORIENTED_EDGE('',*,*,#28044,.T.);
#37199=ORIENTED_EDGE('',*,*,#28027,.F.);
#37200=ORIENTED_EDGE('',*,*,#28046,.F.);
#37201=ORIENTED_EDGE('',*,*,#26375,.T.);
#37202=ORIENTED_EDGE('',*,*,#28045,.T.);
#37203=ORIENTED_EDGE('',*,*,#28026,.F.);
#37204=ORIENTED_EDGE('',*,*,#28047,.F.);
#37205=ORIENTED_EDGE('',*,*,#26376,.T.);
#37206=ORIENTED_EDGE('',*,*,#28046,.T.);
#37207=ORIENTED_EDGE('',*,*,#28025,.F.);
#37208=ORIENTED_EDGE('',*,*,#28048,.F.);
#37209=ORIENTED_EDGE('',*,*,#26377,.T.);
#37210=ORIENTED_EDGE('',*,*,#28047,.T.);
#37211=ORIENTED_EDGE('',*,*,#28024,.F.);
#37212=ORIENTED_EDGE('',*,*,#28049,.F.);
#37213=ORIENTED_EDGE('',*,*,#26378,.T.);
#37214=ORIENTED_EDGE('',*,*,#28048,.T.);
#37215=ORIENTED_EDGE('',*,*,#26793,.T.);
#37216=ORIENTED_EDGE('',*,*,#26379,.T.);
#37217=ORIENTED_EDGE('',*,*,#28049,.T.);
#37218=ORIENTED_EDGE('',*,*,#28023,.F.);
#37219=ORIENTED_EDGE('',*,*,#28050,.F.);
#37220=ORIENTED_EDGE('',*,*,#27355,.T.);
#37221=ORIENTED_EDGE('',*,*,#27313,.T.);
#37222=ORIENTED_EDGE('',*,*,#28051,.F.);
#37223=ORIENTED_EDGE('',*,*,#28052,.F.);
#37224=ORIENTED_EDGE('',*,*,#26382,.T.);
#37225=ORIENTED_EDGE('',*,*,#26998,.T.);
#37226=ORIENTED_EDGE('',*,*,#28053,.F.);
#37227=ORIENTED_EDGE('',*,*,#28054,.F.);
#37228=ORIENTED_EDGE('',*,*,#26383,.T.);
#37229=ORIENTED_EDGE('',*,*,#28052,.T.);
#37230=ORIENTED_EDGE('',*,*,#28055,.F.);
#37231=ORIENTED_EDGE('',*,*,#28056,.F.);
#37232=ORIENTED_EDGE('',*,*,#26384,.T.);
#37233=ORIENTED_EDGE('',*,*,#28054,.T.);
#37234=ORIENTED_EDGE('',*,*,#28057,.F.);
#37235=ORIENTED_EDGE('',*,*,#28058,.F.);
#37236=ORIENTED_EDGE('',*,*,#26385,.T.);
#37237=ORIENTED_EDGE('',*,*,#28056,.T.);
#37238=ORIENTED_EDGE('',*,*,#28059,.F.);
#37239=ORIENTED_EDGE('',*,*,#28060,.F.);
#37240=ORIENTED_EDGE('',*,*,#26386,.T.);
#37241=ORIENTED_EDGE('',*,*,#28058,.T.);
#37242=ORIENTED_EDGE('',*,*,#28061,.F.);
#37243=ORIENTED_EDGE('',*,*,#28062,.F.);
#37244=ORIENTED_EDGE('',*,*,#26387,.T.);
#37245=ORIENTED_EDGE('',*,*,#28060,.T.);
#37246=ORIENTED_EDGE('',*,*,#28063,.F.);
#37247=ORIENTED_EDGE('',*,*,#28064,.F.);
#37248=ORIENTED_EDGE('',*,*,#26388,.T.);
#37249=ORIENTED_EDGE('',*,*,#28062,.T.);
#37250=ORIENTED_EDGE('',*,*,#28065,.F.);
#37251=ORIENTED_EDGE('',*,*,#28066,.F.);
#37252=ORIENTED_EDGE('',*,*,#26389,.T.);
#37253=ORIENTED_EDGE('',*,*,#28064,.T.);
#37254=ORIENTED_EDGE('',*,*,#28067,.F.);
#37255=ORIENTED_EDGE('',*,*,#28068,.F.);
#37256=ORIENTED_EDGE('',*,*,#26390,.T.);
#37257=ORIENTED_EDGE('',*,*,#28066,.T.);
#37258=ORIENTED_EDGE('',*,*,#28069,.F.);
#37259=ORIENTED_EDGE('',*,*,#28070,.F.);
#37260=ORIENTED_EDGE('',*,*,#26391,.T.);
#37261=ORIENTED_EDGE('',*,*,#28068,.T.);
#37262=ORIENTED_EDGE('',*,*,#28071,.F.);
#37263=ORIENTED_EDGE('',*,*,#28072,.F.);
#37264=ORIENTED_EDGE('',*,*,#26392,.T.);
#37265=ORIENTED_EDGE('',*,*,#28070,.T.);
#37266=ORIENTED_EDGE('',*,*,#28073,.F.);
#37267=ORIENTED_EDGE('',*,*,#28074,.F.);
#37268=ORIENTED_EDGE('',*,*,#26393,.T.);
#37269=ORIENTED_EDGE('',*,*,#28072,.T.);
#37270=ORIENTED_EDGE('',*,*,#28075,.F.);
#37271=ORIENTED_EDGE('',*,*,#27161,.F.);
#37272=ORIENTED_EDGE('',*,*,#26394,.T.);
#37273=ORIENTED_EDGE('',*,*,#28074,.T.);
#37274=ORIENTED_EDGE('',*,*,#27100,.T.);
#37275=ORIENTED_EDGE('',*,*,#27164,.F.);
#37276=ORIENTED_EDGE('',*,*,#27521,.F.);
#37277=ORIENTED_EDGE('',*,*,#26397,.F.);
#37278=ORIENTED_EDGE('',*,*,#27162,.T.);
#37279=ORIENTED_EDGE('',*,*,#28075,.T.);
#37280=ORIENTED_EDGE('',*,*,#28073,.T.);
#37281=ORIENTED_EDGE('',*,*,#28071,.T.);
#37282=ORIENTED_EDGE('',*,*,#28069,.T.);
#37283=ORIENTED_EDGE('',*,*,#28067,.T.);
#37284=ORIENTED_EDGE('',*,*,#28065,.T.);
#37285=ORIENTED_EDGE('',*,*,#28063,.T.);
#37286=ORIENTED_EDGE('',*,*,#28061,.T.);
#37287=ORIENTED_EDGE('',*,*,#28059,.T.);
#37288=ORIENTED_EDGE('',*,*,#28057,.T.);
#37289=ORIENTED_EDGE('',*,*,#28055,.T.);
#37290=ORIENTED_EDGE('',*,*,#28053,.T.);
#37291=ORIENTED_EDGE('',*,*,#28051,.T.);
#37292=ORIENTED_EDGE('',*,*,#26997,.T.);
#37293=ORIENTED_EDGE('',*,*,#28076,.F.);
#37294=ORIENTED_EDGE('',*,*,#28077,.T.);
#37295=ORIENTED_EDGE('',*,*,#28078,.T.);
#37296=ORIENTED_EDGE('',*,*,#28079,.T.);
#37297=ORIENTED_EDGE('',*,*,#28080,.T.);
#37298=ORIENTED_EDGE('',*,*,#28081,.T.);
#37299=ORIENTED_EDGE('',*,*,#28082,.T.);
#37300=ORIENTED_EDGE('',*,*,#28083,.T.);
#37301=ORIENTED_EDGE('',*,*,#28084,.T.);
#37302=ORIENTED_EDGE('',*,*,#28085,.T.);
#37303=ORIENTED_EDGE('',*,*,#28086,.T.);
#37304=ORIENTED_EDGE('',*,*,#28087,.T.);
#37305=ORIENTED_EDGE('',*,*,#28088,.T.);
#37306=ORIENTED_EDGE('',*,*,#28089,.T.);
#37307=ORIENTED_EDGE('',*,*,#28090,.T.);
#37308=ORIENTED_EDGE('',*,*,#26363,.T.);
#37309=ORIENTED_EDGE('',*,*,#27522,.T.);
#37310=ORIENTED_EDGE('',*,*,#28090,.F.);
#37311=ORIENTED_EDGE('',*,*,#28091,.F.);
#37312=ORIENTED_EDGE('',*,*,#26330,.T.);
#37313=ORIENTED_EDGE('',*,*,#26364,.T.);
#37314=ORIENTED_EDGE('',*,*,#28089,.F.);
#37315=ORIENTED_EDGE('',*,*,#28092,.F.);
#37316=ORIENTED_EDGE('',*,*,#26331,.T.);
#37317=ORIENTED_EDGE('',*,*,#28091,.T.);
#37318=ORIENTED_EDGE('',*,*,#28088,.F.);
#37319=ORIENTED_EDGE('',*,*,#28093,.F.);
#37320=ORIENTED_EDGE('',*,*,#26332,.T.);
#37321=ORIENTED_EDGE('',*,*,#28092,.T.);
#37322=ORIENTED_EDGE('',*,*,#28087,.F.);
#37323=ORIENTED_EDGE('',*,*,#28094,.F.);
#37324=ORIENTED_EDGE('',*,*,#26333,.T.);
#37325=ORIENTED_EDGE('',*,*,#28093,.T.);
#37326=ORIENTED_EDGE('',*,*,#28086,.F.);
#37327=ORIENTED_EDGE('',*,*,#28095,.F.);
#37328=ORIENTED_EDGE('',*,*,#26334,.T.);
#37329=ORIENTED_EDGE('',*,*,#28094,.T.);
#37330=ORIENTED_EDGE('',*,*,#28085,.F.);
#37331=ORIENTED_EDGE('',*,*,#28096,.F.);
#37332=ORIENTED_EDGE('',*,*,#26335,.T.);
#37333=ORIENTED_EDGE('',*,*,#28095,.T.);
#37334=ORIENTED_EDGE('',*,*,#28084,.F.);
#37335=ORIENTED_EDGE('',*,*,#28097,.F.);
#37336=ORIENTED_EDGE('',*,*,#26336,.T.);
#37337=ORIENTED_EDGE('',*,*,#28096,.T.);
#37338=ORIENTED_EDGE('',*,*,#28083,.F.);
#37339=ORIENTED_EDGE('',*,*,#28098,.F.);
#37340=ORIENTED_EDGE('',*,*,#26337,.T.);
#37341=ORIENTED_EDGE('',*,*,#28097,.T.);
#37342=ORIENTED_EDGE('',*,*,#28082,.F.);
#37343=ORIENTED_EDGE('',*,*,#28099,.F.);
#37344=ORIENTED_EDGE('',*,*,#26338,.T.);
#37345=ORIENTED_EDGE('',*,*,#28098,.T.);
#37346=ORIENTED_EDGE('',*,*,#28081,.F.);
#37347=ORIENTED_EDGE('',*,*,#28100,.F.);
#37348=ORIENTED_EDGE('',*,*,#26339,.T.);
#37349=ORIENTED_EDGE('',*,*,#28099,.T.);
#37350=ORIENTED_EDGE('',*,*,#28080,.F.);
#37351=ORIENTED_EDGE('',*,*,#28101,.F.);
#37352=ORIENTED_EDGE('',*,*,#26340,.T.);
#37353=ORIENTED_EDGE('',*,*,#28100,.T.);
#37354=ORIENTED_EDGE('',*,*,#28079,.F.);
#37355=ORIENTED_EDGE('',*,*,#28102,.F.);
#37356=ORIENTED_EDGE('',*,*,#26341,.T.);
#37357=ORIENTED_EDGE('',*,*,#28101,.T.);
#37358=ORIENTED_EDGE('',*,*,#28078,.F.);
#37359=ORIENTED_EDGE('',*,*,#28103,.F.);
#37360=ORIENTED_EDGE('',*,*,#26342,.T.);
#37361=ORIENTED_EDGE('',*,*,#28102,.T.);
#37362=ORIENTED_EDGE('',*,*,#26796,.T.);
#37363=ORIENTED_EDGE('',*,*,#26343,.T.);
#37364=ORIENTED_EDGE('',*,*,#28103,.T.);
#37365=ORIENTED_EDGE('',*,*,#28077,.F.);
#37366=ORIENTED_EDGE('',*,*,#28104,.F.);
#37367=ORIENTED_EDGE('',*,*,#27357,.T.);
#37368=ORIENTED_EDGE('',*,*,#27311,.T.);
#37369=ORIENTED_EDGE('',*,*,#28105,.F.);
#37370=ORIENTED_EDGE('',*,*,#28106,.F.);
#37371=ORIENTED_EDGE('',*,*,#26346,.T.);
#37372=ORIENTED_EDGE('',*,*,#26993,.T.);
#37373=ORIENTED_EDGE('',*,*,#28107,.F.);
#37374=ORIENTED_EDGE('',*,*,#28108,.F.);
#37375=ORIENTED_EDGE('',*,*,#26347,.T.);
#37376=ORIENTED_EDGE('',*,*,#28106,.T.);
#37377=ORIENTED_EDGE('',*,*,#28109,.F.);
#37378=ORIENTED_EDGE('',*,*,#28110,.F.);
#37379=ORIENTED_EDGE('',*,*,#26348,.T.);
#37380=ORIENTED_EDGE('',*,*,#28108,.T.);
#37381=ORIENTED_EDGE('',*,*,#28111,.F.);
#37382=ORIENTED_EDGE('',*,*,#28112,.F.);
#37383=ORIENTED_EDGE('',*,*,#26349,.T.);
#37384=ORIENTED_EDGE('',*,*,#28110,.T.);
#37385=ORIENTED_EDGE('',*,*,#28113,.F.);
#37386=ORIENTED_EDGE('',*,*,#28114,.F.);
#37387=ORIENTED_EDGE('',*,*,#26350,.T.);
#37388=ORIENTED_EDGE('',*,*,#28112,.T.);
#37389=ORIENTED_EDGE('',*,*,#28115,.F.);
#37390=ORIENTED_EDGE('',*,*,#28116,.F.);
#37391=ORIENTED_EDGE('',*,*,#26351,.T.);
#37392=ORIENTED_EDGE('',*,*,#28114,.T.);
#37393=ORIENTED_EDGE('',*,*,#28117,.F.);
#37394=ORIENTED_EDGE('',*,*,#28118,.F.);
#37395=ORIENTED_EDGE('',*,*,#26352,.T.);
#37396=ORIENTED_EDGE('',*,*,#28116,.T.);
#37397=ORIENTED_EDGE('',*,*,#28119,.F.);
#37398=ORIENTED_EDGE('',*,*,#28120,.F.);
#37399=ORIENTED_EDGE('',*,*,#26353,.T.);
#37400=ORIENTED_EDGE('',*,*,#28118,.T.);
#37401=ORIENTED_EDGE('',*,*,#28121,.F.);
#37402=ORIENTED_EDGE('',*,*,#28122,.F.);
#37403=ORIENTED_EDGE('',*,*,#26354,.T.);
#37404=ORIENTED_EDGE('',*,*,#28120,.T.);
#37405=ORIENTED_EDGE('',*,*,#28123,.F.);
#37406=ORIENTED_EDGE('',*,*,#28124,.F.);
#37407=ORIENTED_EDGE('',*,*,#26355,.T.);
#37408=ORIENTED_EDGE('',*,*,#28122,.T.);
#37409=ORIENTED_EDGE('',*,*,#28125,.F.);
#37410=ORIENTED_EDGE('',*,*,#28126,.F.);
#37411=ORIENTED_EDGE('',*,*,#26356,.T.);
#37412=ORIENTED_EDGE('',*,*,#28124,.T.);
#37413=ORIENTED_EDGE('',*,*,#28127,.F.);
#37414=ORIENTED_EDGE('',*,*,#28128,.F.);
#37415=ORIENTED_EDGE('',*,*,#26357,.T.);
#37416=ORIENTED_EDGE('',*,*,#28126,.T.);
#37417=ORIENTED_EDGE('',*,*,#28129,.F.);
#37418=ORIENTED_EDGE('',*,*,#27165,.F.);
#37419=ORIENTED_EDGE('',*,*,#26358,.T.);
#37420=ORIENTED_EDGE('',*,*,#28128,.T.);
#37421=ORIENTED_EDGE('',*,*,#27098,.T.);
#37422=ORIENTED_EDGE('',*,*,#27168,.F.);
#37423=ORIENTED_EDGE('',*,*,#27523,.F.);
#37424=ORIENTED_EDGE('',*,*,#26361,.F.);
#37425=ORIENTED_EDGE('',*,*,#27166,.T.);
#37426=ORIENTED_EDGE('',*,*,#28129,.T.);
#37427=ORIENTED_EDGE('',*,*,#28127,.T.);
#37428=ORIENTED_EDGE('',*,*,#28125,.T.);
#37429=ORIENTED_EDGE('',*,*,#28123,.T.);
#37430=ORIENTED_EDGE('',*,*,#28121,.T.);
#37431=ORIENTED_EDGE('',*,*,#28119,.T.);
#37432=ORIENTED_EDGE('',*,*,#28117,.T.);
#37433=ORIENTED_EDGE('',*,*,#28115,.T.);
#37434=ORIENTED_EDGE('',*,*,#28113,.T.);
#37435=ORIENTED_EDGE('',*,*,#28111,.T.);
#37436=ORIENTED_EDGE('',*,*,#28109,.T.);
#37437=ORIENTED_EDGE('',*,*,#28107,.T.);
#37438=ORIENTED_EDGE('',*,*,#28105,.T.);
#37439=ORIENTED_EDGE('',*,*,#26992,.T.);
#37440=ORIENTED_EDGE('',*,*,#28130,.F.);
#37441=ORIENTED_EDGE('',*,*,#28131,.T.);
#37442=ORIENTED_EDGE('',*,*,#28132,.T.);
#37443=ORIENTED_EDGE('',*,*,#28133,.T.);
#37444=ORIENTED_EDGE('',*,*,#28134,.T.);
#37445=ORIENTED_EDGE('',*,*,#28135,.T.);
#37446=ORIENTED_EDGE('',*,*,#28136,.T.);
#37447=ORIENTED_EDGE('',*,*,#28137,.T.);
#37448=ORIENTED_EDGE('',*,*,#28138,.T.);
#37449=ORIENTED_EDGE('',*,*,#28139,.T.);
#37450=ORIENTED_EDGE('',*,*,#28140,.T.);
#37451=ORIENTED_EDGE('',*,*,#28141,.T.);
#37452=ORIENTED_EDGE('',*,*,#28142,.T.);
#37453=ORIENTED_EDGE('',*,*,#28143,.T.);
#37454=ORIENTED_EDGE('',*,*,#28144,.T.);
#37455=ORIENTED_EDGE('',*,*,#26327,.T.);
#37456=ORIENTED_EDGE('',*,*,#27524,.T.);
#37457=ORIENTED_EDGE('',*,*,#28144,.F.);
#37458=ORIENTED_EDGE('',*,*,#28145,.F.);
#37459=ORIENTED_EDGE('',*,*,#26294,.T.);
#37460=ORIENTED_EDGE('',*,*,#26328,.T.);
#37461=ORIENTED_EDGE('',*,*,#28143,.F.);
#37462=ORIENTED_EDGE('',*,*,#28146,.F.);
#37463=ORIENTED_EDGE('',*,*,#26295,.T.);
#37464=ORIENTED_EDGE('',*,*,#28145,.T.);
#37465=ORIENTED_EDGE('',*,*,#28142,.F.);
#37466=ORIENTED_EDGE('',*,*,#28147,.F.);
#37467=ORIENTED_EDGE('',*,*,#26296,.T.);
#37468=ORIENTED_EDGE('',*,*,#28146,.T.);
#37469=ORIENTED_EDGE('',*,*,#28141,.F.);
#37470=ORIENTED_EDGE('',*,*,#28148,.F.);
#37471=ORIENTED_EDGE('',*,*,#26297,.T.);
#37472=ORIENTED_EDGE('',*,*,#28147,.T.);
#37473=ORIENTED_EDGE('',*,*,#28140,.F.);
#37474=ORIENTED_EDGE('',*,*,#28149,.F.);
#37475=ORIENTED_EDGE('',*,*,#26298,.T.);
#37476=ORIENTED_EDGE('',*,*,#28148,.T.);
#37477=ORIENTED_EDGE('',*,*,#28139,.F.);
#37478=ORIENTED_EDGE('',*,*,#28150,.F.);
#37479=ORIENTED_EDGE('',*,*,#26299,.T.);
#37480=ORIENTED_EDGE('',*,*,#28149,.T.);
#37481=ORIENTED_EDGE('',*,*,#28138,.F.);
#37482=ORIENTED_EDGE('',*,*,#28151,.F.);
#37483=ORIENTED_EDGE('',*,*,#26300,.T.);
#37484=ORIENTED_EDGE('',*,*,#28150,.T.);
#37485=ORIENTED_EDGE('',*,*,#28137,.F.);
#37486=ORIENTED_EDGE('',*,*,#28152,.F.);
#37487=ORIENTED_EDGE('',*,*,#26301,.T.);
#37488=ORIENTED_EDGE('',*,*,#28151,.T.);
#37489=ORIENTED_EDGE('',*,*,#28136,.F.);
#37490=ORIENTED_EDGE('',*,*,#28153,.F.);
#37491=ORIENTED_EDGE('',*,*,#26302,.T.);
#37492=ORIENTED_EDGE('',*,*,#28152,.T.);
#37493=ORIENTED_EDGE('',*,*,#28135,.F.);
#37494=ORIENTED_EDGE('',*,*,#28154,.F.);
#37495=ORIENTED_EDGE('',*,*,#26303,.T.);
#37496=ORIENTED_EDGE('',*,*,#28153,.T.);
#37497=ORIENTED_EDGE('',*,*,#28134,.F.);
#37498=ORIENTED_EDGE('',*,*,#28155,.F.);
#37499=ORIENTED_EDGE('',*,*,#26304,.T.);
#37500=ORIENTED_EDGE('',*,*,#28154,.T.);
#37501=ORIENTED_EDGE('',*,*,#28133,.F.);
#37502=ORIENTED_EDGE('',*,*,#28156,.F.);
#37503=ORIENTED_EDGE('',*,*,#26305,.T.);
#37504=ORIENTED_EDGE('',*,*,#28155,.T.);
#37505=ORIENTED_EDGE('',*,*,#28132,.F.);
#37506=ORIENTED_EDGE('',*,*,#28157,.F.);
#37507=ORIENTED_EDGE('',*,*,#26306,.T.);
#37508=ORIENTED_EDGE('',*,*,#28156,.T.);
#37509=ORIENTED_EDGE('',*,*,#26799,.T.);
#37510=ORIENTED_EDGE('',*,*,#26307,.T.);
#37511=ORIENTED_EDGE('',*,*,#28157,.T.);
#37512=ORIENTED_EDGE('',*,*,#28131,.F.);
#37513=ORIENTED_EDGE('',*,*,#28158,.F.);
#37514=ORIENTED_EDGE('',*,*,#27359,.T.);
#37515=ORIENTED_EDGE('',*,*,#27309,.T.);
#37516=ORIENTED_EDGE('',*,*,#28159,.F.);
#37517=ORIENTED_EDGE('',*,*,#28160,.F.);
#37518=ORIENTED_EDGE('',*,*,#26310,.T.);
#37519=ORIENTED_EDGE('',*,*,#26988,.T.);
#37520=ORIENTED_EDGE('',*,*,#28161,.F.);
#37521=ORIENTED_EDGE('',*,*,#28162,.F.);
#37522=ORIENTED_EDGE('',*,*,#26311,.T.);
#37523=ORIENTED_EDGE('',*,*,#28160,.T.);
#37524=ORIENTED_EDGE('',*,*,#28163,.F.);
#37525=ORIENTED_EDGE('',*,*,#28164,.F.);
#37526=ORIENTED_EDGE('',*,*,#26312,.T.);
#37527=ORIENTED_EDGE('',*,*,#28162,.T.);
#37528=ORIENTED_EDGE('',*,*,#28165,.F.);
#37529=ORIENTED_EDGE('',*,*,#28166,.F.);
#37530=ORIENTED_EDGE('',*,*,#26313,.T.);
#37531=ORIENTED_EDGE('',*,*,#28164,.T.);
#37532=ORIENTED_EDGE('',*,*,#28167,.F.);
#37533=ORIENTED_EDGE('',*,*,#28168,.F.);
#37534=ORIENTED_EDGE('',*,*,#26314,.T.);
#37535=ORIENTED_EDGE('',*,*,#28166,.T.);
#37536=ORIENTED_EDGE('',*,*,#28169,.F.);
#37537=ORIENTED_EDGE('',*,*,#28170,.F.);
#37538=ORIENTED_EDGE('',*,*,#26315,.T.);
#37539=ORIENTED_EDGE('',*,*,#28168,.T.);
#37540=ORIENTED_EDGE('',*,*,#28171,.F.);
#37541=ORIENTED_EDGE('',*,*,#28172,.F.);
#37542=ORIENTED_EDGE('',*,*,#26316,.T.);
#37543=ORIENTED_EDGE('',*,*,#28170,.T.);
#37544=ORIENTED_EDGE('',*,*,#28173,.F.);
#37545=ORIENTED_EDGE('',*,*,#28174,.F.);
#37546=ORIENTED_EDGE('',*,*,#26317,.T.);
#37547=ORIENTED_EDGE('',*,*,#28172,.T.);
#37548=ORIENTED_EDGE('',*,*,#28175,.F.);
#37549=ORIENTED_EDGE('',*,*,#28176,.F.);
#37550=ORIENTED_EDGE('',*,*,#26318,.T.);
#37551=ORIENTED_EDGE('',*,*,#28174,.T.);
#37552=ORIENTED_EDGE('',*,*,#28177,.F.);
#37553=ORIENTED_EDGE('',*,*,#28178,.F.);
#37554=ORIENTED_EDGE('',*,*,#26319,.T.);
#37555=ORIENTED_EDGE('',*,*,#28176,.T.);
#37556=ORIENTED_EDGE('',*,*,#28179,.F.);
#37557=ORIENTED_EDGE('',*,*,#28180,.F.);
#37558=ORIENTED_EDGE('',*,*,#26320,.T.);
#37559=ORIENTED_EDGE('',*,*,#28178,.T.);
#37560=ORIENTED_EDGE('',*,*,#28181,.F.);
#37561=ORIENTED_EDGE('',*,*,#28182,.F.);
#37562=ORIENTED_EDGE('',*,*,#26321,.T.);
#37563=ORIENTED_EDGE('',*,*,#28180,.T.);
#37564=ORIENTED_EDGE('',*,*,#28183,.F.);
#37565=ORIENTED_EDGE('',*,*,#27169,.F.);
#37566=ORIENTED_EDGE('',*,*,#26322,.T.);
#37567=ORIENTED_EDGE('',*,*,#28182,.T.);
#37568=ORIENTED_EDGE('',*,*,#27096,.T.);
#37569=ORIENTED_EDGE('',*,*,#27172,.F.);
#37570=ORIENTED_EDGE('',*,*,#27525,.F.);
#37571=ORIENTED_EDGE('',*,*,#26325,.F.);
#37572=ORIENTED_EDGE('',*,*,#27170,.T.);
#37573=ORIENTED_EDGE('',*,*,#28183,.T.);
#37574=ORIENTED_EDGE('',*,*,#28181,.T.);
#37575=ORIENTED_EDGE('',*,*,#28179,.T.);
#37576=ORIENTED_EDGE('',*,*,#28177,.T.);
#37577=ORIENTED_EDGE('',*,*,#28175,.T.);
#37578=ORIENTED_EDGE('',*,*,#28173,.T.);
#37579=ORIENTED_EDGE('',*,*,#28171,.T.);
#37580=ORIENTED_EDGE('',*,*,#28169,.T.);
#37581=ORIENTED_EDGE('',*,*,#28167,.T.);
#37582=ORIENTED_EDGE('',*,*,#28165,.T.);
#37583=ORIENTED_EDGE('',*,*,#28163,.T.);
#37584=ORIENTED_EDGE('',*,*,#28161,.T.);
#37585=ORIENTED_EDGE('',*,*,#28159,.T.);
#37586=ORIENTED_EDGE('',*,*,#26987,.T.);
#37587=ORIENTED_EDGE('',*,*,#28184,.F.);
#37588=ORIENTED_EDGE('',*,*,#28185,.T.);
#37589=ORIENTED_EDGE('',*,*,#28186,.T.);
#37590=ORIENTED_EDGE('',*,*,#28187,.T.);
#37591=ORIENTED_EDGE('',*,*,#28188,.T.);
#37592=ORIENTED_EDGE('',*,*,#28189,.T.);
#37593=ORIENTED_EDGE('',*,*,#28190,.T.);
#37594=ORIENTED_EDGE('',*,*,#28191,.T.);
#37595=ORIENTED_EDGE('',*,*,#28192,.T.);
#37596=ORIENTED_EDGE('',*,*,#28193,.T.);
#37597=ORIENTED_EDGE('',*,*,#28194,.T.);
#37598=ORIENTED_EDGE('',*,*,#28195,.T.);
#37599=ORIENTED_EDGE('',*,*,#28196,.T.);
#37600=ORIENTED_EDGE('',*,*,#28197,.T.);
#37601=ORIENTED_EDGE('',*,*,#28198,.T.);
#37602=ORIENTED_EDGE('',*,*,#26291,.T.);
#37603=ORIENTED_EDGE('',*,*,#27526,.T.);
#37604=ORIENTED_EDGE('',*,*,#28198,.F.);
#37605=ORIENTED_EDGE('',*,*,#28199,.F.);
#37606=ORIENTED_EDGE('',*,*,#26258,.T.);
#37607=ORIENTED_EDGE('',*,*,#26292,.T.);
#37608=ORIENTED_EDGE('',*,*,#28197,.F.);
#37609=ORIENTED_EDGE('',*,*,#28200,.F.);
#37610=ORIENTED_EDGE('',*,*,#26259,.T.);
#37611=ORIENTED_EDGE('',*,*,#28199,.T.);
#37612=ORIENTED_EDGE('',*,*,#28196,.F.);
#37613=ORIENTED_EDGE('',*,*,#28201,.F.);
#37614=ORIENTED_EDGE('',*,*,#26260,.T.);
#37615=ORIENTED_EDGE('',*,*,#28200,.T.);
#37616=ORIENTED_EDGE('',*,*,#28195,.F.);
#37617=ORIENTED_EDGE('',*,*,#28202,.F.);
#37618=ORIENTED_EDGE('',*,*,#26261,.T.);
#37619=ORIENTED_EDGE('',*,*,#28201,.T.);
#37620=ORIENTED_EDGE('',*,*,#28194,.F.);
#37621=ORIENTED_EDGE('',*,*,#28203,.F.);
#37622=ORIENTED_EDGE('',*,*,#26262,.T.);
#37623=ORIENTED_EDGE('',*,*,#28202,.T.);
#37624=ORIENTED_EDGE('',*,*,#28193,.F.);
#37625=ORIENTED_EDGE('',*,*,#28204,.F.);
#37626=ORIENTED_EDGE('',*,*,#26263,.T.);
#37627=ORIENTED_EDGE('',*,*,#28203,.T.);
#37628=ORIENTED_EDGE('',*,*,#28192,.F.);
#37629=ORIENTED_EDGE('',*,*,#28205,.F.);
#37630=ORIENTED_EDGE('',*,*,#26264,.T.);
#37631=ORIENTED_EDGE('',*,*,#28204,.T.);
#37632=ORIENTED_EDGE('',*,*,#28191,.F.);
#37633=ORIENTED_EDGE('',*,*,#28206,.F.);
#37634=ORIENTED_EDGE('',*,*,#26265,.T.);
#37635=ORIENTED_EDGE('',*,*,#28205,.T.);
#37636=ORIENTED_EDGE('',*,*,#28190,.F.);
#37637=ORIENTED_EDGE('',*,*,#28207,.F.);
#37638=ORIENTED_EDGE('',*,*,#26266,.T.);
#37639=ORIENTED_EDGE('',*,*,#28206,.T.);
#37640=ORIENTED_EDGE('',*,*,#28189,.F.);
#37641=ORIENTED_EDGE('',*,*,#28208,.F.);
#37642=ORIENTED_EDGE('',*,*,#26267,.T.);
#37643=ORIENTED_EDGE('',*,*,#28207,.T.);
#37644=ORIENTED_EDGE('',*,*,#28188,.F.);
#37645=ORIENTED_EDGE('',*,*,#28209,.F.);
#37646=ORIENTED_EDGE('',*,*,#26268,.T.);
#37647=ORIENTED_EDGE('',*,*,#28208,.T.);
#37648=ORIENTED_EDGE('',*,*,#28187,.F.);
#37649=ORIENTED_EDGE('',*,*,#28210,.F.);
#37650=ORIENTED_EDGE('',*,*,#26269,.T.);
#37651=ORIENTED_EDGE('',*,*,#28209,.T.);
#37652=ORIENTED_EDGE('',*,*,#28186,.F.);
#37653=ORIENTED_EDGE('',*,*,#28211,.F.);
#37654=ORIENTED_EDGE('',*,*,#26270,.T.);
#37655=ORIENTED_EDGE('',*,*,#28210,.T.);
#37656=ORIENTED_EDGE('',*,*,#26802,.T.);
#37657=ORIENTED_EDGE('',*,*,#26271,.T.);
#37658=ORIENTED_EDGE('',*,*,#28211,.T.);
#37659=ORIENTED_EDGE('',*,*,#28185,.F.);
#37660=ORIENTED_EDGE('',*,*,#28212,.F.);
#37661=ORIENTED_EDGE('',*,*,#27361,.T.);
#37662=ORIENTED_EDGE('',*,*,#27307,.T.);
#37663=ORIENTED_EDGE('',*,*,#28213,.F.);
#37664=ORIENTED_EDGE('',*,*,#28214,.F.);
#37665=ORIENTED_EDGE('',*,*,#26274,.T.);
#37666=ORIENTED_EDGE('',*,*,#26983,.T.);
#37667=ORIENTED_EDGE('',*,*,#28215,.F.);
#37668=ORIENTED_EDGE('',*,*,#28216,.F.);
#37669=ORIENTED_EDGE('',*,*,#26275,.T.);
#37670=ORIENTED_EDGE('',*,*,#28214,.T.);
#37671=ORIENTED_EDGE('',*,*,#28217,.F.);
#37672=ORIENTED_EDGE('',*,*,#28218,.F.);
#37673=ORIENTED_EDGE('',*,*,#26276,.T.);
#37674=ORIENTED_EDGE('',*,*,#28216,.T.);
#37675=ORIENTED_EDGE('',*,*,#28219,.F.);
#37676=ORIENTED_EDGE('',*,*,#28220,.F.);
#37677=ORIENTED_EDGE('',*,*,#26277,.T.);
#37678=ORIENTED_EDGE('',*,*,#28218,.T.);
#37679=ORIENTED_EDGE('',*,*,#28221,.F.);
#37680=ORIENTED_EDGE('',*,*,#28222,.F.);
#37681=ORIENTED_EDGE('',*,*,#26278,.T.);
#37682=ORIENTED_EDGE('',*,*,#28220,.T.);
#37683=ORIENTED_EDGE('',*,*,#28223,.F.);
#37684=ORIENTED_EDGE('',*,*,#28224,.F.);
#37685=ORIENTED_EDGE('',*,*,#26279,.T.);
#37686=ORIENTED_EDGE('',*,*,#28222,.T.);
#37687=ORIENTED_EDGE('',*,*,#28225,.F.);
#37688=ORIENTED_EDGE('',*,*,#28226,.F.);
#37689=ORIENTED_EDGE('',*,*,#26280,.T.);
#37690=ORIENTED_EDGE('',*,*,#28224,.T.);
#37691=ORIENTED_EDGE('',*,*,#28227,.F.);
#37692=ORIENTED_EDGE('',*,*,#28228,.F.);
#37693=ORIENTED_EDGE('',*,*,#26281,.T.);
#37694=ORIENTED_EDGE('',*,*,#28226,.T.);
#37695=ORIENTED_EDGE('',*,*,#28229,.F.);
#37696=ORIENTED_EDGE('',*,*,#28230,.F.);
#37697=ORIENTED_EDGE('',*,*,#26282,.T.);
#37698=ORIENTED_EDGE('',*,*,#28228,.T.);
#37699=ORIENTED_EDGE('',*,*,#28231,.F.);
#37700=ORIENTED_EDGE('',*,*,#28232,.F.);
#37701=ORIENTED_EDGE('',*,*,#26283,.T.);
#37702=ORIENTED_EDGE('',*,*,#28230,.T.);
#37703=ORIENTED_EDGE('',*,*,#28233,.F.);
#37704=ORIENTED_EDGE('',*,*,#28234,.F.);
#37705=ORIENTED_EDGE('',*,*,#26284,.T.);
#37706=ORIENTED_EDGE('',*,*,#28232,.T.);
#37707=ORIENTED_EDGE('',*,*,#28235,.F.);
#37708=ORIENTED_EDGE('',*,*,#28236,.F.);
#37709=ORIENTED_EDGE('',*,*,#26285,.T.);
#37710=ORIENTED_EDGE('',*,*,#28234,.T.);
#37711=ORIENTED_EDGE('',*,*,#28237,.F.);
#37712=ORIENTED_EDGE('',*,*,#27173,.F.);
#37713=ORIENTED_EDGE('',*,*,#26286,.T.);
#37714=ORIENTED_EDGE('',*,*,#28236,.T.);
#37715=ORIENTED_EDGE('',*,*,#27094,.T.);
#37716=ORIENTED_EDGE('',*,*,#27176,.F.);
#37717=ORIENTED_EDGE('',*,*,#27527,.F.);
#37718=ORIENTED_EDGE('',*,*,#26289,.F.);
#37719=ORIENTED_EDGE('',*,*,#27174,.T.);
#37720=ORIENTED_EDGE('',*,*,#28237,.T.);
#37721=ORIENTED_EDGE('',*,*,#28235,.T.);
#37722=ORIENTED_EDGE('',*,*,#28233,.T.);
#37723=ORIENTED_EDGE('',*,*,#28231,.T.);
#37724=ORIENTED_EDGE('',*,*,#28229,.T.);
#37725=ORIENTED_EDGE('',*,*,#28227,.T.);
#37726=ORIENTED_EDGE('',*,*,#28225,.T.);
#37727=ORIENTED_EDGE('',*,*,#28223,.T.);
#37728=ORIENTED_EDGE('',*,*,#28221,.T.);
#37729=ORIENTED_EDGE('',*,*,#28219,.T.);
#37730=ORIENTED_EDGE('',*,*,#28217,.T.);
#37731=ORIENTED_EDGE('',*,*,#28215,.T.);
#37732=ORIENTED_EDGE('',*,*,#28213,.T.);
#37733=ORIENTED_EDGE('',*,*,#26982,.T.);
#37734=ORIENTED_EDGE('',*,*,#28238,.F.);
#37735=ORIENTED_EDGE('',*,*,#28239,.T.);
#37736=ORIENTED_EDGE('',*,*,#28240,.T.);
#37737=ORIENTED_EDGE('',*,*,#28241,.T.);
#37738=ORIENTED_EDGE('',*,*,#28242,.T.);
#37739=ORIENTED_EDGE('',*,*,#28243,.T.);
#37740=ORIENTED_EDGE('',*,*,#28244,.T.);
#37741=ORIENTED_EDGE('',*,*,#28245,.T.);
#37742=ORIENTED_EDGE('',*,*,#28246,.T.);
#37743=ORIENTED_EDGE('',*,*,#28247,.T.);
#37744=ORIENTED_EDGE('',*,*,#28248,.T.);
#37745=ORIENTED_EDGE('',*,*,#28249,.T.);
#37746=ORIENTED_EDGE('',*,*,#28250,.T.);
#37747=ORIENTED_EDGE('',*,*,#28251,.T.);
#37748=ORIENTED_EDGE('',*,*,#28252,.T.);
#37749=ORIENTED_EDGE('',*,*,#26255,.T.);
#37750=ORIENTED_EDGE('',*,*,#27528,.T.);
#37751=ORIENTED_EDGE('',*,*,#28252,.F.);
#37752=ORIENTED_EDGE('',*,*,#28253,.F.);
#37753=ORIENTED_EDGE('',*,*,#26222,.T.);
#37754=ORIENTED_EDGE('',*,*,#26256,.T.);
#37755=ORIENTED_EDGE('',*,*,#28251,.F.);
#37756=ORIENTED_EDGE('',*,*,#28254,.F.);
#37757=ORIENTED_EDGE('',*,*,#26223,.T.);
#37758=ORIENTED_EDGE('',*,*,#28253,.T.);
#37759=ORIENTED_EDGE('',*,*,#28250,.F.);
#37760=ORIENTED_EDGE('',*,*,#28255,.F.);
#37761=ORIENTED_EDGE('',*,*,#26224,.T.);
#37762=ORIENTED_EDGE('',*,*,#28254,.T.);
#37763=ORIENTED_EDGE('',*,*,#28249,.F.);
#37764=ORIENTED_EDGE('',*,*,#28256,.F.);
#37765=ORIENTED_EDGE('',*,*,#26225,.T.);
#37766=ORIENTED_EDGE('',*,*,#28255,.T.);
#37767=ORIENTED_EDGE('',*,*,#28248,.F.);
#37768=ORIENTED_EDGE('',*,*,#28257,.F.);
#37769=ORIENTED_EDGE('',*,*,#26226,.T.);
#37770=ORIENTED_EDGE('',*,*,#28256,.T.);
#37771=ORIENTED_EDGE('',*,*,#28247,.F.);
#37772=ORIENTED_EDGE('',*,*,#28258,.F.);
#37773=ORIENTED_EDGE('',*,*,#26227,.T.);
#37774=ORIENTED_EDGE('',*,*,#28257,.T.);
#37775=ORIENTED_EDGE('',*,*,#28246,.F.);
#37776=ORIENTED_EDGE('',*,*,#28259,.F.);
#37777=ORIENTED_EDGE('',*,*,#26228,.T.);
#37778=ORIENTED_EDGE('',*,*,#28258,.T.);
#37779=ORIENTED_EDGE('',*,*,#28245,.F.);
#37780=ORIENTED_EDGE('',*,*,#28260,.F.);
#37781=ORIENTED_EDGE('',*,*,#26229,.T.);
#37782=ORIENTED_EDGE('',*,*,#28259,.T.);
#37783=ORIENTED_EDGE('',*,*,#28244,.F.);
#37784=ORIENTED_EDGE('',*,*,#28261,.F.);
#37785=ORIENTED_EDGE('',*,*,#26230,.T.);
#37786=ORIENTED_EDGE('',*,*,#28260,.T.);
#37787=ORIENTED_EDGE('',*,*,#28243,.F.);
#37788=ORIENTED_EDGE('',*,*,#28262,.F.);
#37789=ORIENTED_EDGE('',*,*,#26231,.T.);
#37790=ORIENTED_EDGE('',*,*,#28261,.T.);
#37791=ORIENTED_EDGE('',*,*,#28242,.F.);
#37792=ORIENTED_EDGE('',*,*,#28263,.F.);
#37793=ORIENTED_EDGE('',*,*,#26232,.T.);
#37794=ORIENTED_EDGE('',*,*,#28262,.T.);
#37795=ORIENTED_EDGE('',*,*,#28241,.F.);
#37796=ORIENTED_EDGE('',*,*,#28264,.F.);
#37797=ORIENTED_EDGE('',*,*,#26233,.T.);
#37798=ORIENTED_EDGE('',*,*,#28263,.T.);
#37799=ORIENTED_EDGE('',*,*,#28240,.F.);
#37800=ORIENTED_EDGE('',*,*,#28265,.F.);
#37801=ORIENTED_EDGE('',*,*,#26234,.T.);
#37802=ORIENTED_EDGE('',*,*,#28264,.T.);
#37803=ORIENTED_EDGE('',*,*,#26805,.T.);
#37804=ORIENTED_EDGE('',*,*,#26235,.T.);
#37805=ORIENTED_EDGE('',*,*,#28265,.T.);
#37806=ORIENTED_EDGE('',*,*,#28239,.F.);
#37807=ORIENTED_EDGE('',*,*,#28266,.F.);
#37808=ORIENTED_EDGE('',*,*,#27363,.T.);
#37809=ORIENTED_EDGE('',*,*,#27305,.T.);
#37810=ORIENTED_EDGE('',*,*,#28267,.F.);
#37811=ORIENTED_EDGE('',*,*,#28268,.F.);
#37812=ORIENTED_EDGE('',*,*,#26238,.T.);
#37813=ORIENTED_EDGE('',*,*,#26978,.T.);
#37814=ORIENTED_EDGE('',*,*,#28269,.F.);
#37815=ORIENTED_EDGE('',*,*,#28270,.F.);
#37816=ORIENTED_EDGE('',*,*,#26239,.T.);
#37817=ORIENTED_EDGE('',*,*,#28268,.T.);
#37818=ORIENTED_EDGE('',*,*,#28271,.F.);
#37819=ORIENTED_EDGE('',*,*,#28272,.F.);
#37820=ORIENTED_EDGE('',*,*,#26240,.T.);
#37821=ORIENTED_EDGE('',*,*,#28270,.T.);
#37822=ORIENTED_EDGE('',*,*,#28273,.F.);
#37823=ORIENTED_EDGE('',*,*,#28274,.F.);
#37824=ORIENTED_EDGE('',*,*,#26241,.T.);
#37825=ORIENTED_EDGE('',*,*,#28272,.T.);
#37826=ORIENTED_EDGE('',*,*,#28275,.F.);
#37827=ORIENTED_EDGE('',*,*,#28276,.F.);
#37828=ORIENTED_EDGE('',*,*,#26242,.T.);
#37829=ORIENTED_EDGE('',*,*,#28274,.T.);
#37830=ORIENTED_EDGE('',*,*,#28277,.F.);
#37831=ORIENTED_EDGE('',*,*,#28278,.F.);
#37832=ORIENTED_EDGE('',*,*,#26243,.T.);
#37833=ORIENTED_EDGE('',*,*,#28276,.T.);
#37834=ORIENTED_EDGE('',*,*,#28279,.F.);
#37835=ORIENTED_EDGE('',*,*,#28280,.F.);
#37836=ORIENTED_EDGE('',*,*,#26244,.T.);
#37837=ORIENTED_EDGE('',*,*,#28278,.T.);
#37838=ORIENTED_EDGE('',*,*,#28281,.F.);
#37839=ORIENTED_EDGE('',*,*,#28282,.F.);
#37840=ORIENTED_EDGE('',*,*,#26245,.T.);
#37841=ORIENTED_EDGE('',*,*,#28280,.T.);
#37842=ORIENTED_EDGE('',*,*,#28283,.F.);
#37843=ORIENTED_EDGE('',*,*,#28284,.F.);
#37844=ORIENTED_EDGE('',*,*,#26246,.T.);
#37845=ORIENTED_EDGE('',*,*,#28282,.T.);
#37846=ORIENTED_EDGE('',*,*,#28285,.F.);
#37847=ORIENTED_EDGE('',*,*,#28286,.F.);
#37848=ORIENTED_EDGE('',*,*,#26247,.T.);
#37849=ORIENTED_EDGE('',*,*,#28284,.T.);
#37850=ORIENTED_EDGE('',*,*,#28287,.F.);
#37851=ORIENTED_EDGE('',*,*,#28288,.F.);
#37852=ORIENTED_EDGE('',*,*,#26248,.T.);
#37853=ORIENTED_EDGE('',*,*,#28286,.T.);
#37854=ORIENTED_EDGE('',*,*,#28289,.F.);
#37855=ORIENTED_EDGE('',*,*,#28290,.F.);
#37856=ORIENTED_EDGE('',*,*,#26249,.T.);
#37857=ORIENTED_EDGE('',*,*,#28288,.T.);
#37858=ORIENTED_EDGE('',*,*,#28291,.F.);
#37859=ORIENTED_EDGE('',*,*,#27177,.F.);
#37860=ORIENTED_EDGE('',*,*,#26250,.T.);
#37861=ORIENTED_EDGE('',*,*,#28290,.T.);
#37862=ORIENTED_EDGE('',*,*,#27092,.T.);
#37863=ORIENTED_EDGE('',*,*,#27180,.F.);
#37864=ORIENTED_EDGE('',*,*,#27529,.F.);
#37865=ORIENTED_EDGE('',*,*,#26253,.F.);
#37866=ORIENTED_EDGE('',*,*,#27178,.T.);
#37867=ORIENTED_EDGE('',*,*,#28291,.T.);
#37868=ORIENTED_EDGE('',*,*,#28289,.T.);
#37869=ORIENTED_EDGE('',*,*,#28287,.T.);
#37870=ORIENTED_EDGE('',*,*,#28285,.T.);
#37871=ORIENTED_EDGE('',*,*,#28283,.T.);
#37872=ORIENTED_EDGE('',*,*,#28281,.T.);
#37873=ORIENTED_EDGE('',*,*,#28279,.T.);
#37874=ORIENTED_EDGE('',*,*,#28277,.T.);
#37875=ORIENTED_EDGE('',*,*,#28275,.T.);
#37876=ORIENTED_EDGE('',*,*,#28273,.T.);
#37877=ORIENTED_EDGE('',*,*,#28271,.T.);
#37878=ORIENTED_EDGE('',*,*,#28269,.T.);
#37879=ORIENTED_EDGE('',*,*,#28267,.T.);
#37880=ORIENTED_EDGE('',*,*,#26977,.T.);
#37881=ORIENTED_EDGE('',*,*,#28292,.F.);
#37882=ORIENTED_EDGE('',*,*,#28293,.T.);
#37883=ORIENTED_EDGE('',*,*,#28294,.T.);
#37884=ORIENTED_EDGE('',*,*,#28295,.T.);
#37885=ORIENTED_EDGE('',*,*,#28296,.T.);
#37886=ORIENTED_EDGE('',*,*,#28297,.T.);
#37887=ORIENTED_EDGE('',*,*,#28298,.T.);
#37888=ORIENTED_EDGE('',*,*,#28299,.T.);
#37889=ORIENTED_EDGE('',*,*,#28300,.T.);
#37890=ORIENTED_EDGE('',*,*,#28301,.T.);
#37891=ORIENTED_EDGE('',*,*,#28302,.T.);
#37892=ORIENTED_EDGE('',*,*,#28303,.T.);
#37893=ORIENTED_EDGE('',*,*,#28304,.T.);
#37894=ORIENTED_EDGE('',*,*,#28305,.T.);
#37895=ORIENTED_EDGE('',*,*,#28306,.T.);
#37896=ORIENTED_EDGE('',*,*,#26219,.T.);
#37897=ORIENTED_EDGE('',*,*,#27530,.T.);
#37898=ORIENTED_EDGE('',*,*,#28306,.F.);
#37899=ORIENTED_EDGE('',*,*,#28307,.F.);
#37900=ORIENTED_EDGE('',*,*,#26186,.T.);
#37901=ORIENTED_EDGE('',*,*,#26220,.T.);
#37902=ORIENTED_EDGE('',*,*,#28305,.F.);
#37903=ORIENTED_EDGE('',*,*,#28308,.F.);
#37904=ORIENTED_EDGE('',*,*,#26187,.T.);
#37905=ORIENTED_EDGE('',*,*,#28307,.T.);
#37906=ORIENTED_EDGE('',*,*,#28304,.F.);
#37907=ORIENTED_EDGE('',*,*,#28309,.F.);
#37908=ORIENTED_EDGE('',*,*,#26188,.T.);
#37909=ORIENTED_EDGE('',*,*,#28308,.T.);
#37910=ORIENTED_EDGE('',*,*,#28303,.F.);
#37911=ORIENTED_EDGE('',*,*,#28310,.F.);
#37912=ORIENTED_EDGE('',*,*,#26189,.T.);
#37913=ORIENTED_EDGE('',*,*,#28309,.T.);
#37914=ORIENTED_EDGE('',*,*,#28302,.F.);
#37915=ORIENTED_EDGE('',*,*,#28311,.F.);
#37916=ORIENTED_EDGE('',*,*,#26190,.T.);
#37917=ORIENTED_EDGE('',*,*,#28310,.T.);
#37918=ORIENTED_EDGE('',*,*,#28301,.F.);
#37919=ORIENTED_EDGE('',*,*,#28312,.F.);
#37920=ORIENTED_EDGE('',*,*,#26191,.T.);
#37921=ORIENTED_EDGE('',*,*,#28311,.T.);
#37922=ORIENTED_EDGE('',*,*,#28300,.F.);
#37923=ORIENTED_EDGE('',*,*,#28313,.F.);
#37924=ORIENTED_EDGE('',*,*,#26192,.T.);
#37925=ORIENTED_EDGE('',*,*,#28312,.T.);
#37926=ORIENTED_EDGE('',*,*,#28299,.F.);
#37927=ORIENTED_EDGE('',*,*,#28314,.F.);
#37928=ORIENTED_EDGE('',*,*,#26193,.T.);
#37929=ORIENTED_EDGE('',*,*,#28313,.T.);
#37930=ORIENTED_EDGE('',*,*,#28298,.F.);
#37931=ORIENTED_EDGE('',*,*,#28315,.F.);
#37932=ORIENTED_EDGE('',*,*,#26194,.T.);
#37933=ORIENTED_EDGE('',*,*,#28314,.T.);
#37934=ORIENTED_EDGE('',*,*,#28297,.F.);
#37935=ORIENTED_EDGE('',*,*,#28316,.F.);
#37936=ORIENTED_EDGE('',*,*,#26195,.T.);
#37937=ORIENTED_EDGE('',*,*,#28315,.T.);
#37938=ORIENTED_EDGE('',*,*,#28296,.F.);
#37939=ORIENTED_EDGE('',*,*,#28317,.F.);
#37940=ORIENTED_EDGE('',*,*,#26196,.T.);
#37941=ORIENTED_EDGE('',*,*,#28316,.T.);
#37942=ORIENTED_EDGE('',*,*,#28295,.F.);
#37943=ORIENTED_EDGE('',*,*,#28318,.F.);
#37944=ORIENTED_EDGE('',*,*,#26197,.T.);
#37945=ORIENTED_EDGE('',*,*,#28317,.T.);
#37946=ORIENTED_EDGE('',*,*,#28294,.F.);
#37947=ORIENTED_EDGE('',*,*,#28319,.F.);
#37948=ORIENTED_EDGE('',*,*,#26198,.T.);
#37949=ORIENTED_EDGE('',*,*,#28318,.T.);
#37950=ORIENTED_EDGE('',*,*,#26808,.T.);
#37951=ORIENTED_EDGE('',*,*,#26199,.T.);
#37952=ORIENTED_EDGE('',*,*,#28319,.T.);
#37953=ORIENTED_EDGE('',*,*,#28293,.F.);
#37954=ORIENTED_EDGE('',*,*,#28320,.F.);
#37955=ORIENTED_EDGE('',*,*,#27365,.T.);
#37956=ORIENTED_EDGE('',*,*,#27303,.T.);
#37957=ORIENTED_EDGE('',*,*,#28321,.F.);
#37958=ORIENTED_EDGE('',*,*,#28322,.F.);
#37959=ORIENTED_EDGE('',*,*,#26202,.T.);
#37960=ORIENTED_EDGE('',*,*,#26973,.T.);
#37961=ORIENTED_EDGE('',*,*,#28323,.F.);
#37962=ORIENTED_EDGE('',*,*,#28324,.F.);
#37963=ORIENTED_EDGE('',*,*,#26203,.T.);
#37964=ORIENTED_EDGE('',*,*,#28322,.T.);
#37965=ORIENTED_EDGE('',*,*,#28325,.F.);
#37966=ORIENTED_EDGE('',*,*,#28326,.F.);
#37967=ORIENTED_EDGE('',*,*,#26204,.T.);
#37968=ORIENTED_EDGE('',*,*,#28324,.T.);
#37969=ORIENTED_EDGE('',*,*,#28327,.F.);
#37970=ORIENTED_EDGE('',*,*,#28328,.F.);
#37971=ORIENTED_EDGE('',*,*,#26205,.T.);
#37972=ORIENTED_EDGE('',*,*,#28326,.T.);
#37973=ORIENTED_EDGE('',*,*,#28329,.F.);
#37974=ORIENTED_EDGE('',*,*,#28330,.F.);
#37975=ORIENTED_EDGE('',*,*,#26206,.T.);
#37976=ORIENTED_EDGE('',*,*,#28328,.T.);
#37977=ORIENTED_EDGE('',*,*,#28331,.F.);
#37978=ORIENTED_EDGE('',*,*,#28332,.F.);
#37979=ORIENTED_EDGE('',*,*,#26207,.T.);
#37980=ORIENTED_EDGE('',*,*,#28330,.T.);
#37981=ORIENTED_EDGE('',*,*,#28333,.F.);
#37982=ORIENTED_EDGE('',*,*,#28334,.F.);
#37983=ORIENTED_EDGE('',*,*,#26208,.T.);
#37984=ORIENTED_EDGE('',*,*,#28332,.T.);
#37985=ORIENTED_EDGE('',*,*,#28335,.F.);
#37986=ORIENTED_EDGE('',*,*,#28336,.F.);
#37987=ORIENTED_EDGE('',*,*,#26209,.T.);
#37988=ORIENTED_EDGE('',*,*,#28334,.T.);
#37989=ORIENTED_EDGE('',*,*,#28337,.F.);
#37990=ORIENTED_EDGE('',*,*,#28338,.F.);
#37991=ORIENTED_EDGE('',*,*,#26210,.T.);
#37992=ORIENTED_EDGE('',*,*,#28336,.T.);
#37993=ORIENTED_EDGE('',*,*,#28339,.F.);
#37994=ORIENTED_EDGE('',*,*,#28340,.F.);
#37995=ORIENTED_EDGE('',*,*,#26211,.T.);
#37996=ORIENTED_EDGE('',*,*,#28338,.T.);
#37997=ORIENTED_EDGE('',*,*,#28341,.F.);
#37998=ORIENTED_EDGE('',*,*,#28342,.F.);
#37999=ORIENTED_EDGE('',*,*,#26212,.T.);
#38000=ORIENTED_EDGE('',*,*,#28340,.T.);
#38001=ORIENTED_EDGE('',*,*,#28343,.F.);
#38002=ORIENTED_EDGE('',*,*,#28344,.F.);
#38003=ORIENTED_EDGE('',*,*,#26213,.T.);
#38004=ORIENTED_EDGE('',*,*,#28342,.T.);
#38005=ORIENTED_EDGE('',*,*,#28345,.F.);
#38006=ORIENTED_EDGE('',*,*,#27181,.F.);
#38007=ORIENTED_EDGE('',*,*,#26214,.T.);
#38008=ORIENTED_EDGE('',*,*,#28344,.T.);
#38009=ORIENTED_EDGE('',*,*,#27090,.T.);
#38010=ORIENTED_EDGE('',*,*,#27184,.F.);
#38011=ORIENTED_EDGE('',*,*,#27531,.F.);
#38012=ORIENTED_EDGE('',*,*,#26217,.F.);
#38013=ORIENTED_EDGE('',*,*,#27182,.T.);
#38014=ORIENTED_EDGE('',*,*,#28345,.T.);
#38015=ORIENTED_EDGE('',*,*,#28343,.T.);
#38016=ORIENTED_EDGE('',*,*,#28341,.T.);
#38017=ORIENTED_EDGE('',*,*,#28339,.T.);
#38018=ORIENTED_EDGE('',*,*,#28337,.T.);
#38019=ORIENTED_EDGE('',*,*,#28335,.T.);
#38020=ORIENTED_EDGE('',*,*,#28333,.T.);
#38021=ORIENTED_EDGE('',*,*,#28331,.T.);
#38022=ORIENTED_EDGE('',*,*,#28329,.T.);
#38023=ORIENTED_EDGE('',*,*,#28327,.T.);
#38024=ORIENTED_EDGE('',*,*,#28325,.T.);
#38025=ORIENTED_EDGE('',*,*,#28323,.T.);
#38026=ORIENTED_EDGE('',*,*,#28321,.T.);
#38027=ORIENTED_EDGE('',*,*,#26972,.T.);
#38028=ORIENTED_EDGE('',*,*,#28346,.F.);
#38029=ORIENTED_EDGE('',*,*,#28347,.T.);
#38030=ORIENTED_EDGE('',*,*,#28348,.T.);
#38031=ORIENTED_EDGE('',*,*,#28349,.T.);
#38032=ORIENTED_EDGE('',*,*,#28350,.T.);
#38033=ORIENTED_EDGE('',*,*,#28351,.T.);
#38034=ORIENTED_EDGE('',*,*,#28352,.T.);
#38035=ORIENTED_EDGE('',*,*,#28353,.T.);
#38036=ORIENTED_EDGE('',*,*,#28354,.T.);
#38037=ORIENTED_EDGE('',*,*,#28355,.T.);
#38038=ORIENTED_EDGE('',*,*,#28356,.T.);
#38039=ORIENTED_EDGE('',*,*,#28357,.T.);
#38040=ORIENTED_EDGE('',*,*,#28358,.T.);
#38041=ORIENTED_EDGE('',*,*,#28359,.T.);
#38042=ORIENTED_EDGE('',*,*,#28360,.T.);
#38043=ORIENTED_EDGE('',*,*,#26183,.T.);
#38044=ORIENTED_EDGE('',*,*,#27532,.T.);
#38045=ORIENTED_EDGE('',*,*,#28360,.F.);
#38046=ORIENTED_EDGE('',*,*,#28361,.F.);
#38047=ORIENTED_EDGE('',*,*,#26150,.T.);
#38048=ORIENTED_EDGE('',*,*,#26184,.T.);
#38049=ORIENTED_EDGE('',*,*,#28359,.F.);
#38050=ORIENTED_EDGE('',*,*,#28362,.F.);
#38051=ORIENTED_EDGE('',*,*,#26151,.T.);
#38052=ORIENTED_EDGE('',*,*,#28361,.T.);
#38053=ORIENTED_EDGE('',*,*,#28358,.F.);
#38054=ORIENTED_EDGE('',*,*,#28363,.F.);
#38055=ORIENTED_EDGE('',*,*,#26152,.T.);
#38056=ORIENTED_EDGE('',*,*,#28362,.T.);
#38057=ORIENTED_EDGE('',*,*,#28357,.F.);
#38058=ORIENTED_EDGE('',*,*,#28364,.F.);
#38059=ORIENTED_EDGE('',*,*,#26153,.T.);
#38060=ORIENTED_EDGE('',*,*,#28363,.T.);
#38061=ORIENTED_EDGE('',*,*,#28356,.F.);
#38062=ORIENTED_EDGE('',*,*,#28365,.F.);
#38063=ORIENTED_EDGE('',*,*,#26154,.T.);
#38064=ORIENTED_EDGE('',*,*,#28364,.T.);
#38065=ORIENTED_EDGE('',*,*,#28355,.F.);
#38066=ORIENTED_EDGE('',*,*,#28366,.F.);
#38067=ORIENTED_EDGE('',*,*,#26155,.T.);
#38068=ORIENTED_EDGE('',*,*,#28365,.T.);
#38069=ORIENTED_EDGE('',*,*,#28354,.F.);
#38070=ORIENTED_EDGE('',*,*,#28367,.F.);
#38071=ORIENTED_EDGE('',*,*,#26156,.T.);
#38072=ORIENTED_EDGE('',*,*,#28366,.T.);
#38073=ORIENTED_EDGE('',*,*,#28353,.F.);
#38074=ORIENTED_EDGE('',*,*,#28368,.F.);
#38075=ORIENTED_EDGE('',*,*,#26157,.T.);
#38076=ORIENTED_EDGE('',*,*,#28367,.T.);
#38077=ORIENTED_EDGE('',*,*,#28352,.F.);
#38078=ORIENTED_EDGE('',*,*,#28369,.F.);
#38079=ORIENTED_EDGE('',*,*,#26158,.T.);
#38080=ORIENTED_EDGE('',*,*,#28368,.T.);
#38081=ORIENTED_EDGE('',*,*,#28351,.F.);
#38082=ORIENTED_EDGE('',*,*,#28370,.F.);
#38083=ORIENTED_EDGE('',*,*,#26159,.T.);
#38084=ORIENTED_EDGE('',*,*,#28369,.T.);
#38085=ORIENTED_EDGE('',*,*,#28350,.F.);
#38086=ORIENTED_EDGE('',*,*,#28371,.F.);
#38087=ORIENTED_EDGE('',*,*,#26160,.T.);
#38088=ORIENTED_EDGE('',*,*,#28370,.T.);
#38089=ORIENTED_EDGE('',*,*,#28349,.F.);
#38090=ORIENTED_EDGE('',*,*,#28372,.F.);
#38091=ORIENTED_EDGE('',*,*,#26161,.T.);
#38092=ORIENTED_EDGE('',*,*,#28371,.T.);
#38093=ORIENTED_EDGE('',*,*,#28348,.F.);
#38094=ORIENTED_EDGE('',*,*,#28373,.F.);
#38095=ORIENTED_EDGE('',*,*,#26162,.T.);
#38096=ORIENTED_EDGE('',*,*,#28372,.T.);
#38097=ORIENTED_EDGE('',*,*,#26811,.T.);
#38098=ORIENTED_EDGE('',*,*,#26163,.T.);
#38099=ORIENTED_EDGE('',*,*,#28373,.T.);
#38100=ORIENTED_EDGE('',*,*,#28347,.F.);
#38101=ORIENTED_EDGE('',*,*,#28374,.F.);
#38102=ORIENTED_EDGE('',*,*,#27367,.T.);
#38103=ORIENTED_EDGE('',*,*,#27301,.T.);
#38104=ORIENTED_EDGE('',*,*,#28375,.F.);
#38105=ORIENTED_EDGE('',*,*,#28376,.F.);
#38106=ORIENTED_EDGE('',*,*,#26166,.T.);
#38107=ORIENTED_EDGE('',*,*,#26968,.T.);
#38108=ORIENTED_EDGE('',*,*,#28377,.F.);
#38109=ORIENTED_EDGE('',*,*,#28378,.F.);
#38110=ORIENTED_EDGE('',*,*,#26167,.T.);
#38111=ORIENTED_EDGE('',*,*,#28376,.T.);
#38112=ORIENTED_EDGE('',*,*,#28379,.F.);
#38113=ORIENTED_EDGE('',*,*,#28380,.F.);
#38114=ORIENTED_EDGE('',*,*,#26168,.T.);
#38115=ORIENTED_EDGE('',*,*,#28378,.T.);
#38116=ORIENTED_EDGE('',*,*,#28381,.F.);
#38117=ORIENTED_EDGE('',*,*,#28382,.F.);
#38118=ORIENTED_EDGE('',*,*,#26169,.T.);
#38119=ORIENTED_EDGE('',*,*,#28380,.T.);
#38120=ORIENTED_EDGE('',*,*,#28383,.F.);
#38121=ORIENTED_EDGE('',*,*,#28384,.F.);
#38122=ORIENTED_EDGE('',*,*,#26170,.T.);
#38123=ORIENTED_EDGE('',*,*,#28382,.T.);
#38124=ORIENTED_EDGE('',*,*,#28385,.F.);
#38125=ORIENTED_EDGE('',*,*,#28386,.F.);
#38126=ORIENTED_EDGE('',*,*,#26171,.T.);
#38127=ORIENTED_EDGE('',*,*,#28384,.T.);
#38128=ORIENTED_EDGE('',*,*,#28387,.F.);
#38129=ORIENTED_EDGE('',*,*,#28388,.F.);
#38130=ORIENTED_EDGE('',*,*,#26172,.T.);
#38131=ORIENTED_EDGE('',*,*,#28386,.T.);
#38132=ORIENTED_EDGE('',*,*,#28389,.F.);
#38133=ORIENTED_EDGE('',*,*,#28390,.F.);
#38134=ORIENTED_EDGE('',*,*,#26173,.T.);
#38135=ORIENTED_EDGE('',*,*,#28388,.T.);
#38136=ORIENTED_EDGE('',*,*,#28391,.F.);
#38137=ORIENTED_EDGE('',*,*,#28392,.F.);
#38138=ORIENTED_EDGE('',*,*,#26174,.T.);
#38139=ORIENTED_EDGE('',*,*,#28390,.T.);
#38140=ORIENTED_EDGE('',*,*,#28393,.F.);
#38141=ORIENTED_EDGE('',*,*,#28394,.F.);
#38142=ORIENTED_EDGE('',*,*,#26175,.T.);
#38143=ORIENTED_EDGE('',*,*,#28392,.T.);
#38144=ORIENTED_EDGE('',*,*,#28395,.F.);
#38145=ORIENTED_EDGE('',*,*,#28396,.F.);
#38146=ORIENTED_EDGE('',*,*,#26176,.T.);
#38147=ORIENTED_EDGE('',*,*,#28394,.T.);
#38148=ORIENTED_EDGE('',*,*,#28397,.F.);
#38149=ORIENTED_EDGE('',*,*,#28398,.F.);
#38150=ORIENTED_EDGE('',*,*,#26177,.T.);
#38151=ORIENTED_EDGE('',*,*,#28396,.T.);
#38152=ORIENTED_EDGE('',*,*,#28399,.F.);
#38153=ORIENTED_EDGE('',*,*,#27185,.F.);
#38154=ORIENTED_EDGE('',*,*,#26178,.T.);
#38155=ORIENTED_EDGE('',*,*,#28398,.T.);
#38156=ORIENTED_EDGE('',*,*,#27088,.T.);
#38157=ORIENTED_EDGE('',*,*,#27188,.F.);
#38158=ORIENTED_EDGE('',*,*,#27533,.F.);
#38159=ORIENTED_EDGE('',*,*,#26181,.F.);
#38160=ORIENTED_EDGE('',*,*,#27186,.T.);
#38161=ORIENTED_EDGE('',*,*,#28399,.T.);
#38162=ORIENTED_EDGE('',*,*,#28397,.T.);
#38163=ORIENTED_EDGE('',*,*,#28395,.T.);
#38164=ORIENTED_EDGE('',*,*,#28393,.T.);
#38165=ORIENTED_EDGE('',*,*,#28391,.T.);
#38166=ORIENTED_EDGE('',*,*,#28389,.T.);
#38167=ORIENTED_EDGE('',*,*,#28387,.T.);
#38168=ORIENTED_EDGE('',*,*,#28385,.T.);
#38169=ORIENTED_EDGE('',*,*,#28383,.T.);
#38170=ORIENTED_EDGE('',*,*,#28381,.T.);
#38171=ORIENTED_EDGE('',*,*,#28379,.T.);
#38172=ORIENTED_EDGE('',*,*,#28377,.T.);
#38173=ORIENTED_EDGE('',*,*,#28375,.T.);
#38174=ORIENTED_EDGE('',*,*,#26967,.T.);
#38175=ORIENTED_EDGE('',*,*,#28400,.F.);
#38176=ORIENTED_EDGE('',*,*,#28401,.T.);
#38177=ORIENTED_EDGE('',*,*,#28402,.T.);
#38178=ORIENTED_EDGE('',*,*,#28403,.T.);
#38179=ORIENTED_EDGE('',*,*,#28404,.T.);
#38180=ORIENTED_EDGE('',*,*,#28405,.T.);
#38181=ORIENTED_EDGE('',*,*,#28406,.T.);
#38182=ORIENTED_EDGE('',*,*,#28407,.T.);
#38183=ORIENTED_EDGE('',*,*,#28408,.T.);
#38184=ORIENTED_EDGE('',*,*,#28409,.T.);
#38185=ORIENTED_EDGE('',*,*,#28410,.T.);
#38186=ORIENTED_EDGE('',*,*,#28411,.T.);
#38187=ORIENTED_EDGE('',*,*,#28412,.T.);
#38188=ORIENTED_EDGE('',*,*,#28413,.T.);
#38189=ORIENTED_EDGE('',*,*,#28414,.T.);
#38190=ORIENTED_EDGE('',*,*,#26147,.T.);
#38191=ORIENTED_EDGE('',*,*,#27534,.T.);
#38192=ORIENTED_EDGE('',*,*,#28414,.F.);
#38193=ORIENTED_EDGE('',*,*,#28415,.F.);
#38194=ORIENTED_EDGE('',*,*,#26114,.T.);
#38195=ORIENTED_EDGE('',*,*,#26148,.T.);
#38196=ORIENTED_EDGE('',*,*,#28413,.F.);
#38197=ORIENTED_EDGE('',*,*,#28416,.F.);
#38198=ORIENTED_EDGE('',*,*,#26115,.T.);
#38199=ORIENTED_EDGE('',*,*,#28415,.T.);
#38200=ORIENTED_EDGE('',*,*,#28412,.F.);
#38201=ORIENTED_EDGE('',*,*,#28417,.F.);
#38202=ORIENTED_EDGE('',*,*,#26116,.T.);
#38203=ORIENTED_EDGE('',*,*,#28416,.T.);
#38204=ORIENTED_EDGE('',*,*,#28411,.F.);
#38205=ORIENTED_EDGE('',*,*,#28418,.F.);
#38206=ORIENTED_EDGE('',*,*,#26117,.T.);
#38207=ORIENTED_EDGE('',*,*,#28417,.T.);
#38208=ORIENTED_EDGE('',*,*,#28410,.F.);
#38209=ORIENTED_EDGE('',*,*,#28419,.F.);
#38210=ORIENTED_EDGE('',*,*,#26118,.T.);
#38211=ORIENTED_EDGE('',*,*,#28418,.T.);
#38212=ORIENTED_EDGE('',*,*,#28409,.F.);
#38213=ORIENTED_EDGE('',*,*,#28420,.F.);
#38214=ORIENTED_EDGE('',*,*,#26119,.T.);
#38215=ORIENTED_EDGE('',*,*,#28419,.T.);
#38216=ORIENTED_EDGE('',*,*,#28408,.F.);
#38217=ORIENTED_EDGE('',*,*,#28421,.F.);
#38218=ORIENTED_EDGE('',*,*,#26120,.T.);
#38219=ORIENTED_EDGE('',*,*,#28420,.T.);
#38220=ORIENTED_EDGE('',*,*,#28407,.F.);
#38221=ORIENTED_EDGE('',*,*,#28422,.F.);
#38222=ORIENTED_EDGE('',*,*,#26121,.T.);
#38223=ORIENTED_EDGE('',*,*,#28421,.T.);
#38224=ORIENTED_EDGE('',*,*,#28406,.F.);
#38225=ORIENTED_EDGE('',*,*,#28423,.F.);
#38226=ORIENTED_EDGE('',*,*,#26122,.T.);
#38227=ORIENTED_EDGE('',*,*,#28422,.T.);
#38228=ORIENTED_EDGE('',*,*,#28405,.F.);
#38229=ORIENTED_EDGE('',*,*,#28424,.F.);
#38230=ORIENTED_EDGE('',*,*,#26123,.T.);
#38231=ORIENTED_EDGE('',*,*,#28423,.T.);
#38232=ORIENTED_EDGE('',*,*,#28404,.F.);
#38233=ORIENTED_EDGE('',*,*,#28425,.F.);
#38234=ORIENTED_EDGE('',*,*,#26124,.T.);
#38235=ORIENTED_EDGE('',*,*,#28424,.T.);
#38236=ORIENTED_EDGE('',*,*,#28403,.F.);
#38237=ORIENTED_EDGE('',*,*,#28426,.F.);
#38238=ORIENTED_EDGE('',*,*,#26125,.T.);
#38239=ORIENTED_EDGE('',*,*,#28425,.T.);
#38240=ORIENTED_EDGE('',*,*,#28402,.F.);
#38241=ORIENTED_EDGE('',*,*,#28427,.F.);
#38242=ORIENTED_EDGE('',*,*,#26126,.T.);
#38243=ORIENTED_EDGE('',*,*,#28426,.T.);
#38244=ORIENTED_EDGE('',*,*,#26814,.T.);
#38245=ORIENTED_EDGE('',*,*,#26127,.T.);
#38246=ORIENTED_EDGE('',*,*,#28427,.T.);
#38247=ORIENTED_EDGE('',*,*,#28401,.F.);
#38248=ORIENTED_EDGE('',*,*,#28428,.F.);
#38249=ORIENTED_EDGE('',*,*,#27369,.T.);
#38250=ORIENTED_EDGE('',*,*,#27299,.T.);
#38251=ORIENTED_EDGE('',*,*,#28429,.F.);
#38252=ORIENTED_EDGE('',*,*,#28430,.F.);
#38253=ORIENTED_EDGE('',*,*,#26130,.T.);
#38254=ORIENTED_EDGE('',*,*,#26963,.T.);
#38255=ORIENTED_EDGE('',*,*,#28431,.F.);
#38256=ORIENTED_EDGE('',*,*,#28432,.F.);
#38257=ORIENTED_EDGE('',*,*,#26131,.T.);
#38258=ORIENTED_EDGE('',*,*,#28430,.T.);
#38259=ORIENTED_EDGE('',*,*,#28433,.F.);
#38260=ORIENTED_EDGE('',*,*,#28434,.F.);
#38261=ORIENTED_EDGE('',*,*,#26132,.T.);
#38262=ORIENTED_EDGE('',*,*,#28432,.T.);
#38263=ORIENTED_EDGE('',*,*,#28435,.F.);
#38264=ORIENTED_EDGE('',*,*,#28436,.F.);
#38265=ORIENTED_EDGE('',*,*,#26133,.T.);
#38266=ORIENTED_EDGE('',*,*,#28434,.T.);
#38267=ORIENTED_EDGE('',*,*,#28437,.F.);
#38268=ORIENTED_EDGE('',*,*,#28438,.F.);
#38269=ORIENTED_EDGE('',*,*,#26134,.T.);
#38270=ORIENTED_EDGE('',*,*,#28436,.T.);
#38271=ORIENTED_EDGE('',*,*,#28439,.F.);
#38272=ORIENTED_EDGE('',*,*,#28440,.F.);
#38273=ORIENTED_EDGE('',*,*,#26135,.T.);
#38274=ORIENTED_EDGE('',*,*,#28438,.T.);
#38275=ORIENTED_EDGE('',*,*,#28441,.F.);
#38276=ORIENTED_EDGE('',*,*,#28442,.F.);
#38277=ORIENTED_EDGE('',*,*,#26136,.T.);
#38278=ORIENTED_EDGE('',*,*,#28440,.T.);
#38279=ORIENTED_EDGE('',*,*,#28443,.F.);
#38280=ORIENTED_EDGE('',*,*,#28444,.F.);
#38281=ORIENTED_EDGE('',*,*,#26137,.T.);
#38282=ORIENTED_EDGE('',*,*,#28442,.T.);
#38283=ORIENTED_EDGE('',*,*,#28445,.F.);
#38284=ORIENTED_EDGE('',*,*,#28446,.F.);
#38285=ORIENTED_EDGE('',*,*,#26138,.T.);
#38286=ORIENTED_EDGE('',*,*,#28444,.T.);
#38287=ORIENTED_EDGE('',*,*,#28447,.F.);
#38288=ORIENTED_EDGE('',*,*,#28448,.F.);
#38289=ORIENTED_EDGE('',*,*,#26139,.T.);
#38290=ORIENTED_EDGE('',*,*,#28446,.T.);
#38291=ORIENTED_EDGE('',*,*,#28449,.F.);
#38292=ORIENTED_EDGE('',*,*,#28450,.F.);
#38293=ORIENTED_EDGE('',*,*,#26140,.T.);
#38294=ORIENTED_EDGE('',*,*,#28448,.T.);
#38295=ORIENTED_EDGE('',*,*,#28451,.F.);
#38296=ORIENTED_EDGE('',*,*,#28452,.F.);
#38297=ORIENTED_EDGE('',*,*,#26141,.T.);
#38298=ORIENTED_EDGE('',*,*,#28450,.T.);
#38299=ORIENTED_EDGE('',*,*,#28453,.F.);
#38300=ORIENTED_EDGE('',*,*,#27189,.F.);
#38301=ORIENTED_EDGE('',*,*,#26142,.T.);
#38302=ORIENTED_EDGE('',*,*,#28452,.T.);
#38303=ORIENTED_EDGE('',*,*,#27086,.T.);
#38304=ORIENTED_EDGE('',*,*,#27192,.F.);
#38305=ORIENTED_EDGE('',*,*,#27464,.F.);
#38306=ORIENTED_EDGE('',*,*,#27535,.F.);
#38307=ORIENTED_EDGE('',*,*,#26145,.F.);
#38308=ORIENTED_EDGE('',*,*,#27190,.T.);
#38309=ORIENTED_EDGE('',*,*,#28453,.T.);
#38310=ORIENTED_EDGE('',*,*,#28451,.T.);
#38311=ORIENTED_EDGE('',*,*,#28449,.T.);
#38312=ORIENTED_EDGE('',*,*,#28447,.T.);
#38313=ORIENTED_EDGE('',*,*,#28445,.T.);
#38314=ORIENTED_EDGE('',*,*,#28443,.T.);
#38315=ORIENTED_EDGE('',*,*,#28441,.T.);
#38316=ORIENTED_EDGE('',*,*,#28439,.T.);
#38317=ORIENTED_EDGE('',*,*,#28437,.T.);
#38318=ORIENTED_EDGE('',*,*,#28435,.T.);
#38319=ORIENTED_EDGE('',*,*,#28433,.T.);
#38320=ORIENTED_EDGE('',*,*,#28431,.T.);
#38321=ORIENTED_EDGE('',*,*,#28429,.T.);
#38322=ORIENTED_EDGE('',*,*,#26962,.T.);
#38323=ORIENTED_EDGE('',*,*,#28454,.F.);
#38324=ORIENTED_EDGE('',*,*,#28455,.T.);
#38325=ORIENTED_EDGE('',*,*,#28456,.T.);
#38326=ORIENTED_EDGE('',*,*,#28457,.T.);
#38327=ORIENTED_EDGE('',*,*,#28458,.T.);
#38328=ORIENTED_EDGE('',*,*,#28459,.T.);
#38329=ORIENTED_EDGE('',*,*,#28460,.T.);
#38330=ORIENTED_EDGE('',*,*,#28461,.T.);
#38331=ORIENTED_EDGE('',*,*,#28462,.T.);
#38332=ORIENTED_EDGE('',*,*,#28463,.T.);
#38333=ORIENTED_EDGE('',*,*,#28464,.T.);
#38334=ORIENTED_EDGE('',*,*,#28465,.T.);
#38335=ORIENTED_EDGE('',*,*,#28466,.T.);
#38336=ORIENTED_EDGE('',*,*,#28467,.T.);
#38337=ORIENTED_EDGE('',*,*,#28468,.T.);
#38338=ORIENTED_EDGE('',*,*,#26111,.T.);
#38339=ORIENTED_EDGE('',*,*,#27465,.T.);
#38340=ORIENTED_EDGE('',*,*,#28468,.F.);
#38341=ORIENTED_EDGE('',*,*,#28469,.F.);
#38342=ORIENTED_EDGE('',*,*,#26078,.T.);
#38343=ORIENTED_EDGE('',*,*,#26112,.T.);
#38344=ORIENTED_EDGE('',*,*,#28467,.F.);
#38345=ORIENTED_EDGE('',*,*,#28470,.F.);
#38346=ORIENTED_EDGE('',*,*,#26079,.T.);
#38347=ORIENTED_EDGE('',*,*,#28469,.T.);
#38348=ORIENTED_EDGE('',*,*,#28466,.F.);
#38349=ORIENTED_EDGE('',*,*,#28471,.F.);
#38350=ORIENTED_EDGE('',*,*,#26080,.T.);
#38351=ORIENTED_EDGE('',*,*,#28470,.T.);
#38352=ORIENTED_EDGE('',*,*,#28465,.F.);
#38353=ORIENTED_EDGE('',*,*,#28472,.F.);
#38354=ORIENTED_EDGE('',*,*,#26081,.T.);
#38355=ORIENTED_EDGE('',*,*,#28471,.T.);
#38356=ORIENTED_EDGE('',*,*,#28464,.F.);
#38357=ORIENTED_EDGE('',*,*,#28473,.F.);
#38358=ORIENTED_EDGE('',*,*,#26082,.T.);
#38359=ORIENTED_EDGE('',*,*,#28472,.T.);
#38360=ORIENTED_EDGE('',*,*,#28463,.F.);
#38361=ORIENTED_EDGE('',*,*,#28474,.F.);
#38362=ORIENTED_EDGE('',*,*,#26083,.T.);
#38363=ORIENTED_EDGE('',*,*,#28473,.T.);
#38364=ORIENTED_EDGE('',*,*,#28462,.F.);
#38365=ORIENTED_EDGE('',*,*,#28475,.F.);
#38366=ORIENTED_EDGE('',*,*,#26084,.T.);
#38367=ORIENTED_EDGE('',*,*,#28474,.T.);
#38368=ORIENTED_EDGE('',*,*,#28461,.F.);
#38369=ORIENTED_EDGE('',*,*,#28476,.F.);
#38370=ORIENTED_EDGE('',*,*,#26085,.T.);
#38371=ORIENTED_EDGE('',*,*,#28475,.T.);
#38372=ORIENTED_EDGE('',*,*,#28460,.F.);
#38373=ORIENTED_EDGE('',*,*,#28477,.F.);
#38374=ORIENTED_EDGE('',*,*,#26086,.T.);
#38375=ORIENTED_EDGE('',*,*,#28476,.T.);
#38376=ORIENTED_EDGE('',*,*,#28459,.F.);
#38377=ORIENTED_EDGE('',*,*,#28478,.F.);
#38378=ORIENTED_EDGE('',*,*,#26087,.T.);
#38379=ORIENTED_EDGE('',*,*,#28477,.T.);
#38380=ORIENTED_EDGE('',*,*,#28458,.F.);
#38381=ORIENTED_EDGE('',*,*,#28479,.F.);
#38382=ORIENTED_EDGE('',*,*,#26088,.T.);
#38383=ORIENTED_EDGE('',*,*,#28478,.T.);
#38384=ORIENTED_EDGE('',*,*,#28457,.F.);
#38385=ORIENTED_EDGE('',*,*,#28480,.F.);
#38386=ORIENTED_EDGE('',*,*,#26089,.T.);
#38387=ORIENTED_EDGE('',*,*,#28479,.T.);
#38388=ORIENTED_EDGE('',*,*,#28456,.F.);
#38389=ORIENTED_EDGE('',*,*,#28481,.F.);
#38390=ORIENTED_EDGE('',*,*,#26090,.T.);
#38391=ORIENTED_EDGE('',*,*,#28480,.T.);
#38392=ORIENTED_EDGE('',*,*,#26817,.T.);
#38393=ORIENTED_EDGE('',*,*,#26091,.T.);
#38394=ORIENTED_EDGE('',*,*,#28481,.T.);
#38395=ORIENTED_EDGE('',*,*,#28455,.F.);
#38396=ORIENTED_EDGE('',*,*,#28482,.F.);
#38397=ORIENTED_EDGE('',*,*,#27372,.T.);
#38398=ORIENTED_EDGE('',*,*,#27297,.T.);
#38399=ORIENTED_EDGE('',*,*,#28483,.F.);
#38400=ORIENTED_EDGE('',*,*,#28484,.F.);
#38401=ORIENTED_EDGE('',*,*,#26094,.T.);
#38402=ORIENTED_EDGE('',*,*,#26958,.T.);
#38403=ORIENTED_EDGE('',*,*,#28485,.F.);
#38404=ORIENTED_EDGE('',*,*,#28486,.F.);
#38405=ORIENTED_EDGE('',*,*,#26095,.T.);
#38406=ORIENTED_EDGE('',*,*,#28484,.T.);
#38407=ORIENTED_EDGE('',*,*,#28487,.F.);
#38408=ORIENTED_EDGE('',*,*,#28488,.F.);
#38409=ORIENTED_EDGE('',*,*,#26096,.T.);
#38410=ORIENTED_EDGE('',*,*,#28486,.T.);
#38411=ORIENTED_EDGE('',*,*,#28489,.F.);
#38412=ORIENTED_EDGE('',*,*,#28490,.F.);
#38413=ORIENTED_EDGE('',*,*,#26097,.T.);
#38414=ORIENTED_EDGE('',*,*,#28488,.T.);
#38415=ORIENTED_EDGE('',*,*,#28491,.F.);
#38416=ORIENTED_EDGE('',*,*,#28492,.F.);
#38417=ORIENTED_EDGE('',*,*,#26098,.T.);
#38418=ORIENTED_EDGE('',*,*,#28490,.T.);
#38419=ORIENTED_EDGE('',*,*,#28493,.F.);
#38420=ORIENTED_EDGE('',*,*,#28494,.F.);
#38421=ORIENTED_EDGE('',*,*,#26099,.T.);
#38422=ORIENTED_EDGE('',*,*,#28492,.T.);
#38423=ORIENTED_EDGE('',*,*,#28495,.F.);
#38424=ORIENTED_EDGE('',*,*,#28496,.F.);
#38425=ORIENTED_EDGE('',*,*,#26100,.T.);
#38426=ORIENTED_EDGE('',*,*,#28494,.T.);
#38427=ORIENTED_EDGE('',*,*,#28497,.F.);
#38428=ORIENTED_EDGE('',*,*,#28498,.F.);
#38429=ORIENTED_EDGE('',*,*,#26101,.T.);
#38430=ORIENTED_EDGE('',*,*,#28496,.T.);
#38431=ORIENTED_EDGE('',*,*,#28499,.F.);
#38432=ORIENTED_EDGE('',*,*,#28500,.F.);
#38433=ORIENTED_EDGE('',*,*,#26102,.T.);
#38434=ORIENTED_EDGE('',*,*,#28498,.T.);
#38435=ORIENTED_EDGE('',*,*,#28501,.F.);
#38436=ORIENTED_EDGE('',*,*,#28502,.F.);
#38437=ORIENTED_EDGE('',*,*,#26103,.T.);
#38438=ORIENTED_EDGE('',*,*,#28500,.T.);
#38439=ORIENTED_EDGE('',*,*,#28503,.F.);
#38440=ORIENTED_EDGE('',*,*,#28504,.F.);
#38441=ORIENTED_EDGE('',*,*,#26104,.T.);
#38442=ORIENTED_EDGE('',*,*,#28502,.T.);
#38443=ORIENTED_EDGE('',*,*,#28505,.F.);
#38444=ORIENTED_EDGE('',*,*,#28506,.F.);
#38445=ORIENTED_EDGE('',*,*,#26105,.T.);
#38446=ORIENTED_EDGE('',*,*,#28504,.T.);
#38447=ORIENTED_EDGE('',*,*,#28507,.F.);
#38448=ORIENTED_EDGE('',*,*,#27193,.F.);
#38449=ORIENTED_EDGE('',*,*,#26106,.T.);
#38450=ORIENTED_EDGE('',*,*,#28506,.T.);
#38451=ORIENTED_EDGE('',*,*,#27084,.T.);
#38452=ORIENTED_EDGE('',*,*,#27196,.F.);
#38453=ORIENTED_EDGE('',*,*,#27466,.F.);
#38454=ORIENTED_EDGE('',*,*,#26109,.F.);
#38455=ORIENTED_EDGE('',*,*,#27194,.T.);
#38456=ORIENTED_EDGE('',*,*,#28507,.T.);
#38457=ORIENTED_EDGE('',*,*,#28505,.T.);
#38458=ORIENTED_EDGE('',*,*,#28503,.T.);
#38459=ORIENTED_EDGE('',*,*,#28501,.T.);
#38460=ORIENTED_EDGE('',*,*,#28499,.T.);
#38461=ORIENTED_EDGE('',*,*,#28497,.T.);
#38462=ORIENTED_EDGE('',*,*,#28495,.T.);
#38463=ORIENTED_EDGE('',*,*,#28493,.T.);
#38464=ORIENTED_EDGE('',*,*,#28491,.T.);
#38465=ORIENTED_EDGE('',*,*,#28489,.T.);
#38466=ORIENTED_EDGE('',*,*,#28487,.T.);
#38467=ORIENTED_EDGE('',*,*,#28485,.T.);
#38468=ORIENTED_EDGE('',*,*,#28483,.T.);
#38469=ORIENTED_EDGE('',*,*,#26957,.T.);
#38470=ORIENTED_EDGE('',*,*,#28508,.F.);
#38471=ORIENTED_EDGE('',*,*,#28509,.T.);
#38472=ORIENTED_EDGE('',*,*,#28510,.T.);
#38473=ORIENTED_EDGE('',*,*,#28511,.T.);
#38474=ORIENTED_EDGE('',*,*,#28512,.T.);
#38475=ORIENTED_EDGE('',*,*,#28513,.T.);
#38476=ORIENTED_EDGE('',*,*,#28514,.T.);
#38477=ORIENTED_EDGE('',*,*,#28515,.T.);
#38478=ORIENTED_EDGE('',*,*,#28516,.T.);
#38479=ORIENTED_EDGE('',*,*,#28517,.T.);
#38480=ORIENTED_EDGE('',*,*,#28518,.T.);
#38481=ORIENTED_EDGE('',*,*,#28519,.T.);
#38482=ORIENTED_EDGE('',*,*,#28520,.T.);
#38483=ORIENTED_EDGE('',*,*,#28521,.T.);
#38484=ORIENTED_EDGE('',*,*,#28522,.T.);
#38485=ORIENTED_EDGE('',*,*,#26075,.T.);
#38486=ORIENTED_EDGE('',*,*,#27467,.T.);
#38487=ORIENTED_EDGE('',*,*,#28522,.F.);
#38488=ORIENTED_EDGE('',*,*,#28523,.F.);
#38489=ORIENTED_EDGE('',*,*,#26042,.T.);
#38490=ORIENTED_EDGE('',*,*,#26076,.T.);
#38491=ORIENTED_EDGE('',*,*,#28521,.F.);
#38492=ORIENTED_EDGE('',*,*,#28524,.F.);
#38493=ORIENTED_EDGE('',*,*,#26043,.T.);
#38494=ORIENTED_EDGE('',*,*,#28523,.T.);
#38495=ORIENTED_EDGE('',*,*,#28520,.F.);
#38496=ORIENTED_EDGE('',*,*,#28525,.F.);
#38497=ORIENTED_EDGE('',*,*,#26044,.T.);
#38498=ORIENTED_EDGE('',*,*,#28524,.T.);
#38499=ORIENTED_EDGE('',*,*,#28519,.F.);
#38500=ORIENTED_EDGE('',*,*,#28526,.F.);
#38501=ORIENTED_EDGE('',*,*,#26045,.T.);
#38502=ORIENTED_EDGE('',*,*,#28525,.T.);
#38503=ORIENTED_EDGE('',*,*,#28518,.F.);
#38504=ORIENTED_EDGE('',*,*,#28527,.F.);
#38505=ORIENTED_EDGE('',*,*,#26046,.T.);
#38506=ORIENTED_EDGE('',*,*,#28526,.T.);
#38507=ORIENTED_EDGE('',*,*,#28517,.F.);
#38508=ORIENTED_EDGE('',*,*,#28528,.F.);
#38509=ORIENTED_EDGE('',*,*,#26047,.T.);
#38510=ORIENTED_EDGE('',*,*,#28527,.T.);
#38511=ORIENTED_EDGE('',*,*,#28516,.F.);
#38512=ORIENTED_EDGE('',*,*,#28529,.F.);
#38513=ORIENTED_EDGE('',*,*,#26048,.T.);
#38514=ORIENTED_EDGE('',*,*,#28528,.T.);
#38515=ORIENTED_EDGE('',*,*,#28515,.F.);
#38516=ORIENTED_EDGE('',*,*,#28530,.F.);
#38517=ORIENTED_EDGE('',*,*,#26049,.T.);
#38518=ORIENTED_EDGE('',*,*,#28529,.T.);
#38519=ORIENTED_EDGE('',*,*,#28514,.F.);
#38520=ORIENTED_EDGE('',*,*,#28531,.F.);
#38521=ORIENTED_EDGE('',*,*,#26050,.T.);
#38522=ORIENTED_EDGE('',*,*,#28530,.T.);
#38523=ORIENTED_EDGE('',*,*,#28513,.F.);
#38524=ORIENTED_EDGE('',*,*,#28532,.F.);
#38525=ORIENTED_EDGE('',*,*,#26051,.T.);
#38526=ORIENTED_EDGE('',*,*,#28531,.T.);
#38527=ORIENTED_EDGE('',*,*,#28512,.F.);
#38528=ORIENTED_EDGE('',*,*,#28533,.F.);
#38529=ORIENTED_EDGE('',*,*,#26052,.T.);
#38530=ORIENTED_EDGE('',*,*,#28532,.T.);
#38531=ORIENTED_EDGE('',*,*,#28511,.F.);
#38532=ORIENTED_EDGE('',*,*,#28534,.F.);
#38533=ORIENTED_EDGE('',*,*,#26053,.T.);
#38534=ORIENTED_EDGE('',*,*,#28533,.T.);
#38535=ORIENTED_EDGE('',*,*,#28510,.F.);
#38536=ORIENTED_EDGE('',*,*,#28535,.F.);
#38537=ORIENTED_EDGE('',*,*,#26054,.T.);
#38538=ORIENTED_EDGE('',*,*,#28534,.T.);
#38539=ORIENTED_EDGE('',*,*,#26820,.T.);
#38540=ORIENTED_EDGE('',*,*,#26055,.T.);
#38541=ORIENTED_EDGE('',*,*,#28535,.T.);
#38542=ORIENTED_EDGE('',*,*,#28509,.F.);
#38543=ORIENTED_EDGE('',*,*,#28536,.F.);
#38544=ORIENTED_EDGE('',*,*,#27374,.T.);
#38545=ORIENTED_EDGE('',*,*,#27295,.T.);
#38546=ORIENTED_EDGE('',*,*,#28537,.F.);
#38547=ORIENTED_EDGE('',*,*,#28538,.F.);
#38548=ORIENTED_EDGE('',*,*,#26058,.T.);
#38549=ORIENTED_EDGE('',*,*,#26953,.T.);
#38550=ORIENTED_EDGE('',*,*,#28539,.F.);
#38551=ORIENTED_EDGE('',*,*,#28540,.F.);
#38552=ORIENTED_EDGE('',*,*,#26059,.T.);
#38553=ORIENTED_EDGE('',*,*,#28538,.T.);
#38554=ORIENTED_EDGE('',*,*,#28541,.F.);
#38555=ORIENTED_EDGE('',*,*,#28542,.F.);
#38556=ORIENTED_EDGE('',*,*,#26060,.T.);
#38557=ORIENTED_EDGE('',*,*,#28540,.T.);
#38558=ORIENTED_EDGE('',*,*,#28543,.F.);
#38559=ORIENTED_EDGE('',*,*,#28544,.F.);
#38560=ORIENTED_EDGE('',*,*,#26061,.T.);
#38561=ORIENTED_EDGE('',*,*,#28542,.T.);
#38562=ORIENTED_EDGE('',*,*,#28545,.F.);
#38563=ORIENTED_EDGE('',*,*,#28546,.F.);
#38564=ORIENTED_EDGE('',*,*,#26062,.T.);
#38565=ORIENTED_EDGE('',*,*,#28544,.T.);
#38566=ORIENTED_EDGE('',*,*,#28547,.F.);
#38567=ORIENTED_EDGE('',*,*,#28548,.F.);
#38568=ORIENTED_EDGE('',*,*,#26063,.T.);
#38569=ORIENTED_EDGE('',*,*,#28546,.T.);
#38570=ORIENTED_EDGE('',*,*,#28549,.F.);
#38571=ORIENTED_EDGE('',*,*,#28550,.F.);
#38572=ORIENTED_EDGE('',*,*,#26064,.T.);
#38573=ORIENTED_EDGE('',*,*,#28548,.T.);
#38574=ORIENTED_EDGE('',*,*,#28551,.F.);
#38575=ORIENTED_EDGE('',*,*,#28552,.F.);
#38576=ORIENTED_EDGE('',*,*,#26065,.T.);
#38577=ORIENTED_EDGE('',*,*,#28550,.T.);
#38578=ORIENTED_EDGE('',*,*,#28553,.F.);
#38579=ORIENTED_EDGE('',*,*,#28554,.F.);
#38580=ORIENTED_EDGE('',*,*,#26066,.T.);
#38581=ORIENTED_EDGE('',*,*,#28552,.T.);
#38582=ORIENTED_EDGE('',*,*,#28555,.F.);
#38583=ORIENTED_EDGE('',*,*,#28556,.F.);
#38584=ORIENTED_EDGE('',*,*,#26067,.T.);
#38585=ORIENTED_EDGE('',*,*,#28554,.T.);
#38586=ORIENTED_EDGE('',*,*,#28557,.F.);
#38587=ORIENTED_EDGE('',*,*,#28558,.F.);
#38588=ORIENTED_EDGE('',*,*,#26068,.T.);
#38589=ORIENTED_EDGE('',*,*,#28556,.T.);
#38590=ORIENTED_EDGE('',*,*,#28559,.F.);
#38591=ORIENTED_EDGE('',*,*,#28560,.F.);
#38592=ORIENTED_EDGE('',*,*,#26069,.T.);
#38593=ORIENTED_EDGE('',*,*,#28558,.T.);
#38594=ORIENTED_EDGE('',*,*,#28561,.F.);
#38595=ORIENTED_EDGE('',*,*,#27197,.F.);
#38596=ORIENTED_EDGE('',*,*,#26070,.T.);
#38597=ORIENTED_EDGE('',*,*,#28560,.T.);
#38598=ORIENTED_EDGE('',*,*,#27082,.T.);
#38599=ORIENTED_EDGE('',*,*,#27200,.F.);
#38600=ORIENTED_EDGE('',*,*,#27468,.F.);
#38601=ORIENTED_EDGE('',*,*,#26073,.F.);
#38602=ORIENTED_EDGE('',*,*,#27198,.T.);
#38603=ORIENTED_EDGE('',*,*,#28561,.T.);
#38604=ORIENTED_EDGE('',*,*,#28559,.T.);
#38605=ORIENTED_EDGE('',*,*,#28557,.T.);
#38606=ORIENTED_EDGE('',*,*,#28555,.T.);
#38607=ORIENTED_EDGE('',*,*,#28553,.T.);
#38608=ORIENTED_EDGE('',*,*,#28551,.T.);
#38609=ORIENTED_EDGE('',*,*,#28549,.T.);
#38610=ORIENTED_EDGE('',*,*,#28547,.T.);
#38611=ORIENTED_EDGE('',*,*,#28545,.T.);
#38612=ORIENTED_EDGE('',*,*,#28543,.T.);
#38613=ORIENTED_EDGE('',*,*,#28541,.T.);
#38614=ORIENTED_EDGE('',*,*,#28539,.T.);
#38615=ORIENTED_EDGE('',*,*,#28537,.T.);
#38616=ORIENTED_EDGE('',*,*,#26952,.T.);
#38617=ORIENTED_EDGE('',*,*,#28562,.F.);
#38618=ORIENTED_EDGE('',*,*,#28563,.T.);
#38619=ORIENTED_EDGE('',*,*,#28564,.T.);
#38620=ORIENTED_EDGE('',*,*,#28565,.T.);
#38621=ORIENTED_EDGE('',*,*,#28566,.T.);
#38622=ORIENTED_EDGE('',*,*,#28567,.T.);
#38623=ORIENTED_EDGE('',*,*,#28568,.T.);
#38624=ORIENTED_EDGE('',*,*,#28569,.T.);
#38625=ORIENTED_EDGE('',*,*,#28570,.T.);
#38626=ORIENTED_EDGE('',*,*,#28571,.T.);
#38627=ORIENTED_EDGE('',*,*,#28572,.T.);
#38628=ORIENTED_EDGE('',*,*,#28573,.T.);
#38629=ORIENTED_EDGE('',*,*,#28574,.T.);
#38630=ORIENTED_EDGE('',*,*,#28575,.T.);
#38631=ORIENTED_EDGE('',*,*,#28576,.T.);
#38632=ORIENTED_EDGE('',*,*,#26039,.T.);
#38633=ORIENTED_EDGE('',*,*,#27469,.T.);
#38634=ORIENTED_EDGE('',*,*,#28576,.F.);
#38635=ORIENTED_EDGE('',*,*,#28577,.F.);
#38636=ORIENTED_EDGE('',*,*,#26006,.T.);
#38637=ORIENTED_EDGE('',*,*,#26040,.T.);
#38638=ORIENTED_EDGE('',*,*,#28575,.F.);
#38639=ORIENTED_EDGE('',*,*,#28578,.F.);
#38640=ORIENTED_EDGE('',*,*,#26007,.T.);
#38641=ORIENTED_EDGE('',*,*,#28577,.T.);
#38642=ORIENTED_EDGE('',*,*,#28574,.F.);
#38643=ORIENTED_EDGE('',*,*,#28579,.F.);
#38644=ORIENTED_EDGE('',*,*,#26008,.T.);
#38645=ORIENTED_EDGE('',*,*,#28578,.T.);
#38646=ORIENTED_EDGE('',*,*,#28573,.F.);
#38647=ORIENTED_EDGE('',*,*,#28580,.F.);
#38648=ORIENTED_EDGE('',*,*,#26009,.T.);
#38649=ORIENTED_EDGE('',*,*,#28579,.T.);
#38650=ORIENTED_EDGE('',*,*,#28572,.F.);
#38651=ORIENTED_EDGE('',*,*,#28581,.F.);
#38652=ORIENTED_EDGE('',*,*,#26010,.T.);
#38653=ORIENTED_EDGE('',*,*,#28580,.T.);
#38654=ORIENTED_EDGE('',*,*,#28571,.F.);
#38655=ORIENTED_EDGE('',*,*,#28582,.F.);
#38656=ORIENTED_EDGE('',*,*,#26011,.T.);
#38657=ORIENTED_EDGE('',*,*,#28581,.T.);
#38658=ORIENTED_EDGE('',*,*,#28570,.F.);
#38659=ORIENTED_EDGE('',*,*,#28583,.F.);
#38660=ORIENTED_EDGE('',*,*,#26012,.T.);
#38661=ORIENTED_EDGE('',*,*,#28582,.T.);
#38662=ORIENTED_EDGE('',*,*,#28569,.F.);
#38663=ORIENTED_EDGE('',*,*,#28584,.F.);
#38664=ORIENTED_EDGE('',*,*,#26013,.T.);
#38665=ORIENTED_EDGE('',*,*,#28583,.T.);
#38666=ORIENTED_EDGE('',*,*,#28568,.F.);
#38667=ORIENTED_EDGE('',*,*,#28585,.F.);
#38668=ORIENTED_EDGE('',*,*,#26014,.T.);
#38669=ORIENTED_EDGE('',*,*,#28584,.T.);
#38670=ORIENTED_EDGE('',*,*,#28567,.F.);
#38671=ORIENTED_EDGE('',*,*,#28586,.F.);
#38672=ORIENTED_EDGE('',*,*,#26015,.T.);
#38673=ORIENTED_EDGE('',*,*,#28585,.T.);
#38674=ORIENTED_EDGE('',*,*,#28566,.F.);
#38675=ORIENTED_EDGE('',*,*,#28587,.F.);
#38676=ORIENTED_EDGE('',*,*,#26016,.T.);
#38677=ORIENTED_EDGE('',*,*,#28586,.T.);
#38678=ORIENTED_EDGE('',*,*,#28565,.F.);
#38679=ORIENTED_EDGE('',*,*,#28588,.F.);
#38680=ORIENTED_EDGE('',*,*,#26017,.T.);
#38681=ORIENTED_EDGE('',*,*,#28587,.T.);
#38682=ORIENTED_EDGE('',*,*,#28564,.F.);
#38683=ORIENTED_EDGE('',*,*,#28589,.F.);
#38684=ORIENTED_EDGE('',*,*,#26018,.T.);
#38685=ORIENTED_EDGE('',*,*,#28588,.T.);
#38686=ORIENTED_EDGE('',*,*,#26823,.T.);
#38687=ORIENTED_EDGE('',*,*,#26019,.T.);
#38688=ORIENTED_EDGE('',*,*,#28589,.T.);
#38689=ORIENTED_EDGE('',*,*,#28563,.F.);
#38690=ORIENTED_EDGE('',*,*,#28590,.F.);
#38691=ORIENTED_EDGE('',*,*,#27376,.T.);
#38692=ORIENTED_EDGE('',*,*,#27293,.T.);
#38693=ORIENTED_EDGE('',*,*,#28591,.F.);
#38694=ORIENTED_EDGE('',*,*,#28592,.F.);
#38695=ORIENTED_EDGE('',*,*,#26022,.T.);
#38696=ORIENTED_EDGE('',*,*,#26948,.T.);
#38697=ORIENTED_EDGE('',*,*,#28593,.F.);
#38698=ORIENTED_EDGE('',*,*,#28594,.F.);
#38699=ORIENTED_EDGE('',*,*,#26023,.T.);
#38700=ORIENTED_EDGE('',*,*,#28592,.T.);
#38701=ORIENTED_EDGE('',*,*,#28595,.F.);
#38702=ORIENTED_EDGE('',*,*,#28596,.F.);
#38703=ORIENTED_EDGE('',*,*,#26024,.T.);
#38704=ORIENTED_EDGE('',*,*,#28594,.T.);
#38705=ORIENTED_EDGE('',*,*,#28597,.F.);
#38706=ORIENTED_EDGE('',*,*,#28598,.F.);
#38707=ORIENTED_EDGE('',*,*,#26025,.T.);
#38708=ORIENTED_EDGE('',*,*,#28596,.T.);
#38709=ORIENTED_EDGE('',*,*,#28599,.F.);
#38710=ORIENTED_EDGE('',*,*,#28600,.F.);
#38711=ORIENTED_EDGE('',*,*,#26026,.T.);
#38712=ORIENTED_EDGE('',*,*,#28598,.T.);
#38713=ORIENTED_EDGE('',*,*,#28601,.F.);
#38714=ORIENTED_EDGE('',*,*,#28602,.F.);
#38715=ORIENTED_EDGE('',*,*,#26027,.T.);
#38716=ORIENTED_EDGE('',*,*,#28600,.T.);
#38717=ORIENTED_EDGE('',*,*,#28603,.F.);
#38718=ORIENTED_EDGE('',*,*,#28604,.F.);
#38719=ORIENTED_EDGE('',*,*,#26028,.T.);
#38720=ORIENTED_EDGE('',*,*,#28602,.T.);
#38721=ORIENTED_EDGE('',*,*,#28605,.F.);
#38722=ORIENTED_EDGE('',*,*,#28606,.F.);
#38723=ORIENTED_EDGE('',*,*,#26029,.T.);
#38724=ORIENTED_EDGE('',*,*,#28604,.T.);
#38725=ORIENTED_EDGE('',*,*,#28607,.F.);
#38726=ORIENTED_EDGE('',*,*,#28608,.F.);
#38727=ORIENTED_EDGE('',*,*,#26030,.T.);
#38728=ORIENTED_EDGE('',*,*,#28606,.T.);
#38729=ORIENTED_EDGE('',*,*,#28609,.F.);
#38730=ORIENTED_EDGE('',*,*,#28610,.F.);
#38731=ORIENTED_EDGE('',*,*,#26031,.T.);
#38732=ORIENTED_EDGE('',*,*,#28608,.T.);
#38733=ORIENTED_EDGE('',*,*,#28611,.F.);
#38734=ORIENTED_EDGE('',*,*,#28612,.F.);
#38735=ORIENTED_EDGE('',*,*,#26032,.T.);
#38736=ORIENTED_EDGE('',*,*,#28610,.T.);
#38737=ORIENTED_EDGE('',*,*,#28613,.F.);
#38738=ORIENTED_EDGE('',*,*,#28614,.F.);
#38739=ORIENTED_EDGE('',*,*,#26033,.T.);
#38740=ORIENTED_EDGE('',*,*,#28612,.T.);
#38741=ORIENTED_EDGE('',*,*,#28615,.F.);
#38742=ORIENTED_EDGE('',*,*,#27201,.F.);
#38743=ORIENTED_EDGE('',*,*,#26034,.T.);
#38744=ORIENTED_EDGE('',*,*,#28614,.T.);
#38745=ORIENTED_EDGE('',*,*,#27080,.T.);
#38746=ORIENTED_EDGE('',*,*,#27204,.F.);
#38747=ORIENTED_EDGE('',*,*,#27470,.F.);
#38748=ORIENTED_EDGE('',*,*,#26037,.F.);
#38749=ORIENTED_EDGE('',*,*,#27202,.T.);
#38750=ORIENTED_EDGE('',*,*,#28615,.T.);
#38751=ORIENTED_EDGE('',*,*,#28613,.T.);
#38752=ORIENTED_EDGE('',*,*,#28611,.T.);
#38753=ORIENTED_EDGE('',*,*,#28609,.T.);
#38754=ORIENTED_EDGE('',*,*,#28607,.T.);
#38755=ORIENTED_EDGE('',*,*,#28605,.T.);
#38756=ORIENTED_EDGE('',*,*,#28603,.T.);
#38757=ORIENTED_EDGE('',*,*,#28601,.T.);
#38758=ORIENTED_EDGE('',*,*,#28599,.T.);
#38759=ORIENTED_EDGE('',*,*,#28597,.T.);
#38760=ORIENTED_EDGE('',*,*,#28595,.T.);
#38761=ORIENTED_EDGE('',*,*,#28593,.T.);
#38762=ORIENTED_EDGE('',*,*,#28591,.T.);
#38763=ORIENTED_EDGE('',*,*,#26947,.T.);
#38764=ORIENTED_EDGE('',*,*,#28616,.F.);
#38765=ORIENTED_EDGE('',*,*,#28617,.T.);
#38766=ORIENTED_EDGE('',*,*,#28618,.T.);
#38767=ORIENTED_EDGE('',*,*,#28619,.T.);
#38768=ORIENTED_EDGE('',*,*,#28620,.T.);
#38769=ORIENTED_EDGE('',*,*,#28621,.T.);
#38770=ORIENTED_EDGE('',*,*,#28622,.T.);
#38771=ORIENTED_EDGE('',*,*,#28623,.T.);
#38772=ORIENTED_EDGE('',*,*,#28624,.T.);
#38773=ORIENTED_EDGE('',*,*,#28625,.T.);
#38774=ORIENTED_EDGE('',*,*,#28626,.T.);
#38775=ORIENTED_EDGE('',*,*,#28627,.T.);
#38776=ORIENTED_EDGE('',*,*,#28628,.T.);
#38777=ORIENTED_EDGE('',*,*,#28629,.T.);
#38778=ORIENTED_EDGE('',*,*,#28630,.T.);
#38779=ORIENTED_EDGE('',*,*,#26003,.T.);
#38780=ORIENTED_EDGE('',*,*,#27471,.T.);
#38781=ORIENTED_EDGE('',*,*,#28630,.F.);
#38782=ORIENTED_EDGE('',*,*,#28631,.F.);
#38783=ORIENTED_EDGE('',*,*,#25970,.T.);
#38784=ORIENTED_EDGE('',*,*,#26004,.T.);
#38785=ORIENTED_EDGE('',*,*,#28629,.F.);
#38786=ORIENTED_EDGE('',*,*,#28632,.F.);
#38787=ORIENTED_EDGE('',*,*,#25971,.T.);
#38788=ORIENTED_EDGE('',*,*,#28631,.T.);
#38789=ORIENTED_EDGE('',*,*,#28628,.F.);
#38790=ORIENTED_EDGE('',*,*,#28633,.F.);
#38791=ORIENTED_EDGE('',*,*,#25972,.T.);
#38792=ORIENTED_EDGE('',*,*,#28632,.T.);
#38793=ORIENTED_EDGE('',*,*,#28627,.F.);
#38794=ORIENTED_EDGE('',*,*,#28634,.F.);
#38795=ORIENTED_EDGE('',*,*,#25973,.T.);
#38796=ORIENTED_EDGE('',*,*,#28633,.T.);
#38797=ORIENTED_EDGE('',*,*,#28626,.F.);
#38798=ORIENTED_EDGE('',*,*,#28635,.F.);
#38799=ORIENTED_EDGE('',*,*,#25974,.T.);
#38800=ORIENTED_EDGE('',*,*,#28634,.T.);
#38801=ORIENTED_EDGE('',*,*,#28625,.F.);
#38802=ORIENTED_EDGE('',*,*,#28636,.F.);
#38803=ORIENTED_EDGE('',*,*,#25975,.T.);
#38804=ORIENTED_EDGE('',*,*,#28635,.T.);
#38805=ORIENTED_EDGE('',*,*,#28624,.F.);
#38806=ORIENTED_EDGE('',*,*,#28637,.F.);
#38807=ORIENTED_EDGE('',*,*,#25976,.T.);
#38808=ORIENTED_EDGE('',*,*,#28636,.T.);
#38809=ORIENTED_EDGE('',*,*,#28623,.F.);
#38810=ORIENTED_EDGE('',*,*,#28638,.F.);
#38811=ORIENTED_EDGE('',*,*,#25977,.T.);
#38812=ORIENTED_EDGE('',*,*,#28637,.T.);
#38813=ORIENTED_EDGE('',*,*,#28622,.F.);
#38814=ORIENTED_EDGE('',*,*,#28639,.F.);
#38815=ORIENTED_EDGE('',*,*,#25978,.T.);
#38816=ORIENTED_EDGE('',*,*,#28638,.T.);
#38817=ORIENTED_EDGE('',*,*,#28621,.F.);
#38818=ORIENTED_EDGE('',*,*,#28640,.F.);
#38819=ORIENTED_EDGE('',*,*,#25979,.T.);
#38820=ORIENTED_EDGE('',*,*,#28639,.T.);
#38821=ORIENTED_EDGE('',*,*,#28620,.F.);
#38822=ORIENTED_EDGE('',*,*,#28641,.F.);
#38823=ORIENTED_EDGE('',*,*,#25980,.T.);
#38824=ORIENTED_EDGE('',*,*,#28640,.T.);
#38825=ORIENTED_EDGE('',*,*,#28619,.F.);
#38826=ORIENTED_EDGE('',*,*,#28642,.F.);
#38827=ORIENTED_EDGE('',*,*,#25981,.T.);
#38828=ORIENTED_EDGE('',*,*,#28641,.T.);
#38829=ORIENTED_EDGE('',*,*,#28618,.F.);
#38830=ORIENTED_EDGE('',*,*,#28643,.F.);
#38831=ORIENTED_EDGE('',*,*,#25982,.T.);
#38832=ORIENTED_EDGE('',*,*,#28642,.T.);
#38833=ORIENTED_EDGE('',*,*,#26826,.T.);
#38834=ORIENTED_EDGE('',*,*,#25983,.T.);
#38835=ORIENTED_EDGE('',*,*,#28643,.T.);
#38836=ORIENTED_EDGE('',*,*,#28617,.F.);
#38837=ORIENTED_EDGE('',*,*,#28644,.F.);
#38838=ORIENTED_EDGE('',*,*,#27378,.T.);
#38839=ORIENTED_EDGE('',*,*,#27291,.T.);
#38840=ORIENTED_EDGE('',*,*,#28645,.F.);
#38841=ORIENTED_EDGE('',*,*,#28646,.F.);
#38842=ORIENTED_EDGE('',*,*,#25986,.T.);
#38843=ORIENTED_EDGE('',*,*,#26943,.T.);
#38844=ORIENTED_EDGE('',*,*,#28647,.F.);
#38845=ORIENTED_EDGE('',*,*,#28648,.F.);
#38846=ORIENTED_EDGE('',*,*,#25987,.T.);
#38847=ORIENTED_EDGE('',*,*,#28646,.T.);
#38848=ORIENTED_EDGE('',*,*,#28649,.F.);
#38849=ORIENTED_EDGE('',*,*,#28650,.F.);
#38850=ORIENTED_EDGE('',*,*,#25988,.T.);
#38851=ORIENTED_EDGE('',*,*,#28648,.T.);
#38852=ORIENTED_EDGE('',*,*,#28651,.F.);
#38853=ORIENTED_EDGE('',*,*,#28652,.F.);
#38854=ORIENTED_EDGE('',*,*,#25989,.T.);
#38855=ORIENTED_EDGE('',*,*,#28650,.T.);
#38856=ORIENTED_EDGE('',*,*,#28653,.F.);
#38857=ORIENTED_EDGE('',*,*,#28654,.F.);
#38858=ORIENTED_EDGE('',*,*,#25990,.T.);
#38859=ORIENTED_EDGE('',*,*,#28652,.T.);
#38860=ORIENTED_EDGE('',*,*,#28655,.F.);
#38861=ORIENTED_EDGE('',*,*,#28656,.F.);
#38862=ORIENTED_EDGE('',*,*,#25991,.T.);
#38863=ORIENTED_EDGE('',*,*,#28654,.T.);
#38864=ORIENTED_EDGE('',*,*,#28657,.F.);
#38865=ORIENTED_EDGE('',*,*,#28658,.F.);
#38866=ORIENTED_EDGE('',*,*,#25992,.T.);
#38867=ORIENTED_EDGE('',*,*,#28656,.T.);
#38868=ORIENTED_EDGE('',*,*,#28659,.F.);
#38869=ORIENTED_EDGE('',*,*,#28660,.F.);
#38870=ORIENTED_EDGE('',*,*,#25993,.T.);
#38871=ORIENTED_EDGE('',*,*,#28658,.T.);
#38872=ORIENTED_EDGE('',*,*,#28661,.F.);
#38873=ORIENTED_EDGE('',*,*,#28662,.F.);
#38874=ORIENTED_EDGE('',*,*,#25994,.T.);
#38875=ORIENTED_EDGE('',*,*,#28660,.T.);
#38876=ORIENTED_EDGE('',*,*,#28663,.F.);
#38877=ORIENTED_EDGE('',*,*,#28664,.F.);
#38878=ORIENTED_EDGE('',*,*,#25995,.T.);
#38879=ORIENTED_EDGE('',*,*,#28662,.T.);
#38880=ORIENTED_EDGE('',*,*,#28665,.F.);
#38881=ORIENTED_EDGE('',*,*,#28666,.F.);
#38882=ORIENTED_EDGE('',*,*,#25996,.T.);
#38883=ORIENTED_EDGE('',*,*,#28664,.T.);
#38884=ORIENTED_EDGE('',*,*,#28667,.F.);
#38885=ORIENTED_EDGE('',*,*,#28668,.F.);
#38886=ORIENTED_EDGE('',*,*,#25997,.T.);
#38887=ORIENTED_EDGE('',*,*,#28666,.T.);
#38888=ORIENTED_EDGE('',*,*,#28669,.F.);
#38889=ORIENTED_EDGE('',*,*,#27205,.F.);
#38890=ORIENTED_EDGE('',*,*,#25998,.T.);
#38891=ORIENTED_EDGE('',*,*,#28668,.T.);
#38892=ORIENTED_EDGE('',*,*,#27078,.T.);
#38893=ORIENTED_EDGE('',*,*,#27208,.F.);
#38894=ORIENTED_EDGE('',*,*,#27472,.F.);
#38895=ORIENTED_EDGE('',*,*,#26001,.F.);
#38896=ORIENTED_EDGE('',*,*,#27206,.T.);
#38897=ORIENTED_EDGE('',*,*,#28669,.T.);
#38898=ORIENTED_EDGE('',*,*,#28667,.T.);
#38899=ORIENTED_EDGE('',*,*,#28665,.T.);
#38900=ORIENTED_EDGE('',*,*,#28663,.T.);
#38901=ORIENTED_EDGE('',*,*,#28661,.T.);
#38902=ORIENTED_EDGE('',*,*,#28659,.T.);
#38903=ORIENTED_EDGE('',*,*,#28657,.T.);
#38904=ORIENTED_EDGE('',*,*,#28655,.T.);
#38905=ORIENTED_EDGE('',*,*,#28653,.T.);
#38906=ORIENTED_EDGE('',*,*,#28651,.T.);
#38907=ORIENTED_EDGE('',*,*,#28649,.T.);
#38908=ORIENTED_EDGE('',*,*,#28647,.T.);
#38909=ORIENTED_EDGE('',*,*,#28645,.T.);
#38910=ORIENTED_EDGE('',*,*,#26942,.T.);
#38911=ORIENTED_EDGE('',*,*,#28670,.F.);
#38912=ORIENTED_EDGE('',*,*,#28671,.T.);
#38913=ORIENTED_EDGE('',*,*,#28672,.T.);
#38914=ORIENTED_EDGE('',*,*,#28673,.T.);
#38915=ORIENTED_EDGE('',*,*,#28674,.T.);
#38916=ORIENTED_EDGE('',*,*,#28675,.T.);
#38917=ORIENTED_EDGE('',*,*,#28676,.T.);
#38918=ORIENTED_EDGE('',*,*,#28677,.T.);
#38919=ORIENTED_EDGE('',*,*,#28678,.T.);
#38920=ORIENTED_EDGE('',*,*,#28679,.T.);
#38921=ORIENTED_EDGE('',*,*,#28680,.T.);
#38922=ORIENTED_EDGE('',*,*,#28681,.T.);
#38923=ORIENTED_EDGE('',*,*,#28682,.T.);
#38924=ORIENTED_EDGE('',*,*,#28683,.T.);
#38925=ORIENTED_EDGE('',*,*,#28684,.T.);
#38926=ORIENTED_EDGE('',*,*,#25967,.T.);
#38927=ORIENTED_EDGE('',*,*,#27473,.T.);
#38928=ORIENTED_EDGE('',*,*,#28684,.F.);
#38929=ORIENTED_EDGE('',*,*,#28685,.F.);
#38930=ORIENTED_EDGE('',*,*,#25934,.T.);
#38931=ORIENTED_EDGE('',*,*,#25968,.T.);
#38932=ORIENTED_EDGE('',*,*,#28683,.F.);
#38933=ORIENTED_EDGE('',*,*,#28686,.F.);
#38934=ORIENTED_EDGE('',*,*,#25935,.T.);
#38935=ORIENTED_EDGE('',*,*,#28685,.T.);
#38936=ORIENTED_EDGE('',*,*,#28682,.F.);
#38937=ORIENTED_EDGE('',*,*,#28687,.F.);
#38938=ORIENTED_EDGE('',*,*,#25936,.T.);
#38939=ORIENTED_EDGE('',*,*,#28686,.T.);
#38940=ORIENTED_EDGE('',*,*,#28681,.F.);
#38941=ORIENTED_EDGE('',*,*,#28688,.F.);
#38942=ORIENTED_EDGE('',*,*,#25937,.T.);
#38943=ORIENTED_EDGE('',*,*,#28687,.T.);
#38944=ORIENTED_EDGE('',*,*,#28680,.F.);
#38945=ORIENTED_EDGE('',*,*,#28689,.F.);
#38946=ORIENTED_EDGE('',*,*,#25938,.T.);
#38947=ORIENTED_EDGE('',*,*,#28688,.T.);
#38948=ORIENTED_EDGE('',*,*,#28679,.F.);
#38949=ORIENTED_EDGE('',*,*,#28690,.F.);
#38950=ORIENTED_EDGE('',*,*,#25939,.T.);
#38951=ORIENTED_EDGE('',*,*,#28689,.T.);
#38952=ORIENTED_EDGE('',*,*,#28678,.F.);
#38953=ORIENTED_EDGE('',*,*,#28691,.F.);
#38954=ORIENTED_EDGE('',*,*,#25940,.T.);
#38955=ORIENTED_EDGE('',*,*,#28690,.T.);
#38956=ORIENTED_EDGE('',*,*,#28677,.F.);
#38957=ORIENTED_EDGE('',*,*,#28692,.F.);
#38958=ORIENTED_EDGE('',*,*,#25941,.T.);
#38959=ORIENTED_EDGE('',*,*,#28691,.T.);
#38960=ORIENTED_EDGE('',*,*,#28676,.F.);
#38961=ORIENTED_EDGE('',*,*,#28693,.F.);
#38962=ORIENTED_EDGE('',*,*,#25942,.T.);
#38963=ORIENTED_EDGE('',*,*,#28692,.T.);
#38964=ORIENTED_EDGE('',*,*,#28675,.F.);
#38965=ORIENTED_EDGE('',*,*,#28694,.F.);
#38966=ORIENTED_EDGE('',*,*,#25943,.T.);
#38967=ORIENTED_EDGE('',*,*,#28693,.T.);
#38968=ORIENTED_EDGE('',*,*,#28674,.F.);
#38969=ORIENTED_EDGE('',*,*,#28695,.F.);
#38970=ORIENTED_EDGE('',*,*,#25944,.T.);
#38971=ORIENTED_EDGE('',*,*,#28694,.T.);
#38972=ORIENTED_EDGE('',*,*,#28673,.F.);
#38973=ORIENTED_EDGE('',*,*,#28696,.F.);
#38974=ORIENTED_EDGE('',*,*,#25945,.T.);
#38975=ORIENTED_EDGE('',*,*,#28695,.T.);
#38976=ORIENTED_EDGE('',*,*,#28672,.F.);
#38977=ORIENTED_EDGE('',*,*,#28697,.F.);
#38978=ORIENTED_EDGE('',*,*,#25946,.T.);
#38979=ORIENTED_EDGE('',*,*,#28696,.T.);
#38980=ORIENTED_EDGE('',*,*,#26829,.T.);
#38981=ORIENTED_EDGE('',*,*,#25947,.T.);
#38982=ORIENTED_EDGE('',*,*,#28697,.T.);
#38983=ORIENTED_EDGE('',*,*,#28671,.F.);
#38984=ORIENTED_EDGE('',*,*,#28698,.F.);
#38985=ORIENTED_EDGE('',*,*,#27380,.T.);
#38986=ORIENTED_EDGE('',*,*,#27289,.T.);
#38987=ORIENTED_EDGE('',*,*,#28699,.F.);
#38988=ORIENTED_EDGE('',*,*,#28700,.F.);
#38989=ORIENTED_EDGE('',*,*,#25950,.T.);
#38990=ORIENTED_EDGE('',*,*,#26938,.T.);
#38991=ORIENTED_EDGE('',*,*,#28701,.F.);
#38992=ORIENTED_EDGE('',*,*,#28702,.F.);
#38993=ORIENTED_EDGE('',*,*,#25951,.T.);
#38994=ORIENTED_EDGE('',*,*,#28700,.T.);
#38995=ORIENTED_EDGE('',*,*,#28703,.F.);
#38996=ORIENTED_EDGE('',*,*,#28704,.F.);
#38997=ORIENTED_EDGE('',*,*,#25952,.T.);
#38998=ORIENTED_EDGE('',*,*,#28702,.T.);
#38999=ORIENTED_EDGE('',*,*,#28705,.F.);
#39000=ORIENTED_EDGE('',*,*,#28706,.F.);
#39001=ORIENTED_EDGE('',*,*,#25953,.T.);
#39002=ORIENTED_EDGE('',*,*,#28704,.T.);
#39003=ORIENTED_EDGE('',*,*,#28707,.F.);
#39004=ORIENTED_EDGE('',*,*,#28708,.F.);
#39005=ORIENTED_EDGE('',*,*,#25954,.T.);
#39006=ORIENTED_EDGE('',*,*,#28706,.T.);
#39007=ORIENTED_EDGE('',*,*,#28709,.F.);
#39008=ORIENTED_EDGE('',*,*,#28710,.F.);
#39009=ORIENTED_EDGE('',*,*,#25955,.T.);
#39010=ORIENTED_EDGE('',*,*,#28708,.T.);
#39011=ORIENTED_EDGE('',*,*,#28711,.F.);
#39012=ORIENTED_EDGE('',*,*,#28712,.F.);
#39013=ORIENTED_EDGE('',*,*,#25956,.T.);
#39014=ORIENTED_EDGE('',*,*,#28710,.T.);
#39015=ORIENTED_EDGE('',*,*,#28713,.F.);
#39016=ORIENTED_EDGE('',*,*,#28714,.F.);
#39017=ORIENTED_EDGE('',*,*,#25957,.T.);
#39018=ORIENTED_EDGE('',*,*,#28712,.T.);
#39019=ORIENTED_EDGE('',*,*,#28715,.F.);
#39020=ORIENTED_EDGE('',*,*,#28716,.F.);
#39021=ORIENTED_EDGE('',*,*,#25958,.T.);
#39022=ORIENTED_EDGE('',*,*,#28714,.T.);
#39023=ORIENTED_EDGE('',*,*,#28717,.F.);
#39024=ORIENTED_EDGE('',*,*,#28718,.F.);
#39025=ORIENTED_EDGE('',*,*,#25959,.T.);
#39026=ORIENTED_EDGE('',*,*,#28716,.T.);
#39027=ORIENTED_EDGE('',*,*,#28719,.F.);
#39028=ORIENTED_EDGE('',*,*,#28720,.F.);
#39029=ORIENTED_EDGE('',*,*,#25960,.T.);
#39030=ORIENTED_EDGE('',*,*,#28718,.T.);
#39031=ORIENTED_EDGE('',*,*,#28721,.F.);
#39032=ORIENTED_EDGE('',*,*,#28722,.F.);
#39033=ORIENTED_EDGE('',*,*,#25961,.T.);
#39034=ORIENTED_EDGE('',*,*,#28720,.T.);
#39035=ORIENTED_EDGE('',*,*,#28723,.F.);
#39036=ORIENTED_EDGE('',*,*,#27209,.F.);
#39037=ORIENTED_EDGE('',*,*,#25962,.T.);
#39038=ORIENTED_EDGE('',*,*,#28722,.T.);
#39039=ORIENTED_EDGE('',*,*,#27076,.T.);
#39040=ORIENTED_EDGE('',*,*,#27212,.F.);
#39041=ORIENTED_EDGE('',*,*,#27474,.F.);
#39042=ORIENTED_EDGE('',*,*,#25965,.F.);
#39043=ORIENTED_EDGE('',*,*,#27210,.T.);
#39044=ORIENTED_EDGE('',*,*,#28723,.T.);
#39045=ORIENTED_EDGE('',*,*,#28721,.T.);
#39046=ORIENTED_EDGE('',*,*,#28719,.T.);
#39047=ORIENTED_EDGE('',*,*,#28717,.T.);
#39048=ORIENTED_EDGE('',*,*,#28715,.T.);
#39049=ORIENTED_EDGE('',*,*,#28713,.T.);
#39050=ORIENTED_EDGE('',*,*,#28711,.T.);
#39051=ORIENTED_EDGE('',*,*,#28709,.T.);
#39052=ORIENTED_EDGE('',*,*,#28707,.T.);
#39053=ORIENTED_EDGE('',*,*,#28705,.T.);
#39054=ORIENTED_EDGE('',*,*,#28703,.T.);
#39055=ORIENTED_EDGE('',*,*,#28701,.T.);
#39056=ORIENTED_EDGE('',*,*,#28699,.T.);
#39057=ORIENTED_EDGE('',*,*,#26937,.T.);
#39058=ORIENTED_EDGE('',*,*,#28724,.F.);
#39059=ORIENTED_EDGE('',*,*,#28725,.T.);
#39060=ORIENTED_EDGE('',*,*,#28726,.T.);
#39061=ORIENTED_EDGE('',*,*,#28727,.T.);
#39062=ORIENTED_EDGE('',*,*,#28728,.T.);
#39063=ORIENTED_EDGE('',*,*,#28729,.T.);
#39064=ORIENTED_EDGE('',*,*,#28730,.T.);
#39065=ORIENTED_EDGE('',*,*,#28731,.T.);
#39066=ORIENTED_EDGE('',*,*,#28732,.T.);
#39067=ORIENTED_EDGE('',*,*,#28733,.T.);
#39068=ORIENTED_EDGE('',*,*,#28734,.T.);
#39069=ORIENTED_EDGE('',*,*,#28735,.T.);
#39070=ORIENTED_EDGE('',*,*,#28736,.T.);
#39071=ORIENTED_EDGE('',*,*,#28737,.T.);
#39072=ORIENTED_EDGE('',*,*,#28738,.T.);
#39073=ORIENTED_EDGE('',*,*,#25931,.T.);
#39074=ORIENTED_EDGE('',*,*,#27475,.T.);
#39075=ORIENTED_EDGE('',*,*,#28738,.F.);
#39076=ORIENTED_EDGE('',*,*,#28739,.F.);
#39077=ORIENTED_EDGE('',*,*,#25898,.T.);
#39078=ORIENTED_EDGE('',*,*,#25932,.T.);
#39079=ORIENTED_EDGE('',*,*,#28737,.F.);
#39080=ORIENTED_EDGE('',*,*,#28740,.F.);
#39081=ORIENTED_EDGE('',*,*,#25899,.T.);
#39082=ORIENTED_EDGE('',*,*,#28739,.T.);
#39083=ORIENTED_EDGE('',*,*,#28736,.F.);
#39084=ORIENTED_EDGE('',*,*,#28741,.F.);
#39085=ORIENTED_EDGE('',*,*,#25900,.T.);
#39086=ORIENTED_EDGE('',*,*,#28740,.T.);
#39087=ORIENTED_EDGE('',*,*,#28735,.F.);
#39088=ORIENTED_EDGE('',*,*,#28742,.F.);
#39089=ORIENTED_EDGE('',*,*,#25901,.T.);
#39090=ORIENTED_EDGE('',*,*,#28741,.T.);
#39091=ORIENTED_EDGE('',*,*,#28734,.F.);
#39092=ORIENTED_EDGE('',*,*,#28743,.F.);
#39093=ORIENTED_EDGE('',*,*,#25902,.T.);
#39094=ORIENTED_EDGE('',*,*,#28742,.T.);
#39095=ORIENTED_EDGE('',*,*,#28733,.F.);
#39096=ORIENTED_EDGE('',*,*,#28744,.F.);
#39097=ORIENTED_EDGE('',*,*,#25903,.T.);
#39098=ORIENTED_EDGE('',*,*,#28743,.T.);
#39099=ORIENTED_EDGE('',*,*,#28732,.F.);
#39100=ORIENTED_EDGE('',*,*,#28745,.F.);
#39101=ORIENTED_EDGE('',*,*,#25904,.T.);
#39102=ORIENTED_EDGE('',*,*,#28744,.T.);
#39103=ORIENTED_EDGE('',*,*,#28731,.F.);
#39104=ORIENTED_EDGE('',*,*,#28746,.F.);
#39105=ORIENTED_EDGE('',*,*,#25905,.T.);
#39106=ORIENTED_EDGE('',*,*,#28745,.T.);
#39107=ORIENTED_EDGE('',*,*,#28730,.F.);
#39108=ORIENTED_EDGE('',*,*,#28747,.F.);
#39109=ORIENTED_EDGE('',*,*,#25906,.T.);
#39110=ORIENTED_EDGE('',*,*,#28746,.T.);
#39111=ORIENTED_EDGE('',*,*,#28729,.F.);
#39112=ORIENTED_EDGE('',*,*,#28748,.F.);
#39113=ORIENTED_EDGE('',*,*,#25907,.T.);
#39114=ORIENTED_EDGE('',*,*,#28747,.T.);
#39115=ORIENTED_EDGE('',*,*,#28728,.F.);
#39116=ORIENTED_EDGE('',*,*,#28749,.F.);
#39117=ORIENTED_EDGE('',*,*,#25908,.T.);
#39118=ORIENTED_EDGE('',*,*,#28748,.T.);
#39119=ORIENTED_EDGE('',*,*,#28727,.F.);
#39120=ORIENTED_EDGE('',*,*,#28750,.F.);
#39121=ORIENTED_EDGE('',*,*,#25909,.T.);
#39122=ORIENTED_EDGE('',*,*,#28749,.T.);
#39123=ORIENTED_EDGE('',*,*,#28726,.F.);
#39124=ORIENTED_EDGE('',*,*,#28751,.F.);
#39125=ORIENTED_EDGE('',*,*,#25910,.T.);
#39126=ORIENTED_EDGE('',*,*,#28750,.T.);
#39127=ORIENTED_EDGE('',*,*,#26832,.T.);
#39128=ORIENTED_EDGE('',*,*,#25911,.T.);
#39129=ORIENTED_EDGE('',*,*,#28751,.T.);
#39130=ORIENTED_EDGE('',*,*,#28725,.F.);
#39131=ORIENTED_EDGE('',*,*,#28752,.F.);
#39132=ORIENTED_EDGE('',*,*,#27382,.T.);
#39133=ORIENTED_EDGE('',*,*,#27287,.T.);
#39134=ORIENTED_EDGE('',*,*,#28753,.F.);
#39135=ORIENTED_EDGE('',*,*,#28754,.F.);
#39136=ORIENTED_EDGE('',*,*,#25914,.T.);
#39137=ORIENTED_EDGE('',*,*,#26933,.T.);
#39138=ORIENTED_EDGE('',*,*,#28755,.F.);
#39139=ORIENTED_EDGE('',*,*,#28756,.F.);
#39140=ORIENTED_EDGE('',*,*,#25915,.T.);
#39141=ORIENTED_EDGE('',*,*,#28754,.T.);
#39142=ORIENTED_EDGE('',*,*,#28757,.F.);
#39143=ORIENTED_EDGE('',*,*,#28758,.F.);
#39144=ORIENTED_EDGE('',*,*,#25916,.T.);
#39145=ORIENTED_EDGE('',*,*,#28756,.T.);
#39146=ORIENTED_EDGE('',*,*,#28759,.F.);
#39147=ORIENTED_EDGE('',*,*,#28760,.F.);
#39148=ORIENTED_EDGE('',*,*,#25917,.T.);
#39149=ORIENTED_EDGE('',*,*,#28758,.T.);
#39150=ORIENTED_EDGE('',*,*,#28761,.F.);
#39151=ORIENTED_EDGE('',*,*,#28762,.F.);
#39152=ORIENTED_EDGE('',*,*,#25918,.T.);
#39153=ORIENTED_EDGE('',*,*,#28760,.T.);
#39154=ORIENTED_EDGE('',*,*,#28763,.F.);
#39155=ORIENTED_EDGE('',*,*,#28764,.F.);
#39156=ORIENTED_EDGE('',*,*,#25919,.T.);
#39157=ORIENTED_EDGE('',*,*,#28762,.T.);
#39158=ORIENTED_EDGE('',*,*,#28765,.F.);
#39159=ORIENTED_EDGE('',*,*,#28766,.F.);
#39160=ORIENTED_EDGE('',*,*,#25920,.T.);
#39161=ORIENTED_EDGE('',*,*,#28764,.T.);
#39162=ORIENTED_EDGE('',*,*,#28767,.F.);
#39163=ORIENTED_EDGE('',*,*,#28768,.F.);
#39164=ORIENTED_EDGE('',*,*,#25921,.T.);
#39165=ORIENTED_EDGE('',*,*,#28766,.T.);
#39166=ORIENTED_EDGE('',*,*,#28769,.F.);
#39167=ORIENTED_EDGE('',*,*,#28770,.F.);
#39168=ORIENTED_EDGE('',*,*,#25922,.T.);
#39169=ORIENTED_EDGE('',*,*,#28768,.T.);
#39170=ORIENTED_EDGE('',*,*,#28771,.F.);
#39171=ORIENTED_EDGE('',*,*,#28772,.F.);
#39172=ORIENTED_EDGE('',*,*,#25923,.T.);
#39173=ORIENTED_EDGE('',*,*,#28770,.T.);
#39174=ORIENTED_EDGE('',*,*,#28773,.F.);
#39175=ORIENTED_EDGE('',*,*,#28774,.F.);
#39176=ORIENTED_EDGE('',*,*,#25924,.T.);
#39177=ORIENTED_EDGE('',*,*,#28772,.T.);
#39178=ORIENTED_EDGE('',*,*,#28775,.F.);
#39179=ORIENTED_EDGE('',*,*,#28776,.F.);
#39180=ORIENTED_EDGE('',*,*,#25925,.T.);
#39181=ORIENTED_EDGE('',*,*,#28774,.T.);
#39182=ORIENTED_EDGE('',*,*,#28777,.F.);
#39183=ORIENTED_EDGE('',*,*,#27213,.F.);
#39184=ORIENTED_EDGE('',*,*,#25926,.T.);
#39185=ORIENTED_EDGE('',*,*,#28776,.T.);
#39186=ORIENTED_EDGE('',*,*,#27074,.T.);
#39187=ORIENTED_EDGE('',*,*,#27216,.F.);
#39188=ORIENTED_EDGE('',*,*,#27476,.F.);
#39189=ORIENTED_EDGE('',*,*,#25929,.F.);
#39190=ORIENTED_EDGE('',*,*,#27214,.T.);
#39191=ORIENTED_EDGE('',*,*,#28777,.T.);
#39192=ORIENTED_EDGE('',*,*,#28775,.T.);
#39193=ORIENTED_EDGE('',*,*,#28773,.T.);
#39194=ORIENTED_EDGE('',*,*,#28771,.T.);
#39195=ORIENTED_EDGE('',*,*,#28769,.T.);
#39196=ORIENTED_EDGE('',*,*,#28767,.T.);
#39197=ORIENTED_EDGE('',*,*,#28765,.T.);
#39198=ORIENTED_EDGE('',*,*,#28763,.T.);
#39199=ORIENTED_EDGE('',*,*,#28761,.T.);
#39200=ORIENTED_EDGE('',*,*,#28759,.T.);
#39201=ORIENTED_EDGE('',*,*,#28757,.T.);
#39202=ORIENTED_EDGE('',*,*,#28755,.T.);
#39203=ORIENTED_EDGE('',*,*,#28753,.T.);
#39204=ORIENTED_EDGE('',*,*,#26932,.T.);
#39205=ORIENTED_EDGE('',*,*,#28778,.F.);
#39206=ORIENTED_EDGE('',*,*,#28779,.T.);
#39207=ORIENTED_EDGE('',*,*,#28780,.T.);
#39208=ORIENTED_EDGE('',*,*,#28781,.T.);
#39209=ORIENTED_EDGE('',*,*,#28782,.T.);
#39210=ORIENTED_EDGE('',*,*,#28783,.T.);
#39211=ORIENTED_EDGE('',*,*,#28784,.T.);
#39212=ORIENTED_EDGE('',*,*,#28785,.T.);
#39213=ORIENTED_EDGE('',*,*,#28786,.T.);
#39214=ORIENTED_EDGE('',*,*,#28787,.T.);
#39215=ORIENTED_EDGE('',*,*,#28788,.T.);
#39216=ORIENTED_EDGE('',*,*,#28789,.T.);
#39217=ORIENTED_EDGE('',*,*,#28790,.T.);
#39218=ORIENTED_EDGE('',*,*,#28791,.T.);
#39219=ORIENTED_EDGE('',*,*,#28792,.T.);
#39220=ORIENTED_EDGE('',*,*,#25895,.T.);
#39221=ORIENTED_EDGE('',*,*,#27477,.T.);
#39222=ORIENTED_EDGE('',*,*,#28792,.F.);
#39223=ORIENTED_EDGE('',*,*,#28793,.F.);
#39224=ORIENTED_EDGE('',*,*,#25862,.T.);
#39225=ORIENTED_EDGE('',*,*,#25896,.T.);
#39226=ORIENTED_EDGE('',*,*,#28791,.F.);
#39227=ORIENTED_EDGE('',*,*,#28794,.F.);
#39228=ORIENTED_EDGE('',*,*,#25863,.T.);
#39229=ORIENTED_EDGE('',*,*,#28793,.T.);
#39230=ORIENTED_EDGE('',*,*,#28790,.F.);
#39231=ORIENTED_EDGE('',*,*,#28795,.F.);
#39232=ORIENTED_EDGE('',*,*,#25864,.T.);
#39233=ORIENTED_EDGE('',*,*,#28794,.T.);
#39234=ORIENTED_EDGE('',*,*,#28789,.F.);
#39235=ORIENTED_EDGE('',*,*,#28796,.F.);
#39236=ORIENTED_EDGE('',*,*,#25865,.T.);
#39237=ORIENTED_EDGE('',*,*,#28795,.T.);
#39238=ORIENTED_EDGE('',*,*,#28788,.F.);
#39239=ORIENTED_EDGE('',*,*,#28797,.F.);
#39240=ORIENTED_EDGE('',*,*,#25866,.T.);
#39241=ORIENTED_EDGE('',*,*,#28796,.T.);
#39242=ORIENTED_EDGE('',*,*,#28787,.F.);
#39243=ORIENTED_EDGE('',*,*,#28798,.F.);
#39244=ORIENTED_EDGE('',*,*,#25867,.T.);
#39245=ORIENTED_EDGE('',*,*,#28797,.T.);
#39246=ORIENTED_EDGE('',*,*,#28786,.F.);
#39247=ORIENTED_EDGE('',*,*,#28799,.F.);
#39248=ORIENTED_EDGE('',*,*,#25868,.T.);
#39249=ORIENTED_EDGE('',*,*,#28798,.T.);
#39250=ORIENTED_EDGE('',*,*,#28785,.F.);
#39251=ORIENTED_EDGE('',*,*,#28800,.F.);
#39252=ORIENTED_EDGE('',*,*,#25869,.T.);
#39253=ORIENTED_EDGE('',*,*,#28799,.T.);
#39254=ORIENTED_EDGE('',*,*,#28784,.F.);
#39255=ORIENTED_EDGE('',*,*,#28801,.F.);
#39256=ORIENTED_EDGE('',*,*,#25870,.T.);
#39257=ORIENTED_EDGE('',*,*,#28800,.T.);
#39258=ORIENTED_EDGE('',*,*,#28783,.F.);
#39259=ORIENTED_EDGE('',*,*,#28802,.F.);
#39260=ORIENTED_EDGE('',*,*,#25871,.T.);
#39261=ORIENTED_EDGE('',*,*,#28801,.T.);
#39262=ORIENTED_EDGE('',*,*,#28782,.F.);
#39263=ORIENTED_EDGE('',*,*,#28803,.F.);
#39264=ORIENTED_EDGE('',*,*,#25872,.T.);
#39265=ORIENTED_EDGE('',*,*,#28802,.T.);
#39266=ORIENTED_EDGE('',*,*,#28781,.F.);
#39267=ORIENTED_EDGE('',*,*,#28804,.F.);
#39268=ORIENTED_EDGE('',*,*,#25873,.T.);
#39269=ORIENTED_EDGE('',*,*,#28803,.T.);
#39270=ORIENTED_EDGE('',*,*,#28780,.F.);
#39271=ORIENTED_EDGE('',*,*,#28805,.F.);
#39272=ORIENTED_EDGE('',*,*,#25874,.T.);
#39273=ORIENTED_EDGE('',*,*,#28804,.T.);
#39274=ORIENTED_EDGE('',*,*,#26835,.T.);
#39275=ORIENTED_EDGE('',*,*,#25875,.T.);
#39276=ORIENTED_EDGE('',*,*,#28805,.T.);
#39277=ORIENTED_EDGE('',*,*,#28779,.F.);
#39278=ORIENTED_EDGE('',*,*,#28806,.F.);
#39279=ORIENTED_EDGE('',*,*,#27384,.T.);
#39280=ORIENTED_EDGE('',*,*,#27285,.T.);
#39281=ORIENTED_EDGE('',*,*,#28807,.F.);
#39282=ORIENTED_EDGE('',*,*,#28808,.F.);
#39283=ORIENTED_EDGE('',*,*,#25878,.T.);
#39284=ORIENTED_EDGE('',*,*,#26928,.T.);
#39285=ORIENTED_EDGE('',*,*,#28809,.F.);
#39286=ORIENTED_EDGE('',*,*,#28810,.F.);
#39287=ORIENTED_EDGE('',*,*,#25879,.T.);
#39288=ORIENTED_EDGE('',*,*,#28808,.T.);
#39289=ORIENTED_EDGE('',*,*,#28811,.F.);
#39290=ORIENTED_EDGE('',*,*,#28812,.F.);
#39291=ORIENTED_EDGE('',*,*,#25880,.T.);
#39292=ORIENTED_EDGE('',*,*,#28810,.T.);
#39293=ORIENTED_EDGE('',*,*,#28813,.F.);
#39294=ORIENTED_EDGE('',*,*,#28814,.F.);
#39295=ORIENTED_EDGE('',*,*,#25881,.T.);
#39296=ORIENTED_EDGE('',*,*,#28812,.T.);
#39297=ORIENTED_EDGE('',*,*,#28815,.F.);
#39298=ORIENTED_EDGE('',*,*,#28816,.F.);
#39299=ORIENTED_EDGE('',*,*,#25882,.T.);
#39300=ORIENTED_EDGE('',*,*,#28814,.T.);
#39301=ORIENTED_EDGE('',*,*,#28817,.F.);
#39302=ORIENTED_EDGE('',*,*,#28818,.F.);
#39303=ORIENTED_EDGE('',*,*,#25883,.T.);
#39304=ORIENTED_EDGE('',*,*,#28816,.T.);
#39305=ORIENTED_EDGE('',*,*,#28819,.F.);
#39306=ORIENTED_EDGE('',*,*,#28820,.F.);
#39307=ORIENTED_EDGE('',*,*,#25884,.T.);
#39308=ORIENTED_EDGE('',*,*,#28818,.T.);
#39309=ORIENTED_EDGE('',*,*,#28821,.F.);
#39310=ORIENTED_EDGE('',*,*,#28822,.F.);
#39311=ORIENTED_EDGE('',*,*,#25885,.T.);
#39312=ORIENTED_EDGE('',*,*,#28820,.T.);
#39313=ORIENTED_EDGE('',*,*,#28823,.F.);
#39314=ORIENTED_EDGE('',*,*,#28824,.F.);
#39315=ORIENTED_EDGE('',*,*,#25886,.T.);
#39316=ORIENTED_EDGE('',*,*,#28822,.T.);
#39317=ORIENTED_EDGE('',*,*,#28825,.F.);
#39318=ORIENTED_EDGE('',*,*,#28826,.F.);
#39319=ORIENTED_EDGE('',*,*,#25887,.T.);
#39320=ORIENTED_EDGE('',*,*,#28824,.T.);
#39321=ORIENTED_EDGE('',*,*,#28827,.F.);
#39322=ORIENTED_EDGE('',*,*,#28828,.F.);
#39323=ORIENTED_EDGE('',*,*,#25888,.T.);
#39324=ORIENTED_EDGE('',*,*,#28826,.T.);
#39325=ORIENTED_EDGE('',*,*,#28829,.F.);
#39326=ORIENTED_EDGE('',*,*,#28830,.F.);
#39327=ORIENTED_EDGE('',*,*,#25889,.T.);
#39328=ORIENTED_EDGE('',*,*,#28828,.T.);
#39329=ORIENTED_EDGE('',*,*,#28831,.F.);
#39330=ORIENTED_EDGE('',*,*,#27217,.F.);
#39331=ORIENTED_EDGE('',*,*,#25890,.T.);
#39332=ORIENTED_EDGE('',*,*,#28830,.T.);
#39333=ORIENTED_EDGE('',*,*,#27072,.T.);
#39334=ORIENTED_EDGE('',*,*,#27220,.F.);
#39335=ORIENTED_EDGE('',*,*,#27478,.F.);
#39336=ORIENTED_EDGE('',*,*,#25893,.F.);
#39337=ORIENTED_EDGE('',*,*,#27218,.T.);
#39338=ORIENTED_EDGE('',*,*,#28831,.T.);
#39339=ORIENTED_EDGE('',*,*,#28829,.T.);
#39340=ORIENTED_EDGE('',*,*,#28827,.T.);
#39341=ORIENTED_EDGE('',*,*,#28825,.T.);
#39342=ORIENTED_EDGE('',*,*,#28823,.T.);
#39343=ORIENTED_EDGE('',*,*,#28821,.T.);
#39344=ORIENTED_EDGE('',*,*,#28819,.T.);
#39345=ORIENTED_EDGE('',*,*,#28817,.T.);
#39346=ORIENTED_EDGE('',*,*,#28815,.T.);
#39347=ORIENTED_EDGE('',*,*,#28813,.T.);
#39348=ORIENTED_EDGE('',*,*,#28811,.T.);
#39349=ORIENTED_EDGE('',*,*,#28809,.T.);
#39350=ORIENTED_EDGE('',*,*,#28807,.T.);
#39351=ORIENTED_EDGE('',*,*,#26927,.T.);
#39352=ORIENTED_EDGE('',*,*,#28832,.F.);
#39353=ORIENTED_EDGE('',*,*,#28833,.T.);
#39354=ORIENTED_EDGE('',*,*,#28834,.T.);
#39355=ORIENTED_EDGE('',*,*,#28835,.T.);
#39356=ORIENTED_EDGE('',*,*,#28836,.T.);
#39357=ORIENTED_EDGE('',*,*,#28837,.T.);
#39358=ORIENTED_EDGE('',*,*,#28838,.T.);
#39359=ORIENTED_EDGE('',*,*,#28839,.T.);
#39360=ORIENTED_EDGE('',*,*,#28840,.T.);
#39361=ORIENTED_EDGE('',*,*,#28841,.T.);
#39362=ORIENTED_EDGE('',*,*,#28842,.T.);
#39363=ORIENTED_EDGE('',*,*,#28843,.T.);
#39364=ORIENTED_EDGE('',*,*,#28844,.T.);
#39365=ORIENTED_EDGE('',*,*,#28845,.T.);
#39366=ORIENTED_EDGE('',*,*,#28846,.T.);
#39367=ORIENTED_EDGE('',*,*,#25859,.T.);
#39368=ORIENTED_EDGE('',*,*,#27479,.T.);
#39369=ORIENTED_EDGE('',*,*,#28846,.F.);
#39370=ORIENTED_EDGE('',*,*,#28847,.F.);
#39371=ORIENTED_EDGE('',*,*,#25826,.T.);
#39372=ORIENTED_EDGE('',*,*,#25860,.T.);
#39373=ORIENTED_EDGE('',*,*,#28845,.F.);
#39374=ORIENTED_EDGE('',*,*,#28848,.F.);
#39375=ORIENTED_EDGE('',*,*,#25827,.T.);
#39376=ORIENTED_EDGE('',*,*,#28847,.T.);
#39377=ORIENTED_EDGE('',*,*,#28844,.F.);
#39378=ORIENTED_EDGE('',*,*,#28849,.F.);
#39379=ORIENTED_EDGE('',*,*,#25828,.T.);
#39380=ORIENTED_EDGE('',*,*,#28848,.T.);
#39381=ORIENTED_EDGE('',*,*,#28843,.F.);
#39382=ORIENTED_EDGE('',*,*,#28850,.F.);
#39383=ORIENTED_EDGE('',*,*,#25829,.T.);
#39384=ORIENTED_EDGE('',*,*,#28849,.T.);
#39385=ORIENTED_EDGE('',*,*,#28842,.F.);
#39386=ORIENTED_EDGE('',*,*,#28851,.F.);
#39387=ORIENTED_EDGE('',*,*,#25830,.T.);
#39388=ORIENTED_EDGE('',*,*,#28850,.T.);
#39389=ORIENTED_EDGE('',*,*,#28841,.F.);
#39390=ORIENTED_EDGE('',*,*,#28852,.F.);
#39391=ORIENTED_EDGE('',*,*,#25831,.T.);
#39392=ORIENTED_EDGE('',*,*,#28851,.T.);
#39393=ORIENTED_EDGE('',*,*,#28840,.F.);
#39394=ORIENTED_EDGE('',*,*,#28853,.F.);
#39395=ORIENTED_EDGE('',*,*,#25832,.T.);
#39396=ORIENTED_EDGE('',*,*,#28852,.T.);
#39397=ORIENTED_EDGE('',*,*,#28839,.F.);
#39398=ORIENTED_EDGE('',*,*,#28854,.F.);
#39399=ORIENTED_EDGE('',*,*,#25833,.T.);
#39400=ORIENTED_EDGE('',*,*,#28853,.T.);
#39401=ORIENTED_EDGE('',*,*,#28838,.F.);
#39402=ORIENTED_EDGE('',*,*,#28855,.F.);
#39403=ORIENTED_EDGE('',*,*,#25834,.T.);
#39404=ORIENTED_EDGE('',*,*,#28854,.T.);
#39405=ORIENTED_EDGE('',*,*,#28837,.F.);
#39406=ORIENTED_EDGE('',*,*,#28856,.F.);
#39407=ORIENTED_EDGE('',*,*,#25835,.T.);
#39408=ORIENTED_EDGE('',*,*,#28855,.T.);
#39409=ORIENTED_EDGE('',*,*,#28836,.F.);
#39410=ORIENTED_EDGE('',*,*,#28857,.F.);
#39411=ORIENTED_EDGE('',*,*,#25836,.T.);
#39412=ORIENTED_EDGE('',*,*,#28856,.T.);
#39413=ORIENTED_EDGE('',*,*,#28835,.F.);
#39414=ORIENTED_EDGE('',*,*,#28858,.F.);
#39415=ORIENTED_EDGE('',*,*,#25837,.T.);
#39416=ORIENTED_EDGE('',*,*,#28857,.T.);
#39417=ORIENTED_EDGE('',*,*,#28834,.F.);
#39418=ORIENTED_EDGE('',*,*,#28859,.F.);
#39419=ORIENTED_EDGE('',*,*,#25838,.T.);
#39420=ORIENTED_EDGE('',*,*,#28858,.T.);
#39421=ORIENTED_EDGE('',*,*,#26838,.T.);
#39422=ORIENTED_EDGE('',*,*,#25839,.T.);
#39423=ORIENTED_EDGE('',*,*,#28859,.T.);
#39424=ORIENTED_EDGE('',*,*,#28833,.F.);
#39425=ORIENTED_EDGE('',*,*,#28860,.F.);
#39426=ORIENTED_EDGE('',*,*,#27386,.T.);
#39427=ORIENTED_EDGE('',*,*,#27283,.T.);
#39428=ORIENTED_EDGE('',*,*,#28861,.F.);
#39429=ORIENTED_EDGE('',*,*,#28862,.F.);
#39430=ORIENTED_EDGE('',*,*,#25842,.T.);
#39431=ORIENTED_EDGE('',*,*,#26923,.T.);
#39432=ORIENTED_EDGE('',*,*,#28863,.F.);
#39433=ORIENTED_EDGE('',*,*,#28864,.F.);
#39434=ORIENTED_EDGE('',*,*,#25843,.T.);
#39435=ORIENTED_EDGE('',*,*,#28862,.T.);
#39436=ORIENTED_EDGE('',*,*,#28865,.F.);
#39437=ORIENTED_EDGE('',*,*,#28866,.F.);
#39438=ORIENTED_EDGE('',*,*,#25844,.T.);
#39439=ORIENTED_EDGE('',*,*,#28864,.T.);
#39440=ORIENTED_EDGE('',*,*,#28867,.F.);
#39441=ORIENTED_EDGE('',*,*,#28868,.F.);
#39442=ORIENTED_EDGE('',*,*,#25845,.T.);
#39443=ORIENTED_EDGE('',*,*,#28866,.T.);
#39444=ORIENTED_EDGE('',*,*,#28869,.F.);
#39445=ORIENTED_EDGE('',*,*,#28870,.F.);
#39446=ORIENTED_EDGE('',*,*,#25846,.T.);
#39447=ORIENTED_EDGE('',*,*,#28868,.T.);
#39448=ORIENTED_EDGE('',*,*,#28871,.F.);
#39449=ORIENTED_EDGE('',*,*,#28872,.F.);
#39450=ORIENTED_EDGE('',*,*,#25847,.T.);
#39451=ORIENTED_EDGE('',*,*,#28870,.T.);
#39452=ORIENTED_EDGE('',*,*,#28873,.F.);
#39453=ORIENTED_EDGE('',*,*,#28874,.F.);
#39454=ORIENTED_EDGE('',*,*,#25848,.T.);
#39455=ORIENTED_EDGE('',*,*,#28872,.T.);
#39456=ORIENTED_EDGE('',*,*,#28875,.F.);
#39457=ORIENTED_EDGE('',*,*,#28876,.F.);
#39458=ORIENTED_EDGE('',*,*,#25849,.T.);
#39459=ORIENTED_EDGE('',*,*,#28874,.T.);
#39460=ORIENTED_EDGE('',*,*,#28877,.F.);
#39461=ORIENTED_EDGE('',*,*,#28878,.F.);
#39462=ORIENTED_EDGE('',*,*,#25850,.T.);
#39463=ORIENTED_EDGE('',*,*,#28876,.T.);
#39464=ORIENTED_EDGE('',*,*,#28879,.F.);
#39465=ORIENTED_EDGE('',*,*,#28880,.F.);
#39466=ORIENTED_EDGE('',*,*,#25851,.T.);
#39467=ORIENTED_EDGE('',*,*,#28878,.T.);
#39468=ORIENTED_EDGE('',*,*,#28881,.F.);
#39469=ORIENTED_EDGE('',*,*,#28882,.F.);
#39470=ORIENTED_EDGE('',*,*,#25852,.T.);
#39471=ORIENTED_EDGE('',*,*,#28880,.T.);
#39472=ORIENTED_EDGE('',*,*,#28883,.F.);
#39473=ORIENTED_EDGE('',*,*,#28884,.F.);
#39474=ORIENTED_EDGE('',*,*,#25853,.T.);
#39475=ORIENTED_EDGE('',*,*,#28882,.T.);
#39476=ORIENTED_EDGE('',*,*,#28885,.F.);
#39477=ORIENTED_EDGE('',*,*,#27221,.F.);
#39478=ORIENTED_EDGE('',*,*,#25854,.T.);
#39479=ORIENTED_EDGE('',*,*,#28884,.T.);
#39480=ORIENTED_EDGE('',*,*,#27070,.T.);
#39481=ORIENTED_EDGE('',*,*,#27224,.F.);
#39482=ORIENTED_EDGE('',*,*,#27480,.F.);
#39483=ORIENTED_EDGE('',*,*,#25857,.F.);
#39484=ORIENTED_EDGE('',*,*,#27222,.T.);
#39485=ORIENTED_EDGE('',*,*,#28885,.T.);
#39486=ORIENTED_EDGE('',*,*,#28883,.T.);
#39487=ORIENTED_EDGE('',*,*,#28881,.T.);
#39488=ORIENTED_EDGE('',*,*,#28879,.T.);
#39489=ORIENTED_EDGE('',*,*,#28877,.T.);
#39490=ORIENTED_EDGE('',*,*,#28875,.T.);
#39491=ORIENTED_EDGE('',*,*,#28873,.T.);
#39492=ORIENTED_EDGE('',*,*,#28871,.T.);
#39493=ORIENTED_EDGE('',*,*,#28869,.T.);
#39494=ORIENTED_EDGE('',*,*,#28867,.T.);
#39495=ORIENTED_EDGE('',*,*,#28865,.T.);
#39496=ORIENTED_EDGE('',*,*,#28863,.T.);
#39497=ORIENTED_EDGE('',*,*,#28861,.T.);
#39498=ORIENTED_EDGE('',*,*,#26922,.T.);
#39499=ORIENTED_EDGE('',*,*,#28886,.F.);
#39500=ORIENTED_EDGE('',*,*,#28887,.T.);
#39501=ORIENTED_EDGE('',*,*,#28888,.T.);
#39502=ORIENTED_EDGE('',*,*,#28889,.T.);
#39503=ORIENTED_EDGE('',*,*,#28890,.T.);
#39504=ORIENTED_EDGE('',*,*,#28891,.T.);
#39505=ORIENTED_EDGE('',*,*,#28892,.T.);
#39506=ORIENTED_EDGE('',*,*,#28893,.T.);
#39507=ORIENTED_EDGE('',*,*,#28894,.T.);
#39508=ORIENTED_EDGE('',*,*,#28895,.T.);
#39509=ORIENTED_EDGE('',*,*,#28896,.T.);
#39510=ORIENTED_EDGE('',*,*,#28897,.T.);
#39511=ORIENTED_EDGE('',*,*,#28898,.T.);
#39512=ORIENTED_EDGE('',*,*,#28899,.T.);
#39513=ORIENTED_EDGE('',*,*,#28900,.T.);
#39514=ORIENTED_EDGE('',*,*,#25823,.T.);
#39515=ORIENTED_EDGE('',*,*,#27481,.T.);
#39516=ORIENTED_EDGE('',*,*,#28900,.F.);
#39517=ORIENTED_EDGE('',*,*,#28901,.F.);
#39518=ORIENTED_EDGE('',*,*,#25790,.T.);
#39519=ORIENTED_EDGE('',*,*,#25824,.T.);
#39520=ORIENTED_EDGE('',*,*,#28899,.F.);
#39521=ORIENTED_EDGE('',*,*,#28902,.F.);
#39522=ORIENTED_EDGE('',*,*,#25791,.T.);
#39523=ORIENTED_EDGE('',*,*,#28901,.T.);
#39524=ORIENTED_EDGE('',*,*,#28898,.F.);
#39525=ORIENTED_EDGE('',*,*,#28903,.F.);
#39526=ORIENTED_EDGE('',*,*,#25792,.T.);
#39527=ORIENTED_EDGE('',*,*,#28902,.T.);
#39528=ORIENTED_EDGE('',*,*,#28897,.F.);
#39529=ORIENTED_EDGE('',*,*,#28904,.F.);
#39530=ORIENTED_EDGE('',*,*,#25793,.T.);
#39531=ORIENTED_EDGE('',*,*,#28903,.T.);
#39532=ORIENTED_EDGE('',*,*,#28896,.F.);
#39533=ORIENTED_EDGE('',*,*,#28905,.F.);
#39534=ORIENTED_EDGE('',*,*,#25794,.T.);
#39535=ORIENTED_EDGE('',*,*,#28904,.T.);
#39536=ORIENTED_EDGE('',*,*,#28895,.F.);
#39537=ORIENTED_EDGE('',*,*,#28906,.F.);
#39538=ORIENTED_EDGE('',*,*,#25795,.T.);
#39539=ORIENTED_EDGE('',*,*,#28905,.T.);
#39540=ORIENTED_EDGE('',*,*,#28894,.F.);
#39541=ORIENTED_EDGE('',*,*,#28907,.F.);
#39542=ORIENTED_EDGE('',*,*,#25796,.T.);
#39543=ORIENTED_EDGE('',*,*,#28906,.T.);
#39544=ORIENTED_EDGE('',*,*,#28893,.F.);
#39545=ORIENTED_EDGE('',*,*,#28908,.F.);
#39546=ORIENTED_EDGE('',*,*,#25797,.T.);
#39547=ORIENTED_EDGE('',*,*,#28907,.T.);
#39548=ORIENTED_EDGE('',*,*,#28892,.F.);
#39549=ORIENTED_EDGE('',*,*,#28909,.F.);
#39550=ORIENTED_EDGE('',*,*,#25798,.T.);
#39551=ORIENTED_EDGE('',*,*,#28908,.T.);
#39552=ORIENTED_EDGE('',*,*,#28891,.F.);
#39553=ORIENTED_EDGE('',*,*,#28910,.F.);
#39554=ORIENTED_EDGE('',*,*,#25799,.T.);
#39555=ORIENTED_EDGE('',*,*,#28909,.T.);
#39556=ORIENTED_EDGE('',*,*,#28890,.F.);
#39557=ORIENTED_EDGE('',*,*,#28911,.F.);
#39558=ORIENTED_EDGE('',*,*,#25800,.T.);
#39559=ORIENTED_EDGE('',*,*,#28910,.T.);
#39560=ORIENTED_EDGE('',*,*,#28889,.F.);
#39561=ORIENTED_EDGE('',*,*,#28912,.F.);
#39562=ORIENTED_EDGE('',*,*,#25801,.T.);
#39563=ORIENTED_EDGE('',*,*,#28911,.T.);
#39564=ORIENTED_EDGE('',*,*,#28888,.F.);
#39565=ORIENTED_EDGE('',*,*,#28913,.F.);
#39566=ORIENTED_EDGE('',*,*,#25802,.T.);
#39567=ORIENTED_EDGE('',*,*,#28912,.T.);
#39568=ORIENTED_EDGE('',*,*,#26841,.T.);
#39569=ORIENTED_EDGE('',*,*,#25803,.T.);
#39570=ORIENTED_EDGE('',*,*,#28913,.T.);
#39571=ORIENTED_EDGE('',*,*,#28887,.F.);
#39572=ORIENTED_EDGE('',*,*,#28914,.F.);
#39573=ORIENTED_EDGE('',*,*,#27388,.T.);
#39574=ORIENTED_EDGE('',*,*,#27281,.T.);
#39575=ORIENTED_EDGE('',*,*,#28915,.F.);
#39576=ORIENTED_EDGE('',*,*,#28916,.F.);
#39577=ORIENTED_EDGE('',*,*,#25806,.T.);
#39578=ORIENTED_EDGE('',*,*,#26918,.T.);
#39579=ORIENTED_EDGE('',*,*,#28917,.F.);
#39580=ORIENTED_EDGE('',*,*,#28918,.F.);
#39581=ORIENTED_EDGE('',*,*,#25807,.T.);
#39582=ORIENTED_EDGE('',*,*,#28916,.T.);
#39583=ORIENTED_EDGE('',*,*,#28919,.F.);
#39584=ORIENTED_EDGE('',*,*,#28920,.F.);
#39585=ORIENTED_EDGE('',*,*,#25808,.T.);
#39586=ORIENTED_EDGE('',*,*,#28918,.T.);
#39587=ORIENTED_EDGE('',*,*,#28921,.F.);
#39588=ORIENTED_EDGE('',*,*,#28922,.F.);
#39589=ORIENTED_EDGE('',*,*,#25809,.T.);
#39590=ORIENTED_EDGE('',*,*,#28920,.T.);
#39591=ORIENTED_EDGE('',*,*,#28923,.F.);
#39592=ORIENTED_EDGE('',*,*,#28924,.F.);
#39593=ORIENTED_EDGE('',*,*,#25810,.T.);
#39594=ORIENTED_EDGE('',*,*,#28922,.T.);
#39595=ORIENTED_EDGE('',*,*,#28925,.F.);
#39596=ORIENTED_EDGE('',*,*,#28926,.F.);
#39597=ORIENTED_EDGE('',*,*,#25811,.T.);
#39598=ORIENTED_EDGE('',*,*,#28924,.T.);
#39599=ORIENTED_EDGE('',*,*,#28927,.F.);
#39600=ORIENTED_EDGE('',*,*,#28928,.F.);
#39601=ORIENTED_EDGE('',*,*,#25812,.T.);
#39602=ORIENTED_EDGE('',*,*,#28926,.T.);
#39603=ORIENTED_EDGE('',*,*,#28929,.F.);
#39604=ORIENTED_EDGE('',*,*,#28930,.F.);
#39605=ORIENTED_EDGE('',*,*,#25813,.T.);
#39606=ORIENTED_EDGE('',*,*,#28928,.T.);
#39607=ORIENTED_EDGE('',*,*,#28931,.F.);
#39608=ORIENTED_EDGE('',*,*,#28932,.F.);
#39609=ORIENTED_EDGE('',*,*,#25814,.T.);
#39610=ORIENTED_EDGE('',*,*,#28930,.T.);
#39611=ORIENTED_EDGE('',*,*,#28933,.F.);
#39612=ORIENTED_EDGE('',*,*,#28934,.F.);
#39613=ORIENTED_EDGE('',*,*,#25815,.T.);
#39614=ORIENTED_EDGE('',*,*,#28932,.T.);
#39615=ORIENTED_EDGE('',*,*,#28935,.F.);
#39616=ORIENTED_EDGE('',*,*,#28936,.F.);
#39617=ORIENTED_EDGE('',*,*,#25816,.T.);
#39618=ORIENTED_EDGE('',*,*,#28934,.T.);
#39619=ORIENTED_EDGE('',*,*,#28937,.F.);
#39620=ORIENTED_EDGE('',*,*,#28938,.F.);
#39621=ORIENTED_EDGE('',*,*,#25817,.T.);
#39622=ORIENTED_EDGE('',*,*,#28936,.T.);
#39623=ORIENTED_EDGE('',*,*,#28939,.F.);
#39624=ORIENTED_EDGE('',*,*,#27225,.F.);
#39625=ORIENTED_EDGE('',*,*,#25818,.T.);
#39626=ORIENTED_EDGE('',*,*,#28938,.T.);
#39627=ORIENTED_EDGE('',*,*,#27068,.T.);
#39628=ORIENTED_EDGE('',*,*,#27228,.F.);
#39629=ORIENTED_EDGE('',*,*,#27482,.F.);
#39630=ORIENTED_EDGE('',*,*,#25821,.F.);
#39631=ORIENTED_EDGE('',*,*,#27226,.T.);
#39632=ORIENTED_EDGE('',*,*,#28939,.T.);
#39633=ORIENTED_EDGE('',*,*,#28937,.T.);
#39634=ORIENTED_EDGE('',*,*,#28935,.T.);
#39635=ORIENTED_EDGE('',*,*,#28933,.T.);
#39636=ORIENTED_EDGE('',*,*,#28931,.T.);
#39637=ORIENTED_EDGE('',*,*,#28929,.T.);
#39638=ORIENTED_EDGE('',*,*,#28927,.T.);
#39639=ORIENTED_EDGE('',*,*,#28925,.T.);
#39640=ORIENTED_EDGE('',*,*,#28923,.T.);
#39641=ORIENTED_EDGE('',*,*,#28921,.T.);
#39642=ORIENTED_EDGE('',*,*,#28919,.T.);
#39643=ORIENTED_EDGE('',*,*,#28917,.T.);
#39644=ORIENTED_EDGE('',*,*,#28915,.T.);
#39645=ORIENTED_EDGE('',*,*,#26917,.T.);
#39646=ORIENTED_EDGE('',*,*,#28940,.F.);
#39647=ORIENTED_EDGE('',*,*,#28941,.T.);
#39648=ORIENTED_EDGE('',*,*,#28942,.T.);
#39649=ORIENTED_EDGE('',*,*,#28943,.T.);
#39650=ORIENTED_EDGE('',*,*,#28944,.T.);
#39651=ORIENTED_EDGE('',*,*,#28945,.T.);
#39652=ORIENTED_EDGE('',*,*,#28946,.T.);
#39653=ORIENTED_EDGE('',*,*,#28947,.T.);
#39654=ORIENTED_EDGE('',*,*,#28948,.T.);
#39655=ORIENTED_EDGE('',*,*,#28949,.T.);
#39656=ORIENTED_EDGE('',*,*,#28950,.T.);
#39657=ORIENTED_EDGE('',*,*,#28951,.T.);
#39658=ORIENTED_EDGE('',*,*,#28952,.T.);
#39659=ORIENTED_EDGE('',*,*,#28953,.T.);
#39660=ORIENTED_EDGE('',*,*,#28954,.T.);
#39661=ORIENTED_EDGE('',*,*,#25787,.T.);
#39662=ORIENTED_EDGE('',*,*,#27483,.T.);
#39663=ORIENTED_EDGE('',*,*,#28954,.F.);
#39664=ORIENTED_EDGE('',*,*,#28955,.F.);
#39665=ORIENTED_EDGE('',*,*,#25754,.T.);
#39666=ORIENTED_EDGE('',*,*,#25788,.T.);
#39667=ORIENTED_EDGE('',*,*,#28953,.F.);
#39668=ORIENTED_EDGE('',*,*,#28956,.F.);
#39669=ORIENTED_EDGE('',*,*,#25755,.T.);
#39670=ORIENTED_EDGE('',*,*,#28955,.T.);
#39671=ORIENTED_EDGE('',*,*,#28952,.F.);
#39672=ORIENTED_EDGE('',*,*,#28957,.F.);
#39673=ORIENTED_EDGE('',*,*,#25756,.T.);
#39674=ORIENTED_EDGE('',*,*,#28956,.T.);
#39675=ORIENTED_EDGE('',*,*,#28951,.F.);
#39676=ORIENTED_EDGE('',*,*,#28958,.F.);
#39677=ORIENTED_EDGE('',*,*,#25757,.T.);
#39678=ORIENTED_EDGE('',*,*,#28957,.T.);
#39679=ORIENTED_EDGE('',*,*,#28950,.F.);
#39680=ORIENTED_EDGE('',*,*,#28959,.F.);
#39681=ORIENTED_EDGE('',*,*,#25758,.T.);
#39682=ORIENTED_EDGE('',*,*,#28958,.T.);
#39683=ORIENTED_EDGE('',*,*,#28949,.F.);
#39684=ORIENTED_EDGE('',*,*,#28960,.F.);
#39685=ORIENTED_EDGE('',*,*,#25759,.T.);
#39686=ORIENTED_EDGE('',*,*,#28959,.T.);
#39687=ORIENTED_EDGE('',*,*,#28948,.F.);
#39688=ORIENTED_EDGE('',*,*,#28961,.F.);
#39689=ORIENTED_EDGE('',*,*,#25760,.T.);
#39690=ORIENTED_EDGE('',*,*,#28960,.T.);
#39691=ORIENTED_EDGE('',*,*,#28947,.F.);
#39692=ORIENTED_EDGE('',*,*,#28962,.F.);
#39693=ORIENTED_EDGE('',*,*,#25761,.T.);
#39694=ORIENTED_EDGE('',*,*,#28961,.T.);
#39695=ORIENTED_EDGE('',*,*,#28946,.F.);
#39696=ORIENTED_EDGE('',*,*,#28963,.F.);
#39697=ORIENTED_EDGE('',*,*,#25762,.T.);
#39698=ORIENTED_EDGE('',*,*,#28962,.T.);
#39699=ORIENTED_EDGE('',*,*,#28945,.F.);
#39700=ORIENTED_EDGE('',*,*,#28964,.F.);
#39701=ORIENTED_EDGE('',*,*,#25763,.T.);
#39702=ORIENTED_EDGE('',*,*,#28963,.T.);
#39703=ORIENTED_EDGE('',*,*,#28944,.F.);
#39704=ORIENTED_EDGE('',*,*,#28965,.F.);
#39705=ORIENTED_EDGE('',*,*,#25764,.T.);
#39706=ORIENTED_EDGE('',*,*,#28964,.T.);
#39707=ORIENTED_EDGE('',*,*,#28943,.F.);
#39708=ORIENTED_EDGE('',*,*,#28966,.F.);
#39709=ORIENTED_EDGE('',*,*,#25765,.T.);
#39710=ORIENTED_EDGE('',*,*,#28965,.T.);
#39711=ORIENTED_EDGE('',*,*,#28942,.F.);
#39712=ORIENTED_EDGE('',*,*,#28967,.F.);
#39713=ORIENTED_EDGE('',*,*,#25766,.T.);
#39714=ORIENTED_EDGE('',*,*,#28966,.T.);
#39715=ORIENTED_EDGE('',*,*,#26844,.T.);
#39716=ORIENTED_EDGE('',*,*,#25767,.T.);
#39717=ORIENTED_EDGE('',*,*,#28967,.T.);
#39718=ORIENTED_EDGE('',*,*,#28941,.F.);
#39719=ORIENTED_EDGE('',*,*,#28968,.F.);
#39720=ORIENTED_EDGE('',*,*,#27390,.T.);
#39721=ORIENTED_EDGE('',*,*,#27279,.T.);
#39722=ORIENTED_EDGE('',*,*,#28969,.F.);
#39723=ORIENTED_EDGE('',*,*,#28970,.F.);
#39724=ORIENTED_EDGE('',*,*,#25770,.T.);
#39725=ORIENTED_EDGE('',*,*,#26913,.T.);
#39726=ORIENTED_EDGE('',*,*,#28971,.F.);
#39727=ORIENTED_EDGE('',*,*,#28972,.F.);
#39728=ORIENTED_EDGE('',*,*,#25771,.T.);
#39729=ORIENTED_EDGE('',*,*,#28970,.T.);
#39730=ORIENTED_EDGE('',*,*,#28973,.F.);
#39731=ORIENTED_EDGE('',*,*,#28974,.F.);
#39732=ORIENTED_EDGE('',*,*,#25772,.T.);
#39733=ORIENTED_EDGE('',*,*,#28972,.T.);
#39734=ORIENTED_EDGE('',*,*,#28975,.F.);
#39735=ORIENTED_EDGE('',*,*,#28976,.F.);
#39736=ORIENTED_EDGE('',*,*,#25773,.T.);
#39737=ORIENTED_EDGE('',*,*,#28974,.T.);
#39738=ORIENTED_EDGE('',*,*,#28977,.F.);
#39739=ORIENTED_EDGE('',*,*,#28978,.F.);
#39740=ORIENTED_EDGE('',*,*,#25774,.T.);
#39741=ORIENTED_EDGE('',*,*,#28976,.T.);
#39742=ORIENTED_EDGE('',*,*,#28979,.F.);
#39743=ORIENTED_EDGE('',*,*,#28980,.F.);
#39744=ORIENTED_EDGE('',*,*,#25775,.T.);
#39745=ORIENTED_EDGE('',*,*,#28978,.T.);
#39746=ORIENTED_EDGE('',*,*,#28981,.F.);
#39747=ORIENTED_EDGE('',*,*,#28982,.F.);
#39748=ORIENTED_EDGE('',*,*,#25776,.T.);
#39749=ORIENTED_EDGE('',*,*,#28980,.T.);
#39750=ORIENTED_EDGE('',*,*,#28983,.F.);
#39751=ORIENTED_EDGE('',*,*,#28984,.F.);
#39752=ORIENTED_EDGE('',*,*,#25777,.T.);
#39753=ORIENTED_EDGE('',*,*,#28982,.T.);
#39754=ORIENTED_EDGE('',*,*,#28985,.F.);
#39755=ORIENTED_EDGE('',*,*,#28986,.F.);
#39756=ORIENTED_EDGE('',*,*,#25778,.T.);
#39757=ORIENTED_EDGE('',*,*,#28984,.T.);
#39758=ORIENTED_EDGE('',*,*,#28987,.F.);
#39759=ORIENTED_EDGE('',*,*,#28988,.F.);
#39760=ORIENTED_EDGE('',*,*,#25779,.T.);
#39761=ORIENTED_EDGE('',*,*,#28986,.T.);
#39762=ORIENTED_EDGE('',*,*,#28989,.F.);
#39763=ORIENTED_EDGE('',*,*,#28990,.F.);
#39764=ORIENTED_EDGE('',*,*,#25780,.T.);
#39765=ORIENTED_EDGE('',*,*,#28988,.T.);
#39766=ORIENTED_EDGE('',*,*,#28991,.F.);
#39767=ORIENTED_EDGE('',*,*,#28992,.F.);
#39768=ORIENTED_EDGE('',*,*,#25781,.T.);
#39769=ORIENTED_EDGE('',*,*,#28990,.T.);
#39770=ORIENTED_EDGE('',*,*,#28993,.F.);
#39771=ORIENTED_EDGE('',*,*,#27229,.F.);
#39772=ORIENTED_EDGE('',*,*,#25782,.T.);
#39773=ORIENTED_EDGE('',*,*,#28992,.T.);
#39774=ORIENTED_EDGE('',*,*,#27066,.T.);
#39775=ORIENTED_EDGE('',*,*,#27232,.F.);
#39776=ORIENTED_EDGE('',*,*,#27484,.F.);
#39777=ORIENTED_EDGE('',*,*,#25785,.F.);
#39778=ORIENTED_EDGE('',*,*,#27230,.T.);
#39779=ORIENTED_EDGE('',*,*,#28993,.T.);
#39780=ORIENTED_EDGE('',*,*,#28991,.T.);
#39781=ORIENTED_EDGE('',*,*,#28989,.T.);
#39782=ORIENTED_EDGE('',*,*,#28987,.T.);
#39783=ORIENTED_EDGE('',*,*,#28985,.T.);
#39784=ORIENTED_EDGE('',*,*,#28983,.T.);
#39785=ORIENTED_EDGE('',*,*,#28981,.T.);
#39786=ORIENTED_EDGE('',*,*,#28979,.T.);
#39787=ORIENTED_EDGE('',*,*,#28977,.T.);
#39788=ORIENTED_EDGE('',*,*,#28975,.T.);
#39789=ORIENTED_EDGE('',*,*,#28973,.T.);
#39790=ORIENTED_EDGE('',*,*,#28971,.T.);
#39791=ORIENTED_EDGE('',*,*,#28969,.T.);
#39792=ORIENTED_EDGE('',*,*,#26912,.T.);
#39793=ORIENTED_EDGE('',*,*,#28994,.F.);
#39794=ORIENTED_EDGE('',*,*,#28995,.T.);
#39795=ORIENTED_EDGE('',*,*,#28996,.T.);
#39796=ORIENTED_EDGE('',*,*,#28997,.T.);
#39797=ORIENTED_EDGE('',*,*,#28998,.T.);
#39798=ORIENTED_EDGE('',*,*,#28999,.T.);
#39799=ORIENTED_EDGE('',*,*,#29000,.T.);
#39800=ORIENTED_EDGE('',*,*,#29001,.T.);
#39801=ORIENTED_EDGE('',*,*,#29002,.T.);
#39802=ORIENTED_EDGE('',*,*,#29003,.T.);
#39803=ORIENTED_EDGE('',*,*,#29004,.T.);
#39804=ORIENTED_EDGE('',*,*,#29005,.T.);
#39805=ORIENTED_EDGE('',*,*,#29006,.T.);
#39806=ORIENTED_EDGE('',*,*,#29007,.T.);
#39807=ORIENTED_EDGE('',*,*,#29008,.T.);
#39808=ORIENTED_EDGE('',*,*,#25751,.T.);
#39809=ORIENTED_EDGE('',*,*,#27485,.T.);
#39810=ORIENTED_EDGE('',*,*,#29008,.F.);
#39811=ORIENTED_EDGE('',*,*,#29009,.F.);
#39812=ORIENTED_EDGE('',*,*,#25718,.T.);
#39813=ORIENTED_EDGE('',*,*,#25752,.T.);
#39814=ORIENTED_EDGE('',*,*,#29007,.F.);
#39815=ORIENTED_EDGE('',*,*,#29010,.F.);
#39816=ORIENTED_EDGE('',*,*,#25719,.T.);
#39817=ORIENTED_EDGE('',*,*,#29009,.T.);
#39818=ORIENTED_EDGE('',*,*,#29006,.F.);
#39819=ORIENTED_EDGE('',*,*,#29011,.F.);
#39820=ORIENTED_EDGE('',*,*,#25720,.T.);
#39821=ORIENTED_EDGE('',*,*,#29010,.T.);
#39822=ORIENTED_EDGE('',*,*,#29005,.F.);
#39823=ORIENTED_EDGE('',*,*,#29012,.F.);
#39824=ORIENTED_EDGE('',*,*,#25721,.T.);
#39825=ORIENTED_EDGE('',*,*,#29011,.T.);
#39826=ORIENTED_EDGE('',*,*,#29004,.F.);
#39827=ORIENTED_EDGE('',*,*,#29013,.F.);
#39828=ORIENTED_EDGE('',*,*,#25722,.T.);
#39829=ORIENTED_EDGE('',*,*,#29012,.T.);
#39830=ORIENTED_EDGE('',*,*,#29003,.F.);
#39831=ORIENTED_EDGE('',*,*,#29014,.F.);
#39832=ORIENTED_EDGE('',*,*,#25723,.T.);
#39833=ORIENTED_EDGE('',*,*,#29013,.T.);
#39834=ORIENTED_EDGE('',*,*,#29002,.F.);
#39835=ORIENTED_EDGE('',*,*,#29015,.F.);
#39836=ORIENTED_EDGE('',*,*,#25724,.T.);
#39837=ORIENTED_EDGE('',*,*,#29014,.T.);
#39838=ORIENTED_EDGE('',*,*,#29001,.F.);
#39839=ORIENTED_EDGE('',*,*,#29016,.F.);
#39840=ORIENTED_EDGE('',*,*,#25725,.T.);
#39841=ORIENTED_EDGE('',*,*,#29015,.T.);
#39842=ORIENTED_EDGE('',*,*,#29000,.F.);
#39843=ORIENTED_EDGE('',*,*,#29017,.F.);
#39844=ORIENTED_EDGE('',*,*,#25726,.T.);
#39845=ORIENTED_EDGE('',*,*,#29016,.T.);
#39846=ORIENTED_EDGE('',*,*,#28999,.F.);
#39847=ORIENTED_EDGE('',*,*,#29018,.F.);
#39848=ORIENTED_EDGE('',*,*,#25727,.T.);
#39849=ORIENTED_EDGE('',*,*,#29017,.T.);
#39850=ORIENTED_EDGE('',*,*,#28998,.F.);
#39851=ORIENTED_EDGE('',*,*,#29019,.F.);
#39852=ORIENTED_EDGE('',*,*,#25728,.T.);
#39853=ORIENTED_EDGE('',*,*,#29018,.T.);
#39854=ORIENTED_EDGE('',*,*,#28997,.F.);
#39855=ORIENTED_EDGE('',*,*,#29020,.F.);
#39856=ORIENTED_EDGE('',*,*,#25729,.T.);
#39857=ORIENTED_EDGE('',*,*,#29019,.T.);
#39858=ORIENTED_EDGE('',*,*,#28996,.F.);
#39859=ORIENTED_EDGE('',*,*,#29021,.F.);
#39860=ORIENTED_EDGE('',*,*,#25730,.T.);
#39861=ORIENTED_EDGE('',*,*,#29020,.T.);
#39862=ORIENTED_EDGE('',*,*,#26847,.T.);
#39863=ORIENTED_EDGE('',*,*,#25731,.T.);
#39864=ORIENTED_EDGE('',*,*,#29021,.T.);
#39865=ORIENTED_EDGE('',*,*,#28995,.F.);
#39866=ORIENTED_EDGE('',*,*,#29022,.F.);
#39867=ORIENTED_EDGE('',*,*,#27392,.T.);
#39868=ORIENTED_EDGE('',*,*,#27277,.T.);
#39869=ORIENTED_EDGE('',*,*,#29023,.F.);
#39870=ORIENTED_EDGE('',*,*,#29024,.F.);
#39871=ORIENTED_EDGE('',*,*,#25734,.T.);
#39872=ORIENTED_EDGE('',*,*,#26908,.T.);
#39873=ORIENTED_EDGE('',*,*,#29025,.F.);
#39874=ORIENTED_EDGE('',*,*,#29026,.F.);
#39875=ORIENTED_EDGE('',*,*,#25735,.T.);
#39876=ORIENTED_EDGE('',*,*,#29024,.T.);
#39877=ORIENTED_EDGE('',*,*,#29027,.F.);
#39878=ORIENTED_EDGE('',*,*,#29028,.F.);
#39879=ORIENTED_EDGE('',*,*,#25736,.T.);
#39880=ORIENTED_EDGE('',*,*,#29026,.T.);
#39881=ORIENTED_EDGE('',*,*,#29029,.F.);
#39882=ORIENTED_EDGE('',*,*,#29030,.F.);
#39883=ORIENTED_EDGE('',*,*,#25737,.T.);
#39884=ORIENTED_EDGE('',*,*,#29028,.T.);
#39885=ORIENTED_EDGE('',*,*,#29031,.F.);
#39886=ORIENTED_EDGE('',*,*,#29032,.F.);
#39887=ORIENTED_EDGE('',*,*,#25738,.T.);
#39888=ORIENTED_EDGE('',*,*,#29030,.T.);
#39889=ORIENTED_EDGE('',*,*,#29033,.F.);
#39890=ORIENTED_EDGE('',*,*,#29034,.F.);
#39891=ORIENTED_EDGE('',*,*,#25739,.T.);
#39892=ORIENTED_EDGE('',*,*,#29032,.T.);
#39893=ORIENTED_EDGE('',*,*,#29035,.F.);
#39894=ORIENTED_EDGE('',*,*,#29036,.F.);
#39895=ORIENTED_EDGE('',*,*,#25740,.T.);
#39896=ORIENTED_EDGE('',*,*,#29034,.T.);
#39897=ORIENTED_EDGE('',*,*,#29037,.F.);
#39898=ORIENTED_EDGE('',*,*,#29038,.F.);
#39899=ORIENTED_EDGE('',*,*,#25741,.T.);
#39900=ORIENTED_EDGE('',*,*,#29036,.T.);
#39901=ORIENTED_EDGE('',*,*,#29039,.F.);
#39902=ORIENTED_EDGE('',*,*,#29040,.F.);
#39903=ORIENTED_EDGE('',*,*,#25742,.T.);
#39904=ORIENTED_EDGE('',*,*,#29038,.T.);
#39905=ORIENTED_EDGE('',*,*,#29041,.F.);
#39906=ORIENTED_EDGE('',*,*,#29042,.F.);
#39907=ORIENTED_EDGE('',*,*,#25743,.T.);
#39908=ORIENTED_EDGE('',*,*,#29040,.T.);
#39909=ORIENTED_EDGE('',*,*,#29043,.F.);
#39910=ORIENTED_EDGE('',*,*,#29044,.F.);
#39911=ORIENTED_EDGE('',*,*,#25744,.T.);
#39912=ORIENTED_EDGE('',*,*,#29042,.T.);
#39913=ORIENTED_EDGE('',*,*,#29045,.F.);
#39914=ORIENTED_EDGE('',*,*,#29046,.F.);
#39915=ORIENTED_EDGE('',*,*,#25745,.T.);
#39916=ORIENTED_EDGE('',*,*,#29044,.T.);
#39917=ORIENTED_EDGE('',*,*,#29047,.F.);
#39918=ORIENTED_EDGE('',*,*,#27233,.F.);
#39919=ORIENTED_EDGE('',*,*,#25746,.T.);
#39920=ORIENTED_EDGE('',*,*,#29046,.T.);
#39921=ORIENTED_EDGE('',*,*,#27064,.T.);
#39922=ORIENTED_EDGE('',*,*,#27236,.F.);
#39923=ORIENTED_EDGE('',*,*,#27486,.F.);
#39924=ORIENTED_EDGE('',*,*,#25749,.F.);
#39925=ORIENTED_EDGE('',*,*,#27234,.T.);
#39926=ORIENTED_EDGE('',*,*,#29047,.T.);
#39927=ORIENTED_EDGE('',*,*,#29045,.T.);
#39928=ORIENTED_EDGE('',*,*,#29043,.T.);
#39929=ORIENTED_EDGE('',*,*,#29041,.T.);
#39930=ORIENTED_EDGE('',*,*,#29039,.T.);
#39931=ORIENTED_EDGE('',*,*,#29037,.T.);
#39932=ORIENTED_EDGE('',*,*,#29035,.T.);
#39933=ORIENTED_EDGE('',*,*,#29033,.T.);
#39934=ORIENTED_EDGE('',*,*,#29031,.T.);
#39935=ORIENTED_EDGE('',*,*,#29029,.T.);
#39936=ORIENTED_EDGE('',*,*,#29027,.T.);
#39937=ORIENTED_EDGE('',*,*,#29025,.T.);
#39938=ORIENTED_EDGE('',*,*,#29023,.T.);
#39939=ORIENTED_EDGE('',*,*,#26907,.T.);
#39940=ORIENTED_EDGE('',*,*,#29048,.F.);
#39941=ORIENTED_EDGE('',*,*,#29049,.T.);
#39942=ORIENTED_EDGE('',*,*,#29050,.T.);
#39943=ORIENTED_EDGE('',*,*,#29051,.T.);
#39944=ORIENTED_EDGE('',*,*,#29052,.T.);
#39945=ORIENTED_EDGE('',*,*,#29053,.T.);
#39946=ORIENTED_EDGE('',*,*,#29054,.T.);
#39947=ORIENTED_EDGE('',*,*,#29055,.T.);
#39948=ORIENTED_EDGE('',*,*,#29056,.T.);
#39949=ORIENTED_EDGE('',*,*,#29057,.T.);
#39950=ORIENTED_EDGE('',*,*,#29058,.T.);
#39951=ORIENTED_EDGE('',*,*,#29059,.T.);
#39952=ORIENTED_EDGE('',*,*,#29060,.T.);
#39953=ORIENTED_EDGE('',*,*,#29061,.T.);
#39954=ORIENTED_EDGE('',*,*,#29062,.T.);
#39955=ORIENTED_EDGE('',*,*,#25715,.T.);
#39956=ORIENTED_EDGE('',*,*,#27487,.T.);
#39957=ORIENTED_EDGE('',*,*,#29062,.F.);
#39958=ORIENTED_EDGE('',*,*,#29063,.F.);
#39959=ORIENTED_EDGE('',*,*,#25682,.T.);
#39960=ORIENTED_EDGE('',*,*,#25716,.T.);
#39961=ORIENTED_EDGE('',*,*,#29061,.F.);
#39962=ORIENTED_EDGE('',*,*,#29064,.F.);
#39963=ORIENTED_EDGE('',*,*,#25683,.T.);
#39964=ORIENTED_EDGE('',*,*,#29063,.T.);
#39965=ORIENTED_EDGE('',*,*,#29060,.F.);
#39966=ORIENTED_EDGE('',*,*,#29065,.F.);
#39967=ORIENTED_EDGE('',*,*,#25684,.T.);
#39968=ORIENTED_EDGE('',*,*,#29064,.T.);
#39969=ORIENTED_EDGE('',*,*,#29059,.F.);
#39970=ORIENTED_EDGE('',*,*,#29066,.F.);
#39971=ORIENTED_EDGE('',*,*,#25685,.T.);
#39972=ORIENTED_EDGE('',*,*,#29065,.T.);
#39973=ORIENTED_EDGE('',*,*,#29058,.F.);
#39974=ORIENTED_EDGE('',*,*,#29067,.F.);
#39975=ORIENTED_EDGE('',*,*,#25686,.T.);
#39976=ORIENTED_EDGE('',*,*,#29066,.T.);
#39977=ORIENTED_EDGE('',*,*,#29057,.F.);
#39978=ORIENTED_EDGE('',*,*,#29068,.F.);
#39979=ORIENTED_EDGE('',*,*,#25687,.T.);
#39980=ORIENTED_EDGE('',*,*,#29067,.T.);
#39981=ORIENTED_EDGE('',*,*,#29056,.F.);
#39982=ORIENTED_EDGE('',*,*,#29069,.F.);
#39983=ORIENTED_EDGE('',*,*,#25688,.T.);
#39984=ORIENTED_EDGE('',*,*,#29068,.T.);
#39985=ORIENTED_EDGE('',*,*,#29055,.F.);
#39986=ORIENTED_EDGE('',*,*,#29070,.F.);
#39987=ORIENTED_EDGE('',*,*,#25689,.T.);
#39988=ORIENTED_EDGE('',*,*,#29069,.T.);
#39989=ORIENTED_EDGE('',*,*,#29054,.F.);
#39990=ORIENTED_EDGE('',*,*,#29071,.F.);
#39991=ORIENTED_EDGE('',*,*,#25690,.T.);
#39992=ORIENTED_EDGE('',*,*,#29070,.T.);
#39993=ORIENTED_EDGE('',*,*,#29053,.F.);
#39994=ORIENTED_EDGE('',*,*,#29072,.F.);
#39995=ORIENTED_EDGE('',*,*,#25691,.T.);
#39996=ORIENTED_EDGE('',*,*,#29071,.T.);
#39997=ORIENTED_EDGE('',*,*,#29052,.F.);
#39998=ORIENTED_EDGE('',*,*,#29073,.F.);
#39999=ORIENTED_EDGE('',*,*,#25692,.T.);
#40000=ORIENTED_EDGE('',*,*,#29072,.T.);
#40001=ORIENTED_EDGE('',*,*,#29051,.F.);
#40002=ORIENTED_EDGE('',*,*,#29074,.F.);
#40003=ORIENTED_EDGE('',*,*,#25693,.T.);
#40004=ORIENTED_EDGE('',*,*,#29073,.T.);
#40005=ORIENTED_EDGE('',*,*,#29050,.F.);
#40006=ORIENTED_EDGE('',*,*,#29075,.F.);
#40007=ORIENTED_EDGE('',*,*,#25694,.T.);
#40008=ORIENTED_EDGE('',*,*,#29074,.T.);
#40009=ORIENTED_EDGE('',*,*,#26850,.T.);
#40010=ORIENTED_EDGE('',*,*,#25695,.T.);
#40011=ORIENTED_EDGE('',*,*,#29075,.T.);
#40012=ORIENTED_EDGE('',*,*,#29049,.F.);
#40013=ORIENTED_EDGE('',*,*,#29076,.F.);
#40014=ORIENTED_EDGE('',*,*,#27394,.T.);
#40015=ORIENTED_EDGE('',*,*,#27275,.T.);
#40016=ORIENTED_EDGE('',*,*,#29077,.F.);
#40017=ORIENTED_EDGE('',*,*,#29078,.F.);
#40018=ORIENTED_EDGE('',*,*,#25698,.T.);
#40019=ORIENTED_EDGE('',*,*,#26903,.T.);
#40020=ORIENTED_EDGE('',*,*,#29079,.F.);
#40021=ORIENTED_EDGE('',*,*,#29080,.F.);
#40022=ORIENTED_EDGE('',*,*,#25699,.T.);
#40023=ORIENTED_EDGE('',*,*,#29078,.T.);
#40024=ORIENTED_EDGE('',*,*,#29081,.F.);
#40025=ORIENTED_EDGE('',*,*,#29082,.F.);
#40026=ORIENTED_EDGE('',*,*,#25700,.T.);
#40027=ORIENTED_EDGE('',*,*,#29080,.T.);
#40028=ORIENTED_EDGE('',*,*,#29083,.F.);
#40029=ORIENTED_EDGE('',*,*,#29084,.F.);
#40030=ORIENTED_EDGE('',*,*,#25701,.T.);
#40031=ORIENTED_EDGE('',*,*,#29082,.T.);
#40032=ORIENTED_EDGE('',*,*,#29085,.F.);
#40033=ORIENTED_EDGE('',*,*,#29086,.F.);
#40034=ORIENTED_EDGE('',*,*,#25702,.T.);
#40035=ORIENTED_EDGE('',*,*,#29084,.T.);
#40036=ORIENTED_EDGE('',*,*,#29087,.F.);
#40037=ORIENTED_EDGE('',*,*,#29088,.F.);
#40038=ORIENTED_EDGE('',*,*,#25703,.T.);
#40039=ORIENTED_EDGE('',*,*,#29086,.T.);
#40040=ORIENTED_EDGE('',*,*,#29089,.F.);
#40041=ORIENTED_EDGE('',*,*,#29090,.F.);
#40042=ORIENTED_EDGE('',*,*,#25704,.T.);
#40043=ORIENTED_EDGE('',*,*,#29088,.T.);
#40044=ORIENTED_EDGE('',*,*,#29091,.F.);
#40045=ORIENTED_EDGE('',*,*,#29092,.F.);
#40046=ORIENTED_EDGE('',*,*,#25705,.T.);
#40047=ORIENTED_EDGE('',*,*,#29090,.T.);
#40048=ORIENTED_EDGE('',*,*,#29093,.F.);
#40049=ORIENTED_EDGE('',*,*,#29094,.F.);
#40050=ORIENTED_EDGE('',*,*,#25706,.T.);
#40051=ORIENTED_EDGE('',*,*,#29092,.T.);
#40052=ORIENTED_EDGE('',*,*,#29095,.F.);
#40053=ORIENTED_EDGE('',*,*,#29096,.F.);
#40054=ORIENTED_EDGE('',*,*,#25707,.T.);
#40055=ORIENTED_EDGE('',*,*,#29094,.T.);
#40056=ORIENTED_EDGE('',*,*,#29097,.F.);
#40057=ORIENTED_EDGE('',*,*,#29098,.F.);
#40058=ORIENTED_EDGE('',*,*,#25708,.T.);
#40059=ORIENTED_EDGE('',*,*,#29096,.T.);
#40060=ORIENTED_EDGE('',*,*,#29099,.F.);
#40061=ORIENTED_EDGE('',*,*,#29100,.F.);
#40062=ORIENTED_EDGE('',*,*,#25709,.T.);
#40063=ORIENTED_EDGE('',*,*,#29098,.T.);
#40064=ORIENTED_EDGE('',*,*,#29101,.F.);
#40065=ORIENTED_EDGE('',*,*,#27237,.F.);
#40066=ORIENTED_EDGE('',*,*,#25710,.T.);
#40067=ORIENTED_EDGE('',*,*,#29100,.T.);
#40068=ORIENTED_EDGE('',*,*,#27062,.T.);
#40069=ORIENTED_EDGE('',*,*,#27240,.F.);
#40070=ORIENTED_EDGE('',*,*,#27488,.F.);
#40071=ORIENTED_EDGE('',*,*,#25713,.F.);
#40072=ORIENTED_EDGE('',*,*,#27238,.T.);
#40073=ORIENTED_EDGE('',*,*,#29101,.T.);
#40074=ORIENTED_EDGE('',*,*,#29099,.T.);
#40075=ORIENTED_EDGE('',*,*,#29097,.T.);
#40076=ORIENTED_EDGE('',*,*,#29095,.T.);
#40077=ORIENTED_EDGE('',*,*,#29093,.T.);
#40078=ORIENTED_EDGE('',*,*,#29091,.T.);
#40079=ORIENTED_EDGE('',*,*,#29089,.T.);
#40080=ORIENTED_EDGE('',*,*,#29087,.T.);
#40081=ORIENTED_EDGE('',*,*,#29085,.T.);
#40082=ORIENTED_EDGE('',*,*,#29083,.T.);
#40083=ORIENTED_EDGE('',*,*,#29081,.T.);
#40084=ORIENTED_EDGE('',*,*,#29079,.T.);
#40085=ORIENTED_EDGE('',*,*,#29077,.T.);
#40086=ORIENTED_EDGE('',*,*,#26902,.T.);
#40087=ORIENTED_EDGE('',*,*,#29102,.F.);
#40088=ORIENTED_EDGE('',*,*,#29103,.T.);
#40089=ORIENTED_EDGE('',*,*,#29104,.T.);
#40090=ORIENTED_EDGE('',*,*,#29105,.T.);
#40091=ORIENTED_EDGE('',*,*,#29106,.T.);
#40092=ORIENTED_EDGE('',*,*,#29107,.T.);
#40093=ORIENTED_EDGE('',*,*,#29108,.T.);
#40094=ORIENTED_EDGE('',*,*,#29109,.T.);
#40095=ORIENTED_EDGE('',*,*,#29110,.T.);
#40096=ORIENTED_EDGE('',*,*,#29111,.T.);
#40097=ORIENTED_EDGE('',*,*,#29112,.T.);
#40098=ORIENTED_EDGE('',*,*,#29113,.T.);
#40099=ORIENTED_EDGE('',*,*,#29114,.T.);
#40100=ORIENTED_EDGE('',*,*,#29115,.T.);
#40101=ORIENTED_EDGE('',*,*,#29116,.T.);
#40102=ORIENTED_EDGE('',*,*,#25679,.T.);
#40103=ORIENTED_EDGE('',*,*,#27489,.T.);
#40104=ORIENTED_EDGE('',*,*,#29116,.F.);
#40105=ORIENTED_EDGE('',*,*,#29117,.F.);
#40106=ORIENTED_EDGE('',*,*,#25646,.T.);
#40107=ORIENTED_EDGE('',*,*,#25680,.T.);
#40108=ORIENTED_EDGE('',*,*,#29115,.F.);
#40109=ORIENTED_EDGE('',*,*,#29118,.F.);
#40110=ORIENTED_EDGE('',*,*,#25647,.T.);
#40111=ORIENTED_EDGE('',*,*,#29117,.T.);
#40112=ORIENTED_EDGE('',*,*,#29114,.F.);
#40113=ORIENTED_EDGE('',*,*,#29119,.F.);
#40114=ORIENTED_EDGE('',*,*,#25648,.T.);
#40115=ORIENTED_EDGE('',*,*,#29118,.T.);
#40116=ORIENTED_EDGE('',*,*,#29113,.F.);
#40117=ORIENTED_EDGE('',*,*,#29120,.F.);
#40118=ORIENTED_EDGE('',*,*,#25649,.T.);
#40119=ORIENTED_EDGE('',*,*,#29119,.T.);
#40120=ORIENTED_EDGE('',*,*,#29112,.F.);
#40121=ORIENTED_EDGE('',*,*,#29121,.F.);
#40122=ORIENTED_EDGE('',*,*,#25650,.T.);
#40123=ORIENTED_EDGE('',*,*,#29120,.T.);
#40124=ORIENTED_EDGE('',*,*,#29111,.F.);
#40125=ORIENTED_EDGE('',*,*,#29122,.F.);
#40126=ORIENTED_EDGE('',*,*,#25651,.T.);
#40127=ORIENTED_EDGE('',*,*,#29121,.T.);
#40128=ORIENTED_EDGE('',*,*,#29110,.F.);
#40129=ORIENTED_EDGE('',*,*,#29123,.F.);
#40130=ORIENTED_EDGE('',*,*,#25652,.T.);
#40131=ORIENTED_EDGE('',*,*,#29122,.T.);
#40132=ORIENTED_EDGE('',*,*,#29109,.F.);
#40133=ORIENTED_EDGE('',*,*,#29124,.F.);
#40134=ORIENTED_EDGE('',*,*,#25653,.T.);
#40135=ORIENTED_EDGE('',*,*,#29123,.T.);
#40136=ORIENTED_EDGE('',*,*,#29108,.F.);
#40137=ORIENTED_EDGE('',*,*,#29125,.F.);
#40138=ORIENTED_EDGE('',*,*,#25654,.T.);
#40139=ORIENTED_EDGE('',*,*,#29124,.T.);
#40140=ORIENTED_EDGE('',*,*,#29107,.F.);
#40141=ORIENTED_EDGE('',*,*,#29126,.F.);
#40142=ORIENTED_EDGE('',*,*,#25655,.T.);
#40143=ORIENTED_EDGE('',*,*,#29125,.T.);
#40144=ORIENTED_EDGE('',*,*,#29106,.F.);
#40145=ORIENTED_EDGE('',*,*,#29127,.F.);
#40146=ORIENTED_EDGE('',*,*,#25656,.T.);
#40147=ORIENTED_EDGE('',*,*,#29126,.T.);
#40148=ORIENTED_EDGE('',*,*,#29105,.F.);
#40149=ORIENTED_EDGE('',*,*,#29128,.F.);
#40150=ORIENTED_EDGE('',*,*,#25657,.T.);
#40151=ORIENTED_EDGE('',*,*,#29127,.T.);
#40152=ORIENTED_EDGE('',*,*,#29104,.F.);
#40153=ORIENTED_EDGE('',*,*,#29129,.F.);
#40154=ORIENTED_EDGE('',*,*,#25658,.T.);
#40155=ORIENTED_EDGE('',*,*,#29128,.T.);
#40156=ORIENTED_EDGE('',*,*,#26853,.T.);
#40157=ORIENTED_EDGE('',*,*,#25659,.T.);
#40158=ORIENTED_EDGE('',*,*,#29129,.T.);
#40159=ORIENTED_EDGE('',*,*,#29103,.F.);
#40160=ORIENTED_EDGE('',*,*,#29130,.F.);
#40161=ORIENTED_EDGE('',*,*,#27396,.T.);
#40162=ORIENTED_EDGE('',*,*,#27273,.T.);
#40163=ORIENTED_EDGE('',*,*,#29131,.F.);
#40164=ORIENTED_EDGE('',*,*,#29132,.F.);
#40165=ORIENTED_EDGE('',*,*,#25662,.T.);
#40166=ORIENTED_EDGE('',*,*,#26898,.T.);
#40167=ORIENTED_EDGE('',*,*,#29133,.F.);
#40168=ORIENTED_EDGE('',*,*,#29134,.F.);
#40169=ORIENTED_EDGE('',*,*,#25663,.T.);
#40170=ORIENTED_EDGE('',*,*,#29132,.T.);
#40171=ORIENTED_EDGE('',*,*,#29135,.F.);
#40172=ORIENTED_EDGE('',*,*,#29136,.F.);
#40173=ORIENTED_EDGE('',*,*,#25664,.T.);
#40174=ORIENTED_EDGE('',*,*,#29134,.T.);
#40175=ORIENTED_EDGE('',*,*,#29137,.F.);
#40176=ORIENTED_EDGE('',*,*,#29138,.F.);
#40177=ORIENTED_EDGE('',*,*,#25665,.T.);
#40178=ORIENTED_EDGE('',*,*,#29136,.T.);
#40179=ORIENTED_EDGE('',*,*,#29139,.F.);
#40180=ORIENTED_EDGE('',*,*,#29140,.F.);
#40181=ORIENTED_EDGE('',*,*,#25666,.T.);
#40182=ORIENTED_EDGE('',*,*,#29138,.T.);
#40183=ORIENTED_EDGE('',*,*,#29141,.F.);
#40184=ORIENTED_EDGE('',*,*,#29142,.F.);
#40185=ORIENTED_EDGE('',*,*,#25667,.T.);
#40186=ORIENTED_EDGE('',*,*,#29140,.T.);
#40187=ORIENTED_EDGE('',*,*,#29143,.F.);
#40188=ORIENTED_EDGE('',*,*,#29144,.F.);
#40189=ORIENTED_EDGE('',*,*,#25668,.T.);
#40190=ORIENTED_EDGE('',*,*,#29142,.T.);
#40191=ORIENTED_EDGE('',*,*,#29145,.F.);
#40192=ORIENTED_EDGE('',*,*,#29146,.F.);
#40193=ORIENTED_EDGE('',*,*,#25669,.T.);
#40194=ORIENTED_EDGE('',*,*,#29144,.T.);
#40195=ORIENTED_EDGE('',*,*,#29147,.F.);
#40196=ORIENTED_EDGE('',*,*,#29148,.F.);
#40197=ORIENTED_EDGE('',*,*,#25670,.T.);
#40198=ORIENTED_EDGE('',*,*,#29146,.T.);
#40199=ORIENTED_EDGE('',*,*,#29149,.F.);
#40200=ORIENTED_EDGE('',*,*,#29150,.F.);
#40201=ORIENTED_EDGE('',*,*,#25671,.T.);
#40202=ORIENTED_EDGE('',*,*,#29148,.T.);
#40203=ORIENTED_EDGE('',*,*,#29151,.F.);
#40204=ORIENTED_EDGE('',*,*,#29152,.F.);
#40205=ORIENTED_EDGE('',*,*,#25672,.T.);
#40206=ORIENTED_EDGE('',*,*,#29150,.T.);
#40207=ORIENTED_EDGE('',*,*,#29153,.F.);
#40208=ORIENTED_EDGE('',*,*,#29154,.F.);
#40209=ORIENTED_EDGE('',*,*,#25673,.T.);
#40210=ORIENTED_EDGE('',*,*,#29152,.T.);
#40211=ORIENTED_EDGE('',*,*,#29155,.F.);
#40212=ORIENTED_EDGE('',*,*,#27241,.F.);
#40213=ORIENTED_EDGE('',*,*,#25674,.T.);
#40214=ORIENTED_EDGE('',*,*,#29154,.T.);
#40215=ORIENTED_EDGE('',*,*,#27060,.T.);
#40216=ORIENTED_EDGE('',*,*,#27244,.F.);
#40217=ORIENTED_EDGE('',*,*,#27490,.F.);
#40218=ORIENTED_EDGE('',*,*,#25677,.F.);
#40219=ORIENTED_EDGE('',*,*,#27242,.T.);
#40220=ORIENTED_EDGE('',*,*,#29155,.T.);
#40221=ORIENTED_EDGE('',*,*,#29153,.T.);
#40222=ORIENTED_EDGE('',*,*,#29151,.T.);
#40223=ORIENTED_EDGE('',*,*,#29149,.T.);
#40224=ORIENTED_EDGE('',*,*,#29147,.T.);
#40225=ORIENTED_EDGE('',*,*,#29145,.T.);
#40226=ORIENTED_EDGE('',*,*,#29143,.T.);
#40227=ORIENTED_EDGE('',*,*,#29141,.T.);
#40228=ORIENTED_EDGE('',*,*,#29139,.T.);
#40229=ORIENTED_EDGE('',*,*,#29137,.T.);
#40230=ORIENTED_EDGE('',*,*,#29135,.T.);
#40231=ORIENTED_EDGE('',*,*,#29133,.T.);
#40232=ORIENTED_EDGE('',*,*,#29131,.T.);
#40233=ORIENTED_EDGE('',*,*,#26897,.T.);
#40234=ORIENTED_EDGE('',*,*,#29156,.F.);
#40235=ORIENTED_EDGE('',*,*,#29157,.T.);
#40236=ORIENTED_EDGE('',*,*,#29158,.T.);
#40237=ORIENTED_EDGE('',*,*,#29159,.T.);
#40238=ORIENTED_EDGE('',*,*,#29160,.T.);
#40239=ORIENTED_EDGE('',*,*,#29161,.T.);
#40240=ORIENTED_EDGE('',*,*,#29162,.T.);
#40241=ORIENTED_EDGE('',*,*,#29163,.T.);
#40242=ORIENTED_EDGE('',*,*,#29164,.T.);
#40243=ORIENTED_EDGE('',*,*,#29165,.T.);
#40244=ORIENTED_EDGE('',*,*,#29166,.T.);
#40245=ORIENTED_EDGE('',*,*,#29167,.T.);
#40246=ORIENTED_EDGE('',*,*,#29168,.T.);
#40247=ORIENTED_EDGE('',*,*,#29169,.T.);
#40248=ORIENTED_EDGE('',*,*,#29170,.T.);
#40249=ORIENTED_EDGE('',*,*,#25643,.T.);
#40250=ORIENTED_EDGE('',*,*,#27491,.T.);
#40251=ORIENTED_EDGE('',*,*,#29170,.F.);
#40252=ORIENTED_EDGE('',*,*,#29171,.F.);
#40253=ORIENTED_EDGE('',*,*,#25610,.T.);
#40254=ORIENTED_EDGE('',*,*,#25644,.T.);
#40255=ORIENTED_EDGE('',*,*,#29169,.F.);
#40256=ORIENTED_EDGE('',*,*,#29172,.F.);
#40257=ORIENTED_EDGE('',*,*,#25611,.T.);
#40258=ORIENTED_EDGE('',*,*,#29171,.T.);
#40259=ORIENTED_EDGE('',*,*,#29168,.F.);
#40260=ORIENTED_EDGE('',*,*,#29173,.F.);
#40261=ORIENTED_EDGE('',*,*,#25612,.T.);
#40262=ORIENTED_EDGE('',*,*,#29172,.T.);
#40263=ORIENTED_EDGE('',*,*,#29167,.F.);
#40264=ORIENTED_EDGE('',*,*,#29174,.F.);
#40265=ORIENTED_EDGE('',*,*,#25613,.T.);
#40266=ORIENTED_EDGE('',*,*,#29173,.T.);
#40267=ORIENTED_EDGE('',*,*,#29166,.F.);
#40268=ORIENTED_EDGE('',*,*,#29175,.F.);
#40269=ORIENTED_EDGE('',*,*,#25614,.T.);
#40270=ORIENTED_EDGE('',*,*,#29174,.T.);
#40271=ORIENTED_EDGE('',*,*,#29165,.F.);
#40272=ORIENTED_EDGE('',*,*,#29176,.F.);
#40273=ORIENTED_EDGE('',*,*,#25615,.T.);
#40274=ORIENTED_EDGE('',*,*,#29175,.T.);
#40275=ORIENTED_EDGE('',*,*,#29164,.F.);
#40276=ORIENTED_EDGE('',*,*,#29177,.F.);
#40277=ORIENTED_EDGE('',*,*,#25616,.T.);
#40278=ORIENTED_EDGE('',*,*,#29176,.T.);
#40279=ORIENTED_EDGE('',*,*,#29163,.F.);
#40280=ORIENTED_EDGE('',*,*,#29178,.F.);
#40281=ORIENTED_EDGE('',*,*,#25617,.T.);
#40282=ORIENTED_EDGE('',*,*,#29177,.T.);
#40283=ORIENTED_EDGE('',*,*,#29162,.F.);
#40284=ORIENTED_EDGE('',*,*,#29179,.F.);
#40285=ORIENTED_EDGE('',*,*,#25618,.T.);
#40286=ORIENTED_EDGE('',*,*,#29178,.T.);
#40287=ORIENTED_EDGE('',*,*,#29161,.F.);
#40288=ORIENTED_EDGE('',*,*,#29180,.F.);
#40289=ORIENTED_EDGE('',*,*,#25619,.T.);
#40290=ORIENTED_EDGE('',*,*,#29179,.T.);
#40291=ORIENTED_EDGE('',*,*,#29160,.F.);
#40292=ORIENTED_EDGE('',*,*,#29181,.F.);
#40293=ORIENTED_EDGE('',*,*,#25620,.T.);
#40294=ORIENTED_EDGE('',*,*,#29180,.T.);
#40295=ORIENTED_EDGE('',*,*,#29159,.F.);
#40296=ORIENTED_EDGE('',*,*,#29182,.F.);
#40297=ORIENTED_EDGE('',*,*,#25621,.T.);
#40298=ORIENTED_EDGE('',*,*,#29181,.T.);
#40299=ORIENTED_EDGE('',*,*,#29158,.F.);
#40300=ORIENTED_EDGE('',*,*,#29183,.F.);
#40301=ORIENTED_EDGE('',*,*,#25622,.T.);
#40302=ORIENTED_EDGE('',*,*,#29182,.T.);
#40303=ORIENTED_EDGE('',*,*,#26856,.T.);
#40304=ORIENTED_EDGE('',*,*,#25623,.T.);
#40305=ORIENTED_EDGE('',*,*,#29183,.T.);
#40306=ORIENTED_EDGE('',*,*,#29157,.F.);
#40307=ORIENTED_EDGE('',*,*,#29184,.F.);
#40308=ORIENTED_EDGE('',*,*,#27398,.T.);
#40309=ORIENTED_EDGE('',*,*,#27271,.T.);
#40310=ORIENTED_EDGE('',*,*,#29185,.F.);
#40311=ORIENTED_EDGE('',*,*,#29186,.F.);
#40312=ORIENTED_EDGE('',*,*,#25626,.T.);
#40313=ORIENTED_EDGE('',*,*,#26893,.T.);
#40314=ORIENTED_EDGE('',*,*,#29187,.F.);
#40315=ORIENTED_EDGE('',*,*,#29188,.F.);
#40316=ORIENTED_EDGE('',*,*,#25627,.T.);
#40317=ORIENTED_EDGE('',*,*,#29186,.T.);
#40318=ORIENTED_EDGE('',*,*,#29189,.F.);
#40319=ORIENTED_EDGE('',*,*,#29190,.F.);
#40320=ORIENTED_EDGE('',*,*,#25628,.T.);
#40321=ORIENTED_EDGE('',*,*,#29188,.T.);
#40322=ORIENTED_EDGE('',*,*,#29191,.F.);
#40323=ORIENTED_EDGE('',*,*,#29192,.F.);
#40324=ORIENTED_EDGE('',*,*,#25629,.T.);
#40325=ORIENTED_EDGE('',*,*,#29190,.T.);
#40326=ORIENTED_EDGE('',*,*,#29193,.F.);
#40327=ORIENTED_EDGE('',*,*,#29194,.F.);
#40328=ORIENTED_EDGE('',*,*,#25630,.T.);
#40329=ORIENTED_EDGE('',*,*,#29192,.T.);
#40330=ORIENTED_EDGE('',*,*,#29195,.F.);
#40331=ORIENTED_EDGE('',*,*,#29196,.F.);
#40332=ORIENTED_EDGE('',*,*,#25631,.T.);
#40333=ORIENTED_EDGE('',*,*,#29194,.T.);
#40334=ORIENTED_EDGE('',*,*,#29197,.F.);
#40335=ORIENTED_EDGE('',*,*,#29198,.F.);
#40336=ORIENTED_EDGE('',*,*,#25632,.T.);
#40337=ORIENTED_EDGE('',*,*,#29196,.T.);
#40338=ORIENTED_EDGE('',*,*,#29199,.F.);
#40339=ORIENTED_EDGE('',*,*,#29200,.F.);
#40340=ORIENTED_EDGE('',*,*,#25633,.T.);
#40341=ORIENTED_EDGE('',*,*,#29198,.T.);
#40342=ORIENTED_EDGE('',*,*,#29201,.F.);
#40343=ORIENTED_EDGE('',*,*,#29202,.F.);
#40344=ORIENTED_EDGE('',*,*,#25634,.T.);
#40345=ORIENTED_EDGE('',*,*,#29200,.T.);
#40346=ORIENTED_EDGE('',*,*,#29203,.F.);
#40347=ORIENTED_EDGE('',*,*,#29204,.F.);
#40348=ORIENTED_EDGE('',*,*,#25635,.T.);
#40349=ORIENTED_EDGE('',*,*,#29202,.T.);
#40350=ORIENTED_EDGE('',*,*,#29205,.F.);
#40351=ORIENTED_EDGE('',*,*,#29206,.F.);
#40352=ORIENTED_EDGE('',*,*,#25636,.T.);
#40353=ORIENTED_EDGE('',*,*,#29204,.T.);
#40354=ORIENTED_EDGE('',*,*,#29207,.F.);
#40355=ORIENTED_EDGE('',*,*,#29208,.F.);
#40356=ORIENTED_EDGE('',*,*,#25637,.T.);
#40357=ORIENTED_EDGE('',*,*,#29206,.T.);
#40358=ORIENTED_EDGE('',*,*,#29209,.F.);
#40359=ORIENTED_EDGE('',*,*,#27245,.F.);
#40360=ORIENTED_EDGE('',*,*,#25638,.T.);
#40361=ORIENTED_EDGE('',*,*,#29208,.T.);
#40362=ORIENTED_EDGE('',*,*,#27058,.T.);
#40363=ORIENTED_EDGE('',*,*,#27248,.F.);
#40364=ORIENTED_EDGE('',*,*,#27492,.F.);
#40365=ORIENTED_EDGE('',*,*,#25641,.F.);
#40366=ORIENTED_EDGE('',*,*,#27246,.T.);
#40367=ORIENTED_EDGE('',*,*,#29209,.T.);
#40368=ORIENTED_EDGE('',*,*,#29207,.T.);
#40369=ORIENTED_EDGE('',*,*,#29205,.T.);
#40370=ORIENTED_EDGE('',*,*,#29203,.T.);
#40371=ORIENTED_EDGE('',*,*,#29201,.T.);
#40372=ORIENTED_EDGE('',*,*,#29199,.T.);
#40373=ORIENTED_EDGE('',*,*,#29197,.T.);
#40374=ORIENTED_EDGE('',*,*,#29195,.T.);
#40375=ORIENTED_EDGE('',*,*,#29193,.T.);
#40376=ORIENTED_EDGE('',*,*,#29191,.T.);
#40377=ORIENTED_EDGE('',*,*,#29189,.T.);
#40378=ORIENTED_EDGE('',*,*,#29187,.T.);
#40379=ORIENTED_EDGE('',*,*,#29185,.T.);
#40380=ORIENTED_EDGE('',*,*,#26892,.T.);
#40381=ORIENTED_EDGE('',*,*,#29210,.F.);
#40382=ORIENTED_EDGE('',*,*,#29211,.T.);
#40383=ORIENTED_EDGE('',*,*,#29212,.T.);
#40384=ORIENTED_EDGE('',*,*,#29213,.T.);
#40385=ORIENTED_EDGE('',*,*,#29214,.T.);
#40386=ORIENTED_EDGE('',*,*,#29215,.T.);
#40387=ORIENTED_EDGE('',*,*,#29216,.T.);
#40388=ORIENTED_EDGE('',*,*,#29217,.T.);
#40389=ORIENTED_EDGE('',*,*,#29218,.T.);
#40390=ORIENTED_EDGE('',*,*,#29219,.T.);
#40391=ORIENTED_EDGE('',*,*,#29220,.T.);
#40392=ORIENTED_EDGE('',*,*,#29221,.T.);
#40393=ORIENTED_EDGE('',*,*,#29222,.T.);
#40394=ORIENTED_EDGE('',*,*,#29223,.T.);
#40395=ORIENTED_EDGE('',*,*,#29224,.T.);
#40396=ORIENTED_EDGE('',*,*,#25607,.T.);
#40397=ORIENTED_EDGE('',*,*,#27493,.T.);
#40398=ORIENTED_EDGE('',*,*,#29224,.F.);
#40399=ORIENTED_EDGE('',*,*,#29225,.F.);
#40400=ORIENTED_EDGE('',*,*,#25574,.T.);
#40401=ORIENTED_EDGE('',*,*,#25608,.T.);
#40402=ORIENTED_EDGE('',*,*,#29223,.F.);
#40403=ORIENTED_EDGE('',*,*,#29226,.F.);
#40404=ORIENTED_EDGE('',*,*,#25575,.T.);
#40405=ORIENTED_EDGE('',*,*,#29225,.T.);
#40406=ORIENTED_EDGE('',*,*,#29222,.F.);
#40407=ORIENTED_EDGE('',*,*,#29227,.F.);
#40408=ORIENTED_EDGE('',*,*,#25576,.T.);
#40409=ORIENTED_EDGE('',*,*,#29226,.T.);
#40410=ORIENTED_EDGE('',*,*,#29221,.F.);
#40411=ORIENTED_EDGE('',*,*,#29228,.F.);
#40412=ORIENTED_EDGE('',*,*,#25577,.T.);
#40413=ORIENTED_EDGE('',*,*,#29227,.T.);
#40414=ORIENTED_EDGE('',*,*,#29220,.F.);
#40415=ORIENTED_EDGE('',*,*,#29229,.F.);
#40416=ORIENTED_EDGE('',*,*,#25578,.T.);
#40417=ORIENTED_EDGE('',*,*,#29228,.T.);
#40418=ORIENTED_EDGE('',*,*,#29219,.F.);
#40419=ORIENTED_EDGE('',*,*,#29230,.F.);
#40420=ORIENTED_EDGE('',*,*,#25579,.T.);
#40421=ORIENTED_EDGE('',*,*,#29229,.T.);
#40422=ORIENTED_EDGE('',*,*,#29218,.F.);
#40423=ORIENTED_EDGE('',*,*,#29231,.F.);
#40424=ORIENTED_EDGE('',*,*,#25580,.T.);
#40425=ORIENTED_EDGE('',*,*,#29230,.T.);
#40426=ORIENTED_EDGE('',*,*,#29217,.F.);
#40427=ORIENTED_EDGE('',*,*,#29232,.F.);
#40428=ORIENTED_EDGE('',*,*,#25581,.T.);
#40429=ORIENTED_EDGE('',*,*,#29231,.T.);
#40430=ORIENTED_EDGE('',*,*,#29216,.F.);
#40431=ORIENTED_EDGE('',*,*,#29233,.F.);
#40432=ORIENTED_EDGE('',*,*,#25582,.T.);
#40433=ORIENTED_EDGE('',*,*,#29232,.T.);
#40434=ORIENTED_EDGE('',*,*,#29215,.F.);
#40435=ORIENTED_EDGE('',*,*,#29234,.F.);
#40436=ORIENTED_EDGE('',*,*,#25583,.T.);
#40437=ORIENTED_EDGE('',*,*,#29233,.T.);
#40438=ORIENTED_EDGE('',*,*,#29214,.F.);
#40439=ORIENTED_EDGE('',*,*,#29235,.F.);
#40440=ORIENTED_EDGE('',*,*,#25584,.T.);
#40441=ORIENTED_EDGE('',*,*,#29234,.T.);
#40442=ORIENTED_EDGE('',*,*,#29213,.F.);
#40443=ORIENTED_EDGE('',*,*,#29236,.F.);
#40444=ORIENTED_EDGE('',*,*,#25585,.T.);
#40445=ORIENTED_EDGE('',*,*,#29235,.T.);
#40446=ORIENTED_EDGE('',*,*,#29212,.F.);
#40447=ORIENTED_EDGE('',*,*,#29237,.F.);
#40448=ORIENTED_EDGE('',*,*,#25586,.T.);
#40449=ORIENTED_EDGE('',*,*,#29236,.T.);
#40450=ORIENTED_EDGE('',*,*,#26859,.T.);
#40451=ORIENTED_EDGE('',*,*,#25587,.T.);
#40452=ORIENTED_EDGE('',*,*,#29237,.T.);
#40453=ORIENTED_EDGE('',*,*,#29211,.F.);
#40454=ORIENTED_EDGE('',*,*,#29238,.F.);
#40455=ORIENTED_EDGE('',*,*,#27400,.T.);
#40456=ORIENTED_EDGE('',*,*,#27269,.T.);
#40457=ORIENTED_EDGE('',*,*,#29239,.F.);
#40458=ORIENTED_EDGE('',*,*,#29240,.F.);
#40459=ORIENTED_EDGE('',*,*,#25590,.T.);
#40460=ORIENTED_EDGE('',*,*,#26888,.T.);
#40461=ORIENTED_EDGE('',*,*,#29241,.F.);
#40462=ORIENTED_EDGE('',*,*,#29242,.F.);
#40463=ORIENTED_EDGE('',*,*,#25591,.T.);
#40464=ORIENTED_EDGE('',*,*,#29240,.T.);
#40465=ORIENTED_EDGE('',*,*,#29243,.F.);
#40466=ORIENTED_EDGE('',*,*,#29244,.F.);
#40467=ORIENTED_EDGE('',*,*,#25592,.T.);
#40468=ORIENTED_EDGE('',*,*,#29242,.T.);
#40469=ORIENTED_EDGE('',*,*,#29245,.F.);
#40470=ORIENTED_EDGE('',*,*,#29246,.F.);
#40471=ORIENTED_EDGE('',*,*,#25593,.T.);
#40472=ORIENTED_EDGE('',*,*,#29244,.T.);
#40473=ORIENTED_EDGE('',*,*,#29247,.F.);
#40474=ORIENTED_EDGE('',*,*,#29248,.F.);
#40475=ORIENTED_EDGE('',*,*,#25594,.T.);
#40476=ORIENTED_EDGE('',*,*,#29246,.T.);
#40477=ORIENTED_EDGE('',*,*,#29249,.F.);
#40478=ORIENTED_EDGE('',*,*,#29250,.F.);
#40479=ORIENTED_EDGE('',*,*,#25595,.T.);
#40480=ORIENTED_EDGE('',*,*,#29248,.T.);
#40481=ORIENTED_EDGE('',*,*,#29251,.F.);
#40482=ORIENTED_EDGE('',*,*,#29252,.F.);
#40483=ORIENTED_EDGE('',*,*,#25596,.T.);
#40484=ORIENTED_EDGE('',*,*,#29250,.T.);
#40485=ORIENTED_EDGE('',*,*,#29253,.F.);
#40486=ORIENTED_EDGE('',*,*,#29254,.F.);
#40487=ORIENTED_EDGE('',*,*,#25597,.T.);
#40488=ORIENTED_EDGE('',*,*,#29252,.T.);
#40489=ORIENTED_EDGE('',*,*,#29255,.F.);
#40490=ORIENTED_EDGE('',*,*,#29256,.F.);
#40491=ORIENTED_EDGE('',*,*,#25598,.T.);
#40492=ORIENTED_EDGE('',*,*,#29254,.T.);
#40493=ORIENTED_EDGE('',*,*,#29257,.F.);
#40494=ORIENTED_EDGE('',*,*,#29258,.F.);
#40495=ORIENTED_EDGE('',*,*,#25599,.T.);
#40496=ORIENTED_EDGE('',*,*,#29256,.T.);
#40497=ORIENTED_EDGE('',*,*,#29259,.F.);
#40498=ORIENTED_EDGE('',*,*,#29260,.F.);
#40499=ORIENTED_EDGE('',*,*,#25600,.T.);
#40500=ORIENTED_EDGE('',*,*,#29258,.T.);
#40501=ORIENTED_EDGE('',*,*,#29261,.F.);
#40502=ORIENTED_EDGE('',*,*,#29262,.F.);
#40503=ORIENTED_EDGE('',*,*,#25601,.T.);
#40504=ORIENTED_EDGE('',*,*,#29260,.T.);
#40505=ORIENTED_EDGE('',*,*,#29263,.F.);
#40506=ORIENTED_EDGE('',*,*,#27249,.F.);
#40507=ORIENTED_EDGE('',*,*,#25602,.T.);
#40508=ORIENTED_EDGE('',*,*,#29262,.T.);
#40509=ORIENTED_EDGE('',*,*,#27056,.T.);
#40510=ORIENTED_EDGE('',*,*,#27252,.F.);
#40511=ORIENTED_EDGE('',*,*,#27494,.F.);
#40512=ORIENTED_EDGE('',*,*,#25605,.F.);
#40513=ORIENTED_EDGE('',*,*,#27250,.T.);
#40514=ORIENTED_EDGE('',*,*,#29263,.T.);
#40515=ORIENTED_EDGE('',*,*,#29261,.T.);
#40516=ORIENTED_EDGE('',*,*,#29259,.T.);
#40517=ORIENTED_EDGE('',*,*,#29257,.T.);
#40518=ORIENTED_EDGE('',*,*,#29255,.T.);
#40519=ORIENTED_EDGE('',*,*,#29253,.T.);
#40520=ORIENTED_EDGE('',*,*,#29251,.T.);
#40521=ORIENTED_EDGE('',*,*,#29249,.T.);
#40522=ORIENTED_EDGE('',*,*,#29247,.T.);
#40523=ORIENTED_EDGE('',*,*,#29245,.T.);
#40524=ORIENTED_EDGE('',*,*,#29243,.T.);
#40525=ORIENTED_EDGE('',*,*,#29241,.T.);
#40526=ORIENTED_EDGE('',*,*,#29239,.T.);
#40527=ORIENTED_EDGE('',*,*,#26887,.T.);
#40528=ORIENTED_EDGE('',*,*,#29264,.F.);
#40529=ORIENTED_EDGE('',*,*,#29265,.T.);
#40530=ORIENTED_EDGE('',*,*,#29266,.T.);
#40531=ORIENTED_EDGE('',*,*,#29267,.T.);
#40532=ORIENTED_EDGE('',*,*,#29268,.T.);
#40533=ORIENTED_EDGE('',*,*,#29269,.T.);
#40534=ORIENTED_EDGE('',*,*,#29270,.T.);
#40535=ORIENTED_EDGE('',*,*,#29271,.T.);
#40536=ORIENTED_EDGE('',*,*,#29272,.T.);
#40537=ORIENTED_EDGE('',*,*,#29273,.T.);
#40538=ORIENTED_EDGE('',*,*,#29274,.T.);
#40539=ORIENTED_EDGE('',*,*,#29275,.T.);
#40540=ORIENTED_EDGE('',*,*,#29276,.T.);
#40541=ORIENTED_EDGE('',*,*,#29277,.T.);
#40542=ORIENTED_EDGE('',*,*,#29278,.T.);
#40543=ORIENTED_EDGE('',*,*,#25571,.T.);
#40544=ORIENTED_EDGE('',*,*,#27495,.T.);
#40545=ORIENTED_EDGE('',*,*,#29278,.F.);
#40546=ORIENTED_EDGE('',*,*,#29279,.F.);
#40547=ORIENTED_EDGE('',*,*,#25538,.T.);
#40548=ORIENTED_EDGE('',*,*,#25572,.T.);
#40549=ORIENTED_EDGE('',*,*,#29277,.F.);
#40550=ORIENTED_EDGE('',*,*,#29280,.F.);
#40551=ORIENTED_EDGE('',*,*,#25539,.T.);
#40552=ORIENTED_EDGE('',*,*,#29279,.T.);
#40553=ORIENTED_EDGE('',*,*,#29276,.F.);
#40554=ORIENTED_EDGE('',*,*,#29281,.F.);
#40555=ORIENTED_EDGE('',*,*,#25540,.T.);
#40556=ORIENTED_EDGE('',*,*,#29280,.T.);
#40557=ORIENTED_EDGE('',*,*,#29275,.F.);
#40558=ORIENTED_EDGE('',*,*,#29282,.F.);
#40559=ORIENTED_EDGE('',*,*,#25541,.T.);
#40560=ORIENTED_EDGE('',*,*,#29281,.T.);
#40561=ORIENTED_EDGE('',*,*,#29274,.F.);
#40562=ORIENTED_EDGE('',*,*,#29283,.F.);
#40563=ORIENTED_EDGE('',*,*,#25542,.T.);
#40564=ORIENTED_EDGE('',*,*,#29282,.T.);
#40565=ORIENTED_EDGE('',*,*,#29273,.F.);
#40566=ORIENTED_EDGE('',*,*,#29284,.F.);
#40567=ORIENTED_EDGE('',*,*,#25543,.T.);
#40568=ORIENTED_EDGE('',*,*,#29283,.T.);
#40569=ORIENTED_EDGE('',*,*,#29272,.F.);
#40570=ORIENTED_EDGE('',*,*,#29285,.F.);
#40571=ORIENTED_EDGE('',*,*,#25544,.T.);
#40572=ORIENTED_EDGE('',*,*,#29284,.T.);
#40573=ORIENTED_EDGE('',*,*,#29271,.F.);
#40574=ORIENTED_EDGE('',*,*,#29286,.F.);
#40575=ORIENTED_EDGE('',*,*,#25545,.T.);
#40576=ORIENTED_EDGE('',*,*,#29285,.T.);
#40577=ORIENTED_EDGE('',*,*,#29270,.F.);
#40578=ORIENTED_EDGE('',*,*,#29287,.F.);
#40579=ORIENTED_EDGE('',*,*,#25546,.T.);
#40580=ORIENTED_EDGE('',*,*,#29286,.T.);
#40581=ORIENTED_EDGE('',*,*,#29269,.F.);
#40582=ORIENTED_EDGE('',*,*,#29288,.F.);
#40583=ORIENTED_EDGE('',*,*,#25547,.T.);
#40584=ORIENTED_EDGE('',*,*,#29287,.T.);
#40585=ORIENTED_EDGE('',*,*,#29268,.F.);
#40586=ORIENTED_EDGE('',*,*,#29289,.F.);
#40587=ORIENTED_EDGE('',*,*,#25548,.T.);
#40588=ORIENTED_EDGE('',*,*,#29288,.T.);
#40589=ORIENTED_EDGE('',*,*,#29267,.F.);
#40590=ORIENTED_EDGE('',*,*,#29290,.F.);
#40591=ORIENTED_EDGE('',*,*,#25549,.T.);
#40592=ORIENTED_EDGE('',*,*,#29289,.T.);
#40593=ORIENTED_EDGE('',*,*,#29266,.F.);
#40594=ORIENTED_EDGE('',*,*,#29291,.F.);
#40595=ORIENTED_EDGE('',*,*,#25550,.T.);
#40596=ORIENTED_EDGE('',*,*,#29290,.T.);
#40597=ORIENTED_EDGE('',*,*,#26862,.T.);
#40598=ORIENTED_EDGE('',*,*,#25551,.T.);
#40599=ORIENTED_EDGE('',*,*,#29291,.T.);
#40600=ORIENTED_EDGE('',*,*,#29265,.F.);
#40601=ORIENTED_EDGE('',*,*,#29292,.F.);
#40602=ORIENTED_EDGE('',*,*,#27402,.T.);
#40603=ORIENTED_EDGE('',*,*,#27267,.T.);
#40604=ORIENTED_EDGE('',*,*,#29293,.F.);
#40605=ORIENTED_EDGE('',*,*,#29294,.F.);
#40606=ORIENTED_EDGE('',*,*,#25554,.T.);
#40607=ORIENTED_EDGE('',*,*,#26883,.T.);
#40608=ORIENTED_EDGE('',*,*,#29295,.F.);
#40609=ORIENTED_EDGE('',*,*,#29296,.F.);
#40610=ORIENTED_EDGE('',*,*,#25555,.T.);
#40611=ORIENTED_EDGE('',*,*,#29294,.T.);
#40612=ORIENTED_EDGE('',*,*,#29297,.F.);
#40613=ORIENTED_EDGE('',*,*,#29298,.F.);
#40614=ORIENTED_EDGE('',*,*,#25556,.T.);
#40615=ORIENTED_EDGE('',*,*,#29296,.T.);
#40616=ORIENTED_EDGE('',*,*,#29299,.F.);
#40617=ORIENTED_EDGE('',*,*,#29300,.F.);
#40618=ORIENTED_EDGE('',*,*,#25557,.T.);
#40619=ORIENTED_EDGE('',*,*,#29298,.T.);
#40620=ORIENTED_EDGE('',*,*,#29301,.F.);
#40621=ORIENTED_EDGE('',*,*,#29302,.F.);
#40622=ORIENTED_EDGE('',*,*,#25558,.T.);
#40623=ORIENTED_EDGE('',*,*,#29300,.T.);
#40624=ORIENTED_EDGE('',*,*,#29303,.F.);
#40625=ORIENTED_EDGE('',*,*,#29304,.F.);
#40626=ORIENTED_EDGE('',*,*,#25559,.T.);
#40627=ORIENTED_EDGE('',*,*,#29302,.T.);
#40628=ORIENTED_EDGE('',*,*,#29305,.F.);
#40629=ORIENTED_EDGE('',*,*,#29306,.F.);
#40630=ORIENTED_EDGE('',*,*,#25560,.T.);
#40631=ORIENTED_EDGE('',*,*,#29304,.T.);
#40632=ORIENTED_EDGE('',*,*,#29307,.F.);
#40633=ORIENTED_EDGE('',*,*,#29308,.F.);
#40634=ORIENTED_EDGE('',*,*,#25561,.T.);
#40635=ORIENTED_EDGE('',*,*,#29306,.T.);
#40636=ORIENTED_EDGE('',*,*,#29309,.F.);
#40637=ORIENTED_EDGE('',*,*,#29310,.F.);
#40638=ORIENTED_EDGE('',*,*,#25562,.T.);
#40639=ORIENTED_EDGE('',*,*,#29308,.T.);
#40640=ORIENTED_EDGE('',*,*,#29311,.F.);
#40641=ORIENTED_EDGE('',*,*,#29312,.F.);
#40642=ORIENTED_EDGE('',*,*,#25563,.T.);
#40643=ORIENTED_EDGE('',*,*,#29310,.T.);
#40644=ORIENTED_EDGE('',*,*,#29313,.F.);
#40645=ORIENTED_EDGE('',*,*,#29314,.F.);
#40646=ORIENTED_EDGE('',*,*,#25564,.T.);
#40647=ORIENTED_EDGE('',*,*,#29312,.T.);
#40648=ORIENTED_EDGE('',*,*,#29315,.F.);
#40649=ORIENTED_EDGE('',*,*,#29316,.F.);
#40650=ORIENTED_EDGE('',*,*,#25565,.T.);
#40651=ORIENTED_EDGE('',*,*,#29314,.T.);
#40652=ORIENTED_EDGE('',*,*,#29317,.F.);
#40653=ORIENTED_EDGE('',*,*,#27253,.F.);
#40654=ORIENTED_EDGE('',*,*,#25566,.T.);
#40655=ORIENTED_EDGE('',*,*,#29316,.T.);
#40656=ORIENTED_EDGE('',*,*,#27054,.T.);
#40657=ORIENTED_EDGE('',*,*,#27256,.F.);
#40658=ORIENTED_EDGE('',*,*,#27496,.F.);
#40659=ORIENTED_EDGE('',*,*,#25569,.F.);
#40660=ORIENTED_EDGE('',*,*,#27254,.T.);
#40661=ORIENTED_EDGE('',*,*,#29317,.T.);
#40662=ORIENTED_EDGE('',*,*,#29315,.T.);
#40663=ORIENTED_EDGE('',*,*,#29313,.T.);
#40664=ORIENTED_EDGE('',*,*,#29311,.T.);
#40665=ORIENTED_EDGE('',*,*,#29309,.T.);
#40666=ORIENTED_EDGE('',*,*,#29307,.T.);
#40667=ORIENTED_EDGE('',*,*,#29305,.T.);
#40668=ORIENTED_EDGE('',*,*,#29303,.T.);
#40669=ORIENTED_EDGE('',*,*,#29301,.T.);
#40670=ORIENTED_EDGE('',*,*,#29299,.T.);
#40671=ORIENTED_EDGE('',*,*,#29297,.T.);
#40672=ORIENTED_EDGE('',*,*,#29295,.T.);
#40673=ORIENTED_EDGE('',*,*,#29293,.T.);
#40674=ORIENTED_EDGE('',*,*,#26882,.T.);
#40675=ORIENTED_EDGE('',*,*,#29318,.F.);
#40676=ORIENTED_EDGE('',*,*,#29319,.T.);
#40677=ORIENTED_EDGE('',*,*,#29320,.T.);
#40678=ORIENTED_EDGE('',*,*,#29321,.T.);
#40679=ORIENTED_EDGE('',*,*,#29322,.T.);
#40680=ORIENTED_EDGE('',*,*,#29323,.T.);
#40681=ORIENTED_EDGE('',*,*,#29324,.T.);
#40682=ORIENTED_EDGE('',*,*,#29325,.T.);
#40683=ORIENTED_EDGE('',*,*,#29326,.T.);
#40684=ORIENTED_EDGE('',*,*,#29327,.T.);
#40685=ORIENTED_EDGE('',*,*,#29328,.T.);
#40686=ORIENTED_EDGE('',*,*,#29329,.T.);
#40687=ORIENTED_EDGE('',*,*,#29330,.T.);
#40688=ORIENTED_EDGE('',*,*,#29331,.T.);
#40689=ORIENTED_EDGE('',*,*,#29332,.T.);
#40690=ORIENTED_EDGE('',*,*,#25535,.T.);
#40691=ORIENTED_EDGE('',*,*,#27497,.T.);
#40692=ORIENTED_EDGE('',*,*,#29332,.F.);
#40693=ORIENTED_EDGE('',*,*,#29333,.F.);
#40694=ORIENTED_EDGE('',*,*,#25502,.T.);
#40695=ORIENTED_EDGE('',*,*,#25536,.T.);
#40696=ORIENTED_EDGE('',*,*,#29331,.F.);
#40697=ORIENTED_EDGE('',*,*,#29334,.F.);
#40698=ORIENTED_EDGE('',*,*,#25503,.T.);
#40699=ORIENTED_EDGE('',*,*,#29333,.T.);
#40700=ORIENTED_EDGE('',*,*,#29330,.F.);
#40701=ORIENTED_EDGE('',*,*,#29335,.F.);
#40702=ORIENTED_EDGE('',*,*,#25504,.T.);
#40703=ORIENTED_EDGE('',*,*,#29334,.T.);
#40704=ORIENTED_EDGE('',*,*,#29329,.F.);
#40705=ORIENTED_EDGE('',*,*,#29336,.F.);
#40706=ORIENTED_EDGE('',*,*,#25505,.T.);
#40707=ORIENTED_EDGE('',*,*,#29335,.T.);
#40708=ORIENTED_EDGE('',*,*,#29328,.F.);
#40709=ORIENTED_EDGE('',*,*,#29337,.F.);
#40710=ORIENTED_EDGE('',*,*,#25506,.T.);
#40711=ORIENTED_EDGE('',*,*,#29336,.T.);
#40712=ORIENTED_EDGE('',*,*,#29327,.F.);
#40713=ORIENTED_EDGE('',*,*,#29338,.F.);
#40714=ORIENTED_EDGE('',*,*,#25507,.T.);
#40715=ORIENTED_EDGE('',*,*,#29337,.T.);
#40716=ORIENTED_EDGE('',*,*,#29326,.F.);
#40717=ORIENTED_EDGE('',*,*,#29339,.F.);
#40718=ORIENTED_EDGE('',*,*,#25508,.T.);
#40719=ORIENTED_EDGE('',*,*,#29338,.T.);
#40720=ORIENTED_EDGE('',*,*,#29325,.F.);
#40721=ORIENTED_EDGE('',*,*,#29340,.F.);
#40722=ORIENTED_EDGE('',*,*,#25509,.T.);
#40723=ORIENTED_EDGE('',*,*,#29339,.T.);
#40724=ORIENTED_EDGE('',*,*,#29324,.F.);
#40725=ORIENTED_EDGE('',*,*,#29341,.F.);
#40726=ORIENTED_EDGE('',*,*,#25510,.T.);
#40727=ORIENTED_EDGE('',*,*,#29340,.T.);
#40728=ORIENTED_EDGE('',*,*,#29323,.F.);
#40729=ORIENTED_EDGE('',*,*,#29342,.F.);
#40730=ORIENTED_EDGE('',*,*,#25511,.T.);
#40731=ORIENTED_EDGE('',*,*,#29341,.T.);
#40732=ORIENTED_EDGE('',*,*,#29322,.F.);
#40733=ORIENTED_EDGE('',*,*,#29343,.F.);
#40734=ORIENTED_EDGE('',*,*,#25512,.T.);
#40735=ORIENTED_EDGE('',*,*,#29342,.T.);
#40736=ORIENTED_EDGE('',*,*,#29321,.F.);
#40737=ORIENTED_EDGE('',*,*,#29344,.F.);
#40738=ORIENTED_EDGE('',*,*,#25513,.T.);
#40739=ORIENTED_EDGE('',*,*,#29343,.T.);
#40740=ORIENTED_EDGE('',*,*,#29320,.F.);
#40741=ORIENTED_EDGE('',*,*,#29345,.F.);
#40742=ORIENTED_EDGE('',*,*,#25514,.T.);
#40743=ORIENTED_EDGE('',*,*,#29344,.T.);
#40744=ORIENTED_EDGE('',*,*,#26865,.T.);
#40745=ORIENTED_EDGE('',*,*,#25515,.T.);
#40746=ORIENTED_EDGE('',*,*,#29345,.T.);
#40747=ORIENTED_EDGE('',*,*,#29319,.F.);
#40748=ORIENTED_EDGE('',*,*,#29346,.F.);
#40749=ORIENTED_EDGE('',*,*,#27404,.T.);
#40750=ORIENTED_EDGE('',*,*,#27265,.T.);
#40751=ORIENTED_EDGE('',*,*,#29347,.F.);
#40752=ORIENTED_EDGE('',*,*,#29348,.F.);
#40753=ORIENTED_EDGE('',*,*,#25518,.T.);
#40754=ORIENTED_EDGE('',*,*,#26878,.T.);
#40755=ORIENTED_EDGE('',*,*,#29349,.F.);
#40756=ORIENTED_EDGE('',*,*,#29350,.F.);
#40757=ORIENTED_EDGE('',*,*,#25519,.T.);
#40758=ORIENTED_EDGE('',*,*,#29348,.T.);
#40759=ORIENTED_EDGE('',*,*,#29351,.F.);
#40760=ORIENTED_EDGE('',*,*,#29352,.F.);
#40761=ORIENTED_EDGE('',*,*,#25520,.T.);
#40762=ORIENTED_EDGE('',*,*,#29350,.T.);
#40763=ORIENTED_EDGE('',*,*,#29353,.F.);
#40764=ORIENTED_EDGE('',*,*,#29354,.F.);
#40765=ORIENTED_EDGE('',*,*,#25521,.T.);
#40766=ORIENTED_EDGE('',*,*,#29352,.T.);
#40767=ORIENTED_EDGE('',*,*,#29355,.F.);
#40768=ORIENTED_EDGE('',*,*,#29356,.F.);
#40769=ORIENTED_EDGE('',*,*,#25522,.T.);
#40770=ORIENTED_EDGE('',*,*,#29354,.T.);
#40771=ORIENTED_EDGE('',*,*,#29357,.F.);
#40772=ORIENTED_EDGE('',*,*,#29358,.F.);
#40773=ORIENTED_EDGE('',*,*,#25523,.T.);
#40774=ORIENTED_EDGE('',*,*,#29356,.T.);
#40775=ORIENTED_EDGE('',*,*,#29359,.F.);
#40776=ORIENTED_EDGE('',*,*,#29360,.F.);
#40777=ORIENTED_EDGE('',*,*,#25524,.T.);
#40778=ORIENTED_EDGE('',*,*,#29358,.T.);
#40779=ORIENTED_EDGE('',*,*,#29361,.F.);
#40780=ORIENTED_EDGE('',*,*,#29362,.F.);
#40781=ORIENTED_EDGE('',*,*,#25525,.T.);
#40782=ORIENTED_EDGE('',*,*,#29360,.T.);
#40783=ORIENTED_EDGE('',*,*,#29363,.F.);
#40784=ORIENTED_EDGE('',*,*,#29364,.F.);
#40785=ORIENTED_EDGE('',*,*,#25526,.T.);
#40786=ORIENTED_EDGE('',*,*,#29362,.T.);
#40787=ORIENTED_EDGE('',*,*,#29365,.F.);
#40788=ORIENTED_EDGE('',*,*,#29366,.F.);
#40789=ORIENTED_EDGE('',*,*,#25527,.T.);
#40790=ORIENTED_EDGE('',*,*,#29364,.T.);
#40791=ORIENTED_EDGE('',*,*,#29367,.F.);
#40792=ORIENTED_EDGE('',*,*,#29368,.F.);
#40793=ORIENTED_EDGE('',*,*,#25528,.T.);
#40794=ORIENTED_EDGE('',*,*,#29366,.T.);
#40795=ORIENTED_EDGE('',*,*,#29369,.F.);
#40796=ORIENTED_EDGE('',*,*,#29370,.F.);
#40797=ORIENTED_EDGE('',*,*,#25529,.T.);
#40798=ORIENTED_EDGE('',*,*,#29368,.T.);
#40799=ORIENTED_EDGE('',*,*,#29371,.F.);
#40800=ORIENTED_EDGE('',*,*,#27257,.F.);
#40801=ORIENTED_EDGE('',*,*,#25530,.T.);
#40802=ORIENTED_EDGE('',*,*,#29370,.T.);
#40803=ORIENTED_EDGE('',*,*,#27052,.T.);
#40804=ORIENTED_EDGE('',*,*,#27260,.F.);
#40805=ORIENTED_EDGE('',*,*,#27498,.F.);
#40806=ORIENTED_EDGE('',*,*,#25533,.F.);
#40807=ORIENTED_EDGE('',*,*,#27258,.T.);
#40808=ORIENTED_EDGE('',*,*,#29371,.T.);
#40809=ORIENTED_EDGE('',*,*,#29369,.T.);
#40810=ORIENTED_EDGE('',*,*,#29367,.T.);
#40811=ORIENTED_EDGE('',*,*,#29365,.T.);
#40812=ORIENTED_EDGE('',*,*,#29363,.T.);
#40813=ORIENTED_EDGE('',*,*,#29361,.T.);
#40814=ORIENTED_EDGE('',*,*,#29359,.T.);
#40815=ORIENTED_EDGE('',*,*,#29357,.T.);
#40816=ORIENTED_EDGE('',*,*,#29355,.T.);
#40817=ORIENTED_EDGE('',*,*,#29353,.T.);
#40818=ORIENTED_EDGE('',*,*,#29351,.T.);
#40819=ORIENTED_EDGE('',*,*,#29349,.T.);
#40820=ORIENTED_EDGE('',*,*,#29347,.T.);
#40821=ORIENTED_EDGE('',*,*,#26877,.T.);
#40822=ORIENTED_EDGE('',*,*,#29372,.F.);
#40823=ORIENTED_EDGE('',*,*,#29373,.T.);
#40824=ORIENTED_EDGE('',*,*,#29374,.T.);
#40825=ORIENTED_EDGE('',*,*,#29375,.T.);
#40826=ORIENTED_EDGE('',*,*,#29376,.T.);
#40827=ORIENTED_EDGE('',*,*,#29377,.T.);
#40828=ORIENTED_EDGE('',*,*,#29378,.T.);
#40829=ORIENTED_EDGE('',*,*,#29379,.T.);
#40830=ORIENTED_EDGE('',*,*,#29380,.T.);
#40831=ORIENTED_EDGE('',*,*,#29381,.T.);
#40832=ORIENTED_EDGE('',*,*,#29382,.T.);
#40833=ORIENTED_EDGE('',*,*,#29383,.T.);
#40834=ORIENTED_EDGE('',*,*,#29384,.T.);
#40835=ORIENTED_EDGE('',*,*,#29385,.T.);
#40836=ORIENTED_EDGE('',*,*,#29386,.T.);
#40837=ORIENTED_EDGE('',*,*,#25499,.T.);
#40838=ORIENTED_EDGE('',*,*,#27499,.T.);
#40839=ORIENTED_EDGE('',*,*,#29387,.F.);
#40840=ORIENTED_EDGE('',*,*,#29388,.F.);
#40841=ORIENTED_EDGE('',*,*,#25482,.T.);
#40842=ORIENTED_EDGE('',*,*,#26873,.T.);
#40843=ORIENTED_EDGE('',*,*,#29389,.F.);
#40844=ORIENTED_EDGE('',*,*,#29390,.F.);
#40845=ORIENTED_EDGE('',*,*,#25483,.T.);
#40846=ORIENTED_EDGE('',*,*,#29388,.T.);
#40847=ORIENTED_EDGE('',*,*,#29391,.F.);
#40848=ORIENTED_EDGE('',*,*,#29392,.F.);
#40849=ORIENTED_EDGE('',*,*,#25484,.T.);
#40850=ORIENTED_EDGE('',*,*,#29390,.T.);
#40851=ORIENTED_EDGE('',*,*,#29393,.F.);
#40852=ORIENTED_EDGE('',*,*,#29394,.F.);
#40853=ORIENTED_EDGE('',*,*,#25485,.T.);
#40854=ORIENTED_EDGE('',*,*,#29392,.T.);
#40855=ORIENTED_EDGE('',*,*,#29395,.F.);
#40856=ORIENTED_EDGE('',*,*,#29396,.F.);
#40857=ORIENTED_EDGE('',*,*,#25486,.T.);
#40858=ORIENTED_EDGE('',*,*,#29394,.T.);
#40859=ORIENTED_EDGE('',*,*,#29397,.F.);
#40860=ORIENTED_EDGE('',*,*,#29398,.F.);
#40861=ORIENTED_EDGE('',*,*,#25487,.T.);
#40862=ORIENTED_EDGE('',*,*,#29396,.T.);
#40863=ORIENTED_EDGE('',*,*,#29399,.F.);
#40864=ORIENTED_EDGE('',*,*,#29400,.F.);
#40865=ORIENTED_EDGE('',*,*,#25488,.T.);
#40866=ORIENTED_EDGE('',*,*,#29398,.T.);
#40867=ORIENTED_EDGE('',*,*,#29401,.F.);
#40868=ORIENTED_EDGE('',*,*,#29402,.F.);
#40869=ORIENTED_EDGE('',*,*,#25489,.T.);
#40870=ORIENTED_EDGE('',*,*,#29400,.T.);
#40871=ORIENTED_EDGE('',*,*,#29403,.F.);
#40872=ORIENTED_EDGE('',*,*,#29404,.F.);
#40873=ORIENTED_EDGE('',*,*,#25490,.T.);
#40874=ORIENTED_EDGE('',*,*,#29402,.T.);
#40875=ORIENTED_EDGE('',*,*,#29405,.F.);
#40876=ORIENTED_EDGE('',*,*,#29406,.F.);
#40877=ORIENTED_EDGE('',*,*,#25491,.T.);
#40878=ORIENTED_EDGE('',*,*,#29404,.T.);
#40879=ORIENTED_EDGE('',*,*,#29407,.F.);
#40880=ORIENTED_EDGE('',*,*,#29408,.F.);
#40881=ORIENTED_EDGE('',*,*,#25492,.T.);
#40882=ORIENTED_EDGE('',*,*,#29406,.T.);
#40883=ORIENTED_EDGE('',*,*,#29409,.F.);
#40884=ORIENTED_EDGE('',*,*,#29410,.F.);
#40885=ORIENTED_EDGE('',*,*,#25493,.T.);
#40886=ORIENTED_EDGE('',*,*,#29408,.T.);
#40887=ORIENTED_EDGE('',*,*,#29411,.F.);
#40888=ORIENTED_EDGE('',*,*,#29412,.F.);
#40889=ORIENTED_EDGE('',*,*,#25494,.T.);
#40890=ORIENTED_EDGE('',*,*,#29410,.T.);
#40891=ORIENTED_EDGE('',*,*,#25464,.T.);
#40892=ORIENTED_EDGE('',*,*,#25495,.T.);
#40893=ORIENTED_EDGE('',*,*,#29412,.T.);
#40894=ORIENTED_EDGE('',*,*,#29413,.F.);
#40895=ORIENTED_EDGE('',*,*,#27500,.F.);
#40896=ORIENTED_EDGE('',*,*,#27261,.T.);
#40897=ORIENTED_EDGE('',*,*,#27049,.T.);
#40898=ORIENTED_EDGE('',*,*,#29386,.F.);
#40899=ORIENTED_EDGE('',*,*,#29414,.F.);
#40900=ORIENTED_EDGE('',*,*,#25466,.T.);
#40901=ORIENTED_EDGE('',*,*,#25500,.T.);
#40902=ORIENTED_EDGE('',*,*,#29385,.F.);
#40903=ORIENTED_EDGE('',*,*,#29415,.F.);
#40904=ORIENTED_EDGE('',*,*,#25467,.T.);
#40905=ORIENTED_EDGE('',*,*,#29414,.T.);
#40906=ORIENTED_EDGE('',*,*,#29384,.F.);
#40907=ORIENTED_EDGE('',*,*,#29416,.F.);
#40908=ORIENTED_EDGE('',*,*,#25468,.T.);
#40909=ORIENTED_EDGE('',*,*,#29415,.T.);
#40910=ORIENTED_EDGE('',*,*,#29383,.F.);
#40911=ORIENTED_EDGE('',*,*,#29417,.F.);
#40912=ORIENTED_EDGE('',*,*,#25469,.T.);
#40913=ORIENTED_EDGE('',*,*,#29416,.T.);
#40914=ORIENTED_EDGE('',*,*,#29382,.F.);
#40915=ORIENTED_EDGE('',*,*,#29418,.F.);
#40916=ORIENTED_EDGE('',*,*,#25470,.T.);
#40917=ORIENTED_EDGE('',*,*,#29417,.T.);
#40918=ORIENTED_EDGE('',*,*,#29381,.F.);
#40919=ORIENTED_EDGE('',*,*,#29419,.F.);
#40920=ORIENTED_EDGE('',*,*,#25471,.T.);
#40921=ORIENTED_EDGE('',*,*,#29418,.T.);
#40922=ORIENTED_EDGE('',*,*,#29380,.F.);
#40923=ORIENTED_EDGE('',*,*,#29420,.F.);
#40924=ORIENTED_EDGE('',*,*,#25472,.T.);
#40925=ORIENTED_EDGE('',*,*,#29419,.T.);
#40926=ORIENTED_EDGE('',*,*,#29379,.F.);
#40927=ORIENTED_EDGE('',*,*,#29421,.F.);
#40928=ORIENTED_EDGE('',*,*,#25473,.T.);
#40929=ORIENTED_EDGE('',*,*,#29420,.T.);
#40930=ORIENTED_EDGE('',*,*,#29378,.F.);
#40931=ORIENTED_EDGE('',*,*,#29422,.F.);
#40932=ORIENTED_EDGE('',*,*,#25474,.T.);
#40933=ORIENTED_EDGE('',*,*,#29421,.T.);
#40934=ORIENTED_EDGE('',*,*,#29377,.F.);
#40935=ORIENTED_EDGE('',*,*,#29423,.F.);
#40936=ORIENTED_EDGE('',*,*,#25475,.T.);
#40937=ORIENTED_EDGE('',*,*,#29422,.T.);
#40938=ORIENTED_EDGE('',*,*,#29376,.F.);
#40939=ORIENTED_EDGE('',*,*,#29424,.F.);
#40940=ORIENTED_EDGE('',*,*,#25476,.T.);
#40941=ORIENTED_EDGE('',*,*,#29423,.T.);
#40942=ORIENTED_EDGE('',*,*,#29375,.F.);
#40943=ORIENTED_EDGE('',*,*,#29425,.F.);
#40944=ORIENTED_EDGE('',*,*,#25477,.T.);
#40945=ORIENTED_EDGE('',*,*,#29424,.T.);
#40946=ORIENTED_EDGE('',*,*,#29374,.F.);
#40947=ORIENTED_EDGE('',*,*,#29426,.F.);
#40948=ORIENTED_EDGE('',*,*,#25478,.T.);
#40949=ORIENTED_EDGE('',*,*,#29425,.T.);
#40950=ORIENTED_EDGE('',*,*,#26868,.T.);
#40951=ORIENTED_EDGE('',*,*,#25479,.T.);
#40952=ORIENTED_EDGE('',*,*,#29426,.T.);
#40953=ORIENTED_EDGE('',*,*,#29373,.F.);
#40954=ORIENTED_EDGE('',*,*,#29427,.F.);
#40955=ORIENTED_EDGE('',*,*,#27406,.T.);
#40956=ORIENTED_EDGE('',*,*,#27263,.T.);
#40957=ORIENTED_EDGE('',*,*,#27435,.T.);
#40958=ORIENTED_EDGE('',*,*,#29428,.T.);
#40959=ORIENTED_EDGE('',*,*,#26871,.T.);
#40960=ORIENTED_EDGE('',*,*,#27407,.T.);
#40961=ORIENTED_EDGE('',*,*,#29427,.T.);
#40962=ORIENTED_EDGE('',*,*,#29372,.T.);
#40963=ORIENTED_EDGE('',*,*,#26876,.T.);
#40964=ORIENTED_EDGE('',*,*,#27405,.T.);
#40965=ORIENTED_EDGE('',*,*,#29346,.T.);
#40966=ORIENTED_EDGE('',*,*,#29318,.T.);
#40967=ORIENTED_EDGE('',*,*,#26881,.T.);
#40968=ORIENTED_EDGE('',*,*,#27403,.T.);
#40969=ORIENTED_EDGE('',*,*,#29292,.T.);
#40970=ORIENTED_EDGE('',*,*,#29264,.T.);
#40971=ORIENTED_EDGE('',*,*,#26886,.T.);
#40972=ORIENTED_EDGE('',*,*,#27401,.T.);
#40973=ORIENTED_EDGE('',*,*,#29238,.T.);
#40974=ORIENTED_EDGE('',*,*,#29210,.T.);
#40975=ORIENTED_EDGE('',*,*,#26891,.T.);
#40976=ORIENTED_EDGE('',*,*,#27399,.T.);
#40977=ORIENTED_EDGE('',*,*,#29184,.T.);
#40978=ORIENTED_EDGE('',*,*,#29156,.T.);
#40979=ORIENTED_EDGE('',*,*,#26896,.T.);
#40980=ORIENTED_EDGE('',*,*,#27397,.T.);
#40981=ORIENTED_EDGE('',*,*,#29130,.T.);
#40982=ORIENTED_EDGE('',*,*,#29102,.T.);
#40983=ORIENTED_EDGE('',*,*,#26901,.T.);
#40984=ORIENTED_EDGE('',*,*,#27395,.T.);
#40985=ORIENTED_EDGE('',*,*,#29076,.T.);
#40986=ORIENTED_EDGE('',*,*,#29048,.T.);
#40987=ORIENTED_EDGE('',*,*,#26906,.T.);
#40988=ORIENTED_EDGE('',*,*,#27393,.T.);
#40989=ORIENTED_EDGE('',*,*,#29022,.T.);
#40990=ORIENTED_EDGE('',*,*,#28994,.T.);
#40991=ORIENTED_EDGE('',*,*,#26911,.T.);
#40992=ORIENTED_EDGE('',*,*,#27391,.T.);
#40993=ORIENTED_EDGE('',*,*,#28968,.T.);
#40994=ORIENTED_EDGE('',*,*,#28940,.T.);
#40995=ORIENTED_EDGE('',*,*,#26916,.T.);
#40996=ORIENTED_EDGE('',*,*,#27389,.T.);
#40997=ORIENTED_EDGE('',*,*,#28914,.T.);
#40998=ORIENTED_EDGE('',*,*,#28886,.T.);
#40999=ORIENTED_EDGE('',*,*,#26921,.T.);
#41000=ORIENTED_EDGE('',*,*,#27387,.T.);
#41001=ORIENTED_EDGE('',*,*,#28860,.T.);
#41002=ORIENTED_EDGE('',*,*,#28832,.T.);
#41003=ORIENTED_EDGE('',*,*,#26926,.T.);
#41004=ORIENTED_EDGE('',*,*,#27385,.T.);
#41005=ORIENTED_EDGE('',*,*,#28806,.T.);
#41006=ORIENTED_EDGE('',*,*,#28778,.T.);
#41007=ORIENTED_EDGE('',*,*,#26931,.T.);
#41008=ORIENTED_EDGE('',*,*,#27383,.T.);
#41009=ORIENTED_EDGE('',*,*,#28752,.T.);
#41010=ORIENTED_EDGE('',*,*,#28724,.T.);
#41011=ORIENTED_EDGE('',*,*,#26936,.T.);
#41012=ORIENTED_EDGE('',*,*,#27381,.T.);
#41013=ORIENTED_EDGE('',*,*,#28698,.T.);
#41014=ORIENTED_EDGE('',*,*,#28670,.T.);
#41015=ORIENTED_EDGE('',*,*,#26941,.T.);
#41016=ORIENTED_EDGE('',*,*,#27379,.T.);
#41017=ORIENTED_EDGE('',*,*,#28644,.T.);
#41018=ORIENTED_EDGE('',*,*,#28616,.T.);
#41019=ORIENTED_EDGE('',*,*,#26946,.T.);
#41020=ORIENTED_EDGE('',*,*,#27377,.T.);
#41021=ORIENTED_EDGE('',*,*,#28590,.T.);
#41022=ORIENTED_EDGE('',*,*,#28562,.T.);
#41023=ORIENTED_EDGE('',*,*,#26951,.T.);
#41024=ORIENTED_EDGE('',*,*,#27375,.T.);
#41025=ORIENTED_EDGE('',*,*,#28536,.T.);
#41026=ORIENTED_EDGE('',*,*,#28508,.T.);
#41027=ORIENTED_EDGE('',*,*,#26956,.T.);
#41028=ORIENTED_EDGE('',*,*,#27373,.T.);
#41029=ORIENTED_EDGE('',*,*,#28482,.T.);
#41030=ORIENTED_EDGE('',*,*,#28454,.T.);
#41031=ORIENTED_EDGE('',*,*,#26961,.T.);
#41032=ORIENTED_EDGE('',*,*,#27371,.T.);
#41033=ORIENTED_EDGE('',*,*,#29429,.T.);
#41034=ORIENTED_EDGE('',*,*,#29430,.F.);
#41035=ORIENTED_EDGE('',*,*,#29429,.F.);
#41036=ORIENTED_EDGE('',*,*,#27370,.T.);
#41037=ORIENTED_EDGE('',*,*,#28428,.T.);
#41038=ORIENTED_EDGE('',*,*,#28400,.T.);
#41039=ORIENTED_EDGE('',*,*,#26966,.T.);
#41040=ORIENTED_EDGE('',*,*,#27368,.T.);
#41041=ORIENTED_EDGE('',*,*,#28374,.T.);
#41042=ORIENTED_EDGE('',*,*,#28346,.T.);
#41043=ORIENTED_EDGE('',*,*,#26971,.T.);
#41044=ORIENTED_EDGE('',*,*,#27366,.T.);
#41045=ORIENTED_EDGE('',*,*,#28320,.T.);
#41046=ORIENTED_EDGE('',*,*,#28292,.T.);
#41047=ORIENTED_EDGE('',*,*,#26976,.T.);
#41048=ORIENTED_EDGE('',*,*,#27364,.T.);
#41049=ORIENTED_EDGE('',*,*,#28266,.T.);
#41050=ORIENTED_EDGE('',*,*,#28238,.T.);
#41051=ORIENTED_EDGE('',*,*,#26981,.T.);
#41052=ORIENTED_EDGE('',*,*,#27362,.T.);
#41053=ORIENTED_EDGE('',*,*,#28212,.T.);
#41054=ORIENTED_EDGE('',*,*,#28184,.T.);
#41055=ORIENTED_EDGE('',*,*,#26986,.T.);
#41056=ORIENTED_EDGE('',*,*,#27360,.T.);
#41057=ORIENTED_EDGE('',*,*,#28158,.T.);
#41058=ORIENTED_EDGE('',*,*,#28130,.T.);
#41059=ORIENTED_EDGE('',*,*,#26991,.T.);
#41060=ORIENTED_EDGE('',*,*,#27358,.T.);
#41061=ORIENTED_EDGE('',*,*,#28104,.T.);
#41062=ORIENTED_EDGE('',*,*,#28076,.T.);
#41063=ORIENTED_EDGE('',*,*,#26996,.T.);
#41064=ORIENTED_EDGE('',*,*,#27356,.T.);
#41065=ORIENTED_EDGE('',*,*,#28050,.T.);
#41066=ORIENTED_EDGE('',*,*,#28022,.T.);
#41067=ORIENTED_EDGE('',*,*,#27001,.T.);
#41068=ORIENTED_EDGE('',*,*,#27354,.T.);
#41069=ORIENTED_EDGE('',*,*,#27996,.T.);
#41070=ORIENTED_EDGE('',*,*,#27968,.T.);
#41071=ORIENTED_EDGE('',*,*,#27006,.T.);
#41072=ORIENTED_EDGE('',*,*,#27352,.T.);
#41073=ORIENTED_EDGE('',*,*,#27942,.T.);
#41074=ORIENTED_EDGE('',*,*,#27914,.T.);
#41075=ORIENTED_EDGE('',*,*,#27011,.T.);
#41076=ORIENTED_EDGE('',*,*,#27350,.T.);
#41077=ORIENTED_EDGE('',*,*,#27888,.T.);
#41078=ORIENTED_EDGE('',*,*,#27860,.T.);
#41079=ORIENTED_EDGE('',*,*,#27016,.T.);
#41080=ORIENTED_EDGE('',*,*,#27348,.T.);
#41081=ORIENTED_EDGE('',*,*,#27834,.T.);
#41082=ORIENTED_EDGE('',*,*,#27806,.T.);
#41083=ORIENTED_EDGE('',*,*,#27021,.T.);
#41084=ORIENTED_EDGE('',*,*,#27346,.T.);
#41085=ORIENTED_EDGE('',*,*,#27780,.T.);
#41086=ORIENTED_EDGE('',*,*,#27752,.T.);
#41087=ORIENTED_EDGE('',*,*,#27026,.T.);
#41088=ORIENTED_EDGE('',*,*,#27344,.T.);
#41089=ORIENTED_EDGE('',*,*,#27726,.T.);
#41090=ORIENTED_EDGE('',*,*,#27698,.T.);
#41091=ORIENTED_EDGE('',*,*,#27031,.T.);
#41092=ORIENTED_EDGE('',*,*,#27342,.T.);
#41093=ORIENTED_EDGE('',*,*,#27672,.T.);
#41094=ORIENTED_EDGE('',*,*,#27644,.T.);
#41095=ORIENTED_EDGE('',*,*,#27036,.T.);
#41096=ORIENTED_EDGE('',*,*,#27340,.T.);
#41097=ORIENTED_EDGE('',*,*,#27618,.T.);
#41098=ORIENTED_EDGE('',*,*,#27590,.T.);
#41099=ORIENTED_EDGE('',*,*,#27041,.T.);
#41100=ORIENTED_EDGE('',*,*,#27338,.T.);
#41101=ORIENTED_EDGE('',*,*,#27564,.T.);
#41102=ORIENTED_EDGE('',*,*,#27536,.T.);
#41103=ORIENTED_EDGE('',*,*,#27046,.T.);
#41104=ORIENTED_EDGE('',*,*,#27336,.T.);
#41105=ORIENTED_EDGE('',*,*,#29431,.T.);
#41106=ORIENTED_EDGE('',*,*,#29432,.T.);
#41107=ORIENTED_EDGE('',*,*,#29433,.T.);
#41108=ORIENTED_EDGE('',*,*,#29434,.T.);
#41109=ORIENTED_EDGE('',*,*,#29432,.F.);
#41110=ORIENTED_EDGE('',*,*,#29433,.F.);
#41111=ORIENTED_EDGE('',*,*,#29434,.F.);
#41112=ORIENTED_EDGE('',*,*,#29435,.T.);
#41113=ORIENTED_EDGE('',*,*,#29436,.F.);
#41114=ORIENTED_EDGE('',*,*,#29437,.F.);
#41115=ORIENTED_EDGE('',*,*,#29435,.F.);
#41116=ORIENTED_EDGE('',*,*,#29431,.F.);
#41117=ORIENTED_EDGE('',*,*,#27462,.F.);
#41118=ORIENTED_EDGE('',*,*,#29436,.T.);
#41119=ORIENTED_EDGE('',*,*,#29437,.T.);
#41120=ORIENTED_EDGE('',*,*,#29438,.T.);
#41121=ORIENTED_EDGE('',*,*,#29439,.T.);
#41122=ORIENTED_EDGE('',*,*,#29440,.T.);
#41123=ORIENTED_EDGE('',*,*,#29438,.F.);
#41124=ORIENTED_EDGE('',*,*,#29440,.F.);
#41125=ORIENTED_EDGE('',*,*,#29441,.T.);
#41126=ORIENTED_EDGE('',*,*,#29442,.T.);
#41127=ORIENTED_EDGE('',*,*,#29441,.F.);
#41128=ORIENTED_EDGE('',*,*,#29439,.F.);
#41129=ORIENTED_EDGE('',*,*,#29443,.T.);
#41130=ORIENTED_EDGE('',*,*,#29444,.T.);
#41131=ORIENTED_EDGE('',*,*,#29445,.T.);
#41132=ORIENTED_EDGE('',*,*,#29444,.F.);
#41133=ORIENTED_EDGE('',*,*,#29446,.T.);
#41134=ORIENTED_EDGE('',*,*,#29443,.F.);
#41135=ORIENTED_EDGE('',*,*,#29447,.T.);
#41136=ORIENTED_EDGE('',*,*,#29448,.F.);
#41137=ORIENTED_EDGE('',*,*,#29449,.F.);
#41138=ORIENTED_EDGE('',*,*,#29447,.F.);
#41139=ORIENTED_EDGE('',*,*,#29446,.F.);
#41140=ORIENTED_EDGE('',*,*,#29450,.F.);
#41141=ORIENTED_EDGE('',*,*,#29445,.F.);
#41142=ORIENTED_EDGE('',*,*,#29451,.T.);
#41143=ORIENTED_EDGE('',*,*,#29452,.T.);
#41144=ORIENTED_EDGE('',*,*,#29448,.T.);
#41145=ORIENTED_EDGE('',*,*,#29449,.T.);
#41146=ORIENTED_EDGE('',*,*,#29452,.F.);
#41147=ORIENTED_EDGE('',*,*,#29453,.T.);
#41148=ORIENTED_EDGE('',*,*,#29451,.F.);
#41149=ORIENTED_EDGE('',*,*,#26759,.T.);
#41150=ORIENTED_EDGE('',*,*,#27501,.T.);
#41151=ORIENTED_EDGE('',*,*,#29413,.T.);
#41152=ORIENTED_EDGE('',*,*,#29411,.T.);
#41153=ORIENTED_EDGE('',*,*,#29409,.T.);
#41154=ORIENTED_EDGE('',*,*,#29407,.T.);
#41155=ORIENTED_EDGE('',*,*,#29405,.T.);
#41156=ORIENTED_EDGE('',*,*,#29403,.T.);
#41157=ORIENTED_EDGE('',*,*,#29401,.T.);
#41158=ORIENTED_EDGE('',*,*,#29399,.T.);
#41159=ORIENTED_EDGE('',*,*,#29397,.T.);
#41160=ORIENTED_EDGE('',*,*,#29395,.T.);
#41161=ORIENTED_EDGE('',*,*,#29393,.T.);
#41162=ORIENTED_EDGE('',*,*,#29391,.T.);
#41163=ORIENTED_EDGE('',*,*,#29389,.T.);
#41164=ORIENTED_EDGE('',*,*,#29387,.T.);
#41165=ORIENTED_EDGE('',*,*,#26872,.T.);
#41166=ORIENTED_EDGE('',*,*,#29428,.F.);
#41167=ORIENTED_EDGE('',*,*,#27434,.T.);
#41168=ORIENTED_EDGE('',*,*,#27432,.T.);
#41169=ORIENTED_EDGE('',*,*,#27430,.T.);
#41170=ORIENTED_EDGE('',*,*,#27428,.T.);
#41171=ORIENTED_EDGE('',*,*,#27426,.T.);
#41172=ORIENTED_EDGE('',*,*,#27424,.T.);
#41173=ORIENTED_EDGE('',*,*,#27422,.T.);
#41174=ORIENTED_EDGE('',*,*,#27420,.T.);
#41175=ORIENTED_EDGE('',*,*,#27418,.T.);
#41176=ORIENTED_EDGE('',*,*,#27416,.T.);
#41177=ORIENTED_EDGE('',*,*,#27414,.T.);
#41178=ORIENTED_EDGE('',*,*,#27412,.T.);
#41179=ORIENTED_EDGE('',*,*,#27410,.T.);
#41180=ORIENTED_EDGE('',*,*,#27408,.T.);
#41181=ORIENTED_EDGE('',*,*,#29454,.F.);
#41182=ORIENTED_EDGE('',*,*,#29430,.T.);
#41183=ORIENTED_EDGE('',*,*,#29455,.F.);
#41184=ORIENTED_EDGE('',*,*,#29456,.T.);
#41185=ORIENTED_EDGE('',*,*,#29454,.T.);
#41186=ORIENTED_EDGE('',*,*,#29456,.F.);
#41187=ORIENTED_EDGE('',*,*,#29457,.F.);
#41188=ORIENTED_EDGE('',*,*,#29458,.T.);
#41189=ORIENTED_EDGE('',*,*,#29455,.T.);
#41190=ORIENTED_EDGE('',*,*,#29458,.F.);
#41191=ORIENTED_EDGE('',*,*,#29453,.F.);
#41192=ORIENTED_EDGE('',*,*,#29459,.T.);
#41193=ORIENTED_EDGE('',*,*,#29457,.T.);
#41194=ORIENTED_EDGE('',*,*,#29459,.F.);
#41195=ORIENTED_EDGE('',*,*,#29460,.F.);
#41196=ORIENTED_EDGE('',*,*,#29461,.T.);
#41197=ORIENTED_EDGE('',*,*,#29450,.T.);
#41198=ORIENTED_EDGE('',*,*,#29461,.F.);
#41199=ORIENTED_EDGE('',*,*,#29442,.F.);
#41200=ORIENTED_EDGE('',*,*,#29462,.T.);
#41201=ORIENTED_EDGE('',*,*,#29460,.T.);
#41202=ORIENTED_EDGE('',*,*,#29462,.F.);
#48115=CONICAL_SURFACE('',#51189,38.8,0.785398163397448);
#48116=CONICAL_SURFACE('',#51191,38.8,0.785398163397448);
#48117=CONICAL_SURFACE('',#51193,38.8,0.785398163397448);
#48118=CONICAL_SURFACE('',#51195,38.8,0.785398163397448);
#48119=CONICAL_SURFACE('',#51197,38.8,0.785398163397448);
#48120=CONICAL_SURFACE('',#51199,38.8,0.785398163397448);
#48121=CONICAL_SURFACE('',#51201,38.8,0.785398163397448);
#48122=CONICAL_SURFACE('',#51203,38.8,0.785398163397448);
#48123=CONICAL_SURFACE('',#51205,38.8,0.785398163397448);
#48124=CONICAL_SURFACE('',#51207,38.8,0.785398163397448);
#48125=CONICAL_SURFACE('',#51209,38.8,0.785398163397448);
#48126=CONICAL_SURFACE('',#51211,38.8,0.785398163397448);
#48127=CONICAL_SURFACE('',#51213,38.8,0.785398163397448);
#48128=CONICAL_SURFACE('',#51215,38.8,0.785398163397448);
#48129=CONICAL_SURFACE('',#51217,38.8,0.785398163397448);
#48130=CONICAL_SURFACE('',#51219,38.8,0.785398163397448);
#48131=CONICAL_SURFACE('',#51221,38.8,0.785398163397448);
#48132=CONICAL_SURFACE('',#51223,38.8,0.785398163397448);
#48133=CONICAL_SURFACE('',#51225,38.8,0.785398163397448);
#48134=CONICAL_SURFACE('',#51227,38.8,0.785398163397448);
#48135=CONICAL_SURFACE('',#51229,38.8,0.785398163397448);
#48136=CONICAL_SURFACE('',#51231,38.8,0.785398163397448);
#48137=CONICAL_SURFACE('',#51233,38.8,0.785398163397448);
#48138=CONICAL_SURFACE('',#51235,38.8,0.785398163397448);
#48139=CONICAL_SURFACE('',#51237,38.8,0.785398163397448);
#48140=CONICAL_SURFACE('',#51239,38.8,0.785398163397448);
#48141=CONICAL_SURFACE('',#51241,38.8,0.785398163397448);
#48142=CONICAL_SURFACE('',#51243,38.8,0.785398163397448);
#48143=CONICAL_SURFACE('',#51245,38.8,0.785398163397448);
#48144=CONICAL_SURFACE('',#51247,38.8,0.785398163397448);
#48145=CONICAL_SURFACE('',#51249,38.8,0.785398163397448);
#48146=CONICAL_SURFACE('',#51251,38.8,0.785398163397448);
#48147=CONICAL_SURFACE('',#51253,38.8,0.785398163397448);
#48148=CONICAL_SURFACE('',#51255,38.8,0.785398163397448);
#48149=CONICAL_SURFACE('',#51257,38.8,0.785398163397448);
#48150=CONICAL_SURFACE('',#51259,38.8,0.785398163397448);
#48151=CONICAL_SURFACE('',#51369,38.8,0.785398163397448);
#48152=CONICAL_SURFACE('',#51371,38.8,0.785398163397448);
#48153=CONICAL_SURFACE('',#51373,38.8,0.785398163397448);
#48154=CONICAL_SURFACE('',#51375,38.8,0.785398163397448);
#48155=CONICAL_SURFACE('',#51377,38.8,0.785398163397448);
#48156=CONICAL_SURFACE('',#51379,38.8,0.785398163397448);
#48157=CONICAL_SURFACE('',#51381,38.8,0.785398163397448);
#48158=CONICAL_SURFACE('',#51383,38.8,0.785398163397448);
#48159=CONICAL_SURFACE('',#51385,38.8,0.785398163397448);
#48160=CONICAL_SURFACE('',#51387,38.8,0.785398163397448);
#48161=CONICAL_SURFACE('',#51389,38.8,0.785398163397448);
#48162=CONICAL_SURFACE('',#51391,38.8,0.785398163397448);
#48163=CONICAL_SURFACE('',#51393,38.8,0.785398163397448);
#48164=CONICAL_SURFACE('',#51395,38.8,0.785398163397448);
#48165=CONICAL_SURFACE('',#51397,38.8,0.785398163397448);
#48166=CONICAL_SURFACE('',#51399,38.8,0.785398163397448);
#48167=CONICAL_SURFACE('',#51401,38.8,0.785398163397448);
#48168=CONICAL_SURFACE('',#51403,38.8,0.785398163397448);
#48169=CONICAL_SURFACE('',#51405,38.8,0.785398163397448);
#48170=CONICAL_SURFACE('',#51407,38.8,0.785398163397448);
#48171=CONICAL_SURFACE('',#51409,38.8,0.785398163397448);
#48172=CONICAL_SURFACE('',#51411,38.8,0.785398163397448);
#48173=CONICAL_SURFACE('',#51413,38.8,0.785398163397448);
#48174=CONICAL_SURFACE('',#51415,38.8,0.785398163397448);
#48175=CONICAL_SURFACE('',#51417,38.8,0.785398163397448);
#48176=CONICAL_SURFACE('',#51419,38.8,0.785398163397448);
#48177=CONICAL_SURFACE('',#51421,38.8,0.785398163397448);
#48178=CONICAL_SURFACE('',#51423,38.8,0.785398163397448);
#48179=CONICAL_SURFACE('',#51425,38.8,0.785398163397448);
#48180=CONICAL_SURFACE('',#51427,38.8,0.785398163397448);
#48181=CONICAL_SURFACE('',#51429,38.8,0.785398163397448);
#48182=CONICAL_SURFACE('',#51431,38.8,0.785398163397448);
#48183=CONICAL_SURFACE('',#51433,38.8,0.785398163397448);
#48184=CONICAL_SURFACE('',#51435,38.8,0.785398163397448);
#48185=CONICAL_SURFACE('',#51437,38.8,0.785398163397448);
#48186=CONICAL_SURFACE('',#51439,38.8,0.785398163397448);
#48187=CONICAL_SURFACE('',#51741,42.6,0.785398163397452);
#48188=CONICAL_SURFACE('',#53565,42.6,0.785398163397452);
#48189=CONICAL_SURFACE('',#53568,47.3660700849456,0.953735573090811);
#48190=CONICAL_SURFACE('',#53572,49.25,0.336674819386727);
#48191=CONICAL_SURFACE('',#53600,50.1,0.785398163397443);
#48192=CONICAL_SURFACE('',#53604,50.25,0.785398163397446);
#48193=CONICAL_SURFACE('',#53607,50.7,1.10714871779409);
#48336=ADVANCED_FACE('',(#13249),#48115,.F.);
#48337=ADVANCED_FACE('',(#13250),#48116,.F.);
#48338=ADVANCED_FACE('',(#13251),#48117,.F.);
#48339=ADVANCED_FACE('',(#13252),#48118,.F.);
#48340=ADVANCED_FACE('',(#13253),#48119,.F.);
#48341=ADVANCED_FACE('',(#13254),#48120,.F.);
#48342=ADVANCED_FACE('',(#13255),#48121,.F.);
#48343=ADVANCED_FACE('',(#13256),#48122,.F.);
#48344=ADVANCED_FACE('',(#13257),#48123,.F.);
#48345=ADVANCED_FACE('',(#13258),#48124,.F.);
#48346=ADVANCED_FACE('',(#13259),#48125,.F.);
#48347=ADVANCED_FACE('',(#13260),#48126,.F.);
#48348=ADVANCED_FACE('',(#13261),#48127,.F.);
#48349=ADVANCED_FACE('',(#13262),#48128,.F.);
#48350=ADVANCED_FACE('',(#13263),#48129,.F.);
#48351=ADVANCED_FACE('',(#13264),#48130,.F.);
#48352=ADVANCED_FACE('',(#13265),#48131,.F.);
#48353=ADVANCED_FACE('',(#13266),#48132,.F.);
#48354=ADVANCED_FACE('',(#13267),#48133,.F.);
#48355=ADVANCED_FACE('',(#13268),#48134,.F.);
#48356=ADVANCED_FACE('',(#13269),#48135,.F.);
#48357=ADVANCED_FACE('',(#13270),#48136,.F.);
#48358=ADVANCED_FACE('',(#13271),#48137,.F.);
#48359=ADVANCED_FACE('',(#13272),#48138,.F.);
#48360=ADVANCED_FACE('',(#13273),#48139,.F.);
#48361=ADVANCED_FACE('',(#13274),#48140,.F.);
#48362=ADVANCED_FACE('',(#13275),#48141,.F.);
#48363=ADVANCED_FACE('',(#13276),#48142,.F.);
#48364=ADVANCED_FACE('',(#13277),#48143,.F.);
#48365=ADVANCED_FACE('',(#13278),#48144,.F.);
#48366=ADVANCED_FACE('',(#13279),#48145,.F.);
#48367=ADVANCED_FACE('',(#13280),#48146,.F.);
#48368=ADVANCED_FACE('',(#13281),#48147,.F.);
#48369=ADVANCED_FACE('',(#13282),#48148,.F.);
#48370=ADVANCED_FACE('',(#13283),#48149,.F.);
#48371=ADVANCED_FACE('',(#13284),#48150,.F.);
#48372=ADVANCED_FACE('',(#13285),#11216,.F.);
#48373=ADVANCED_FACE('',(#13286),#11217,.T.);
#48374=ADVANCED_FACE('',(#13287),#11218,.F.);
#48375=ADVANCED_FACE('',(#13288),#11219,.T.);
#48376=ADVANCED_FACE('',(#13289),#11220,.F.);
#48377=ADVANCED_FACE('',(#13290),#11221,.T.);
#48378=ADVANCED_FACE('',(#13291),#11222,.F.);
#48379=ADVANCED_FACE('',(#13292),#11223,.T.);
#48380=ADVANCED_FACE('',(#13293),#11224,.F.);
#48381=ADVANCED_FACE('',(#13294),#11225,.T.);
#48382=ADVANCED_FACE('',(#13295),#11226,.F.);
#48383=ADVANCED_FACE('',(#13296),#11227,.T.);
#48384=ADVANCED_FACE('',(#13297),#11228,.F.);
#48385=ADVANCED_FACE('',(#13298),#11229,.T.);
#48386=ADVANCED_FACE('',(#13299),#11230,.F.);
#48387=ADVANCED_FACE('',(#13300),#11231,.T.);
#48388=ADVANCED_FACE('',(#13301),#11232,.F.);
#48389=ADVANCED_FACE('',(#13302),#11233,.T.);
#48390=ADVANCED_FACE('',(#13303),#11234,.F.);
#48391=ADVANCED_FACE('',(#13304),#11235,.T.);
#48392=ADVANCED_FACE('',(#13305),#11236,.F.);
#48393=ADVANCED_FACE('',(#13306),#11237,.T.);
#48394=ADVANCED_FACE('',(#13307),#11238,.F.);
#48395=ADVANCED_FACE('',(#13308),#11239,.T.);
#48396=ADVANCED_FACE('',(#13309),#11240,.F.);
#48397=ADVANCED_FACE('',(#13310),#11241,.T.);
#48398=ADVANCED_FACE('',(#13311),#11242,.F.);
#48399=ADVANCED_FACE('',(#13312),#11243,.T.);
#48400=ADVANCED_FACE('',(#13313),#11244,.F.);
#48401=ADVANCED_FACE('',(#13314),#11245,.T.);
#48402=ADVANCED_FACE('',(#13315),#11246,.F.);
#48403=ADVANCED_FACE('',(#13316),#11247,.T.);
#48404=ADVANCED_FACE('',(#13317),#11248,.F.);
#48405=ADVANCED_FACE('',(#13318),#11249,.T.);
#48406=ADVANCED_FACE('',(#13319),#11250,.F.);
#48407=ADVANCED_FACE('',(#13320),#11251,.T.);
#48408=ADVANCED_FACE('',(#13321),#11252,.F.);
#48409=ADVANCED_FACE('',(#13322),#11253,.T.);
#48410=ADVANCED_FACE('',(#13323),#11254,.F.);
#48411=ADVANCED_FACE('',(#13324),#11255,.T.);
#48412=ADVANCED_FACE('',(#13325),#11256,.F.);
#48413=ADVANCED_FACE('',(#13326),#11257,.T.);
#48414=ADVANCED_FACE('',(#13327),#11258,.F.);
#48415=ADVANCED_FACE('',(#13328),#11259,.T.);
#48416=ADVANCED_FACE('',(#13329),#11260,.F.);
#48417=ADVANCED_FACE('',(#13330),#11261,.T.);
#48418=ADVANCED_FACE('',(#13331),#11262,.F.);
#48419=ADVANCED_FACE('',(#13332),#11263,.T.);
#48420=ADVANCED_FACE('',(#13333),#11264,.F.);
#48421=ADVANCED_FACE('',(#13334),#11265,.T.);
#48422=ADVANCED_FACE('',(#13335),#11266,.F.);
#48423=ADVANCED_FACE('',(#13336),#11267,.T.);
#48424=ADVANCED_FACE('',(#13337),#11268,.F.);
#48425=ADVANCED_FACE('',(#13338),#11269,.T.);
#48426=ADVANCED_FACE('',(#13339),#11270,.F.);
#48427=ADVANCED_FACE('',(#13340),#11271,.T.);
#48428=ADVANCED_FACE('',(#13341),#11272,.F.);
#48429=ADVANCED_FACE('',(#13342),#11273,.T.);
#48430=ADVANCED_FACE('',(#13343),#11274,.F.);
#48431=ADVANCED_FACE('',(#13344),#11275,.T.);
#48432=ADVANCED_FACE('',(#13345),#11276,.F.);
#48433=ADVANCED_FACE('',(#13346),#11277,.T.);
#48434=ADVANCED_FACE('',(#13347),#11278,.F.);
#48435=ADVANCED_FACE('',(#13348),#11279,.T.);
#48436=ADVANCED_FACE('',(#13349),#11280,.F.);
#48437=ADVANCED_FACE('',(#13350),#11281,.T.);
#48438=ADVANCED_FACE('',(#13351),#11282,.F.);
#48439=ADVANCED_FACE('',(#13352),#11283,.T.);
#48440=ADVANCED_FACE('',(#13353),#11284,.F.);
#48441=ADVANCED_FACE('',(#13354),#11285,.T.);
#48442=ADVANCED_FACE('',(#13355),#11286,.F.);
#48443=ADVANCED_FACE('',(#13356),#11287,.T.);
#48444=ADVANCED_FACE('',(#13357),#48151,.F.);
#48445=ADVANCED_FACE('',(#13358),#48152,.F.);
#48446=ADVANCED_FACE('',(#13359),#48153,.F.);
#48447=ADVANCED_FACE('',(#13360),#48154,.F.);
#48448=ADVANCED_FACE('',(#13361),#48155,.F.);
#48449=ADVANCED_FACE('',(#13362),#48156,.F.);
#48450=ADVANCED_FACE('',(#13363),#48157,.F.);
#48451=ADVANCED_FACE('',(#13364),#48158,.F.);
#48452=ADVANCED_FACE('',(#13365),#48159,.F.);
#48453=ADVANCED_FACE('',(#13366),#48160,.F.);
#48454=ADVANCED_FACE('',(#13367),#48161,.F.);
#48455=ADVANCED_FACE('',(#13368),#48162,.F.);
#48456=ADVANCED_FACE('',(#13369),#48163,.F.);
#48457=ADVANCED_FACE('',(#13370),#48164,.F.);
#48458=ADVANCED_FACE('',(#13371),#48165,.F.);
#48459=ADVANCED_FACE('',(#13372),#48166,.F.);
#48460=ADVANCED_FACE('',(#13373),#48167,.F.);
#48461=ADVANCED_FACE('',(#13374),#48168,.F.);
#48462=ADVANCED_FACE('',(#13375),#48169,.F.);
#48463=ADVANCED_FACE('',(#13376),#48170,.F.);
#48464=ADVANCED_FACE('',(#13377),#48171,.F.);
#48465=ADVANCED_FACE('',(#13378),#48172,.F.);
#48466=ADVANCED_FACE('',(#13379),#48173,.F.);
#48467=ADVANCED_FACE('',(#13380),#48174,.F.);
#48468=ADVANCED_FACE('',(#13381),#48175,.F.);
#48469=ADVANCED_FACE('',(#13382),#48176,.F.);
#48470=ADVANCED_FACE('',(#13383),#48177,.F.);
#48471=ADVANCED_FACE('',(#13384),#48178,.F.);
#48472=ADVANCED_FACE('',(#13385),#48179,.F.);
#48473=ADVANCED_FACE('',(#13386),#48180,.F.);
#48474=ADVANCED_FACE('',(#13387),#48181,.F.);
#48475=ADVANCED_FACE('',(#13388),#48182,.F.);
#48476=ADVANCED_FACE('',(#13389),#48183,.F.);
#48477=ADVANCED_FACE('',(#13390),#48184,.F.);
#48478=ADVANCED_FACE('',(#13391),#48185,.F.);
#48479=ADVANCED_FACE('',(#13392),#48186,.F.);
#48480=ADVANCED_FACE('',(#13393),#11288,.T.);
#48481=ADVANCED_FACE('',(#13394),#11289,.T.);
#48482=ADVANCED_FACE('',(#13395),#11290,.T.);
#48483=ADVANCED_FACE('',(#13396),#11291,.T.);
#48484=ADVANCED_FACE('',(#13397),#11292,.T.);
#48485=ADVANCED_FACE('',(#13398),#11293,.T.);
#48486=ADVANCED_FACE('',(#13399),#11294,.T.);
#48487=ADVANCED_FACE('',(#13400),#11295,.T.);
#48488=ADVANCED_FACE('',(#13401),#11296,.T.);
#48489=ADVANCED_FACE('',(#13402),#11297,.T.);
#48490=ADVANCED_FACE('',(#13403),#11298,.T.);
#48491=ADVANCED_FACE('',(#13404),#11299,.T.);
#48492=ADVANCED_FACE('',(#13405),#11300,.T.);
#48493=ADVANCED_FACE('',(#13406),#11301,.T.);
#48494=ADVANCED_FACE('',(#13407),#11302,.T.);
#48495=ADVANCED_FACE('',(#13408),#11303,.T.);
#48496=ADVANCED_FACE('',(#13409),#11304,.T.);
#48497=ADVANCED_FACE('',(#13410),#11305,.T.);
#48498=ADVANCED_FACE('',(#13411),#11306,.T.);
#48499=ADVANCED_FACE('',(#13412),#11307,.T.);
#48500=ADVANCED_FACE('',(#13413),#11308,.T.);
#48501=ADVANCED_FACE('',(#13414),#11309,.T.);
#48502=ADVANCED_FACE('',(#13415),#11310,.T.);
#48503=ADVANCED_FACE('',(#13416),#11311,.T.);
#48504=ADVANCED_FACE('',(#13417),#11312,.T.);
#48505=ADVANCED_FACE('',(#13418),#11313,.T.);
#48506=ADVANCED_FACE('',(#13419),#11314,.T.);
#48507=ADVANCED_FACE('',(#13420),#11315,.T.);
#48508=ADVANCED_FACE('',(#13421),#11316,.T.);
#48509=ADVANCED_FACE('',(#13422),#11317,.T.);
#48510=ADVANCED_FACE('',(#13423),#11318,.T.);
#48511=ADVANCED_FACE('',(#13424),#11319,.T.);
#48512=ADVANCED_FACE('',(#13425),#11320,.T.);
#48513=ADVANCED_FACE('',(#13426),#11321,.T.);
#48514=ADVANCED_FACE('',(#13427),#11322,.T.);
#48515=ADVANCED_FACE('',(#13428),#11323,.T.);
#48516=ADVANCED_FACE('',(#13429),#11324,.F.);
#48517=ADVANCED_FACE('',(#13430),#11325,.F.);
#48518=ADVANCED_FACE('',(#13431),#11326,.F.);
#48519=ADVANCED_FACE('',(#13432),#11327,.F.);
#48520=ADVANCED_FACE('',(#13433),#11328,.F.);
#48521=ADVANCED_FACE('',(#13434),#11329,.F.);
#48522=ADVANCED_FACE('',(#13435),#11330,.F.);
#48523=ADVANCED_FACE('',(#13436),#11331,.F.);
#48524=ADVANCED_FACE('',(#13437),#11332,.F.);
#48525=ADVANCED_FACE('',(#13438),#11333,.F.);
#48526=ADVANCED_FACE('',(#13439),#11334,.F.);
#48527=ADVANCED_FACE('',(#13440),#11335,.F.);
#48528=ADVANCED_FACE('',(#13441),#11336,.F.);
#48529=ADVANCED_FACE('',(#13442),#11337,.F.);
#48530=ADVANCED_FACE('',(#13443),#11338,.F.);
#48531=ADVANCED_FACE('',(#13444),#11339,.F.);
#48532=ADVANCED_FACE('',(#13445),#11340,.F.);
#48533=ADVANCED_FACE('',(#13446),#11341,.F.);
#48534=ADVANCED_FACE('',(#13447),#11342,.F.);
#48535=ADVANCED_FACE('',(#13448),#11343,.F.);
#48536=ADVANCED_FACE('',(#13449),#11344,.F.);
#48537=ADVANCED_FACE('',(#13450),#11345,.F.);
#48538=ADVANCED_FACE('',(#13451),#11346,.F.);
#48539=ADVANCED_FACE('',(#13452),#11347,.F.);
#48540=ADVANCED_FACE('',(#13453),#11348,.F.);
#48541=ADVANCED_FACE('',(#13454),#11349,.F.);
#48542=ADVANCED_FACE('',(#13455),#11350,.F.);
#48543=ADVANCED_FACE('',(#13456),#11351,.F.);
#48544=ADVANCED_FACE('',(#13457),#11352,.F.);
#48545=ADVANCED_FACE('',(#13458),#11353,.F.);
#48546=ADVANCED_FACE('',(#13459),#11354,.F.);
#48547=ADVANCED_FACE('',(#13460),#11355,.F.);
#48548=ADVANCED_FACE('',(#13461),#11356,.F.);
#48549=ADVANCED_FACE('',(#13462),#11357,.F.);
#48550=ADVANCED_FACE('',(#13463),#11358,.F.);
#48551=ADVANCED_FACE('',(#13464),#11359,.F.);
#48552=ADVANCED_FACE('',(#13465),#11360,.T.);
#48553=ADVANCED_FACE('',(#13466),#11361,.T.);
#48554=ADVANCED_FACE('',(#13467),#11362,.T.);
#48555=ADVANCED_FACE('',(#13468),#11363,.T.);
#48556=ADVANCED_FACE('',(#13469),#11364,.T.);
#48557=ADVANCED_FACE('',(#13470),#11365,.T.);
#48558=ADVANCED_FACE('',(#13471),#11366,.T.);
#48559=ADVANCED_FACE('',(#13472),#11367,.T.);
#48560=ADVANCED_FACE('',(#13473),#11368,.T.);
#48561=ADVANCED_FACE('',(#13474),#11369,.T.);
#48562=ADVANCED_FACE('',(#13475),#11370,.T.);
#48563=ADVANCED_FACE('',(#13476),#11371,.T.);
#48564=ADVANCED_FACE('',(#13477),#11372,.T.);
#48565=ADVANCED_FACE('',(#13478),#11373,.T.);
#48566=ADVANCED_FACE('',(#13479),#11374,.T.);
#48567=ADVANCED_FACE('',(#13480),#11375,.T.);
#48568=ADVANCED_FACE('',(#13481),#11376,.T.);
#48569=ADVANCED_FACE('',(#13482),#11377,.T.);
#48570=ADVANCED_FACE('',(#13483),#11378,.T.);
#48571=ADVANCED_FACE('',(#13484),#11379,.T.);
#48572=ADVANCED_FACE('',(#13485),#11380,.T.);
#48573=ADVANCED_FACE('',(#13486),#11381,.T.);
#48574=ADVANCED_FACE('',(#13487),#11382,.T.);
#48575=ADVANCED_FACE('',(#13488),#11383,.T.);
#48576=ADVANCED_FACE('',(#13489),#11384,.T.);
#48577=ADVANCED_FACE('',(#13490),#11385,.T.);
#48578=ADVANCED_FACE('',(#13491),#11386,.T.);
#48579=ADVANCED_FACE('',(#13492),#11387,.T.);
#48580=ADVANCED_FACE('',(#13493),#11388,.T.);
#48581=ADVANCED_FACE('',(#13494),#11389,.T.);
#48582=ADVANCED_FACE('',(#13495),#11390,.T.);
#48583=ADVANCED_FACE('',(#13496),#11391,.T.);
#48584=ADVANCED_FACE('',(#13497),#11392,.T.);
#48585=ADVANCED_FACE('',(#13498),#11393,.T.);
#48586=ADVANCED_FACE('',(#13499),#11394,.T.);
#48587=ADVANCED_FACE('',(#13500),#11395,.T.);
#48588=ADVANCED_FACE('',(#13501),#11396,.F.);
#48589=ADVANCED_FACE('',(#13502),#11397,.F.);
#48590=ADVANCED_FACE('',(#13503),#11398,.F.);
#48591=ADVANCED_FACE('',(#13504),#11399,.F.);
#48592=ADVANCED_FACE('',(#13505),#11400,.F.);
#48593=ADVANCED_FACE('',(#13506),#11401,.F.);
#48594=ADVANCED_FACE('',(#13507),#11402,.F.);
#48595=ADVANCED_FACE('',(#13508),#11403,.F.);
#48596=ADVANCED_FACE('',(#13509),#11404,.F.);
#48597=ADVANCED_FACE('',(#13510),#11405,.F.);
#48598=ADVANCED_FACE('',(#13511),#11406,.F.);
#48599=ADVANCED_FACE('',(#13512),#11407,.F.);
#48600=ADVANCED_FACE('',(#13513),#11408,.F.);
#48601=ADVANCED_FACE('',(#13514),#11409,.F.);
#48602=ADVANCED_FACE('',(#13515),#11410,.F.);
#48603=ADVANCED_FACE('',(#13516),#11411,.F.);
#48604=ADVANCED_FACE('',(#13517),#11412,.F.);
#48605=ADVANCED_FACE('',(#13518),#11413,.F.);
#48606=ADVANCED_FACE('',(#13519),#11414,.F.);
#48607=ADVANCED_FACE('',(#13520),#11415,.F.);
#48608=ADVANCED_FACE('',(#13521),#11416,.F.);
#48609=ADVANCED_FACE('',(#13522),#11417,.F.);
#48610=ADVANCED_FACE('',(#13523),#11418,.F.);
#48611=ADVANCED_FACE('',(#13524),#11419,.F.);
#48612=ADVANCED_FACE('',(#13525),#11420,.F.);
#48613=ADVANCED_FACE('',(#13526),#11421,.F.);
#48614=ADVANCED_FACE('',(#13527),#11422,.F.);
#48615=ADVANCED_FACE('',(#13528),#11423,.F.);
#48616=ADVANCED_FACE('',(#13529),#11424,.F.);
#48617=ADVANCED_FACE('',(#13530),#11425,.F.);
#48618=ADVANCED_FACE('',(#13531),#11426,.F.);
#48619=ADVANCED_FACE('',(#13532),#11427,.F.);
#48620=ADVANCED_FACE('',(#13533),#11428,.F.);
#48621=ADVANCED_FACE('',(#13534),#11429,.F.);
#48622=ADVANCED_FACE('',(#13535),#11430,.F.);
#48623=ADVANCED_FACE('',(#13536),#11431,.F.);
#48624=ADVANCED_FACE('',(#13537),#11432,.T.);
#48625=ADVANCED_FACE('',(#13538),#11433,.T.);
#48626=ADVANCED_FACE('',(#13539),#11434,.T.);
#48627=ADVANCED_FACE('',(#13540),#11435,.T.);
#48628=ADVANCED_FACE('',(#13541),#11436,.T.);
#48629=ADVANCED_FACE('',(#13542),#11437,.T.);
#48630=ADVANCED_FACE('',(#13543),#11438,.T.);
#48631=ADVANCED_FACE('',(#13544),#11439,.T.);
#48632=ADVANCED_FACE('',(#13545),#11440,.T.);
#48633=ADVANCED_FACE('',(#13546),#11441,.T.);
#48634=ADVANCED_FACE('',(#13547),#11442,.T.);
#48635=ADVANCED_FACE('',(#13548),#11443,.T.);
#48636=ADVANCED_FACE('',(#13549),#11444,.T.);
#48637=ADVANCED_FACE('',(#13550),#11445,.T.);
#48638=ADVANCED_FACE('',(#13551),#11446,.T.);
#48639=ADVANCED_FACE('',(#13552),#11447,.T.);
#48640=ADVANCED_FACE('',(#13553),#11448,.T.);
#48641=ADVANCED_FACE('',(#13554),#11449,.T.);
#48642=ADVANCED_FACE('',(#13555),#11450,.T.);
#48643=ADVANCED_FACE('',(#13556),#11451,.T.);
#48644=ADVANCED_FACE('',(#13557),#11452,.T.);
#48645=ADVANCED_FACE('',(#13558),#11453,.T.);
#48646=ADVANCED_FACE('',(#13559),#11454,.T.);
#48647=ADVANCED_FACE('',(#13560),#11455,.T.);
#48648=ADVANCED_FACE('',(#13561),#11456,.T.);
#48649=ADVANCED_FACE('',(#13562),#11457,.T.);
#48650=ADVANCED_FACE('',(#13563),#11458,.T.);
#48651=ADVANCED_FACE('',(#13564),#11459,.T.);
#48652=ADVANCED_FACE('',(#13565),#11460,.T.);
#48653=ADVANCED_FACE('',(#13566),#11461,.T.);
#48654=ADVANCED_FACE('',(#13567),#11462,.T.);
#48655=ADVANCED_FACE('',(#13568),#11463,.T.);
#48656=ADVANCED_FACE('',(#13569),#11464,.T.);
#48657=ADVANCED_FACE('',(#13570),#11465,.T.);
#48658=ADVANCED_FACE('',(#13571),#11466,.T.);
#48659=ADVANCED_FACE('',(#13572),#11467,.T.);
#48660=ADVANCED_FACE('',(#13573),#11468,.T.);
#48661=ADVANCED_FACE('',(#13574),#11469,.T.);
#48662=ADVANCED_FACE('',(#13575),#11470,.T.);
#48663=ADVANCED_FACE('',(#13576),#11471,.T.);
#48664=ADVANCED_FACE('',(#13577),#11472,.T.);
#48665=ADVANCED_FACE('',(#13578),#11473,.T.);
#48666=ADVANCED_FACE('',(#13579),#11474,.T.);
#48667=ADVANCED_FACE('',(#13580),#11475,.T.);
#48668=ADVANCED_FACE('',(#13581),#11476,.T.);
#48669=ADVANCED_FACE('',(#13582),#11477,.T.);
#48670=ADVANCED_FACE('',(#13583),#11478,.T.);
#48671=ADVANCED_FACE('',(#13584),#11479,.T.);
#48672=ADVANCED_FACE('',(#13585),#11480,.T.);
#48673=ADVANCED_FACE('',(#13586),#11481,.T.);
#48674=ADVANCED_FACE('',(#13587),#11482,.T.);
#48675=ADVANCED_FACE('',(#13588),#11483,.T.);
#48676=ADVANCED_FACE('',(#13589),#11484,.T.);
#48677=ADVANCED_FACE('',(#13590),#11485,.T.);
#48678=ADVANCED_FACE('',(#13591),#11486,.T.);
#48679=ADVANCED_FACE('',(#13592),#11487,.T.);
#48680=ADVANCED_FACE('',(#13593),#11488,.T.);
#48681=ADVANCED_FACE('',(#13594),#11489,.T.);
#48682=ADVANCED_FACE('',(#13595),#11490,.T.);
#48683=ADVANCED_FACE('',(#13596),#11491,.T.);
#48684=ADVANCED_FACE('',(#13597),#11492,.T.);
#48685=ADVANCED_FACE('',(#13598),#11493,.T.);
#48686=ADVANCED_FACE('',(#13599),#11494,.T.);
#48687=ADVANCED_FACE('',(#13600),#11495,.T.);
#48688=ADVANCED_FACE('',(#13601),#48187,.F.);
#48689=ADVANCED_FACE('',(#13602),#1044,.F.);
#48690=ADVANCED_FACE('',(#13603),#11496,.T.);
#48691=ADVANCED_FACE('',(#13604),#11497,.T.);
#48692=ADVANCED_FACE('',(#13605),#11498,.T.);
#48693=ADVANCED_FACE('',(#13606),#11499,.T.);
#48694=ADVANCED_FACE('',(#13607),#11500,.T.);
#48695=ADVANCED_FACE('',(#13608),#11501,.T.);
#48696=ADVANCED_FACE('',(#13609),#11502,.T.);
#48697=ADVANCED_FACE('',(#13610),#11503,.T.);
#48698=ADVANCED_FACE('',(#13611),#11504,.T.);
#48699=ADVANCED_FACE('',(#13612),#11505,.T.);
#48700=ADVANCED_FACE('',(#13613),#11506,.T.);
#48701=ADVANCED_FACE('',(#13614),#11507,.T.);
#48702=ADVANCED_FACE('',(#13615),#11508,.T.);
#48703=ADVANCED_FACE('',(#13616),#11509,.T.);
#48704=ADVANCED_FACE('',(#13617),#11510,.T.);
#48705=ADVANCED_FACE('',(#13618),#11511,.T.);
#48706=ADVANCED_FACE('',(#13619),#11512,.T.);
#48707=ADVANCED_FACE('',(#13620),#11513,.T.);
#48708=ADVANCED_FACE('',(#13621),#11514,.T.);
#48709=ADVANCED_FACE('',(#13622),#11515,.T.);
#48710=ADVANCED_FACE('',(#13623),#11516,.T.);
#48711=ADVANCED_FACE('',(#13624),#11517,.T.);
#48712=ADVANCED_FACE('',(#13625),#11518,.T.);
#48713=ADVANCED_FACE('',(#13626),#11519,.T.);
#48714=ADVANCED_FACE('',(#13627),#11520,.T.);
#48715=ADVANCED_FACE('',(#13628),#11521,.T.);
#48716=ADVANCED_FACE('',(#13629),#11522,.T.);
#48717=ADVANCED_FACE('',(#13630),#11523,.T.);
#48718=ADVANCED_FACE('',(#13631),#1045,.F.);
#48719=ADVANCED_FACE('',(#13632),#11524,.T.);
#48720=ADVANCED_FACE('',(#13633),#11525,.T.);
#48721=ADVANCED_FACE('',(#13634),#11526,.T.);
#48722=ADVANCED_FACE('',(#13635),#11527,.T.);
#48723=ADVANCED_FACE('',(#13636),#11528,.T.);
#48724=ADVANCED_FACE('',(#13637),#11529,.T.);
#48725=ADVANCED_FACE('',(#13638),#11530,.T.);
#48726=ADVANCED_FACE('',(#13639),#11531,.T.);
#48727=ADVANCED_FACE('',(#13640),#11532,.T.);
#48728=ADVANCED_FACE('',(#13641),#11533,.T.);
#48729=ADVANCED_FACE('',(#13642),#11534,.T.);
#48730=ADVANCED_FACE('',(#13643),#11535,.T.);
#48731=ADVANCED_FACE('',(#13644),#11536,.T.);
#48732=ADVANCED_FACE('',(#13645),#11537,.T.);
#48733=ADVANCED_FACE('',(#13646),#11538,.T.);
#48734=ADVANCED_FACE('',(#13647),#11539,.T.);
#48735=ADVANCED_FACE('',(#13648),#11540,.T.);
#48736=ADVANCED_FACE('',(#13649),#11541,.T.);
#48737=ADVANCED_FACE('',(#13650),#11542,.T.);
#48738=ADVANCED_FACE('',(#13651),#11543,.T.);
#48739=ADVANCED_FACE('',(#13652),#11544,.T.);
#48740=ADVANCED_FACE('',(#13653),#11545,.T.);
#48741=ADVANCED_FACE('',(#13654),#11546,.T.);
#48742=ADVANCED_FACE('',(#13655),#11547,.T.);
#48743=ADVANCED_FACE('',(#13656),#11548,.T.);
#48744=ADVANCED_FACE('',(#13657),#11549,.T.);
#48745=ADVANCED_FACE('',(#13658),#11550,.T.);
#48746=ADVANCED_FACE('',(#13659),#11551,.T.);
#48747=ADVANCED_FACE('',(#13660),#1046,.F.);
#48748=ADVANCED_FACE('',(#13661),#11552,.T.);
#48749=ADVANCED_FACE('',(#13662),#11553,.T.);
#48750=ADVANCED_FACE('',(#13663),#11554,.T.);
#48751=ADVANCED_FACE('',(#13664),#11555,.T.);
#48752=ADVANCED_FACE('',(#13665),#11556,.T.);
#48753=ADVANCED_FACE('',(#13666),#11557,.T.);
#48754=ADVANCED_FACE('',(#13667),#11558,.T.);
#48755=ADVANCED_FACE('',(#13668),#11559,.T.);
#48756=ADVANCED_FACE('',(#13669),#11560,.T.);
#48757=ADVANCED_FACE('',(#13670),#11561,.T.);
#48758=ADVANCED_FACE('',(#13671),#11562,.T.);
#48759=ADVANCED_FACE('',(#13672),#11563,.T.);
#48760=ADVANCED_FACE('',(#13673),#11564,.T.);
#48761=ADVANCED_FACE('',(#13674),#11565,.T.);
#48762=ADVANCED_FACE('',(#13675),#11566,.T.);
#48763=ADVANCED_FACE('',(#13676),#11567,.T.);
#48764=ADVANCED_FACE('',(#13677),#11568,.T.);
#48765=ADVANCED_FACE('',(#13678),#11569,.T.);
#48766=ADVANCED_FACE('',(#13679),#11570,.T.);
#48767=ADVANCED_FACE('',(#13680),#11571,.T.);
#48768=ADVANCED_FACE('',(#13681),#11572,.T.);
#48769=ADVANCED_FACE('',(#13682),#11573,.T.);
#48770=ADVANCED_FACE('',(#13683),#11574,.T.);
#48771=ADVANCED_FACE('',(#13684),#11575,.T.);
#48772=ADVANCED_FACE('',(#13685),#11576,.T.);
#48773=ADVANCED_FACE('',(#13686),#11577,.T.);
#48774=ADVANCED_FACE('',(#13687),#11578,.T.);
#48775=ADVANCED_FACE('',(#13688),#11579,.T.);
#48776=ADVANCED_FACE('',(#13689),#1047,.F.);
#48777=ADVANCED_FACE('',(#13690),#11580,.T.);
#48778=ADVANCED_FACE('',(#13691),#11581,.T.);
#48779=ADVANCED_FACE('',(#13692),#11582,.T.);
#48780=ADVANCED_FACE('',(#13693),#11583,.T.);
#48781=ADVANCED_FACE('',(#13694),#11584,.T.);
#48782=ADVANCED_FACE('',(#13695),#11585,.T.);
#48783=ADVANCED_FACE('',(#13696),#11586,.T.);
#48784=ADVANCED_FACE('',(#13697),#11587,.T.);
#48785=ADVANCED_FACE('',(#13698),#11588,.T.);
#48786=ADVANCED_FACE('',(#13699),#11589,.T.);
#48787=ADVANCED_FACE('',(#13700),#11590,.T.);
#48788=ADVANCED_FACE('',(#13701),#11591,.T.);
#48789=ADVANCED_FACE('',(#13702),#11592,.T.);
#48790=ADVANCED_FACE('',(#13703),#11593,.T.);
#48791=ADVANCED_FACE('',(#13704),#11594,.T.);
#48792=ADVANCED_FACE('',(#13705),#11595,.T.);
#48793=ADVANCED_FACE('',(#13706),#11596,.T.);
#48794=ADVANCED_FACE('',(#13707),#11597,.T.);
#48795=ADVANCED_FACE('',(#13708),#11598,.T.);
#48796=ADVANCED_FACE('',(#13709),#11599,.T.);
#48797=ADVANCED_FACE('',(#13710),#11600,.T.);
#48798=ADVANCED_FACE('',(#13711),#11601,.T.);
#48799=ADVANCED_FACE('',(#13712),#11602,.T.);
#48800=ADVANCED_FACE('',(#13713),#11603,.T.);
#48801=ADVANCED_FACE('',(#13714),#11604,.T.);
#48802=ADVANCED_FACE('',(#13715),#11605,.T.);
#48803=ADVANCED_FACE('',(#13716),#11606,.T.);
#48804=ADVANCED_FACE('',(#13717),#11607,.T.);
#48805=ADVANCED_FACE('',(#13718),#1048,.F.);
#48806=ADVANCED_FACE('',(#13719),#11608,.T.);
#48807=ADVANCED_FACE('',(#13720),#11609,.T.);
#48808=ADVANCED_FACE('',(#13721),#11610,.T.);
#48809=ADVANCED_FACE('',(#13722),#11611,.T.);
#48810=ADVANCED_FACE('',(#13723),#11612,.T.);
#48811=ADVANCED_FACE('',(#13724),#11613,.T.);
#48812=ADVANCED_FACE('',(#13725),#11614,.T.);
#48813=ADVANCED_FACE('',(#13726),#11615,.T.);
#48814=ADVANCED_FACE('',(#13727),#11616,.T.);
#48815=ADVANCED_FACE('',(#13728),#11617,.T.);
#48816=ADVANCED_FACE('',(#13729),#11618,.T.);
#48817=ADVANCED_FACE('',(#13730),#11619,.T.);
#48818=ADVANCED_FACE('',(#13731),#11620,.T.);
#48819=ADVANCED_FACE('',(#13732),#11621,.T.);
#48820=ADVANCED_FACE('',(#13733),#11622,.T.);
#48821=ADVANCED_FACE('',(#13734),#11623,.T.);
#48822=ADVANCED_FACE('',(#13735),#11624,.T.);
#48823=ADVANCED_FACE('',(#13736),#11625,.T.);
#48824=ADVANCED_FACE('',(#13737),#11626,.T.);
#48825=ADVANCED_FACE('',(#13738),#11627,.T.);
#48826=ADVANCED_FACE('',(#13739),#11628,.T.);
#48827=ADVANCED_FACE('',(#13740),#11629,.T.);
#48828=ADVANCED_FACE('',(#13741),#11630,.T.);
#48829=ADVANCED_FACE('',(#13742),#11631,.T.);
#48830=ADVANCED_FACE('',(#13743),#11632,.T.);
#48831=ADVANCED_FACE('',(#13744),#11633,.T.);
#48832=ADVANCED_FACE('',(#13745),#11634,.T.);
#48833=ADVANCED_FACE('',(#13746),#11635,.T.);
#48834=ADVANCED_FACE('',(#13747),#1049,.F.);
#48835=ADVANCED_FACE('',(#13748),#11636,.T.);
#48836=ADVANCED_FACE('',(#13749),#11637,.T.);
#48837=ADVANCED_FACE('',(#13750),#11638,.T.);
#48838=ADVANCED_FACE('',(#13751),#11639,.T.);
#48839=ADVANCED_FACE('',(#13752),#11640,.T.);
#48840=ADVANCED_FACE('',(#13753),#11641,.T.);
#48841=ADVANCED_FACE('',(#13754),#11642,.T.);
#48842=ADVANCED_FACE('',(#13755),#11643,.T.);
#48843=ADVANCED_FACE('',(#13756),#11644,.T.);
#48844=ADVANCED_FACE('',(#13757),#11645,.T.);
#48845=ADVANCED_FACE('',(#13758),#11646,.T.);
#48846=ADVANCED_FACE('',(#13759),#11647,.T.);
#48847=ADVANCED_FACE('',(#13760),#11648,.T.);
#48848=ADVANCED_FACE('',(#13761),#11649,.T.);
#48849=ADVANCED_FACE('',(#13762),#11650,.T.);
#48850=ADVANCED_FACE('',(#13763),#11651,.T.);
#48851=ADVANCED_FACE('',(#13764),#11652,.T.);
#48852=ADVANCED_FACE('',(#13765),#11653,.T.);
#48853=ADVANCED_FACE('',(#13766),#11654,.T.);
#48854=ADVANCED_FACE('',(#13767),#11655,.T.);
#48855=ADVANCED_FACE('',(#13768),#11656,.T.);
#48856=ADVANCED_FACE('',(#13769),#11657,.T.);
#48857=ADVANCED_FACE('',(#13770),#11658,.T.);
#48858=ADVANCED_FACE('',(#13771),#11659,.T.);
#48859=ADVANCED_FACE('',(#13772),#11660,.T.);
#48860=ADVANCED_FACE('',(#13773),#11661,.T.);
#48861=ADVANCED_FACE('',(#13774),#11662,.T.);
#48862=ADVANCED_FACE('',(#13775),#11663,.T.);
#48863=ADVANCED_FACE('',(#13776),#1050,.F.);
#48864=ADVANCED_FACE('',(#13777),#11664,.T.);
#48865=ADVANCED_FACE('',(#13778),#11665,.T.);
#48866=ADVANCED_FACE('',(#13779),#11666,.T.);
#48867=ADVANCED_FACE('',(#13780),#11667,.T.);
#48868=ADVANCED_FACE('',(#13781),#11668,.T.);
#48869=ADVANCED_FACE('',(#13782),#11669,.T.);
#48870=ADVANCED_FACE('',(#13783),#11670,.T.);
#48871=ADVANCED_FACE('',(#13784),#11671,.T.);
#48872=ADVANCED_FACE('',(#13785),#11672,.T.);
#48873=ADVANCED_FACE('',(#13786),#11673,.T.);
#48874=ADVANCED_FACE('',(#13787),#11674,.T.);
#48875=ADVANCED_FACE('',(#13788),#11675,.T.);
#48876=ADVANCED_FACE('',(#13789),#11676,.T.);
#48877=ADVANCED_FACE('',(#13790),#11677,.T.);
#48878=ADVANCED_FACE('',(#13791),#11678,.T.);
#48879=ADVANCED_FACE('',(#13792),#11679,.T.);
#48880=ADVANCED_FACE('',(#13793),#11680,.T.);
#48881=ADVANCED_FACE('',(#13794),#11681,.T.);
#48882=ADVANCED_FACE('',(#13795),#11682,.T.);
#48883=ADVANCED_FACE('',(#13796),#11683,.T.);
#48884=ADVANCED_FACE('',(#13797),#11684,.T.);
#48885=ADVANCED_FACE('',(#13798),#11685,.T.);
#48886=ADVANCED_FACE('',(#13799),#11686,.T.);
#48887=ADVANCED_FACE('',(#13800),#11687,.T.);
#48888=ADVANCED_FACE('',(#13801),#11688,.T.);
#48889=ADVANCED_FACE('',(#13802),#11689,.T.);
#48890=ADVANCED_FACE('',(#13803),#11690,.T.);
#48891=ADVANCED_FACE('',(#13804),#11691,.T.);
#48892=ADVANCED_FACE('',(#13805),#1051,.F.);
#48893=ADVANCED_FACE('',(#13806),#11692,.T.);
#48894=ADVANCED_FACE('',(#13807),#11693,.T.);
#48895=ADVANCED_FACE('',(#13808),#11694,.T.);
#48896=ADVANCED_FACE('',(#13809),#11695,.T.);
#48897=ADVANCED_FACE('',(#13810),#11696,.T.);
#48898=ADVANCED_FACE('',(#13811),#11697,.T.);
#48899=ADVANCED_FACE('',(#13812),#11698,.T.);
#48900=ADVANCED_FACE('',(#13813),#11699,.T.);
#48901=ADVANCED_FACE('',(#13814),#11700,.T.);
#48902=ADVANCED_FACE('',(#13815),#11701,.T.);
#48903=ADVANCED_FACE('',(#13816),#11702,.T.);
#48904=ADVANCED_FACE('',(#13817),#11703,.T.);
#48905=ADVANCED_FACE('',(#13818),#11704,.T.);
#48906=ADVANCED_FACE('',(#13819),#11705,.T.);
#48907=ADVANCED_FACE('',(#13820),#11706,.T.);
#48908=ADVANCED_FACE('',(#13821),#11707,.T.);
#48909=ADVANCED_FACE('',(#13822),#11708,.T.);
#48910=ADVANCED_FACE('',(#13823),#11709,.T.);
#48911=ADVANCED_FACE('',(#13824),#11710,.T.);
#48912=ADVANCED_FACE('',(#13825),#11711,.T.);
#48913=ADVANCED_FACE('',(#13826),#11712,.T.);
#48914=ADVANCED_FACE('',(#13827),#11713,.T.);
#48915=ADVANCED_FACE('',(#13828),#11714,.T.);
#48916=ADVANCED_FACE('',(#13829),#11715,.T.);
#48917=ADVANCED_FACE('',(#13830),#11716,.T.);
#48918=ADVANCED_FACE('',(#13831),#11717,.T.);
#48919=ADVANCED_FACE('',(#13832),#11718,.T.);
#48920=ADVANCED_FACE('',(#13833),#11719,.T.);
#48921=ADVANCED_FACE('',(#13834),#1052,.F.);
#48922=ADVANCED_FACE('',(#13835),#11720,.T.);
#48923=ADVANCED_FACE('',(#13836),#11721,.T.);
#48924=ADVANCED_FACE('',(#13837),#11722,.T.);
#48925=ADVANCED_FACE('',(#13838),#11723,.T.);
#48926=ADVANCED_FACE('',(#13839),#11724,.T.);
#48927=ADVANCED_FACE('',(#13840),#11725,.T.);
#48928=ADVANCED_FACE('',(#13841),#11726,.T.);
#48929=ADVANCED_FACE('',(#13842),#11727,.T.);
#48930=ADVANCED_FACE('',(#13843),#11728,.T.);
#48931=ADVANCED_FACE('',(#13844),#11729,.T.);
#48932=ADVANCED_FACE('',(#13845),#11730,.T.);
#48933=ADVANCED_FACE('',(#13846),#11731,.T.);
#48934=ADVANCED_FACE('',(#13847),#11732,.T.);
#48935=ADVANCED_FACE('',(#13848),#11733,.T.);
#48936=ADVANCED_FACE('',(#13849),#11734,.T.);
#48937=ADVANCED_FACE('',(#13850),#11735,.T.);
#48938=ADVANCED_FACE('',(#13851),#11736,.T.);
#48939=ADVANCED_FACE('',(#13852),#11737,.T.);
#48940=ADVANCED_FACE('',(#13853),#11738,.T.);
#48941=ADVANCED_FACE('',(#13854),#11739,.T.);
#48942=ADVANCED_FACE('',(#13855),#11740,.T.);
#48943=ADVANCED_FACE('',(#13856),#11741,.T.);
#48944=ADVANCED_FACE('',(#13857),#11742,.T.);
#48945=ADVANCED_FACE('',(#13858),#11743,.T.);
#48946=ADVANCED_FACE('',(#13859),#11744,.T.);
#48947=ADVANCED_FACE('',(#13860),#11745,.T.);
#48948=ADVANCED_FACE('',(#13861),#11746,.T.);
#48949=ADVANCED_FACE('',(#13862),#11747,.T.);
#48950=ADVANCED_FACE('',(#13863),#1053,.F.);
#48951=ADVANCED_FACE('',(#13864),#11748,.T.);
#48952=ADVANCED_FACE('',(#13865),#11749,.T.);
#48953=ADVANCED_FACE('',(#13866),#11750,.T.);
#48954=ADVANCED_FACE('',(#13867),#11751,.T.);
#48955=ADVANCED_FACE('',(#13868),#11752,.T.);
#48956=ADVANCED_FACE('',(#13869),#11753,.T.);
#48957=ADVANCED_FACE('',(#13870),#11754,.T.);
#48958=ADVANCED_FACE('',(#13871),#11755,.T.);
#48959=ADVANCED_FACE('',(#13872),#11756,.T.);
#48960=ADVANCED_FACE('',(#13873),#11757,.T.);
#48961=ADVANCED_FACE('',(#13874),#11758,.T.);
#48962=ADVANCED_FACE('',(#13875),#11759,.T.);
#48963=ADVANCED_FACE('',(#13876),#11760,.T.);
#48964=ADVANCED_FACE('',(#13877),#11761,.T.);
#48965=ADVANCED_FACE('',(#13878),#11762,.T.);
#48966=ADVANCED_FACE('',(#13879),#11763,.T.);
#48967=ADVANCED_FACE('',(#13880),#11764,.T.);
#48968=ADVANCED_FACE('',(#13881),#11765,.T.);
#48969=ADVANCED_FACE('',(#13882),#11766,.T.);
#48970=ADVANCED_FACE('',(#13883),#11767,.T.);
#48971=ADVANCED_FACE('',(#13884),#11768,.T.);
#48972=ADVANCED_FACE('',(#13885),#11769,.T.);
#48973=ADVANCED_FACE('',(#13886),#11770,.T.);
#48974=ADVANCED_FACE('',(#13887),#11771,.T.);
#48975=ADVANCED_FACE('',(#13888),#11772,.T.);
#48976=ADVANCED_FACE('',(#13889),#11773,.T.);
#48977=ADVANCED_FACE('',(#13890),#11774,.T.);
#48978=ADVANCED_FACE('',(#13891),#11775,.T.);
#48979=ADVANCED_FACE('',(#13892),#1054,.F.);
#48980=ADVANCED_FACE('',(#13893),#11776,.T.);
#48981=ADVANCED_FACE('',(#13894),#11777,.T.);
#48982=ADVANCED_FACE('',(#13895),#11778,.T.);
#48983=ADVANCED_FACE('',(#13896),#11779,.T.);
#48984=ADVANCED_FACE('',(#13897),#11780,.T.);
#48985=ADVANCED_FACE('',(#13898),#11781,.T.);
#48986=ADVANCED_FACE('',(#13899),#11782,.T.);
#48987=ADVANCED_FACE('',(#13900),#11783,.T.);
#48988=ADVANCED_FACE('',(#13901),#11784,.T.);
#48989=ADVANCED_FACE('',(#13902),#11785,.T.);
#48990=ADVANCED_FACE('',(#13903),#11786,.T.);
#48991=ADVANCED_FACE('',(#13904),#11787,.T.);
#48992=ADVANCED_FACE('',(#13905),#11788,.T.);
#48993=ADVANCED_FACE('',(#13906),#11789,.T.);
#48994=ADVANCED_FACE('',(#13907),#11790,.T.);
#48995=ADVANCED_FACE('',(#13908),#11791,.T.);
#48996=ADVANCED_FACE('',(#13909),#11792,.T.);
#48997=ADVANCED_FACE('',(#13910),#11793,.T.);
#48998=ADVANCED_FACE('',(#13911),#11794,.T.);
#48999=ADVANCED_FACE('',(#13912),#11795,.T.);
#49000=ADVANCED_FACE('',(#13913),#11796,.T.);
#49001=ADVANCED_FACE('',(#13914),#11797,.T.);
#49002=ADVANCED_FACE('',(#13915),#11798,.T.);
#49003=ADVANCED_FACE('',(#13916),#11799,.T.);
#49004=ADVANCED_FACE('',(#13917),#11800,.T.);
#49005=ADVANCED_FACE('',(#13918),#11801,.T.);
#49006=ADVANCED_FACE('',(#13919),#11802,.T.);
#49007=ADVANCED_FACE('',(#13920),#11803,.T.);
#49008=ADVANCED_FACE('',(#13921),#1055,.F.);
#49009=ADVANCED_FACE('',(#13922),#11804,.T.);
#49010=ADVANCED_FACE('',(#13923),#11805,.T.);
#49011=ADVANCED_FACE('',(#13924),#11806,.T.);
#49012=ADVANCED_FACE('',(#13925),#11807,.T.);
#49013=ADVANCED_FACE('',(#13926),#11808,.T.);
#49014=ADVANCED_FACE('',(#13927),#11809,.T.);
#49015=ADVANCED_FACE('',(#13928),#11810,.T.);
#49016=ADVANCED_FACE('',(#13929),#11811,.T.);
#49017=ADVANCED_FACE('',(#13930),#11812,.T.);
#49018=ADVANCED_FACE('',(#13931),#11813,.T.);
#49019=ADVANCED_FACE('',(#13932),#11814,.T.);
#49020=ADVANCED_FACE('',(#13933),#11815,.T.);
#49021=ADVANCED_FACE('',(#13934),#11816,.T.);
#49022=ADVANCED_FACE('',(#13935),#11817,.T.);
#49023=ADVANCED_FACE('',(#13936),#11818,.T.);
#49024=ADVANCED_FACE('',(#13937),#11819,.T.);
#49025=ADVANCED_FACE('',(#13938),#11820,.T.);
#49026=ADVANCED_FACE('',(#13939),#11821,.T.);
#49027=ADVANCED_FACE('',(#13940),#11822,.T.);
#49028=ADVANCED_FACE('',(#13941),#11823,.T.);
#49029=ADVANCED_FACE('',(#13942),#11824,.T.);
#49030=ADVANCED_FACE('',(#13943),#11825,.T.);
#49031=ADVANCED_FACE('',(#13944),#11826,.T.);
#49032=ADVANCED_FACE('',(#13945),#11827,.T.);
#49033=ADVANCED_FACE('',(#13946),#11828,.T.);
#49034=ADVANCED_FACE('',(#13947),#11829,.T.);
#49035=ADVANCED_FACE('',(#13948),#11830,.T.);
#49036=ADVANCED_FACE('',(#13949),#11831,.T.);
#49037=ADVANCED_FACE('',(#13950),#1056,.F.);
#49038=ADVANCED_FACE('',(#13951),#11832,.T.);
#49039=ADVANCED_FACE('',(#13952),#11833,.T.);
#49040=ADVANCED_FACE('',(#13953),#11834,.T.);
#49041=ADVANCED_FACE('',(#13954),#11835,.T.);
#49042=ADVANCED_FACE('',(#13955),#11836,.T.);
#49043=ADVANCED_FACE('',(#13956),#11837,.T.);
#49044=ADVANCED_FACE('',(#13957),#11838,.T.);
#49045=ADVANCED_FACE('',(#13958),#11839,.T.);
#49046=ADVANCED_FACE('',(#13959),#11840,.T.);
#49047=ADVANCED_FACE('',(#13960),#11841,.T.);
#49048=ADVANCED_FACE('',(#13961),#11842,.T.);
#49049=ADVANCED_FACE('',(#13962),#11843,.T.);
#49050=ADVANCED_FACE('',(#13963),#11844,.T.);
#49051=ADVANCED_FACE('',(#13964),#11845,.T.);
#49052=ADVANCED_FACE('',(#13965),#11846,.T.);
#49053=ADVANCED_FACE('',(#13966),#11847,.T.);
#49054=ADVANCED_FACE('',(#13967),#11848,.T.);
#49055=ADVANCED_FACE('',(#13968),#11849,.T.);
#49056=ADVANCED_FACE('',(#13969),#11850,.T.);
#49057=ADVANCED_FACE('',(#13970),#11851,.T.);
#49058=ADVANCED_FACE('',(#13971),#11852,.T.);
#49059=ADVANCED_FACE('',(#13972),#11853,.T.);
#49060=ADVANCED_FACE('',(#13973),#11854,.T.);
#49061=ADVANCED_FACE('',(#13974),#11855,.T.);
#49062=ADVANCED_FACE('',(#13975),#11856,.T.);
#49063=ADVANCED_FACE('',(#13976),#11857,.T.);
#49064=ADVANCED_FACE('',(#13977),#11858,.T.);
#49065=ADVANCED_FACE('',(#13978),#11859,.T.);
#49066=ADVANCED_FACE('',(#13979),#1057,.F.);
#49067=ADVANCED_FACE('',(#13980),#11860,.T.);
#49068=ADVANCED_FACE('',(#13981),#11861,.T.);
#49069=ADVANCED_FACE('',(#13982),#11862,.T.);
#49070=ADVANCED_FACE('',(#13983),#11863,.T.);
#49071=ADVANCED_FACE('',(#13984),#11864,.T.);
#49072=ADVANCED_FACE('',(#13985),#11865,.T.);
#49073=ADVANCED_FACE('',(#13986),#11866,.T.);
#49074=ADVANCED_FACE('',(#13987),#11867,.T.);
#49075=ADVANCED_FACE('',(#13988),#11868,.T.);
#49076=ADVANCED_FACE('',(#13989),#11869,.T.);
#49077=ADVANCED_FACE('',(#13990),#11870,.T.);
#49078=ADVANCED_FACE('',(#13991),#11871,.T.);
#49079=ADVANCED_FACE('',(#13992),#11872,.T.);
#49080=ADVANCED_FACE('',(#13993),#11873,.T.);
#49081=ADVANCED_FACE('',(#13994),#11874,.T.);
#49082=ADVANCED_FACE('',(#13995),#11875,.T.);
#49083=ADVANCED_FACE('',(#13996),#11876,.T.);
#49084=ADVANCED_FACE('',(#13997),#11877,.T.);
#49085=ADVANCED_FACE('',(#13998),#11878,.T.);
#49086=ADVANCED_FACE('',(#13999),#11879,.T.);
#49087=ADVANCED_FACE('',(#14000),#11880,.T.);
#49088=ADVANCED_FACE('',(#14001),#11881,.T.);
#49089=ADVANCED_FACE('',(#14002),#11882,.T.);
#49090=ADVANCED_FACE('',(#14003),#11883,.T.);
#49091=ADVANCED_FACE('',(#14004),#11884,.T.);
#49092=ADVANCED_FACE('',(#14005),#11885,.T.);
#49093=ADVANCED_FACE('',(#14006),#11886,.T.);
#49094=ADVANCED_FACE('',(#14007),#11887,.T.);
#49095=ADVANCED_FACE('',(#14008),#1058,.F.);
#49096=ADVANCED_FACE('',(#14009),#11888,.T.);
#49097=ADVANCED_FACE('',(#14010),#11889,.T.);
#49098=ADVANCED_FACE('',(#14011),#11890,.T.);
#49099=ADVANCED_FACE('',(#14012),#11891,.T.);
#49100=ADVANCED_FACE('',(#14013),#11892,.T.);
#49101=ADVANCED_FACE('',(#14014),#11893,.T.);
#49102=ADVANCED_FACE('',(#14015),#11894,.T.);
#49103=ADVANCED_FACE('',(#14016),#11895,.T.);
#49104=ADVANCED_FACE('',(#14017),#11896,.T.);
#49105=ADVANCED_FACE('',(#14018),#11897,.T.);
#49106=ADVANCED_FACE('',(#14019),#11898,.T.);
#49107=ADVANCED_FACE('',(#14020),#11899,.T.);
#49108=ADVANCED_FACE('',(#14021),#11900,.T.);
#49109=ADVANCED_FACE('',(#14022),#11901,.T.);
#49110=ADVANCED_FACE('',(#14023),#11902,.T.);
#49111=ADVANCED_FACE('',(#14024),#11903,.T.);
#49112=ADVANCED_FACE('',(#14025),#11904,.T.);
#49113=ADVANCED_FACE('',(#14026),#11905,.T.);
#49114=ADVANCED_FACE('',(#14027),#11906,.T.);
#49115=ADVANCED_FACE('',(#14028),#11907,.T.);
#49116=ADVANCED_FACE('',(#14029),#11908,.T.);
#49117=ADVANCED_FACE('',(#14030),#11909,.T.);
#49118=ADVANCED_FACE('',(#14031),#11910,.T.);
#49119=ADVANCED_FACE('',(#14032),#11911,.T.);
#49120=ADVANCED_FACE('',(#14033),#11912,.T.);
#49121=ADVANCED_FACE('',(#14034),#11913,.T.);
#49122=ADVANCED_FACE('',(#14035),#11914,.T.);
#49123=ADVANCED_FACE('',(#14036),#11915,.T.);
#49124=ADVANCED_FACE('',(#14037),#1059,.F.);
#49125=ADVANCED_FACE('',(#14038),#11916,.T.);
#49126=ADVANCED_FACE('',(#14039),#11917,.T.);
#49127=ADVANCED_FACE('',(#14040),#11918,.T.);
#49128=ADVANCED_FACE('',(#14041),#11919,.T.);
#49129=ADVANCED_FACE('',(#14042),#11920,.T.);
#49130=ADVANCED_FACE('',(#14043),#11921,.T.);
#49131=ADVANCED_FACE('',(#14044),#11922,.T.);
#49132=ADVANCED_FACE('',(#14045),#11923,.T.);
#49133=ADVANCED_FACE('',(#14046),#11924,.T.);
#49134=ADVANCED_FACE('',(#14047),#11925,.T.);
#49135=ADVANCED_FACE('',(#14048),#11926,.T.);
#49136=ADVANCED_FACE('',(#14049),#11927,.T.);
#49137=ADVANCED_FACE('',(#14050),#11928,.T.);
#49138=ADVANCED_FACE('',(#14051),#11929,.T.);
#49139=ADVANCED_FACE('',(#14052),#11930,.T.);
#49140=ADVANCED_FACE('',(#14053),#11931,.T.);
#49141=ADVANCED_FACE('',(#14054),#11932,.T.);
#49142=ADVANCED_FACE('',(#14055),#11933,.T.);
#49143=ADVANCED_FACE('',(#14056),#11934,.T.);
#49144=ADVANCED_FACE('',(#14057),#11935,.T.);
#49145=ADVANCED_FACE('',(#14058),#11936,.T.);
#49146=ADVANCED_FACE('',(#14059),#11937,.T.);
#49147=ADVANCED_FACE('',(#14060),#11938,.T.);
#49148=ADVANCED_FACE('',(#14061),#11939,.T.);
#49149=ADVANCED_FACE('',(#14062),#11940,.T.);
#49150=ADVANCED_FACE('',(#14063),#11941,.T.);
#49151=ADVANCED_FACE('',(#14064),#11942,.T.);
#49152=ADVANCED_FACE('',(#14065),#11943,.T.);
#49153=ADVANCED_FACE('',(#14066),#1060,.F.);
#49154=ADVANCED_FACE('',(#14067),#11944,.T.);
#49155=ADVANCED_FACE('',(#14068),#11945,.T.);
#49156=ADVANCED_FACE('',(#14069),#11946,.T.);
#49157=ADVANCED_FACE('',(#14070),#11947,.T.);
#49158=ADVANCED_FACE('',(#14071),#11948,.T.);
#49159=ADVANCED_FACE('',(#14072),#11949,.T.);
#49160=ADVANCED_FACE('',(#14073),#11950,.T.);
#49161=ADVANCED_FACE('',(#14074),#11951,.T.);
#49162=ADVANCED_FACE('',(#14075),#11952,.T.);
#49163=ADVANCED_FACE('',(#14076),#11953,.T.);
#49164=ADVANCED_FACE('',(#14077),#11954,.T.);
#49165=ADVANCED_FACE('',(#14078),#11955,.T.);
#49166=ADVANCED_FACE('',(#14079),#11956,.T.);
#49167=ADVANCED_FACE('',(#14080),#11957,.T.);
#49168=ADVANCED_FACE('',(#14081),#11958,.T.);
#49169=ADVANCED_FACE('',(#14082),#11959,.T.);
#49170=ADVANCED_FACE('',(#14083),#11960,.T.);
#49171=ADVANCED_FACE('',(#14084),#11961,.T.);
#49172=ADVANCED_FACE('',(#14085),#11962,.T.);
#49173=ADVANCED_FACE('',(#14086),#11963,.T.);
#49174=ADVANCED_FACE('',(#14087),#11964,.T.);
#49175=ADVANCED_FACE('',(#14088),#11965,.T.);
#49176=ADVANCED_FACE('',(#14089),#11966,.T.);
#49177=ADVANCED_FACE('',(#14090),#11967,.T.);
#49178=ADVANCED_FACE('',(#14091),#11968,.T.);
#49179=ADVANCED_FACE('',(#14092),#11969,.T.);
#49180=ADVANCED_FACE('',(#14093),#11970,.T.);
#49181=ADVANCED_FACE('',(#14094),#11971,.T.);
#49182=ADVANCED_FACE('',(#14095),#1061,.F.);
#49183=ADVANCED_FACE('',(#14096),#11972,.T.);
#49184=ADVANCED_FACE('',(#14097),#11973,.T.);
#49185=ADVANCED_FACE('',(#14098),#11974,.T.);
#49186=ADVANCED_FACE('',(#14099),#11975,.T.);
#49187=ADVANCED_FACE('',(#14100),#11976,.T.);
#49188=ADVANCED_FACE('',(#14101),#11977,.T.);
#49189=ADVANCED_FACE('',(#14102),#11978,.T.);
#49190=ADVANCED_FACE('',(#14103),#11979,.T.);
#49191=ADVANCED_FACE('',(#14104),#11980,.T.);
#49192=ADVANCED_FACE('',(#14105),#11981,.T.);
#49193=ADVANCED_FACE('',(#14106),#11982,.T.);
#49194=ADVANCED_FACE('',(#14107),#11983,.T.);
#49195=ADVANCED_FACE('',(#14108),#11984,.T.);
#49196=ADVANCED_FACE('',(#14109),#11985,.T.);
#49197=ADVANCED_FACE('',(#14110),#11986,.T.);
#49198=ADVANCED_FACE('',(#14111),#11987,.T.);
#49199=ADVANCED_FACE('',(#14112),#11988,.T.);
#49200=ADVANCED_FACE('',(#14113),#11989,.T.);
#49201=ADVANCED_FACE('',(#14114),#11990,.T.);
#49202=ADVANCED_FACE('',(#14115),#11991,.T.);
#49203=ADVANCED_FACE('',(#14116),#11992,.T.);
#49204=ADVANCED_FACE('',(#14117),#11993,.T.);
#49205=ADVANCED_FACE('',(#14118),#11994,.T.);
#49206=ADVANCED_FACE('',(#14119),#11995,.T.);
#49207=ADVANCED_FACE('',(#14120),#11996,.T.);
#49208=ADVANCED_FACE('',(#14121),#11997,.T.);
#49209=ADVANCED_FACE('',(#14122),#11998,.T.);
#49210=ADVANCED_FACE('',(#14123),#11999,.T.);
#49211=ADVANCED_FACE('',(#14124),#1062,.F.);
#49212=ADVANCED_FACE('',(#14125),#12000,.T.);
#49213=ADVANCED_FACE('',(#14126),#12001,.T.);
#49214=ADVANCED_FACE('',(#14127),#12002,.T.);
#49215=ADVANCED_FACE('',(#14128),#12003,.T.);
#49216=ADVANCED_FACE('',(#14129),#12004,.T.);
#49217=ADVANCED_FACE('',(#14130),#12005,.T.);
#49218=ADVANCED_FACE('',(#14131),#12006,.T.);
#49219=ADVANCED_FACE('',(#14132),#12007,.T.);
#49220=ADVANCED_FACE('',(#14133),#12008,.T.);
#49221=ADVANCED_FACE('',(#14134),#12009,.T.);
#49222=ADVANCED_FACE('',(#14135),#12010,.T.);
#49223=ADVANCED_FACE('',(#14136),#12011,.T.);
#49224=ADVANCED_FACE('',(#14137),#12012,.T.);
#49225=ADVANCED_FACE('',(#14138),#12013,.T.);
#49226=ADVANCED_FACE('',(#14139),#12014,.T.);
#49227=ADVANCED_FACE('',(#14140),#12015,.T.);
#49228=ADVANCED_FACE('',(#14141),#12016,.T.);
#49229=ADVANCED_FACE('',(#14142),#12017,.T.);
#49230=ADVANCED_FACE('',(#14143),#12018,.T.);
#49231=ADVANCED_FACE('',(#14144),#12019,.T.);
#49232=ADVANCED_FACE('',(#14145),#12020,.T.);
#49233=ADVANCED_FACE('',(#14146),#12021,.T.);
#49234=ADVANCED_FACE('',(#14147),#12022,.T.);
#49235=ADVANCED_FACE('',(#14148),#12023,.T.);
#49236=ADVANCED_FACE('',(#14149),#12024,.T.);
#49237=ADVANCED_FACE('',(#14150),#12025,.T.);
#49238=ADVANCED_FACE('',(#14151),#12026,.T.);
#49239=ADVANCED_FACE('',(#14152),#12027,.T.);
#49240=ADVANCED_FACE('',(#14153),#1063,.F.);
#49241=ADVANCED_FACE('',(#14154),#12028,.T.);
#49242=ADVANCED_FACE('',(#14155),#12029,.T.);
#49243=ADVANCED_FACE('',(#14156),#12030,.T.);
#49244=ADVANCED_FACE('',(#14157),#12031,.T.);
#49245=ADVANCED_FACE('',(#14158),#12032,.T.);
#49246=ADVANCED_FACE('',(#14159),#12033,.T.);
#49247=ADVANCED_FACE('',(#14160),#12034,.T.);
#49248=ADVANCED_FACE('',(#14161),#12035,.T.);
#49249=ADVANCED_FACE('',(#14162),#12036,.T.);
#49250=ADVANCED_FACE('',(#14163),#12037,.T.);
#49251=ADVANCED_FACE('',(#14164),#12038,.T.);
#49252=ADVANCED_FACE('',(#14165),#12039,.T.);
#49253=ADVANCED_FACE('',(#14166),#12040,.T.);
#49254=ADVANCED_FACE('',(#14167),#12041,.T.);
#49255=ADVANCED_FACE('',(#14168),#12042,.T.);
#49256=ADVANCED_FACE('',(#14169),#12043,.T.);
#49257=ADVANCED_FACE('',(#14170),#12044,.T.);
#49258=ADVANCED_FACE('',(#14171),#12045,.T.);
#49259=ADVANCED_FACE('',(#14172),#12046,.T.);
#49260=ADVANCED_FACE('',(#14173),#12047,.T.);
#49261=ADVANCED_FACE('',(#14174),#12048,.T.);
#49262=ADVANCED_FACE('',(#14175),#12049,.T.);
#49263=ADVANCED_FACE('',(#14176),#12050,.T.);
#49264=ADVANCED_FACE('',(#14177),#12051,.T.);
#49265=ADVANCED_FACE('',(#14178),#12052,.T.);
#49266=ADVANCED_FACE('',(#14179),#12053,.T.);
#49267=ADVANCED_FACE('',(#14180),#12054,.T.);
#49268=ADVANCED_FACE('',(#14181),#12055,.T.);
#49269=ADVANCED_FACE('',(#14182),#1064,.F.);
#49270=ADVANCED_FACE('',(#14183),#12056,.T.);
#49271=ADVANCED_FACE('',(#14184),#12057,.T.);
#49272=ADVANCED_FACE('',(#14185),#12058,.T.);
#49273=ADVANCED_FACE('',(#14186),#12059,.T.);
#49274=ADVANCED_FACE('',(#14187),#12060,.T.);
#49275=ADVANCED_FACE('',(#14188),#12061,.T.);
#49276=ADVANCED_FACE('',(#14189),#12062,.T.);
#49277=ADVANCED_FACE('',(#14190),#12063,.T.);
#49278=ADVANCED_FACE('',(#14191),#12064,.T.);
#49279=ADVANCED_FACE('',(#14192),#12065,.T.);
#49280=ADVANCED_FACE('',(#14193),#12066,.T.);
#49281=ADVANCED_FACE('',(#14194),#12067,.T.);
#49282=ADVANCED_FACE('',(#14195),#12068,.T.);
#49283=ADVANCED_FACE('',(#14196),#12069,.T.);
#49284=ADVANCED_FACE('',(#14197),#12070,.T.);
#49285=ADVANCED_FACE('',(#14198),#12071,.T.);
#49286=ADVANCED_FACE('',(#14199),#12072,.T.);
#49287=ADVANCED_FACE('',(#14200),#12073,.T.);
#49288=ADVANCED_FACE('',(#14201),#12074,.T.);
#49289=ADVANCED_FACE('',(#14202),#12075,.T.);
#49290=ADVANCED_FACE('',(#14203),#12076,.T.);
#49291=ADVANCED_FACE('',(#14204),#12077,.T.);
#49292=ADVANCED_FACE('',(#14205),#12078,.T.);
#49293=ADVANCED_FACE('',(#14206),#12079,.T.);
#49294=ADVANCED_FACE('',(#14207),#12080,.T.);
#49295=ADVANCED_FACE('',(#14208),#12081,.T.);
#49296=ADVANCED_FACE('',(#14209),#12082,.T.);
#49297=ADVANCED_FACE('',(#14210),#12083,.T.);
#49298=ADVANCED_FACE('',(#14211),#1065,.F.);
#49299=ADVANCED_FACE('',(#14212),#12084,.T.);
#49300=ADVANCED_FACE('',(#14213),#12085,.T.);
#49301=ADVANCED_FACE('',(#14214),#12086,.T.);
#49302=ADVANCED_FACE('',(#14215),#12087,.T.);
#49303=ADVANCED_FACE('',(#14216),#12088,.T.);
#49304=ADVANCED_FACE('',(#14217),#12089,.T.);
#49305=ADVANCED_FACE('',(#14218),#12090,.T.);
#49306=ADVANCED_FACE('',(#14219),#12091,.T.);
#49307=ADVANCED_FACE('',(#14220),#12092,.T.);
#49308=ADVANCED_FACE('',(#14221),#12093,.T.);
#49309=ADVANCED_FACE('',(#14222),#12094,.T.);
#49310=ADVANCED_FACE('',(#14223),#12095,.T.);
#49311=ADVANCED_FACE('',(#14224),#12096,.T.);
#49312=ADVANCED_FACE('',(#14225),#12097,.T.);
#49313=ADVANCED_FACE('',(#14226),#12098,.T.);
#49314=ADVANCED_FACE('',(#14227),#12099,.T.);
#49315=ADVANCED_FACE('',(#14228),#12100,.T.);
#49316=ADVANCED_FACE('',(#14229),#12101,.T.);
#49317=ADVANCED_FACE('',(#14230),#12102,.T.);
#49318=ADVANCED_FACE('',(#14231),#12103,.T.);
#49319=ADVANCED_FACE('',(#14232),#12104,.T.);
#49320=ADVANCED_FACE('',(#14233),#12105,.T.);
#49321=ADVANCED_FACE('',(#14234),#12106,.T.);
#49322=ADVANCED_FACE('',(#14235),#12107,.T.);
#49323=ADVANCED_FACE('',(#14236),#12108,.T.);
#49324=ADVANCED_FACE('',(#14237),#12109,.T.);
#49325=ADVANCED_FACE('',(#14238),#12110,.T.);
#49326=ADVANCED_FACE('',(#14239),#12111,.T.);
#49327=ADVANCED_FACE('',(#14240),#1066,.F.);
#49328=ADVANCED_FACE('',(#14241),#12112,.T.);
#49329=ADVANCED_FACE('',(#14242),#12113,.T.);
#49330=ADVANCED_FACE('',(#14243),#12114,.T.);
#49331=ADVANCED_FACE('',(#14244),#12115,.T.);
#49332=ADVANCED_FACE('',(#14245),#12116,.T.);
#49333=ADVANCED_FACE('',(#14246),#12117,.T.);
#49334=ADVANCED_FACE('',(#14247),#12118,.T.);
#49335=ADVANCED_FACE('',(#14248),#12119,.T.);
#49336=ADVANCED_FACE('',(#14249),#12120,.T.);
#49337=ADVANCED_FACE('',(#14250),#12121,.T.);
#49338=ADVANCED_FACE('',(#14251),#12122,.T.);
#49339=ADVANCED_FACE('',(#14252),#12123,.T.);
#49340=ADVANCED_FACE('',(#14253),#12124,.T.);
#49341=ADVANCED_FACE('',(#14254),#12125,.T.);
#49342=ADVANCED_FACE('',(#14255),#12126,.T.);
#49343=ADVANCED_FACE('',(#14256),#12127,.T.);
#49344=ADVANCED_FACE('',(#14257),#12128,.T.);
#49345=ADVANCED_FACE('',(#14258),#12129,.T.);
#49346=ADVANCED_FACE('',(#14259),#12130,.T.);
#49347=ADVANCED_FACE('',(#14260),#12131,.T.);
#49348=ADVANCED_FACE('',(#14261),#12132,.T.);
#49349=ADVANCED_FACE('',(#14262),#12133,.T.);
#49350=ADVANCED_FACE('',(#14263),#12134,.T.);
#49351=ADVANCED_FACE('',(#14264),#12135,.T.);
#49352=ADVANCED_FACE('',(#14265),#12136,.T.);
#49353=ADVANCED_FACE('',(#14266),#12137,.T.);
#49354=ADVANCED_FACE('',(#14267),#12138,.T.);
#49355=ADVANCED_FACE('',(#14268),#12139,.T.);
#49356=ADVANCED_FACE('',(#14269),#1067,.F.);
#49357=ADVANCED_FACE('',(#14270),#12140,.T.);
#49358=ADVANCED_FACE('',(#14271),#12141,.T.);
#49359=ADVANCED_FACE('',(#14272),#12142,.T.);
#49360=ADVANCED_FACE('',(#14273),#12143,.T.);
#49361=ADVANCED_FACE('',(#14274),#12144,.T.);
#49362=ADVANCED_FACE('',(#14275),#12145,.T.);
#49363=ADVANCED_FACE('',(#14276),#12146,.T.);
#49364=ADVANCED_FACE('',(#14277),#12147,.T.);
#49365=ADVANCED_FACE('',(#14278),#12148,.T.);
#49366=ADVANCED_FACE('',(#14279),#12149,.T.);
#49367=ADVANCED_FACE('',(#14280),#12150,.T.);
#49368=ADVANCED_FACE('',(#14281),#12151,.T.);
#49369=ADVANCED_FACE('',(#14282),#12152,.T.);
#49370=ADVANCED_FACE('',(#14283),#12153,.T.);
#49371=ADVANCED_FACE('',(#14284),#12154,.T.);
#49372=ADVANCED_FACE('',(#14285),#12155,.T.);
#49373=ADVANCED_FACE('',(#14286),#12156,.T.);
#49374=ADVANCED_FACE('',(#14287),#12157,.T.);
#49375=ADVANCED_FACE('',(#14288),#12158,.T.);
#49376=ADVANCED_FACE('',(#14289),#12159,.T.);
#49377=ADVANCED_FACE('',(#14290),#12160,.T.);
#49378=ADVANCED_FACE('',(#14291),#12161,.T.);
#49379=ADVANCED_FACE('',(#14292),#12162,.T.);
#49380=ADVANCED_FACE('',(#14293),#12163,.T.);
#49381=ADVANCED_FACE('',(#14294),#12164,.T.);
#49382=ADVANCED_FACE('',(#14295),#12165,.T.);
#49383=ADVANCED_FACE('',(#14296),#12166,.T.);
#49384=ADVANCED_FACE('',(#14297),#12167,.T.);
#49385=ADVANCED_FACE('',(#14298),#1068,.F.);
#49386=ADVANCED_FACE('',(#14299),#12168,.T.);
#49387=ADVANCED_FACE('',(#14300),#12169,.T.);
#49388=ADVANCED_FACE('',(#14301),#12170,.T.);
#49389=ADVANCED_FACE('',(#14302),#12171,.T.);
#49390=ADVANCED_FACE('',(#14303),#12172,.T.);
#49391=ADVANCED_FACE('',(#14304),#12173,.T.);
#49392=ADVANCED_FACE('',(#14305),#12174,.T.);
#49393=ADVANCED_FACE('',(#14306),#12175,.T.);
#49394=ADVANCED_FACE('',(#14307),#12176,.T.);
#49395=ADVANCED_FACE('',(#14308),#12177,.T.);
#49396=ADVANCED_FACE('',(#14309),#12178,.T.);
#49397=ADVANCED_FACE('',(#14310),#12179,.T.);
#49398=ADVANCED_FACE('',(#14311),#12180,.T.);
#49399=ADVANCED_FACE('',(#14312),#12181,.T.);
#49400=ADVANCED_FACE('',(#14313),#12182,.T.);
#49401=ADVANCED_FACE('',(#14314),#12183,.T.);
#49402=ADVANCED_FACE('',(#14315),#12184,.T.);
#49403=ADVANCED_FACE('',(#14316),#12185,.T.);
#49404=ADVANCED_FACE('',(#14317),#12186,.T.);
#49405=ADVANCED_FACE('',(#14318),#12187,.T.);
#49406=ADVANCED_FACE('',(#14319),#12188,.T.);
#49407=ADVANCED_FACE('',(#14320),#12189,.T.);
#49408=ADVANCED_FACE('',(#14321),#12190,.T.);
#49409=ADVANCED_FACE('',(#14322),#12191,.T.);
#49410=ADVANCED_FACE('',(#14323),#12192,.T.);
#49411=ADVANCED_FACE('',(#14324),#12193,.T.);
#49412=ADVANCED_FACE('',(#14325),#12194,.T.);
#49413=ADVANCED_FACE('',(#14326),#12195,.T.);
#49414=ADVANCED_FACE('',(#14327),#1069,.F.);
#49415=ADVANCED_FACE('',(#14328),#12196,.T.);
#49416=ADVANCED_FACE('',(#14329),#12197,.T.);
#49417=ADVANCED_FACE('',(#14330),#12198,.T.);
#49418=ADVANCED_FACE('',(#14331),#12199,.T.);
#49419=ADVANCED_FACE('',(#14332),#12200,.T.);
#49420=ADVANCED_FACE('',(#14333),#12201,.T.);
#49421=ADVANCED_FACE('',(#14334),#12202,.T.);
#49422=ADVANCED_FACE('',(#14335),#12203,.T.);
#49423=ADVANCED_FACE('',(#14336),#12204,.T.);
#49424=ADVANCED_FACE('',(#14337),#12205,.T.);
#49425=ADVANCED_FACE('',(#14338),#12206,.T.);
#49426=ADVANCED_FACE('',(#14339),#12207,.T.);
#49427=ADVANCED_FACE('',(#14340),#12208,.T.);
#49428=ADVANCED_FACE('',(#14341),#12209,.T.);
#49429=ADVANCED_FACE('',(#14342),#12210,.T.);
#49430=ADVANCED_FACE('',(#14343),#12211,.T.);
#49431=ADVANCED_FACE('',(#14344),#12212,.T.);
#49432=ADVANCED_FACE('',(#14345),#12213,.T.);
#49433=ADVANCED_FACE('',(#14346),#12214,.T.);
#49434=ADVANCED_FACE('',(#14347),#12215,.T.);
#49435=ADVANCED_FACE('',(#14348),#12216,.T.);
#49436=ADVANCED_FACE('',(#14349),#12217,.T.);
#49437=ADVANCED_FACE('',(#14350),#12218,.T.);
#49438=ADVANCED_FACE('',(#14351),#12219,.T.);
#49439=ADVANCED_FACE('',(#14352),#12220,.T.);
#49440=ADVANCED_FACE('',(#14353),#12221,.T.);
#49441=ADVANCED_FACE('',(#14354),#12222,.T.);
#49442=ADVANCED_FACE('',(#14355),#12223,.T.);
#49443=ADVANCED_FACE('',(#14356),#1070,.F.);
#49444=ADVANCED_FACE('',(#14357),#12224,.T.);
#49445=ADVANCED_FACE('',(#14358),#12225,.T.);
#49446=ADVANCED_FACE('',(#14359),#12226,.T.);
#49447=ADVANCED_FACE('',(#14360),#12227,.T.);
#49448=ADVANCED_FACE('',(#14361),#12228,.T.);
#49449=ADVANCED_FACE('',(#14362),#12229,.T.);
#49450=ADVANCED_FACE('',(#14363),#12230,.T.);
#49451=ADVANCED_FACE('',(#14364),#12231,.T.);
#49452=ADVANCED_FACE('',(#14365),#12232,.T.);
#49453=ADVANCED_FACE('',(#14366),#12233,.T.);
#49454=ADVANCED_FACE('',(#14367),#12234,.T.);
#49455=ADVANCED_FACE('',(#14368),#12235,.T.);
#49456=ADVANCED_FACE('',(#14369),#12236,.T.);
#49457=ADVANCED_FACE('',(#14370),#12237,.T.);
#49458=ADVANCED_FACE('',(#14371),#12238,.T.);
#49459=ADVANCED_FACE('',(#14372),#12239,.T.);
#49460=ADVANCED_FACE('',(#14373),#12240,.T.);
#49461=ADVANCED_FACE('',(#14374),#12241,.T.);
#49462=ADVANCED_FACE('',(#14375),#12242,.T.);
#49463=ADVANCED_FACE('',(#14376),#12243,.T.);
#49464=ADVANCED_FACE('',(#14377),#12244,.T.);
#49465=ADVANCED_FACE('',(#14378),#12245,.T.);
#49466=ADVANCED_FACE('',(#14379),#12246,.T.);
#49467=ADVANCED_FACE('',(#14380),#12247,.T.);
#49468=ADVANCED_FACE('',(#14381),#12248,.T.);
#49469=ADVANCED_FACE('',(#14382),#12249,.T.);
#49470=ADVANCED_FACE('',(#14383),#12250,.T.);
#49471=ADVANCED_FACE('',(#14384),#12251,.T.);
#49472=ADVANCED_FACE('',(#14385),#1071,.F.);
#49473=ADVANCED_FACE('',(#14386),#12252,.T.);
#49474=ADVANCED_FACE('',(#14387),#12253,.T.);
#49475=ADVANCED_FACE('',(#14388),#12254,.T.);
#49476=ADVANCED_FACE('',(#14389),#12255,.T.);
#49477=ADVANCED_FACE('',(#14390),#12256,.T.);
#49478=ADVANCED_FACE('',(#14391),#12257,.T.);
#49479=ADVANCED_FACE('',(#14392),#12258,.T.);
#49480=ADVANCED_FACE('',(#14393),#12259,.T.);
#49481=ADVANCED_FACE('',(#14394),#12260,.T.);
#49482=ADVANCED_FACE('',(#14395),#12261,.T.);
#49483=ADVANCED_FACE('',(#14396),#12262,.T.);
#49484=ADVANCED_FACE('',(#14397),#12263,.T.);
#49485=ADVANCED_FACE('',(#14398),#12264,.T.);
#49486=ADVANCED_FACE('',(#14399),#12265,.T.);
#49487=ADVANCED_FACE('',(#14400),#12266,.T.);
#49488=ADVANCED_FACE('',(#14401),#12267,.T.);
#49489=ADVANCED_FACE('',(#14402),#12268,.T.);
#49490=ADVANCED_FACE('',(#14403),#12269,.T.);
#49491=ADVANCED_FACE('',(#14404),#12270,.T.);
#49492=ADVANCED_FACE('',(#14405),#12271,.T.);
#49493=ADVANCED_FACE('',(#14406),#12272,.T.);
#49494=ADVANCED_FACE('',(#14407),#12273,.T.);
#49495=ADVANCED_FACE('',(#14408),#12274,.T.);
#49496=ADVANCED_FACE('',(#14409),#12275,.T.);
#49497=ADVANCED_FACE('',(#14410),#12276,.T.);
#49498=ADVANCED_FACE('',(#14411),#12277,.T.);
#49499=ADVANCED_FACE('',(#14412),#12278,.T.);
#49500=ADVANCED_FACE('',(#14413),#12279,.T.);
#49501=ADVANCED_FACE('',(#14414),#1072,.F.);
#49502=ADVANCED_FACE('',(#14415),#12280,.T.);
#49503=ADVANCED_FACE('',(#14416),#12281,.T.);
#49504=ADVANCED_FACE('',(#14417),#12282,.T.);
#49505=ADVANCED_FACE('',(#14418),#12283,.T.);
#49506=ADVANCED_FACE('',(#14419),#12284,.T.);
#49507=ADVANCED_FACE('',(#14420),#12285,.T.);
#49508=ADVANCED_FACE('',(#14421),#12286,.T.);
#49509=ADVANCED_FACE('',(#14422),#12287,.T.);
#49510=ADVANCED_FACE('',(#14423),#12288,.T.);
#49511=ADVANCED_FACE('',(#14424),#12289,.T.);
#49512=ADVANCED_FACE('',(#14425),#12290,.T.);
#49513=ADVANCED_FACE('',(#14426),#12291,.T.);
#49514=ADVANCED_FACE('',(#14427),#12292,.T.);
#49515=ADVANCED_FACE('',(#14428),#12293,.T.);
#49516=ADVANCED_FACE('',(#14429),#12294,.T.);
#49517=ADVANCED_FACE('',(#14430),#12295,.T.);
#49518=ADVANCED_FACE('',(#14431),#12296,.T.);
#49519=ADVANCED_FACE('',(#14432),#12297,.T.);
#49520=ADVANCED_FACE('',(#14433),#12298,.T.);
#49521=ADVANCED_FACE('',(#14434),#12299,.T.);
#49522=ADVANCED_FACE('',(#14435),#12300,.T.);
#49523=ADVANCED_FACE('',(#14436),#12301,.T.);
#49524=ADVANCED_FACE('',(#14437),#12302,.T.);
#49525=ADVANCED_FACE('',(#14438),#12303,.T.);
#49526=ADVANCED_FACE('',(#14439),#12304,.T.);
#49527=ADVANCED_FACE('',(#14440),#12305,.T.);
#49528=ADVANCED_FACE('',(#14441),#12306,.T.);
#49529=ADVANCED_FACE('',(#14442),#12307,.T.);
#49530=ADVANCED_FACE('',(#14443),#1073,.F.);
#49531=ADVANCED_FACE('',(#14444),#12308,.T.);
#49532=ADVANCED_FACE('',(#14445),#12309,.T.);
#49533=ADVANCED_FACE('',(#14446),#12310,.T.);
#49534=ADVANCED_FACE('',(#14447),#12311,.T.);
#49535=ADVANCED_FACE('',(#14448),#12312,.T.);
#49536=ADVANCED_FACE('',(#14449),#12313,.T.);
#49537=ADVANCED_FACE('',(#14450),#12314,.T.);
#49538=ADVANCED_FACE('',(#14451),#12315,.T.);
#49539=ADVANCED_FACE('',(#14452),#12316,.T.);
#49540=ADVANCED_FACE('',(#14453),#12317,.T.);
#49541=ADVANCED_FACE('',(#14454),#12318,.T.);
#49542=ADVANCED_FACE('',(#14455),#12319,.T.);
#49543=ADVANCED_FACE('',(#14456),#12320,.T.);
#49544=ADVANCED_FACE('',(#14457),#12321,.T.);
#49545=ADVANCED_FACE('',(#14458),#12322,.T.);
#49546=ADVANCED_FACE('',(#14459),#12323,.T.);
#49547=ADVANCED_FACE('',(#14460),#12324,.T.);
#49548=ADVANCED_FACE('',(#14461),#12325,.T.);
#49549=ADVANCED_FACE('',(#14462),#12326,.T.);
#49550=ADVANCED_FACE('',(#14463),#12327,.T.);
#49551=ADVANCED_FACE('',(#14464),#12328,.T.);
#49552=ADVANCED_FACE('',(#14465),#12329,.T.);
#49553=ADVANCED_FACE('',(#14466),#12330,.T.);
#49554=ADVANCED_FACE('',(#14467),#12331,.T.);
#49555=ADVANCED_FACE('',(#14468),#12332,.T.);
#49556=ADVANCED_FACE('',(#14469),#12333,.T.);
#49557=ADVANCED_FACE('',(#14470),#12334,.T.);
#49558=ADVANCED_FACE('',(#14471),#12335,.T.);
#49559=ADVANCED_FACE('',(#14472),#1074,.F.);
#49560=ADVANCED_FACE('',(#14473),#12336,.T.);
#49561=ADVANCED_FACE('',(#14474),#12337,.T.);
#49562=ADVANCED_FACE('',(#14475),#12338,.T.);
#49563=ADVANCED_FACE('',(#14476),#12339,.T.);
#49564=ADVANCED_FACE('',(#14477),#12340,.T.);
#49565=ADVANCED_FACE('',(#14478),#12341,.T.);
#49566=ADVANCED_FACE('',(#14479),#12342,.T.);
#49567=ADVANCED_FACE('',(#14480),#12343,.T.);
#49568=ADVANCED_FACE('',(#14481),#12344,.T.);
#49569=ADVANCED_FACE('',(#14482),#12345,.T.);
#49570=ADVANCED_FACE('',(#14483),#12346,.T.);
#49571=ADVANCED_FACE('',(#14484),#12347,.T.);
#49572=ADVANCED_FACE('',(#14485),#12348,.T.);
#49573=ADVANCED_FACE('',(#14486),#12349,.T.);
#49574=ADVANCED_FACE('',(#14487),#12350,.T.);
#49575=ADVANCED_FACE('',(#14488),#12351,.T.);
#49576=ADVANCED_FACE('',(#14489),#12352,.T.);
#49577=ADVANCED_FACE('',(#14490),#12353,.T.);
#49578=ADVANCED_FACE('',(#14491),#12354,.T.);
#49579=ADVANCED_FACE('',(#14492),#12355,.T.);
#49580=ADVANCED_FACE('',(#14493),#12356,.T.);
#49581=ADVANCED_FACE('',(#14494),#12357,.T.);
#49582=ADVANCED_FACE('',(#14495),#12358,.T.);
#49583=ADVANCED_FACE('',(#14496),#12359,.T.);
#49584=ADVANCED_FACE('',(#14497),#12360,.T.);
#49585=ADVANCED_FACE('',(#14498),#12361,.T.);
#49586=ADVANCED_FACE('',(#14499),#12362,.T.);
#49587=ADVANCED_FACE('',(#14500),#12363,.T.);
#49588=ADVANCED_FACE('',(#14501),#1075,.F.);
#49589=ADVANCED_FACE('',(#14502),#12364,.T.);
#49590=ADVANCED_FACE('',(#14503),#12365,.T.);
#49591=ADVANCED_FACE('',(#14504),#12366,.T.);
#49592=ADVANCED_FACE('',(#14505),#12367,.T.);
#49593=ADVANCED_FACE('',(#14506),#12368,.T.);
#49594=ADVANCED_FACE('',(#14507),#12369,.T.);
#49595=ADVANCED_FACE('',(#14508),#12370,.T.);
#49596=ADVANCED_FACE('',(#14509),#12371,.T.);
#49597=ADVANCED_FACE('',(#14510),#12372,.T.);
#49598=ADVANCED_FACE('',(#14511),#12373,.T.);
#49599=ADVANCED_FACE('',(#14512),#12374,.T.);
#49600=ADVANCED_FACE('',(#14513),#12375,.T.);
#49601=ADVANCED_FACE('',(#14514),#12376,.T.);
#49602=ADVANCED_FACE('',(#14515),#12377,.T.);
#49603=ADVANCED_FACE('',(#14516),#12378,.T.);
#49604=ADVANCED_FACE('',(#14517),#12379,.T.);
#49605=ADVANCED_FACE('',(#14518),#12380,.T.);
#49606=ADVANCED_FACE('',(#14519),#12381,.T.);
#49607=ADVANCED_FACE('',(#14520),#12382,.T.);
#49608=ADVANCED_FACE('',(#14521),#12383,.T.);
#49609=ADVANCED_FACE('',(#14522),#12384,.T.);
#49610=ADVANCED_FACE('',(#14523),#12385,.T.);
#49611=ADVANCED_FACE('',(#14524),#12386,.T.);
#49612=ADVANCED_FACE('',(#14525),#12387,.T.);
#49613=ADVANCED_FACE('',(#14526),#12388,.T.);
#49614=ADVANCED_FACE('',(#14527),#12389,.T.);
#49615=ADVANCED_FACE('',(#14528),#12390,.T.);
#49616=ADVANCED_FACE('',(#14529),#12391,.T.);
#49617=ADVANCED_FACE('',(#14530),#1076,.F.);
#49618=ADVANCED_FACE('',(#14531),#12392,.T.);
#49619=ADVANCED_FACE('',(#14532),#12393,.T.);
#49620=ADVANCED_FACE('',(#14533),#12394,.T.);
#49621=ADVANCED_FACE('',(#14534),#12395,.T.);
#49622=ADVANCED_FACE('',(#14535),#12396,.T.);
#49623=ADVANCED_FACE('',(#14536),#12397,.T.);
#49624=ADVANCED_FACE('',(#14537),#12398,.T.);
#49625=ADVANCED_FACE('',(#14538),#12399,.T.);
#49626=ADVANCED_FACE('',(#14539),#12400,.T.);
#49627=ADVANCED_FACE('',(#14540),#12401,.T.);
#49628=ADVANCED_FACE('',(#14541),#12402,.T.);
#49629=ADVANCED_FACE('',(#14542),#12403,.T.);
#49630=ADVANCED_FACE('',(#14543),#12404,.T.);
#49631=ADVANCED_FACE('',(#14544),#12405,.T.);
#49632=ADVANCED_FACE('',(#14545),#12406,.T.);
#49633=ADVANCED_FACE('',(#14546),#12407,.T.);
#49634=ADVANCED_FACE('',(#14547),#12408,.T.);
#49635=ADVANCED_FACE('',(#14548),#12409,.T.);
#49636=ADVANCED_FACE('',(#14549),#12410,.T.);
#49637=ADVANCED_FACE('',(#14550),#12411,.T.);
#49638=ADVANCED_FACE('',(#14551),#12412,.T.);
#49639=ADVANCED_FACE('',(#14552),#12413,.T.);
#49640=ADVANCED_FACE('',(#14553),#12414,.T.);
#49641=ADVANCED_FACE('',(#14554),#12415,.T.);
#49642=ADVANCED_FACE('',(#14555),#12416,.T.);
#49643=ADVANCED_FACE('',(#14556),#12417,.T.);
#49644=ADVANCED_FACE('',(#14557),#12418,.T.);
#49645=ADVANCED_FACE('',(#14558),#12419,.T.);
#49646=ADVANCED_FACE('',(#14559),#1077,.F.);
#49647=ADVANCED_FACE('',(#14560),#12420,.T.);
#49648=ADVANCED_FACE('',(#14561),#12421,.T.);
#49649=ADVANCED_FACE('',(#14562),#12422,.T.);
#49650=ADVANCED_FACE('',(#14563),#12423,.T.);
#49651=ADVANCED_FACE('',(#14564),#12424,.T.);
#49652=ADVANCED_FACE('',(#14565),#12425,.T.);
#49653=ADVANCED_FACE('',(#14566),#12426,.T.);
#49654=ADVANCED_FACE('',(#14567),#12427,.T.);
#49655=ADVANCED_FACE('',(#14568),#12428,.T.);
#49656=ADVANCED_FACE('',(#14569),#12429,.T.);
#49657=ADVANCED_FACE('',(#14570),#12430,.T.);
#49658=ADVANCED_FACE('',(#14571),#12431,.T.);
#49659=ADVANCED_FACE('',(#14572),#12432,.T.);
#49660=ADVANCED_FACE('',(#14573),#12433,.T.);
#49661=ADVANCED_FACE('',(#14574),#12434,.T.);
#49662=ADVANCED_FACE('',(#14575),#12435,.T.);
#49663=ADVANCED_FACE('',(#14576),#12436,.T.);
#49664=ADVANCED_FACE('',(#14577),#12437,.T.);
#49665=ADVANCED_FACE('',(#14578),#12438,.T.);
#49666=ADVANCED_FACE('',(#14579),#12439,.T.);
#49667=ADVANCED_FACE('',(#14580),#12440,.T.);
#49668=ADVANCED_FACE('',(#14581),#12441,.T.);
#49669=ADVANCED_FACE('',(#14582),#12442,.T.);
#49670=ADVANCED_FACE('',(#14583),#12443,.T.);
#49671=ADVANCED_FACE('',(#14584),#12444,.T.);
#49672=ADVANCED_FACE('',(#14585),#12445,.T.);
#49673=ADVANCED_FACE('',(#14586),#12446,.T.);
#49674=ADVANCED_FACE('',(#14587),#12447,.T.);
#49675=ADVANCED_FACE('',(#14588),#1078,.F.);
#49676=ADVANCED_FACE('',(#14589),#12448,.T.);
#49677=ADVANCED_FACE('',(#14590),#12449,.T.);
#49678=ADVANCED_FACE('',(#14591),#12450,.T.);
#49679=ADVANCED_FACE('',(#14592),#12451,.T.);
#49680=ADVANCED_FACE('',(#14593),#12452,.T.);
#49681=ADVANCED_FACE('',(#14594),#12453,.T.);
#49682=ADVANCED_FACE('',(#14595),#12454,.T.);
#49683=ADVANCED_FACE('',(#14596),#12455,.T.);
#49684=ADVANCED_FACE('',(#14597),#12456,.T.);
#49685=ADVANCED_FACE('',(#14598),#12457,.T.);
#49686=ADVANCED_FACE('',(#14599),#12458,.T.);
#49687=ADVANCED_FACE('',(#14600),#12459,.T.);
#49688=ADVANCED_FACE('',(#14601),#12460,.T.);
#49689=ADVANCED_FACE('',(#14602),#12461,.T.);
#49690=ADVANCED_FACE('',(#14603),#12462,.T.);
#49691=ADVANCED_FACE('',(#14604),#12463,.T.);
#49692=ADVANCED_FACE('',(#14605),#12464,.T.);
#49693=ADVANCED_FACE('',(#14606),#12465,.T.);
#49694=ADVANCED_FACE('',(#14607),#12466,.T.);
#49695=ADVANCED_FACE('',(#14608),#12467,.T.);
#49696=ADVANCED_FACE('',(#14609),#12468,.T.);
#49697=ADVANCED_FACE('',(#14610),#12469,.T.);
#49698=ADVANCED_FACE('',(#14611),#12470,.T.);
#49699=ADVANCED_FACE('',(#14612),#12471,.T.);
#49700=ADVANCED_FACE('',(#14613),#12472,.T.);
#49701=ADVANCED_FACE('',(#14614),#12473,.T.);
#49702=ADVANCED_FACE('',(#14615),#12474,.T.);
#49703=ADVANCED_FACE('',(#14616),#12475,.T.);
#49704=ADVANCED_FACE('',(#14617),#48188,.F.);
#49705=ADVANCED_FACE('',(#14618),#48189,.T.);
#49706=ADVANCED_FACE('',(#14619),#48190,.T.);
#49707=ADVANCED_FACE('',(#14620,#959),#12476,.T.);
#49708=ADVANCED_FACE('',(#14621),#947,.T.);
#49709=ADVANCED_FACE('',(#14622),#1079,.T.);
#49710=ADVANCED_FACE('',(#14623),#948,.F.);
#49711=ADVANCED_FACE('',(#14624),#1080,.T.);
#49712=ADVANCED_FACE('',(#14625,#960),#12477,.T.);
#49713=ADVANCED_FACE('',(#14626),#949,.F.);
#49714=ADVANCED_FACE('',(#14627,#961),#12478,.T.);
#49715=ADVANCED_FACE('',(#14628),#1081,.F.);
#49716=ADVANCED_FACE('',(#14629,#962),#12479,.T.);
#49717=ADVANCED_FACE('',(#14630),#48191,.T.);
#49718=ADVANCED_FACE('',(#14631),#1082,.T.);
#49719=ADVANCED_FACE('',(#14632),#48192,.T.);
#49720=ADVANCED_FACE('',(#14633),#1083,.T.);
#49721=ADVANCED_FACE('',(#14634),#48193,.T.);
#51018=CLOSED_SHELL('',(#48336,#48337,#48338,#48339,#48340,#48341,#48342,
#48343,#48344,#48345,#48346,#48347,#48348,#48349,#48350,#48351,#48352,#48353,
#48354,#48355,#48356,#48357,#48358,#48359,#48360,#48361,#48362,#48363,#48364,
#48365,#48366,#48367,#48368,#48369,#48370,#48371,#48372,#48373,#48374,#48375,
#48376,#48377,#48378,#48379,#48380,#48381,#48382,#48383,#48384,#48385,#48386,
#48387,#48388,#48389,#48390,#48391,#48392,#48393,#48394,#48395,#48396,#48397,
#48398,#48399,#48400,#48401,#48402,#48403,#48404,#48405,#48406,#48407,#48408,
#48409,#48410,#48411,#48412,#48413,#48414,#48415,#48416,#48417,#48418,#48419,
#48420,#48421,#48422,#48423,#48424,#48425,#48426,#48427,#48428,#48429,#48430,
#48431,#48432,#48433,#48434,#48435,#48436,#48437,#48438,#48439,#48440,#48441,
#48442,#48443,#48444,#48445,#48446,#48447,#48448,#48449,#48450,#48451,#48452,
#48453,#48454,#48455,#48456,#48457,#48458,#48459,#48460,#48461,#48462,#48463,
#48464,#48465,#48466,#48467,#48468,#48469,#48470,#48471,#48472,#48473,#48474,
#48475,#48476,#48477,#48478,#48479,#48480,#48481,#48482,#48483,#48484,#48485,
#48486,#48487,#48488,#48489,#48490,#48491,#48492,#48493,#48494,#48495,#48496,
#48497,#48498,#48499,#48500,#48501,#48502,#48503,#48504,#48505,#48506,#48507,
#48508,#48509,#48510,#48511,#48512,#48513,#48514,#48515,#48516,#48517,#48518,
#48519,#48520,#48521,#48522,#48523,#48524,#48525,#48526,#48527,#48528,#48529,
#48530,#48531,#48532,#48533,#48534,#48535,#48536,#48537,#48538,#48539,#48540,
#48541,#48542,#48543,#48544,#48545,#48546,#48547,#48548,#48549,#48550,#48551,
#48552,#48553,#48554,#48555,#48556,#48557,#48558,#48559,#48560,#48561,#48562,
#48563,#48564,#48565,#48566,#48567,#48568,#48569,#48570,#48571,#48572,#48573,
#48574,#48575,#48576,#48577,#48578,#48579,#48580,#48581,#48582,#48583,#48584,
#48585,#48586,#48587,#48588,#48589,#48590,#48591,#48592,#48593,#48594,#48595,
#48596,#48597,#48598,#48599,#48600,#48601,#48602,#48603,#48604,#48605,#48606,
#48607,#48608,#48609,#48610,#48611,#48612,#48613,#48614,#48615,#48616,#48617,
#48618,#48619,#48620,#48621,#48622,#48623,#48624,#48625,#48626,#48627,#48628,
#48629,#48630,#48631,#48632,#48633,#48634,#48635,#48636,#48637,#48638,#48639,
#48640,#48641,#48642,#48643,#48644,#48645,#48646,#48647,#48648,#48649,#48650,
#48651,#48652,#48653,#48654,#48655,#48656,#48657,#48658,#48659,#48660,#48661,
#48662,#48663,#48664,#48665,#48666,#48667,#48668,#48669,#48670,#48671,#48672,
#48673,#48674,#48675,#48676,#48677,#48678,#48679,#48680,#48681,#48682,#48683,
#48684,#48685,#48686,#48687,#48688,#48689,#48690,#48691,#48692,#48693,#48694,
#48695,#48696,#48697,#48698,#48699,#48700,#48701,#48702,#48703,#48704,#48705,
#48706,#48707,#48708,#48709,#48710,#48711,#48712,#48713,#48714,#48715,#48716,
#48717,#48718,#48719,#48720,#48721,#48722,#48723,#48724,#48725,#48726,#48727,
#48728,#48729,#48730,#48731,#48732,#48733,#48734,#48735,#48736,#48737,#48738,
#48739,#48740,#48741,#48742,#48743,#48744,#48745,#48746,#48747,#48748,#48749,
#48750,#48751,#48752,#48753,#48754,#48755,#48756,#48757,#48758,#48759,#48760,
#48761,#48762,#48763,#48764,#48765,#48766,#48767,#48768,#48769,#48770,#48771,
#48772,#48773,#48774,#48775,#48776,#48777,#48778,#48779,#48780,#48781,#48782,
#48783,#48784,#48785,#48786,#48787,#48788,#48789,#48790,#48791,#48792,#48793,
#48794,#48795,#48796,#48797,#48798,#48799,#48800,#48801,#48802,#48803,#48804,
#48805,#48806,#48807,#48808,#48809,#48810,#48811,#48812,#48813,#48814,#48815,
#48816,#48817,#48818,#48819,#48820,#48821,#48822,#48823,#48824,#48825,#48826,
#48827,#48828,#48829,#48830,#48831,#48832,#48833,#48834,#48835,#48836,#48837,
#48838,#48839,#48840,#48841,#48842,#48843,#48844,#48845,#48846,#48847,#48848,
#48849,#48850,#48851,#48852,#48853,#48854,#48855,#48856,#48857,#48858,#48859,
#48860,#48861,#48862,#48863,#48864,#48865,#48866,#48867,#48868,#48869,#48870,
#48871,#48872,#48873,#48874,#48875,#48876,#48877,#48878,#48879,#48880,#48881,
#48882,#48883,#48884,#48885,#48886,#48887,#48888,#48889,#48890,#48891,#48892,
#48893,#48894,#48895,#48896,#48897,#48898,#48899,#48900,#48901,#48902,#48903,
#48904,#48905,#48906,#48907,#48908,#48909,#48910,#48911,#48912,#48913,#48914,
#48915,#48916,#48917,#48918,#48919,#48920,#48921,#48922,#48923,#48924,#48925,
#48926,#48927,#48928,#48929,#48930,#48931,#48932,#48933,#48934,#48935,#48936,
#48937,#48938,#48939,#48940,#48941,#48942,#48943,#48944,#48945,#48946,#48947,
#48948,#48949,#48950,#48951,#48952,#48953,#48954,#48955,#48956,#48957,#48958,
#48959,#48960,#48961,#48962,#48963,#48964,#48965,#48966,#48967,#48968,#48969,
#48970,#48971,#48972,#48973,#48974,#48975,#48976,#48977,#48978,#48979,#48980,
#48981,#48982,#48983,#48984,#48985,#48986,#48987,#48988,#48989,#48990,#48991,
#48992,#48993,#48994,#48995,#48996,#48997,#48998,#48999,#49000,#49001,#49002,
#49003,#49004,#49005,#49006,#49007,#49008,#49009,#49010,#49011,#49012,#49013,
#49014,#49015,#49016,#49017,#49018,#49019,#49020,#49021,#49022,#49023,#49024,
#49025,#49026,#49027,#49028,#49029,#49030,#49031,#49032,#49033,#49034,#49035,
#49036,#49037,#49038,#49039,#49040,#49041,#49042,#49043,#49044,#49045,#49046,
#49047,#49048,#49049,#49050,#49051,#49052,#49053,#49054,#49055,#49056,#49057,
#49058,#49059,#49060,#49061,#49062,#49063,#49064,#49065,#49066,#49067,#49068,
#49069,#49070,#49071,#49072,#49073,#49074,#49075,#49076,#49077,#49078,#49079,
#49080,#49081,#49082,#49083,#49084,#49085,#49086,#49087,#49088,#49089,#49090,
#49091,#49092,#49093,#49094,#49095,#49096,#49097,#49098,#49099,#49100,#49101,
#49102,#49103,#49104,#49105,#49106,#49107,#49108,#49109,#49110,#49111,#49112,
#49113,#49114,#49115,#49116,#49117,#49118,#49119,#49120,#49121,#49122,#49123,
#49124,#49125,#49126,#49127,#49128,#49129,#49130,#49131,#49132,#49133,#49134,
#49135,#49136,#49137,#49138,#49139,#49140,#49141,#49142,#49143,#49144,#49145,
#49146,#49147,#49148,#49149,#49150,#49151,#49152,#49153,#49154,#49155,#49156,
#49157,#49158,#49159,#49160,#49161,#49162,#49163,#49164,#49165,#49166,#49167,
#49168,#49169,#49170,#49171,#49172,#49173,#49174,#49175,#49176,#49177,#49178,
#49179,#49180,#49181,#49182,#49183,#49184,#49185,#49186,#49187,#49188,#49189,
#49190,#49191,#49192,#49193,#49194,#49195,#49196,#49197,#49198,#49199,#49200,
#49201,#49202,#49203,#49204,#49205,#49206,#49207,#49208,#49209,#49210,#49211,
#49212,#49213,#49214,#49215,#49216,#49217,#49218,#49219,#49220,#49221,#49222,
#49223,#49224,#49225,#49226,#49227,#49228,#49229,#49230,#49231,#49232,#49233,
#49234,#49235,#49236,#49237,#49238,#49239,#49240,#49241,#49242,#49243,#49244,
#49245,#49246,#49247,#49248,#49249,#49250,#49251,#49252,#49253,#49254,#49255,
#49256,#49257,#49258,#49259,#49260,#49261,#49262,#49263,#49264,#49265,#49266,
#49267,#49268,#49269,#49270,#49271,#49272,#49273,#49274,#49275,#49276,#49277,
#49278,#49279,#49280,#49281,#49282,#49283,#49284,#49285,#49286,#49287,#49288,
#49289,#49290,#49291,#49292,#49293,#49294,#49295,#49296,#49297,#49298,#49299,
#49300,#49301,#49302,#49303,#49304,#49305,#49306,#49307,#49308,#49309,#49310,
#49311,#49312,#49313,#49314,#49315,#49316,#49317,#49318,#49319,#49320,#49321,
#49322,#49323,#49324,#49325,#49326,#49327,#49328,#49329,#49330,#49331,#49332,
#49333,#49334,#49335,#49336,#49337,#49338,#49339,#49340,#49341,#49342,#49343,
#49344,#49345,#49346,#49347,#49348,#49349,#49350,#49351,#49352,#49353,#49354,
#49355,#49356,#49357,#49358,#49359,#49360,#49361,#49362,#49363,#49364,#49365,
#49366,#49367,#49368,#49369,#49370,#49371,#49372,#49373,#49374,#49375,#49376,
#49377,#49378,#49379,#49380,#49381,#49382,#49383,#49384,#49385,#49386,#49387,
#49388,#49389,#49390,#49391,#49392,#49393,#49394,#49395,#49396,#49397,#49398,
#49399,#49400,#49401,#49402,#49403,#49404,#49405,#49406,#49407,#49408,#49409,
#49410,#49411,#49412,#49413,#49414,#49415,#49416,#49417,#49418,#49419,#49420,
#49421,#49422,#49423,#49424,#49425,#49426,#49427,#49428,#49429,#49430,#49431,
#49432,#49433,#49434,#49435,#49436,#49437,#49438,#49439,#49440,#49441,#49442,
#49443,#49444,#49445,#49446,#49447,#49448,#49449,#49450,#49451,#49452,#49453,
#49454,#49455,#49456,#49457,#49458,#49459,#49460,#49461,#49462,#49463,#49464,
#49465,#49466,#49467,#49468,#49469,#49470,#49471,#49472,#49473,#49474,#49475,
#49476,#49477,#49478,#49479,#49480,#49481,#49482,#49483,#49484,#49485,#49486,
#49487,#49488,#49489,#49490,#49491,#49492,#49493,#49494,#49495,#49496,#49497,
#49498,#49499,#49500,#49501,#49502,#49503,#49504,#49505,#49506,#49507,#49508,
#49509,#49510,#49511,#49512,#49513,#49514,#49515,#49516,#49517,#49518,#49519,
#49520,#49521,#49522,#49523,#49524,#49525,#49526,#49527,#49528,#49529,#49530,
#49531,#49532,#49533,#49534,#49535,#49536,#49537,#49538,#49539,#49540,#49541,
#49542,#49543,#49544,#49545,#49546,#49547,#49548,#49549,#49550,#49551,#49552,
#49553,#49554,#49555,#49556,#49557,#49558,#49559,#49560,#49561,#49562,#49563,
#49564,#49565,#49566,#49567,#49568,#49569,#49570,#49571,#49572,#49573,#49574,
#49575,#49576,#49577,#49578,#49579,#49580,#49581,#49582,#49583,#49584,#49585,
#49586,#49587,#49588,#49589,#49590,#49591,#49592,#49593,#49594,#49595,#49596,
#49597,#49598,#49599,#49600,#49601,#49602,#49603,#49604,#49605,#49606,#49607,
#49608,#49609,#49610,#49611,#49612,#49613,#49614,#49615,#49616,#49617,#49618,
#49619,#49620,#49621,#49622,#49623,#49624,#49625,#49626,#49627,#49628,#49629,
#49630,#49631,#49632,#49633,#49634,#49635,#49636,#49637,#49638,#49639,#49640,
#49641,#49642,#49643,#49644,#49645,#49646,#49647,#49648,#49649,#49650,#49651,
#49652,#49653,#49654,#49655,#49656,#49657,#49658,#49659,#49660,#49661,#49662,
#49663,#49664,#49665,#49666,#49667,#49668,#49669,#49670,#49671,#49672,#49673,
#49674,#49675,#49676,#49677,#49678,#49679,#49680,#49681,#49682,#49683,#49684,
#49685,#49686,#49687,#49688,#49689,#49690,#49691,#49692,#49693,#49694,#49695,
#49696,#49697,#49698,#49699,#49700,#49701,#49702,#49703,#49704,#49705,#49706,
#49707,#49708,#49709,#49710,#49711,#49712,#49713,#49714,#49715,#49716,#49717,
#49718,#49719,#49720,#49721));
#51188=AXIS2_PLACEMENT_3D('',#68259,#55370,#55371);
#51189=AXIS2_PLACEMENT_3D('',#68260,#55372,#55373);
#51190=AXIS2_PLACEMENT_3D('',#68263,#55374,#55375);
#51191=AXIS2_PLACEMENT_3D('',#68275,#55376,#55377);
#51192=AXIS2_PLACEMENT_3D('',#68278,#55378,#55379);
#51193=AXIS2_PLACEMENT_3D('',#68290,#55380,#55381);
#51194=AXIS2_PLACEMENT_3D('',#68293,#55382,#55383);
#51195=AXIS2_PLACEMENT_3D('',#68305,#55384,#55385);
#51196=AXIS2_PLACEMENT_3D('',#68308,#55386,#55387);
#51197=AXIS2_PLACEMENT_3D('',#68320,#55388,#55389);
#51198=AXIS2_PLACEMENT_3D('',#68323,#55390,#55391);
#51199=AXIS2_PLACEMENT_3D('',#68335,#55392,#55393);
#51200=AXIS2_PLACEMENT_3D('',#68338,#55394,#55395);
#51201=AXIS2_PLACEMENT_3D('',#68350,#55396,#55397);
#51202=AXIS2_PLACEMENT_3D('',#68353,#55398,#55399);
#51203=AXIS2_PLACEMENT_3D('',#68365,#55400,#55401);
#51204=AXIS2_PLACEMENT_3D('',#68368,#55402,#55403);
#51205=AXIS2_PLACEMENT_3D('',#68380,#55404,#55405);
#51206=AXIS2_PLACEMENT_3D('',#68383,#55406,#55407);
#51207=AXIS2_PLACEMENT_3D('',#68395,#55408,#55409);
#51208=AXIS2_PLACEMENT_3D('',#68398,#55410,#55411);
#51209=AXIS2_PLACEMENT_3D('',#68410,#55412,#55413);
#51210=AXIS2_PLACEMENT_3D('',#68413,#55414,#55415);
#51211=AXIS2_PLACEMENT_3D('',#68425,#55416,#55417);
#51212=AXIS2_PLACEMENT_3D('',#68428,#55418,#55419);
#51213=AXIS2_PLACEMENT_3D('',#68440,#55420,#55421);
#51214=AXIS2_PLACEMENT_3D('',#68443,#55422,#55423);
#51215=AXIS2_PLACEMENT_3D('',#68455,#55424,#55425);
#51216=AXIS2_PLACEMENT_3D('',#68458,#55426,#55427);
#51217=AXIS2_PLACEMENT_3D('',#68470,#55428,#55429);
#51218=AXIS2_PLACEMENT_3D('',#68473,#55430,#55431);
#51219=AXIS2_PLACEMENT_3D('',#68485,#55432,#55433);
#51220=AXIS2_PLACEMENT_3D('',#68488,#55434,#55435);
#51221=AXIS2_PLACEMENT_3D('',#68500,#55436,#55437);
#51222=AXIS2_PLACEMENT_3D('',#68503,#55438,#55439);
#51223=AXIS2_PLACEMENT_3D('',#68515,#55440,#55441);
#51224=AXIS2_PLACEMENT_3D('',#68518,#55442,#55443);
#51225=AXIS2_PLACEMENT_3D('',#68530,#55444,#55445);
#51226=AXIS2_PLACEMENT_3D('',#68533,#55446,#55447);
#51227=AXIS2_PLACEMENT_3D('',#68545,#55448,#55449);
#51228=AXIS2_PLACEMENT_3D('',#68548,#55450,#55451);
#51229=AXIS2_PLACEMENT_3D('',#68560,#55452,#55453);
#51230=AXIS2_PLACEMENT_3D('',#68563,#55454,#55455);
#51231=AXIS2_PLACEMENT_3D('',#68575,#55456,#55457);
#51232=AXIS2_PLACEMENT_3D('',#68578,#55458,#55459);
#51233=AXIS2_PLACEMENT_3D('',#68590,#55460,#55461);
#51234=AXIS2_PLACEMENT_3D('',#68593,#55462,#55463);
#51235=AXIS2_PLACEMENT_3D('',#68605,#55464,#55465);
#51236=AXIS2_PLACEMENT_3D('',#68608,#55466,#55467);
#51237=AXIS2_PLACEMENT_3D('',#68620,#55468,#55469);
#51238=AXIS2_PLACEMENT_3D('',#68623,#55470,#55471);
#51239=AXIS2_PLACEMENT_3D('',#68635,#55472,#55473);
#51240=AXIS2_PLACEMENT_3D('',#68638,#55474,#55475);
#51241=AXIS2_PLACEMENT_3D('',#68650,#55476,#55477);
#51242=AXIS2_PLACEMENT_3D('',#68653,#55478,#55479);
#51243=AXIS2_PLACEMENT_3D('',#68665,#55480,#55481);
#51244=AXIS2_PLACEMENT_3D('',#68668,#55482,#55483);
#51245=AXIS2_PLACEMENT_3D('',#68680,#55484,#55485);
#51246=AXIS2_PLACEMENT_3D('',#68683,#55486,#55487);
#51247=AXIS2_PLACEMENT_3D('',#68695,#55488,#55489);
#51248=AXIS2_PLACEMENT_3D('',#68698,#55490,#55491);
#51249=AXIS2_PLACEMENT_3D('',#68710,#55492,#55493);
#51250=AXIS2_PLACEMENT_3D('',#68713,#55494,#55495);
#51251=AXIS2_PLACEMENT_3D('',#68725,#55496,#55497);
#51252=AXIS2_PLACEMENT_3D('',#68728,#55498,#55499);
#51253=AXIS2_PLACEMENT_3D('',#68740,#55500,#55501);
#51254=AXIS2_PLACEMENT_3D('',#68743,#55502,#55503);
#51255=AXIS2_PLACEMENT_3D('',#68755,#55504,#55505);
#51256=AXIS2_PLACEMENT_3D('',#68758,#55506,#55507);
#51257=AXIS2_PLACEMENT_3D('',#68770,#55508,#55509);
#51258=AXIS2_PLACEMENT_3D('',#68773,#55510,#55511);
#51259=AXIS2_PLACEMENT_3D('',#68785,#55512,#55513);
#51260=AXIS2_PLACEMENT_3D('',#68788,#55514,#55515);
#51261=AXIS2_PLACEMENT_3D('',#68800,#55516,#55517);
#51262=AXIS2_PLACEMENT_3D('',#68864,#55548,#55549);
#51263=AXIS2_PLACEMENT_3D('',#68874,#55552,#55553);
#51264=AXIS2_PLACEMENT_3D('',#68876,#55555,#55556);
#51265=AXIS2_PLACEMENT_3D('',#68940,#55587,#55588);
#51266=AXIS2_PLACEMENT_3D('',#68950,#55591,#55592);
#51267=AXIS2_PLACEMENT_3D('',#68952,#55594,#55595);
#51268=AXIS2_PLACEMENT_3D('',#69016,#55626,#55627);
#51269=AXIS2_PLACEMENT_3D('',#69026,#55630,#55631);
#51270=AXIS2_PLACEMENT_3D('',#69028,#55633,#55634);
#51271=AXIS2_PLACEMENT_3D('',#69092,#55665,#55666);
#51272=AXIS2_PLACEMENT_3D('',#69102,#55669,#55670);
#51273=AXIS2_PLACEMENT_3D('',#69104,#55672,#55673);
#51274=AXIS2_PLACEMENT_3D('',#69168,#55704,#55705);
#51275=AXIS2_PLACEMENT_3D('',#69178,#55708,#55709);
#51276=AXIS2_PLACEMENT_3D('',#69180,#55711,#55712);
#51277=AXIS2_PLACEMENT_3D('',#69244,#55743,#55744);
#51278=AXIS2_PLACEMENT_3D('',#69254,#55747,#55748);
#51279=AXIS2_PLACEMENT_3D('',#69256,#55750,#55751);
#51280=AXIS2_PLACEMENT_3D('',#69320,#55782,#55783);
#51281=AXIS2_PLACEMENT_3D('',#69330,#55786,#55787);
#51282=AXIS2_PLACEMENT_3D('',#69332,#55789,#55790);
#51283=AXIS2_PLACEMENT_3D('',#69396,#55821,#55822);
#51284=AXIS2_PLACEMENT_3D('',#69406,#55825,#55826);
#51285=AXIS2_PLACEMENT_3D('',#69408,#55828,#55829);
#51286=AXIS2_PLACEMENT_3D('',#69472,#55860,#55861);
#51287=AXIS2_PLACEMENT_3D('',#69482,#55864,#55865);
#51288=AXIS2_PLACEMENT_3D('',#69484,#55867,#55868);
#51289=AXIS2_PLACEMENT_3D('',#69548,#55899,#55900);
#51290=AXIS2_PLACEMENT_3D('',#69558,#55903,#55904);
#51291=AXIS2_PLACEMENT_3D('',#69560,#55906,#55907);
#51292=AXIS2_PLACEMENT_3D('',#69624,#55938,#55939);
#51293=AXIS2_PLACEMENT_3D('',#69634,#55942,#55943);
#51294=AXIS2_PLACEMENT_3D('',#69636,#55945,#55946);
#51295=AXIS2_PLACEMENT_3D('',#69700,#55977,#55978);
#51296=AXIS2_PLACEMENT_3D('',#69710,#55981,#55982);
#51297=AXIS2_PLACEMENT_3D('',#69712,#55984,#55985);
#51298=AXIS2_PLACEMENT_3D('',#69776,#56016,#56017);
#51299=AXIS2_PLACEMENT_3D('',#69786,#56020,#56021);
#51300=AXIS2_PLACEMENT_3D('',#69788,#56023,#56024);
#51301=AXIS2_PLACEMENT_3D('',#69852,#56055,#56056);
#51302=AXIS2_PLACEMENT_3D('',#69862,#56059,#56060);
#51303=AXIS2_PLACEMENT_3D('',#69864,#56062,#56063);
#51304=AXIS2_PLACEMENT_3D('',#69928,#56094,#56095);
#51305=AXIS2_PLACEMENT_3D('',#69938,#56098,#56099);
#51306=AXIS2_PLACEMENT_3D('',#69940,#56101,#56102);
#51307=AXIS2_PLACEMENT_3D('',#70004,#56133,#56134);
#51308=AXIS2_PLACEMENT_3D('',#70014,#56137,#56138);
#51309=AXIS2_PLACEMENT_3D('',#70016,#56140,#56141);
#51310=AXIS2_PLACEMENT_3D('',#70080,#56172,#56173);
#51311=AXIS2_PLACEMENT_3D('',#70090,#56176,#56177);
#51312=AXIS2_PLACEMENT_3D('',#70092,#56179,#56180);
#51313=AXIS2_PLACEMENT_3D('',#70156,#56211,#56212);
#51314=AXIS2_PLACEMENT_3D('',#70166,#56215,#56216);
#51315=AXIS2_PLACEMENT_3D('',#70168,#56218,#56219);
#51316=AXIS2_PLACEMENT_3D('',#70232,#56250,#56251);
#51317=AXIS2_PLACEMENT_3D('',#70242,#56254,#56255);
#51318=AXIS2_PLACEMENT_3D('',#70244,#56257,#56258);
#51319=AXIS2_PLACEMENT_3D('',#70308,#56289,#56290);
#51320=AXIS2_PLACEMENT_3D('',#70318,#56293,#56294);
#51321=AXIS2_PLACEMENT_3D('',#70320,#56296,#56297);
#51322=AXIS2_PLACEMENT_3D('',#70384,#56328,#56329);
#51323=AXIS2_PLACEMENT_3D('',#70394,#56332,#56333);
#51324=AXIS2_PLACEMENT_3D('',#70396,#56335,#56336);
#51325=AXIS2_PLACEMENT_3D('',#70460,#56367,#56368);
#51326=AXIS2_PLACEMENT_3D('',#70470,#56371,#56372);
#51327=AXIS2_PLACEMENT_3D('',#70472,#56374,#56375);
#51328=AXIS2_PLACEMENT_3D('',#70536,#56406,#56407);
#51329=AXIS2_PLACEMENT_3D('',#70546,#56410,#56411);
#51330=AXIS2_PLACEMENT_3D('',#70548,#56413,#56414);
#51331=AXIS2_PLACEMENT_3D('',#70612,#56445,#56446);
#51332=AXIS2_PLACEMENT_3D('',#70622,#56449,#56450);
#51333=AXIS2_PLACEMENT_3D('',#70624,#56452,#56453);
#51334=AXIS2_PLACEMENT_3D('',#70688,#56484,#56485);
#51335=AXIS2_PLACEMENT_3D('',#70698,#56488,#56489);
#51336=AXIS2_PLACEMENT_3D('',#70700,#56491,#56492);
#51337=AXIS2_PLACEMENT_3D('',#70764,#56523,#56524);
#51338=AXIS2_PLACEMENT_3D('',#70774,#56527,#56528);
#51339=AXIS2_PLACEMENT_3D('',#70776,#56530,#56531);
#51340=AXIS2_PLACEMENT_3D('',#70840,#56562,#56563);
#51341=AXIS2_PLACEMENT_3D('',#70850,#56566,#56567);
#51342=AXIS2_PLACEMENT_3D('',#70852,#56569,#56570);
#51343=AXIS2_PLACEMENT_3D('',#70916,#56601,#56602);
#51344=AXIS2_PLACEMENT_3D('',#70926,#56605,#56606);
#51345=AXIS2_PLACEMENT_3D('',#70928,#56608,#56609);
#51346=AXIS2_PLACEMENT_3D('',#70992,#56640,#56641);
#51347=AXIS2_PLACEMENT_3D('',#71002,#56644,#56645);
#51348=AXIS2_PLACEMENT_3D('',#71004,#56647,#56648);
#51349=AXIS2_PLACEMENT_3D('',#71068,#56679,#56680);
#51350=AXIS2_PLACEMENT_3D('',#71078,#56683,#56684);
#51351=AXIS2_PLACEMENT_3D('',#71080,#56686,#56687);
#51352=AXIS2_PLACEMENT_3D('',#71144,#56718,#56719);
#51353=AXIS2_PLACEMENT_3D('',#71154,#56722,#56723);
#51354=AXIS2_PLACEMENT_3D('',#71156,#56725,#56726);
#51355=AXIS2_PLACEMENT_3D('',#71220,#56757,#56758);
#51356=AXIS2_PLACEMENT_3D('',#71230,#56761,#56762);
#51357=AXIS2_PLACEMENT_3D('',#71232,#56764,#56765);
#51358=AXIS2_PLACEMENT_3D('',#71296,#56796,#56797);
#51359=AXIS2_PLACEMENT_3D('',#71306,#56800,#56801);
#51360=AXIS2_PLACEMENT_3D('',#71308,#56803,#56804);
#51361=AXIS2_PLACEMENT_3D('',#71372,#56835,#56836);
#51362=AXIS2_PLACEMENT_3D('',#71382,#56839,#56840);
#51363=AXIS2_PLACEMENT_3D('',#71384,#56842,#56843);
#51364=AXIS2_PLACEMENT_3D('',#71448,#56874,#56875);
#51365=AXIS2_PLACEMENT_3D('',#71458,#56878,#56879);
#51366=AXIS2_PLACEMENT_3D('',#71460,#56881,#56882);
#51367=AXIS2_PLACEMENT_3D('',#71524,#56913,#56914);
#51368=AXIS2_PLACEMENT_3D('',#71534,#56917,#56918);
#51369=AXIS2_PLACEMENT_3D('',#71536,#56920,#56921);
#51370=AXIS2_PLACEMENT_3D('',#71539,#56922,#56923);
#51371=AXIS2_PLACEMENT_3D('',#71546,#56924,#56925);
#51372=AXIS2_PLACEMENT_3D('',#71549,#56926,#56927);
#51373=AXIS2_PLACEMENT_3D('',#71556,#56928,#56929);
#51374=AXIS2_PLACEMENT_3D('',#71559,#56930,#56931);
#51375=AXIS2_PLACEMENT_3D('',#71566,#56932,#56933);
#51376=AXIS2_PLACEMENT_3D('',#71569,#56934,#56935);
#51377=AXIS2_PLACEMENT_3D('',#71576,#56936,#56937);
#51378=AXIS2_PLACEMENT_3D('',#71579,#56938,#56939);
#51379=AXIS2_PLACEMENT_3D('',#71586,#56940,#56941);
#51380=AXIS2_PLACEMENT_3D('',#71589,#56942,#56943);
#51381=AXIS2_PLACEMENT_3D('',#71596,#56944,#56945);
#51382=AXIS2_PLACEMENT_3D('',#71599,#56946,#56947);
#51383=AXIS2_PLACEMENT_3D('',#71606,#56948,#56949);
#51384=AXIS2_PLACEMENT_3D('',#71609,#56950,#56951);
#51385=AXIS2_PLACEMENT_3D('',#71616,#56952,#56953);
#51386=AXIS2_PLACEMENT_3D('',#71619,#56954,#56955);
#51387=AXIS2_PLACEMENT_3D('',#71626,#56956,#56957);
#51388=AXIS2_PLACEMENT_3D('',#71629,#56958,#56959);
#51389=AXIS2_PLACEMENT_3D('',#71636,#56960,#56961);
#51390=AXIS2_PLACEMENT_3D('',#71639,#56962,#56963);
#51391=AXIS2_PLACEMENT_3D('',#71646,#56964,#56965);
#51392=AXIS2_PLACEMENT_3D('',#71649,#56966,#56967);
#51393=AXIS2_PLACEMENT_3D('',#71656,#56968,#56969);
#51394=AXIS2_PLACEMENT_3D('',#71659,#56970,#56971);
#51395=AXIS2_PLACEMENT_3D('',#71666,#56972,#56973);
#51396=AXIS2_PLACEMENT_3D('',#71669,#56974,#56975);
#51397=AXIS2_PLACEMENT_3D('',#71676,#56976,#56977);
#51398=AXIS2_PLACEMENT_3D('',#71679,#56978,#56979);
#51399=AXIS2_PLACEMENT_3D('',#71686,#56980,#56981);
#51400=AXIS2_PLACEMENT_3D('',#71689,#56982,#56983);
#51401=AXIS2_PLACEMENT_3D('',#71696,#56984,#56985);
#51402=AXIS2_PLACEMENT_3D('',#71699,#56986,#56987);
#51403=AXIS2_PLACEMENT_3D('',#71706,#56988,#56989);
#51404=AXIS2_PLACEMENT_3D('',#71709,#56990,#56991);
#51405=AXIS2_PLACEMENT_3D('',#71716,#56992,#56993);
#51406=AXIS2_PLACEMENT_3D('',#71719,#56994,#56995);
#51407=AXIS2_PLACEMENT_3D('',#71726,#56996,#56997);
#51408=AXIS2_PLACEMENT_3D('',#71729,#56998,#56999);
#51409=AXIS2_PLACEMENT_3D('',#71736,#57000,#57001);
#51410=AXIS2_PLACEMENT_3D('',#71739,#57002,#57003);
#51411=AXIS2_PLACEMENT_3D('',#71746,#57004,#57005);
#51412=AXIS2_PLACEMENT_3D('',#71749,#57006,#57007);
#51413=AXIS2_PLACEMENT_3D('',#71756,#57008,#57009);
#51414=AXIS2_PLACEMENT_3D('',#71759,#57010,#57011);
#51415=AXIS2_PLACEMENT_3D('',#71766,#57012,#57013);
#51416=AXIS2_PLACEMENT_3D('',#71769,#57014,#57015);
#51417=AXIS2_PLACEMENT_3D('',#71776,#57016,#57017);
#51418=AXIS2_PLACEMENT_3D('',#71779,#57018,#57019);
#51419=AXIS2_PLACEMENT_3D('',#71786,#57020,#57021);
#51420=AXIS2_PLACEMENT_3D('',#71789,#57022,#57023);
#51421=AXIS2_PLACEMENT_3D('',#71796,#57024,#57025);
#51422=AXIS2_PLACEMENT_3D('',#71799,#57026,#57027);
#51423=AXIS2_PLACEMENT_3D('',#71806,#57028,#57029);
#51424=AXIS2_PLACEMENT_3D('',#71809,#57030,#57031);
#51425=AXIS2_PLACEMENT_3D('',#71816,#57032,#57033);
#51426=AXIS2_PLACEMENT_3D('',#71819,#57034,#57035);
#51427=AXIS2_PLACEMENT_3D('',#71826,#57036,#57037);
#51428=AXIS2_PLACEMENT_3D('',#71829,#57038,#57039);
#51429=AXIS2_PLACEMENT_3D('',#71836,#57040,#57041);
#51430=AXIS2_PLACEMENT_3D('',#71839,#57042,#57043);
#51431=AXIS2_PLACEMENT_3D('',#71846,#57044,#57045);
#51432=AXIS2_PLACEMENT_3D('',#71849,#57046,#57047);
#51433=AXIS2_PLACEMENT_3D('',#71856,#57048,#57049);
#51434=AXIS2_PLACEMENT_3D('',#71859,#57050,#57051);
#51435=AXIS2_PLACEMENT_3D('',#71866,#57052,#57053);
#51436=AXIS2_PLACEMENT_3D('',#71869,#57054,#57055);
#51437=AXIS2_PLACEMENT_3D('',#71876,#57056,#57057);
#51438=AXIS2_PLACEMENT_3D('',#71879,#57058,#57059);
#51439=AXIS2_PLACEMENT_3D('',#71886,#57060,#57061);
#51440=AXIS2_PLACEMENT_3D('',#71889,#57062,#57063);
#51441=AXIS2_PLACEMENT_3D('',#71896,#57064,#57065);
#51442=AXIS2_PLACEMENT_3D('',#71906,#57068,#57069);
#51443=AXIS2_PLACEMENT_3D('',#71908,#57071,#57072);
#51444=AXIS2_PLACEMENT_3D('',#71918,#57075,#57076);
#51445=AXIS2_PLACEMENT_3D('',#71920,#57078,#57079);
#51446=AXIS2_PLACEMENT_3D('',#71930,#57082,#57083);
#51447=AXIS2_PLACEMENT_3D('',#71932,#57085,#57086);
#51448=AXIS2_PLACEMENT_3D('',#71942,#57089,#57090);
#51449=AXIS2_PLACEMENT_3D('',#71944,#57092,#57093);
#51450=AXIS2_PLACEMENT_3D('',#71954,#57096,#57097);
#51451=AXIS2_PLACEMENT_3D('',#71956,#57099,#57100);
#51452=AXIS2_PLACEMENT_3D('',#71966,#57103,#57104);
#51453=AXIS2_PLACEMENT_3D('',#71968,#57106,#57107);
#51454=AXIS2_PLACEMENT_3D('',#71978,#57110,#57111);
#51455=AXIS2_PLACEMENT_3D('',#71980,#57113,#57114);
#51456=AXIS2_PLACEMENT_3D('',#71990,#57117,#57118);
#51457=AXIS2_PLACEMENT_3D('',#71992,#57120,#57121);
#51458=AXIS2_PLACEMENT_3D('',#72002,#57124,#57125);
#51459=AXIS2_PLACEMENT_3D('',#72004,#57127,#57128);
#51460=AXIS2_PLACEMENT_3D('',#72014,#57131,#57132);
#51461=AXIS2_PLACEMENT_3D('',#72016,#57134,#57135);
#51462=AXIS2_PLACEMENT_3D('',#72026,#57138,#57139);
#51463=AXIS2_PLACEMENT_3D('',#72028,#57141,#57142);
#51464=AXIS2_PLACEMENT_3D('',#72038,#57145,#57146);
#51465=AXIS2_PLACEMENT_3D('',#72040,#57148,#57149);
#51466=AXIS2_PLACEMENT_3D('',#72050,#57152,#57153);
#51467=AXIS2_PLACEMENT_3D('',#72052,#57155,#57156);
#51468=AXIS2_PLACEMENT_3D('',#72062,#57159,#57160);
#51469=AXIS2_PLACEMENT_3D('',#72064,#57162,#57163);
#51470=AXIS2_PLACEMENT_3D('',#72074,#57166,#57167);
#51471=AXIS2_PLACEMENT_3D('',#72076,#57169,#57170);
#51472=AXIS2_PLACEMENT_3D('',#72086,#57173,#57174);
#51473=AXIS2_PLACEMENT_3D('',#72088,#57176,#57177);
#51474=AXIS2_PLACEMENT_3D('',#72098,#57180,#57181);
#51475=AXIS2_PLACEMENT_3D('',#72100,#57183,#57184);
#51476=AXIS2_PLACEMENT_3D('',#72110,#57187,#57188);
#51477=AXIS2_PLACEMENT_3D('',#72112,#57190,#57191);
#51478=AXIS2_PLACEMENT_3D('',#72122,#57194,#57195);
#51479=AXIS2_PLACEMENT_3D('',#72124,#57197,#57198);
#51480=AXIS2_PLACEMENT_3D('',#72134,#57201,#57202);
#51481=AXIS2_PLACEMENT_3D('',#72136,#57204,#57205);
#51482=AXIS2_PLACEMENT_3D('',#72146,#57208,#57209);
#51483=AXIS2_PLACEMENT_3D('',#72148,#57211,#57212);
#51484=AXIS2_PLACEMENT_3D('',#72158,#57215,#57216);
#51485=AXIS2_PLACEMENT_3D('',#72160,#57218,#57219);
#51486=AXIS2_PLACEMENT_3D('',#72170,#57222,#57223);
#51487=AXIS2_PLACEMENT_3D('',#72172,#57225,#57226);
#51488=AXIS2_PLACEMENT_3D('',#72182,#57229,#57230);
#51489=AXIS2_PLACEMENT_3D('',#72184,#57232,#57233);
#51490=AXIS2_PLACEMENT_3D('',#72194,#57236,#57237);
#51491=AXIS2_PLACEMENT_3D('',#72196,#57239,#57240);
#51492=AXIS2_PLACEMENT_3D('',#72206,#57243,#57244);
#51493=AXIS2_PLACEMENT_3D('',#72208,#57246,#57247);
#51494=AXIS2_PLACEMENT_3D('',#72218,#57250,#57251);
#51495=AXIS2_PLACEMENT_3D('',#72220,#57253,#57254);
#51496=AXIS2_PLACEMENT_3D('',#72230,#57257,#57258);
#51497=AXIS2_PLACEMENT_3D('',#72232,#57260,#57261);
#51498=AXIS2_PLACEMENT_3D('',#72242,#57264,#57265);
#51499=AXIS2_PLACEMENT_3D('',#72244,#57267,#57268);
#51500=AXIS2_PLACEMENT_3D('',#72254,#57271,#57272);
#51501=AXIS2_PLACEMENT_3D('',#72256,#57274,#57275);
#51502=AXIS2_PLACEMENT_3D('',#72266,#57278,#57279);
#51503=AXIS2_PLACEMENT_3D('',#72268,#57281,#57282);
#51504=AXIS2_PLACEMENT_3D('',#72278,#57285,#57286);
#51505=AXIS2_PLACEMENT_3D('',#72280,#57288,#57289);
#51506=AXIS2_PLACEMENT_3D('',#72290,#57292,#57293);
#51507=AXIS2_PLACEMENT_3D('',#72292,#57295,#57296);
#51508=AXIS2_PLACEMENT_3D('',#72302,#57299,#57300);
#51509=AXIS2_PLACEMENT_3D('',#72304,#57302,#57303);
#51510=AXIS2_PLACEMENT_3D('',#72314,#57306,#57307);
#51511=AXIS2_PLACEMENT_3D('',#72316,#57309,#57310);
#51512=AXIS2_PLACEMENT_3D('',#72326,#57313,#57314);
#51513=AXIS2_PLACEMENT_3D('',#72328,#57316,#57317);
#51514=AXIS2_PLACEMENT_3D('',#72332,#57320,#57321);
#51515=AXIS2_PLACEMENT_3D('',#72336,#57324,#57325);
#51516=AXIS2_PLACEMENT_3D('',#72340,#57328,#57329);
#51517=AXIS2_PLACEMENT_3D('',#72344,#57332,#57333);
#51518=AXIS2_PLACEMENT_3D('',#72348,#57336,#57337);
#51519=AXIS2_PLACEMENT_3D('',#72352,#57340,#57341);
#51520=AXIS2_PLACEMENT_3D('',#72356,#57344,#57345);
#51521=AXIS2_PLACEMENT_3D('',#72360,#57348,#57349);
#51522=AXIS2_PLACEMENT_3D('',#72364,#57352,#57353);
#51523=AXIS2_PLACEMENT_3D('',#72368,#57356,#57357);
#51524=AXIS2_PLACEMENT_3D('',#72372,#57360,#57361);
#51525=AXIS2_PLACEMENT_3D('',#72376,#57364,#57365);
#51526=AXIS2_PLACEMENT_3D('',#72380,#57368,#57369);
#51527=AXIS2_PLACEMENT_3D('',#72384,#57372,#57373);
#51528=AXIS2_PLACEMENT_3D('',#72388,#57376,#57377);
#51529=AXIS2_PLACEMENT_3D('',#72392,#57380,#57381);
#51530=AXIS2_PLACEMENT_3D('',#72396,#57384,#57385);
#51531=AXIS2_PLACEMENT_3D('',#72400,#57388,#57389);
#51532=AXIS2_PLACEMENT_3D('',#72404,#57392,#57393);
#51533=AXIS2_PLACEMENT_3D('',#72408,#57396,#57397);
#51534=AXIS2_PLACEMENT_3D('',#72412,#57400,#57401);
#51535=AXIS2_PLACEMENT_3D('',#72416,#57404,#57405);
#51536=AXIS2_PLACEMENT_3D('',#72420,#57408,#57409);
#51537=AXIS2_PLACEMENT_3D('',#72424,#57412,#57413);
#51538=AXIS2_PLACEMENT_3D('',#72428,#57416,#57417);
#51539=AXIS2_PLACEMENT_3D('',#72432,#57420,#57421);
#51540=AXIS2_PLACEMENT_3D('',#72436,#57424,#57425);
#51541=AXIS2_PLACEMENT_3D('',#72440,#57428,#57429);
#51542=AXIS2_PLACEMENT_3D('',#72444,#57432,#57433);
#51543=AXIS2_PLACEMENT_3D('',#72448,#57436,#57437);
#51544=AXIS2_PLACEMENT_3D('',#72452,#57440,#57441);
#51545=AXIS2_PLACEMENT_3D('',#72456,#57444,#57445);
#51546=AXIS2_PLACEMENT_3D('',#72460,#57448,#57449);
#51547=AXIS2_PLACEMENT_3D('',#72464,#57452,#57453);
#51548=AXIS2_PLACEMENT_3D('',#72468,#57456,#57457);
#51549=AXIS2_PLACEMENT_3D('',#72472,#57460,#57461);
#51550=AXIS2_PLACEMENT_3D('',#72476,#57463,#57464);
#51551=AXIS2_PLACEMENT_3D('',#72482,#57466,#57467);
#51552=AXIS2_PLACEMENT_3D('',#72486,#57469,#57470);
#51553=AXIS2_PLACEMENT_3D('',#72492,#57472,#57473);
#51554=AXIS2_PLACEMENT_3D('',#72496,#57475,#57476);
#51555=AXIS2_PLACEMENT_3D('',#72502,#57478,#57479);
#51556=AXIS2_PLACEMENT_3D('',#72506,#57481,#57482);
#51557=AXIS2_PLACEMENT_3D('',#72512,#57484,#57485);
#51558=AXIS2_PLACEMENT_3D('',#72516,#57487,#57488);
#51559=AXIS2_PLACEMENT_3D('',#72522,#57490,#57491);
#51560=AXIS2_PLACEMENT_3D('',#72526,#57493,#57494);
#51561=AXIS2_PLACEMENT_3D('',#72532,#57496,#57497);
#51562=AXIS2_PLACEMENT_3D('',#72536,#57499,#57500);
#51563=AXIS2_PLACEMENT_3D('',#72542,#57502,#57503);
#51564=AXIS2_PLACEMENT_3D('',#72546,#57505,#57506);
#51565=AXIS2_PLACEMENT_3D('',#72552,#57508,#57509);
#51566=AXIS2_PLACEMENT_3D('',#72556,#57511,#57512);
#51567=AXIS2_PLACEMENT_3D('',#72562,#57514,#57515);
#51568=AXIS2_PLACEMENT_3D('',#72566,#57517,#57518);
#51569=AXIS2_PLACEMENT_3D('',#72572,#57520,#57521);
#51570=AXIS2_PLACEMENT_3D('',#72576,#57523,#57524);
#51571=AXIS2_PLACEMENT_3D('',#72582,#57526,#57527);
#51572=AXIS2_PLACEMENT_3D('',#72586,#57529,#57530);
#51573=AXIS2_PLACEMENT_3D('',#72592,#57532,#57533);
#51574=AXIS2_PLACEMENT_3D('',#72596,#57535,#57536);
#51575=AXIS2_PLACEMENT_3D('',#72602,#57538,#57539);
#51576=AXIS2_PLACEMENT_3D('',#72606,#57541,#57542);
#51577=AXIS2_PLACEMENT_3D('',#72612,#57544,#57545);
#51578=AXIS2_PLACEMENT_3D('',#72616,#57547,#57548);
#51579=AXIS2_PLACEMENT_3D('',#72622,#57550,#57551);
#51580=AXIS2_PLACEMENT_3D('',#72626,#57553,#57554);
#51581=AXIS2_PLACEMENT_3D('',#72632,#57556,#57557);
#51582=AXIS2_PLACEMENT_3D('',#72636,#57559,#57560);
#51583=AXIS2_PLACEMENT_3D('',#72642,#57562,#57563);
#51584=AXIS2_PLACEMENT_3D('',#72646,#57565,#57566);
#51585=AXIS2_PLACEMENT_3D('',#72652,#57568,#57569);
#51586=AXIS2_PLACEMENT_3D('',#72656,#57571,#57572);
#51587=AXIS2_PLACEMENT_3D('',#72662,#57574,#57575);
#51588=AXIS2_PLACEMENT_3D('',#72666,#57577,#57578);
#51589=AXIS2_PLACEMENT_3D('',#72672,#57580,#57581);
#51590=AXIS2_PLACEMENT_3D('',#72676,#57583,#57584);
#51591=AXIS2_PLACEMENT_3D('',#72682,#57586,#57587);
#51592=AXIS2_PLACEMENT_3D('',#72686,#57589,#57590);
#51593=AXIS2_PLACEMENT_3D('',#72692,#57592,#57593);
#51594=AXIS2_PLACEMENT_3D('',#72696,#57595,#57596);
#51595=AXIS2_PLACEMENT_3D('',#72702,#57598,#57599);
#51596=AXIS2_PLACEMENT_3D('',#72706,#57601,#57602);
#51597=AXIS2_PLACEMENT_3D('',#72712,#57604,#57605);
#51598=AXIS2_PLACEMENT_3D('',#72716,#57607,#57608);
#51599=AXIS2_PLACEMENT_3D('',#72722,#57610,#57611);
#51600=AXIS2_PLACEMENT_3D('',#72726,#57613,#57614);
#51601=AXIS2_PLACEMENT_3D('',#72732,#57616,#57617);
#51602=AXIS2_PLACEMENT_3D('',#72736,#57619,#57620);
#51603=AXIS2_PLACEMENT_3D('',#72742,#57622,#57623);
#51604=AXIS2_PLACEMENT_3D('',#72746,#57625,#57626);
#51605=AXIS2_PLACEMENT_3D('',#72752,#57628,#57629);
#51606=AXIS2_PLACEMENT_3D('',#72756,#57631,#57632);
#51607=AXIS2_PLACEMENT_3D('',#72762,#57634,#57635);
#51608=AXIS2_PLACEMENT_3D('',#72766,#57637,#57638);
#51609=AXIS2_PLACEMENT_3D('',#72772,#57640,#57641);
#51610=AXIS2_PLACEMENT_3D('',#72776,#57643,#57644);
#51611=AXIS2_PLACEMENT_3D('',#72782,#57646,#57647);
#51612=AXIS2_PLACEMENT_3D('',#72786,#57649,#57650);
#51613=AXIS2_PLACEMENT_3D('',#72792,#57652,#57653);
#51614=AXIS2_PLACEMENT_3D('',#72796,#57655,#57656);
#51615=AXIS2_PLACEMENT_3D('',#72802,#57658,#57659);
#51616=AXIS2_PLACEMENT_3D('',#72806,#57661,#57662);
#51617=AXIS2_PLACEMENT_3D('',#72812,#57664,#57665);
#51618=AXIS2_PLACEMENT_3D('',#72816,#57667,#57668);
#51619=AXIS2_PLACEMENT_3D('',#72822,#57670,#57671);
#51620=AXIS2_PLACEMENT_3D('',#72828,#57673,#57674);
#51621=AXIS2_PLACEMENT_3D('',#72832,#57677,#57678);
#51622=AXIS2_PLACEMENT_3D('',#72836,#57681,#57682);
#51623=AXIS2_PLACEMENT_3D('',#72840,#57685,#57686);
#51624=AXIS2_PLACEMENT_3D('',#72844,#57689,#57690);
#51625=AXIS2_PLACEMENT_3D('',#72848,#57693,#57694);
#51626=AXIS2_PLACEMENT_3D('',#72852,#57697,#57698);
#51627=AXIS2_PLACEMENT_3D('',#72856,#57701,#57702);
#51628=AXIS2_PLACEMENT_3D('',#72860,#57705,#57706);
#51629=AXIS2_PLACEMENT_3D('',#72864,#57709,#57710);
#51630=AXIS2_PLACEMENT_3D('',#72868,#57713,#57714);
#51631=AXIS2_PLACEMENT_3D('',#72872,#57717,#57718);
#51632=AXIS2_PLACEMENT_3D('',#72876,#57721,#57722);
#51633=AXIS2_PLACEMENT_3D('',#72880,#57725,#57726);
#51634=AXIS2_PLACEMENT_3D('',#72884,#57729,#57730);
#51635=AXIS2_PLACEMENT_3D('',#72888,#57733,#57734);
#51636=AXIS2_PLACEMENT_3D('',#72892,#57737,#57738);
#51637=AXIS2_PLACEMENT_3D('',#72896,#57741,#57742);
#51638=AXIS2_PLACEMENT_3D('',#72900,#57745,#57746);
#51639=AXIS2_PLACEMENT_3D('',#72904,#57749,#57750);
#51640=AXIS2_PLACEMENT_3D('',#72908,#57753,#57754);
#51641=AXIS2_PLACEMENT_3D('',#72912,#57757,#57758);
#51642=AXIS2_PLACEMENT_3D('',#72916,#57761,#57762);
#51643=AXIS2_PLACEMENT_3D('',#72920,#57765,#57766);
#51644=AXIS2_PLACEMENT_3D('',#72924,#57769,#57770);
#51645=AXIS2_PLACEMENT_3D('',#72928,#57773,#57774);
#51646=AXIS2_PLACEMENT_3D('',#72932,#57777,#57778);
#51647=AXIS2_PLACEMENT_3D('',#72936,#57781,#57782);
#51648=AXIS2_PLACEMENT_3D('',#72940,#57785,#57786);
#51649=AXIS2_PLACEMENT_3D('',#72944,#57789,#57790);
#51650=AXIS2_PLACEMENT_3D('',#72948,#57793,#57794);
#51651=AXIS2_PLACEMENT_3D('',#72952,#57797,#57798);
#51652=AXIS2_PLACEMENT_3D('',#72956,#57801,#57802);
#51653=AXIS2_PLACEMENT_3D('',#72960,#57805,#57806);
#51654=AXIS2_PLACEMENT_3D('',#72964,#57809,#57810);
#51655=AXIS2_PLACEMENT_3D('',#72968,#57813,#57814);
#51656=AXIS2_PLACEMENT_3D('',#72972,#57817,#57818);
#51657=AXIS2_PLACEMENT_3D('',#72978,#57820,#57821);
#51658=AXIS2_PLACEMENT_3D('',#72984,#57823,#57824);
#51659=AXIS2_PLACEMENT_3D('',#72990,#57826,#57827);
#51660=AXIS2_PLACEMENT_3D('',#72996,#57829,#57830);
#51661=AXIS2_PLACEMENT_3D('',#73002,#57832,#57833);
#51662=AXIS2_PLACEMENT_3D('',#73008,#57835,#57836);
#51663=AXIS2_PLACEMENT_3D('',#73014,#57838,#57839);
#51664=AXIS2_PLACEMENT_3D('',#73020,#57841,#57842);
#51665=AXIS2_PLACEMENT_3D('',#73026,#57844,#57845);
#51666=AXIS2_PLACEMENT_3D('',#73032,#57847,#57848);
#51667=AXIS2_PLACEMENT_3D('',#73038,#57850,#57851);
#51668=AXIS2_PLACEMENT_3D('',#73044,#57853,#57854);
#51669=AXIS2_PLACEMENT_3D('',#73050,#57856,#57857);
#51670=AXIS2_PLACEMENT_3D('',#73056,#57859,#57860);
#51671=AXIS2_PLACEMENT_3D('',#73062,#57862,#57863);
#51672=AXIS2_PLACEMENT_3D('',#73068,#57865,#57866);
#51673=AXIS2_PLACEMENT_3D('',#73074,#57868,#57869);
#51674=AXIS2_PLACEMENT_3D('',#73084,#57871,#57872);
#51675=AXIS2_PLACEMENT_3D('',#73090,#57874,#57875);
#51676=AXIS2_PLACEMENT_3D('',#73096,#57877,#57878);
#51677=AXIS2_PLACEMENT_3D('',#73102,#57880,#57881);
#51678=AXIS2_PLACEMENT_3D('',#73108,#57883,#57884);
#51679=AXIS2_PLACEMENT_3D('',#73114,#57886,#57887);
#51680=AXIS2_PLACEMENT_3D('',#73120,#57889,#57890);
#51681=AXIS2_PLACEMENT_3D('',#73126,#57892,#57893);
#51682=AXIS2_PLACEMENT_3D('',#73132,#57895,#57896);
#51683=AXIS2_PLACEMENT_3D('',#73138,#57898,#57899);
#51684=AXIS2_PLACEMENT_3D('',#73144,#57901,#57902);
#51685=AXIS2_PLACEMENT_3D('',#73150,#57904,#57905);
#51686=AXIS2_PLACEMENT_3D('',#73156,#57907,#57908);
#51687=AXIS2_PLACEMENT_3D('',#73162,#57910,#57911);
#51688=AXIS2_PLACEMENT_3D('',#73168,#57913,#57914);
#51689=AXIS2_PLACEMENT_3D('',#73174,#57916,#57917);
#51690=AXIS2_PLACEMENT_3D('',#73180,#57919,#57920);
#51691=AXIS2_PLACEMENT_3D('',#73186,#57922,#57923);
#51692=AXIS2_PLACEMENT_3D('',#73192,#57925,#57926);
#51693=AXIS2_PLACEMENT_3D('',#73196,#57929,#57930);
#51694=AXIS2_PLACEMENT_3D('',#73198,#57931,#57932);
#51695=AXIS2_PLACEMENT_3D('',#73200,#57934,#57935);
#51696=AXIS2_PLACEMENT_3D('',#73202,#57936,#57937);
#51697=AXIS2_PLACEMENT_3D('',#73204,#57939,#57940);
#51698=AXIS2_PLACEMENT_3D('',#73206,#57941,#57942);
#51699=AXIS2_PLACEMENT_3D('',#73208,#57944,#57945);
#51700=AXIS2_PLACEMENT_3D('',#73210,#57946,#57947);
#51701=AXIS2_PLACEMENT_3D('',#73212,#57949,#57950);
#51702=AXIS2_PLACEMENT_3D('',#73214,#57951,#57952);
#51703=AXIS2_PLACEMENT_3D('',#73216,#57954,#57955);
#51704=AXIS2_PLACEMENT_3D('',#73220,#57958,#57959);
#51705=AXIS2_PLACEMENT_3D('',#73222,#57960,#57961);
#51706=AXIS2_PLACEMENT_3D('',#73224,#57963,#57964);
#51707=AXIS2_PLACEMENT_3D('',#73226,#57965,#57966);
#51708=AXIS2_PLACEMENT_3D('',#73228,#57968,#57969);
#51709=AXIS2_PLACEMENT_3D('',#73230,#57970,#57971);
#51710=AXIS2_PLACEMENT_3D('',#73232,#57973,#57974);
#51711=AXIS2_PLACEMENT_3D('',#73234,#57975,#57976);
#51712=AXIS2_PLACEMENT_3D('',#73236,#57978,#57979);
#51713=AXIS2_PLACEMENT_3D('',#73238,#57980,#57981);
#51714=AXIS2_PLACEMENT_3D('',#73240,#57983,#57984);
#51715=AXIS2_PLACEMENT_3D('',#73244,#57987,#57988);
#51716=AXIS2_PLACEMENT_3D('',#73246,#57989,#57990);
#51717=AXIS2_PLACEMENT_3D('',#73250,#57991,#57992);
#51718=AXIS2_PLACEMENT_3D('',#73254,#57995,#57996);
#51719=AXIS2_PLACEMENT_3D('',#73256,#57997,#57998);
#51720=AXIS2_PLACEMENT_3D('',#73258,#58000,#58001);
#51721=AXIS2_PLACEMENT_3D('',#73260,#58002,#58003);
#51722=AXIS2_PLACEMENT_3D('',#73262,#58005,#58006);
#51723=AXIS2_PLACEMENT_3D('',#73264,#58007,#58008);
#51724=AXIS2_PLACEMENT_3D('',#73266,#58010,#58011);
#51725=AXIS2_PLACEMENT_3D('',#73268,#58012,#58013);
#51726=AXIS2_PLACEMENT_3D('',#73270,#58015,#58016);
#51727=AXIS2_PLACEMENT_3D('',#73272,#58017,#58018);
#51728=AXIS2_PLACEMENT_3D('',#73274,#58020,#58021);
#51729=AXIS2_PLACEMENT_3D('',#73278,#58024,#58025);
#51730=AXIS2_PLACEMENT_3D('',#73280,#58026,#58027);
#51731=AXIS2_PLACEMENT_3D('',#73282,#58029,#58030);
#51732=AXIS2_PLACEMENT_3D('',#73284,#58031,#58032);
#51733=AXIS2_PLACEMENT_3D('',#73286,#58034,#58035);
#51734=AXIS2_PLACEMENT_3D('',#73288,#58036,#58037);
#51735=AXIS2_PLACEMENT_3D('',#73290,#58039,#58040);
#51736=AXIS2_PLACEMENT_3D('',#73292,#58041,#58042);
#51737=AXIS2_PLACEMENT_3D('',#73294,#58044,#58045);
#51738=AXIS2_PLACEMENT_3D('',#73296,#58046,#58047);
#51739=AXIS2_PLACEMENT_3D('',#73298,#58049,#58050);
#51740=AXIS2_PLACEMENT_3D('',#73300,#58052,#58053);
#51741=AXIS2_PLACEMENT_3D('',#73304,#58054,#58055);
#51742=AXIS2_PLACEMENT_3D('',#73306,#58056,#58057);
#51743=AXIS2_PLACEMENT_3D('',#73312,#58059,#58060);
#51744=AXIS2_PLACEMENT_3D('',#73316,#58061,#58062);
#51745=AXIS2_PLACEMENT_3D('',#73320,#58063,#58064);
#51746=AXIS2_PLACEMENT_3D('',#73324,#58065,#58066);
#51747=AXIS2_PLACEMENT_3D('',#73328,#58067,#58068);
#51748=AXIS2_PLACEMENT_3D('',#73332,#58069,#58070);
#51749=AXIS2_PLACEMENT_3D('',#73336,#58071,#58072);
#51750=AXIS2_PLACEMENT_3D('',#73340,#58073,#58074);
#51751=AXIS2_PLACEMENT_3D('',#73344,#58075,#58076);
#51752=AXIS2_PLACEMENT_3D('',#73348,#58077,#58078);
#51753=AXIS2_PLACEMENT_3D('',#73352,#58079,#58080);
#51754=AXIS2_PLACEMENT_3D('',#73356,#58081,#58082);
#51755=AXIS2_PLACEMENT_3D('',#73360,#58083,#58084);
#51756=AXIS2_PLACEMENT_3D('',#73364,#58085,#58086);
#51757=AXIS2_PLACEMENT_3D('',#73368,#58087,#58088);
#51758=AXIS2_PLACEMENT_3D('',#73372,#58089,#58090);
#51759=AXIS2_PLACEMENT_3D('',#73376,#58091,#58092);
#51760=AXIS2_PLACEMENT_3D('',#73380,#58093,#58094);
#51761=AXIS2_PLACEMENT_3D('',#73385,#58095,#58096);
#51762=AXIS2_PLACEMENT_3D('',#73386,#58097,#58098);
#51763=AXIS2_PLACEMENT_3D('',#73390,#58099,#58100);
#51764=AXIS2_PLACEMENT_3D('',#73394,#58101,#58102);
#51765=AXIS2_PLACEMENT_3D('',#73398,#58103,#58104);
#51766=AXIS2_PLACEMENT_3D('',#73402,#58105,#58106);
#51767=AXIS2_PLACEMENT_3D('',#73406,#58107,#58108);
#51768=AXIS2_PLACEMENT_3D('',#73410,#58109,#58110);
#51769=AXIS2_PLACEMENT_3D('',#73414,#58111,#58112);
#51770=AXIS2_PLACEMENT_3D('',#73418,#58113,#58114);
#51771=AXIS2_PLACEMENT_3D('',#73422,#58115,#58116);
#51772=AXIS2_PLACEMENT_3D('',#73426,#58117,#58118);
#51773=AXIS2_PLACEMENT_3D('',#73430,#58119,#58120);
#51774=AXIS2_PLACEMENT_3D('',#73434,#58121,#58122);
#51775=AXIS2_PLACEMENT_3D('',#73438,#58123,#58124);
#51776=AXIS2_PLACEMENT_3D('',#73442,#58125,#58126);
#51777=AXIS2_PLACEMENT_3D('',#73446,#58127,#58128);
#51778=AXIS2_PLACEMENT_3D('',#73450,#58129,#58130);
#51779=AXIS2_PLACEMENT_3D('',#73454,#58131,#58132);
#51780=AXIS2_PLACEMENT_3D('',#73456,#58133,#58134);
#51781=AXIS2_PLACEMENT_3D('',#73458,#58135,#58136);
#51782=AXIS2_PLACEMENT_3D('',#73462,#58138,#58139);
#51783=AXIS2_PLACEMENT_3D('',#73464,#58140,#58141);
#51784=AXIS2_PLACEMENT_3D('',#73466,#58142,#58143);
#51785=AXIS2_PLACEMENT_3D('',#73468,#58144,#58145);
#51786=AXIS2_PLACEMENT_3D('',#73470,#58146,#58147);
#51787=AXIS2_PLACEMENT_3D('',#73474,#58149,#58150);
#51788=AXIS2_PLACEMENT_3D('',#73476,#58151,#58152);
#51789=AXIS2_PLACEMENT_3D('',#73478,#58153,#58154);
#51790=AXIS2_PLACEMENT_3D('',#73480,#58155,#58156);
#51791=AXIS2_PLACEMENT_3D('',#73482,#58157,#58158);
#51792=AXIS2_PLACEMENT_3D('',#73484,#58160,#58161);
#51793=AXIS2_PLACEMENT_3D('',#73486,#58163,#58164);
#51794=AXIS2_PLACEMENT_3D('',#73488,#58166,#58167);
#51795=AXIS2_PLACEMENT_3D('',#73490,#58169,#58170);
#51796=AXIS2_PLACEMENT_3D('',#73492,#58172,#58173);
#51797=AXIS2_PLACEMENT_3D('',#73494,#58175,#58176);
#51798=AXIS2_PLACEMENT_3D('',#73496,#58178,#58179);
#51799=AXIS2_PLACEMENT_3D('',#73498,#58181,#58182);
#51800=AXIS2_PLACEMENT_3D('',#73500,#58184,#58185);
#51801=AXIS2_PLACEMENT_3D('',#73502,#58187,#58188);
#51802=AXIS2_PLACEMENT_3D('',#73504,#58190,#58191);
#51803=AXIS2_PLACEMENT_3D('',#73506,#58193,#58194);
#51804=AXIS2_PLACEMENT_3D('',#73508,#58196,#58197);
#51805=AXIS2_PLACEMENT_3D('',#73510,#58199,#58200);
#51806=AXIS2_PLACEMENT_3D('',#73514,#58201,#58202);
#51807=AXIS2_PLACEMENT_3D('',#73518,#58205,#58206);
#51808=AXIS2_PLACEMENT_3D('',#73520,#58207,#58208);
#51809=AXIS2_PLACEMENT_3D('',#73522,#58210,#58211);
#51810=AXIS2_PLACEMENT_3D('',#73524,#58212,#58213);
#51811=AXIS2_PLACEMENT_3D('',#73526,#58215,#58216);
#51812=AXIS2_PLACEMENT_3D('',#73528,#58217,#58218);
#51813=AXIS2_PLACEMENT_3D('',#73530,#58220,#58221);
#51814=AXIS2_PLACEMENT_3D('',#73532,#58222,#58223);
#51815=AXIS2_PLACEMENT_3D('',#73534,#58225,#58226);
#51816=AXIS2_PLACEMENT_3D('',#73536,#58227,#58228);
#51817=AXIS2_PLACEMENT_3D('',#73538,#58230,#58231);
#51818=AXIS2_PLACEMENT_3D('',#73542,#58234,#58235);
#51819=AXIS2_PLACEMENT_3D('',#73544,#58236,#58237);
#51820=AXIS2_PLACEMENT_3D('',#73546,#58239,#58240);
#51821=AXIS2_PLACEMENT_3D('',#73548,#58241,#58242);
#51822=AXIS2_PLACEMENT_3D('',#73550,#58244,#58245);
#51823=AXIS2_PLACEMENT_3D('',#73552,#58246,#58247);
#51824=AXIS2_PLACEMENT_3D('',#73554,#58249,#58250);
#51825=AXIS2_PLACEMENT_3D('',#73556,#58251,#58252);
#51826=AXIS2_PLACEMENT_3D('',#73558,#58254,#58255);
#51827=AXIS2_PLACEMENT_3D('',#73560,#58256,#58257);
#51828=AXIS2_PLACEMENT_3D('',#73562,#58259,#58260);
#51829=AXIS2_PLACEMENT_3D('',#73564,#58262,#58263);
#51830=AXIS2_PLACEMENT_3D('',#73565,#58264,#58265);
#51831=AXIS2_PLACEMENT_3D('',#73567,#58266,#58267);
#51832=AXIS2_PLACEMENT_3D('',#73569,#58268,#58269);
#51833=AXIS2_PLACEMENT_3D('',#73573,#58271,#58272);
#51834=AXIS2_PLACEMENT_3D('',#73575,#58273,#58274);
#51835=AXIS2_PLACEMENT_3D('',#73577,#58275,#58276);
#51836=AXIS2_PLACEMENT_3D('',#73579,#58277,#58278);
#51837=AXIS2_PLACEMENT_3D('',#73581,#58279,#58280);
#51838=AXIS2_PLACEMENT_3D('',#73585,#58282,#58283);
#51839=AXIS2_PLACEMENT_3D('',#73587,#58284,#58285);
#51840=AXIS2_PLACEMENT_3D('',#73589,#58286,#58287);
#51841=AXIS2_PLACEMENT_3D('',#73591,#58288,#58289);
#51842=AXIS2_PLACEMENT_3D('',#73593,#58290,#58291);
#51843=AXIS2_PLACEMENT_3D('',#73595,#58293,#58294);
#51844=AXIS2_PLACEMENT_3D('',#73597,#58296,#58297);
#51845=AXIS2_PLACEMENT_3D('',#73599,#58299,#58300);
#51846=AXIS2_PLACEMENT_3D('',#73601,#58302,#58303);
#51847=AXIS2_PLACEMENT_3D('',#73603,#58305,#58306);
#51848=AXIS2_PLACEMENT_3D('',#73605,#58308,#58309);
#51849=AXIS2_PLACEMENT_3D('',#73607,#58311,#58312);
#51850=AXIS2_PLACEMENT_3D('',#73609,#58314,#58315);
#51851=AXIS2_PLACEMENT_3D('',#73611,#58317,#58318);
#51852=AXIS2_PLACEMENT_3D('',#73613,#58320,#58321);
#51853=AXIS2_PLACEMENT_3D('',#73615,#58323,#58324);
#51854=AXIS2_PLACEMENT_3D('',#73617,#58326,#58327);
#51855=AXIS2_PLACEMENT_3D('',#73619,#58329,#58330);
#51856=AXIS2_PLACEMENT_3D('',#73621,#58332,#58333);
#51857=AXIS2_PLACEMENT_3D('',#73625,#58334,#58335);
#51858=AXIS2_PLACEMENT_3D('',#73629,#58338,#58339);
#51859=AXIS2_PLACEMENT_3D('',#73631,#58340,#58341);
#51860=AXIS2_PLACEMENT_3D('',#73633,#58343,#58344);
#51861=AXIS2_PLACEMENT_3D('',#73635,#58345,#58346);
#51862=AXIS2_PLACEMENT_3D('',#73637,#58348,#58349);
#51863=AXIS2_PLACEMENT_3D('',#73639,#58350,#58351);
#51864=AXIS2_PLACEMENT_3D('',#73641,#58353,#58354);
#51865=AXIS2_PLACEMENT_3D('',#73643,#58355,#58356);
#51866=AXIS2_PLACEMENT_3D('',#73645,#58358,#58359);
#51867=AXIS2_PLACEMENT_3D('',#73647,#58360,#58361);
#51868=AXIS2_PLACEMENT_3D('',#73649,#58363,#58364);
#51869=AXIS2_PLACEMENT_3D('',#73653,#58367,#58368);
#51870=AXIS2_PLACEMENT_3D('',#73655,#58369,#58370);
#51871=AXIS2_PLACEMENT_3D('',#73657,#58372,#58373);
#51872=AXIS2_PLACEMENT_3D('',#73659,#58374,#58375);
#51873=AXIS2_PLACEMENT_3D('',#73661,#58377,#58378);
#51874=AXIS2_PLACEMENT_3D('',#73663,#58379,#58380);
#51875=AXIS2_PLACEMENT_3D('',#73665,#58382,#58383);
#51876=AXIS2_PLACEMENT_3D('',#73667,#58384,#58385);
#51877=AXIS2_PLACEMENT_3D('',#73669,#58387,#58388);
#51878=AXIS2_PLACEMENT_3D('',#73671,#58389,#58390);
#51879=AXIS2_PLACEMENT_3D('',#73673,#58392,#58393);
#51880=AXIS2_PLACEMENT_3D('',#73675,#58395,#58396);
#51881=AXIS2_PLACEMENT_3D('',#73676,#58397,#58398);
#51882=AXIS2_PLACEMENT_3D('',#73678,#58399,#58400);
#51883=AXIS2_PLACEMENT_3D('',#73680,#58401,#58402);
#51884=AXIS2_PLACEMENT_3D('',#73684,#58404,#58405);
#51885=AXIS2_PLACEMENT_3D('',#73686,#58406,#58407);
#51886=AXIS2_PLACEMENT_3D('',#73688,#58408,#58409);
#51887=AXIS2_PLACEMENT_3D('',#73690,#58410,#58411);
#51888=AXIS2_PLACEMENT_3D('',#73692,#58412,#58413);
#51889=AXIS2_PLACEMENT_3D('',#73696,#58415,#58416);
#51890=AXIS2_PLACEMENT_3D('',#73698,#58417,#58418);
#51891=AXIS2_PLACEMENT_3D('',#73700,#58419,#58420);
#51892=AXIS2_PLACEMENT_3D('',#73702,#58421,#58422);
#51893=AXIS2_PLACEMENT_3D('',#73704,#58423,#58424);
#51894=AXIS2_PLACEMENT_3D('',#73706,#58426,#58427);
#51895=AXIS2_PLACEMENT_3D('',#73708,#58429,#58430);
#51896=AXIS2_PLACEMENT_3D('',#73710,#58432,#58433);
#51897=AXIS2_PLACEMENT_3D('',#73712,#58435,#58436);
#51898=AXIS2_PLACEMENT_3D('',#73714,#58438,#58439);
#51899=AXIS2_PLACEMENT_3D('',#73716,#58441,#58442);
#51900=AXIS2_PLACEMENT_3D('',#73718,#58444,#58445);
#51901=AXIS2_PLACEMENT_3D('',#73720,#58447,#58448);
#51902=AXIS2_PLACEMENT_3D('',#73722,#58450,#58451);
#51903=AXIS2_PLACEMENT_3D('',#73724,#58453,#58454);
#51904=AXIS2_PLACEMENT_3D('',#73726,#58456,#58457);
#51905=AXIS2_PLACEMENT_3D('',#73728,#58459,#58460);
#51906=AXIS2_PLACEMENT_3D('',#73730,#58462,#58463);
#51907=AXIS2_PLACEMENT_3D('',#73732,#58465,#58466);
#51908=AXIS2_PLACEMENT_3D('',#73736,#58467,#58468);
#51909=AXIS2_PLACEMENT_3D('',#73740,#58471,#58472);
#51910=AXIS2_PLACEMENT_3D('',#73742,#58473,#58474);
#51911=AXIS2_PLACEMENT_3D('',#73744,#58476,#58477);
#51912=AXIS2_PLACEMENT_3D('',#73746,#58478,#58479);
#51913=AXIS2_PLACEMENT_3D('',#73748,#58481,#58482);
#51914=AXIS2_PLACEMENT_3D('',#73750,#58483,#58484);
#51915=AXIS2_PLACEMENT_3D('',#73752,#58486,#58487);
#51916=AXIS2_PLACEMENT_3D('',#73754,#58488,#58489);
#51917=AXIS2_PLACEMENT_3D('',#73756,#58491,#58492);
#51918=AXIS2_PLACEMENT_3D('',#73758,#58493,#58494);
#51919=AXIS2_PLACEMENT_3D('',#73760,#58496,#58497);
#51920=AXIS2_PLACEMENT_3D('',#73764,#58500,#58501);
#51921=AXIS2_PLACEMENT_3D('',#73766,#58502,#58503);
#51922=AXIS2_PLACEMENT_3D('',#73768,#58505,#58506);
#51923=AXIS2_PLACEMENT_3D('',#73770,#58507,#58508);
#51924=AXIS2_PLACEMENT_3D('',#73772,#58510,#58511);
#51925=AXIS2_PLACEMENT_3D('',#73774,#58512,#58513);
#51926=AXIS2_PLACEMENT_3D('',#73776,#58515,#58516);
#51927=AXIS2_PLACEMENT_3D('',#73778,#58517,#58518);
#51928=AXIS2_PLACEMENT_3D('',#73780,#58520,#58521);
#51929=AXIS2_PLACEMENT_3D('',#73782,#58522,#58523);
#51930=AXIS2_PLACEMENT_3D('',#73784,#58525,#58526);
#51931=AXIS2_PLACEMENT_3D('',#73786,#58528,#58529);
#51932=AXIS2_PLACEMENT_3D('',#73787,#58530,#58531);
#51933=AXIS2_PLACEMENT_3D('',#73789,#58532,#58533);
#51934=AXIS2_PLACEMENT_3D('',#73791,#58534,#58535);
#51935=AXIS2_PLACEMENT_3D('',#73795,#58537,#58538);
#51936=AXIS2_PLACEMENT_3D('',#73797,#58539,#58540);
#51937=AXIS2_PLACEMENT_3D('',#73799,#58541,#58542);
#51938=AXIS2_PLACEMENT_3D('',#73801,#58543,#58544);
#51939=AXIS2_PLACEMENT_3D('',#73803,#58545,#58546);
#51940=AXIS2_PLACEMENT_3D('',#73807,#58548,#58549);
#51941=AXIS2_PLACEMENT_3D('',#73809,#58550,#58551);
#51942=AXIS2_PLACEMENT_3D('',#73811,#58552,#58553);
#51943=AXIS2_PLACEMENT_3D('',#73813,#58554,#58555);
#51944=AXIS2_PLACEMENT_3D('',#73815,#58556,#58557);
#51945=AXIS2_PLACEMENT_3D('',#73817,#58559,#58560);
#51946=AXIS2_PLACEMENT_3D('',#73819,#58562,#58563);
#51947=AXIS2_PLACEMENT_3D('',#73821,#58565,#58566);
#51948=AXIS2_PLACEMENT_3D('',#73823,#58568,#58569);
#51949=AXIS2_PLACEMENT_3D('',#73825,#58571,#58572);
#51950=AXIS2_PLACEMENT_3D('',#73827,#58574,#58575);
#51951=AXIS2_PLACEMENT_3D('',#73829,#58577,#58578);
#51952=AXIS2_PLACEMENT_3D('',#73831,#58580,#58581);
#51953=AXIS2_PLACEMENT_3D('',#73833,#58583,#58584);
#51954=AXIS2_PLACEMENT_3D('',#73835,#58586,#58587);
#51955=AXIS2_PLACEMENT_3D('',#73837,#58589,#58590);
#51956=AXIS2_PLACEMENT_3D('',#73839,#58592,#58593);
#51957=AXIS2_PLACEMENT_3D('',#73841,#58595,#58596);
#51958=AXIS2_PLACEMENT_3D('',#73843,#58598,#58599);
#51959=AXIS2_PLACEMENT_3D('',#73847,#58600,#58601);
#51960=AXIS2_PLACEMENT_3D('',#73851,#58604,#58605);
#51961=AXIS2_PLACEMENT_3D('',#73853,#58606,#58607);
#51962=AXIS2_PLACEMENT_3D('',#73855,#58609,#58610);
#51963=AXIS2_PLACEMENT_3D('',#73857,#58611,#58612);
#51964=AXIS2_PLACEMENT_3D('',#73859,#58614,#58615);
#51965=AXIS2_PLACEMENT_3D('',#73861,#58616,#58617);
#51966=AXIS2_PLACEMENT_3D('',#73863,#58619,#58620);
#51967=AXIS2_PLACEMENT_3D('',#73865,#58621,#58622);
#51968=AXIS2_PLACEMENT_3D('',#73867,#58624,#58625);
#51969=AXIS2_PLACEMENT_3D('',#73869,#58626,#58627);
#51970=AXIS2_PLACEMENT_3D('',#73871,#58629,#58630);
#51971=AXIS2_PLACEMENT_3D('',#73875,#58633,#58634);
#51972=AXIS2_PLACEMENT_3D('',#73877,#58635,#58636);
#51973=AXIS2_PLACEMENT_3D('',#73879,#58638,#58639);
#51974=AXIS2_PLACEMENT_3D('',#73881,#58640,#58641);
#51975=AXIS2_PLACEMENT_3D('',#73883,#58643,#58644);
#51976=AXIS2_PLACEMENT_3D('',#73885,#58645,#58646);
#51977=AXIS2_PLACEMENT_3D('',#73887,#58648,#58649);
#51978=AXIS2_PLACEMENT_3D('',#73889,#58650,#58651);
#51979=AXIS2_PLACEMENT_3D('',#73891,#58653,#58654);
#51980=AXIS2_PLACEMENT_3D('',#73893,#58655,#58656);
#51981=AXIS2_PLACEMENT_3D('',#73895,#58658,#58659);
#51982=AXIS2_PLACEMENT_3D('',#73897,#58661,#58662);
#51983=AXIS2_PLACEMENT_3D('',#73898,#58663,#58664);
#51984=AXIS2_PLACEMENT_3D('',#73900,#58665,#58666);
#51985=AXIS2_PLACEMENT_3D('',#73902,#58667,#58668);
#51986=AXIS2_PLACEMENT_3D('',#73906,#58670,#58671);
#51987=AXIS2_PLACEMENT_3D('',#73908,#58672,#58673);
#51988=AXIS2_PLACEMENT_3D('',#73910,#58674,#58675);
#51989=AXIS2_PLACEMENT_3D('',#73912,#58676,#58677);
#51990=AXIS2_PLACEMENT_3D('',#73914,#58678,#58679);
#51991=AXIS2_PLACEMENT_3D('',#73918,#58681,#58682);
#51992=AXIS2_PLACEMENT_3D('',#73920,#58683,#58684);
#51993=AXIS2_PLACEMENT_3D('',#73922,#58685,#58686);
#51994=AXIS2_PLACEMENT_3D('',#73924,#58687,#58688);
#51995=AXIS2_PLACEMENT_3D('',#73926,#58689,#58690);
#51996=AXIS2_PLACEMENT_3D('',#73928,#58692,#58693);
#51997=AXIS2_PLACEMENT_3D('',#73930,#58695,#58696);
#51998=AXIS2_PLACEMENT_3D('',#73932,#58698,#58699);
#51999=AXIS2_PLACEMENT_3D('',#73934,#58701,#58702);
#52000=AXIS2_PLACEMENT_3D('',#73936,#58704,#58705);
#52001=AXIS2_PLACEMENT_3D('',#73938,#58707,#58708);
#52002=AXIS2_PLACEMENT_3D('',#73940,#58710,#58711);
#52003=AXIS2_PLACEMENT_3D('',#73942,#58713,#58714);
#52004=AXIS2_PLACEMENT_3D('',#73944,#58716,#58717);
#52005=AXIS2_PLACEMENT_3D('',#73946,#58719,#58720);
#52006=AXIS2_PLACEMENT_3D('',#73948,#58722,#58723);
#52007=AXIS2_PLACEMENT_3D('',#73950,#58725,#58726);
#52008=AXIS2_PLACEMENT_3D('',#73952,#58728,#58729);
#52009=AXIS2_PLACEMENT_3D('',#73954,#58731,#58732);
#52010=AXIS2_PLACEMENT_3D('',#73958,#58733,#58734);
#52011=AXIS2_PLACEMENT_3D('',#73962,#58737,#58738);
#52012=AXIS2_PLACEMENT_3D('',#73964,#58739,#58740);
#52013=AXIS2_PLACEMENT_3D('',#73966,#58742,#58743);
#52014=AXIS2_PLACEMENT_3D('',#73968,#58744,#58745);
#52015=AXIS2_PLACEMENT_3D('',#73970,#58747,#58748);
#52016=AXIS2_PLACEMENT_3D('',#73972,#58749,#58750);
#52017=AXIS2_PLACEMENT_3D('',#73974,#58752,#58753);
#52018=AXIS2_PLACEMENT_3D('',#73976,#58754,#58755);
#52019=AXIS2_PLACEMENT_3D('',#73978,#58757,#58758);
#52020=AXIS2_PLACEMENT_3D('',#73980,#58759,#58760);
#52021=AXIS2_PLACEMENT_3D('',#73982,#58762,#58763);
#52022=AXIS2_PLACEMENT_3D('',#73986,#58766,#58767);
#52023=AXIS2_PLACEMENT_3D('',#73988,#58768,#58769);
#52024=AXIS2_PLACEMENT_3D('',#73990,#58771,#58772);
#52025=AXIS2_PLACEMENT_3D('',#73992,#58773,#58774);
#52026=AXIS2_PLACEMENT_3D('',#73994,#58776,#58777);
#52027=AXIS2_PLACEMENT_3D('',#73996,#58778,#58779);
#52028=AXIS2_PLACEMENT_3D('',#73998,#58781,#58782);
#52029=AXIS2_PLACEMENT_3D('',#74000,#58783,#58784);
#52030=AXIS2_PLACEMENT_3D('',#74002,#58786,#58787);
#52031=AXIS2_PLACEMENT_3D('',#74004,#58788,#58789);
#52032=AXIS2_PLACEMENT_3D('',#74006,#58791,#58792);
#52033=AXIS2_PLACEMENT_3D('',#74008,#58794,#58795);
#52034=AXIS2_PLACEMENT_3D('',#74009,#58796,#58797);
#52035=AXIS2_PLACEMENT_3D('',#74011,#58798,#58799);
#52036=AXIS2_PLACEMENT_3D('',#74013,#58800,#58801);
#52037=AXIS2_PLACEMENT_3D('',#74017,#58803,#58804);
#52038=AXIS2_PLACEMENT_3D('',#74019,#58805,#58806);
#52039=AXIS2_PLACEMENT_3D('',#74021,#58807,#58808);
#52040=AXIS2_PLACEMENT_3D('',#74023,#58809,#58810);
#52041=AXIS2_PLACEMENT_3D('',#74025,#58811,#58812);
#52042=AXIS2_PLACEMENT_3D('',#74029,#58814,#58815);
#52043=AXIS2_PLACEMENT_3D('',#74031,#58816,#58817);
#52044=AXIS2_PLACEMENT_3D('',#74033,#58818,#58819);
#52045=AXIS2_PLACEMENT_3D('',#74035,#58820,#58821);
#52046=AXIS2_PLACEMENT_3D('',#74037,#58822,#58823);
#52047=AXIS2_PLACEMENT_3D('',#74039,#58825,#58826);
#52048=AXIS2_PLACEMENT_3D('',#74041,#58828,#58829);
#52049=AXIS2_PLACEMENT_3D('',#74043,#58831,#58832);
#52050=AXIS2_PLACEMENT_3D('',#74045,#58834,#58835);
#52051=AXIS2_PLACEMENT_3D('',#74047,#58837,#58838);
#52052=AXIS2_PLACEMENT_3D('',#74049,#58840,#58841);
#52053=AXIS2_PLACEMENT_3D('',#74051,#58843,#58844);
#52054=AXIS2_PLACEMENT_3D('',#74053,#58846,#58847);
#52055=AXIS2_PLACEMENT_3D('',#74055,#58849,#58850);
#52056=AXIS2_PLACEMENT_3D('',#74057,#58852,#58853);
#52057=AXIS2_PLACEMENT_3D('',#74059,#58855,#58856);
#52058=AXIS2_PLACEMENT_3D('',#74061,#58858,#58859);
#52059=AXIS2_PLACEMENT_3D('',#74063,#58861,#58862);
#52060=AXIS2_PLACEMENT_3D('',#74065,#58864,#58865);
#52061=AXIS2_PLACEMENT_3D('',#74069,#58866,#58867);
#52062=AXIS2_PLACEMENT_3D('',#74073,#58870,#58871);
#52063=AXIS2_PLACEMENT_3D('',#74075,#58872,#58873);
#52064=AXIS2_PLACEMENT_3D('',#74077,#58875,#58876);
#52065=AXIS2_PLACEMENT_3D('',#74079,#58877,#58878);
#52066=AXIS2_PLACEMENT_3D('',#74081,#58880,#58881);
#52067=AXIS2_PLACEMENT_3D('',#74083,#58882,#58883);
#52068=AXIS2_PLACEMENT_3D('',#74085,#58885,#58886);
#52069=AXIS2_PLACEMENT_3D('',#74087,#58887,#58888);
#52070=AXIS2_PLACEMENT_3D('',#74089,#58890,#58891);
#52071=AXIS2_PLACEMENT_3D('',#74091,#58892,#58893);
#52072=AXIS2_PLACEMENT_3D('',#74093,#58895,#58896);
#52073=AXIS2_PLACEMENT_3D('',#74097,#58899,#58900);
#52074=AXIS2_PLACEMENT_3D('',#74099,#58901,#58902);
#52075=AXIS2_PLACEMENT_3D('',#74101,#58904,#58905);
#52076=AXIS2_PLACEMENT_3D('',#74103,#58906,#58907);
#52077=AXIS2_PLACEMENT_3D('',#74105,#58909,#58910);
#52078=AXIS2_PLACEMENT_3D('',#74107,#58911,#58912);
#52079=AXIS2_PLACEMENT_3D('',#74109,#58914,#58915);
#52080=AXIS2_PLACEMENT_3D('',#74111,#58916,#58917);
#52081=AXIS2_PLACEMENT_3D('',#74113,#58919,#58920);
#52082=AXIS2_PLACEMENT_3D('',#74115,#58921,#58922);
#52083=AXIS2_PLACEMENT_3D('',#74117,#58924,#58925);
#52084=AXIS2_PLACEMENT_3D('',#74119,#58927,#58928);
#52085=AXIS2_PLACEMENT_3D('',#74120,#58929,#58930);
#52086=AXIS2_PLACEMENT_3D('',#74122,#58931,#58932);
#52087=AXIS2_PLACEMENT_3D('',#74124,#58933,#58934);
#52088=AXIS2_PLACEMENT_3D('',#74128,#58936,#58937);
#52089=AXIS2_PLACEMENT_3D('',#74130,#58938,#58939);
#52090=AXIS2_PLACEMENT_3D('',#74132,#58940,#58941);
#52091=AXIS2_PLACEMENT_3D('',#74134,#58942,#58943);
#52092=AXIS2_PLACEMENT_3D('',#74136,#58944,#58945);
#52093=AXIS2_PLACEMENT_3D('',#74140,#58947,#58948);
#52094=AXIS2_PLACEMENT_3D('',#74142,#58949,#58950);
#52095=AXIS2_PLACEMENT_3D('',#74144,#58951,#58952);
#52096=AXIS2_PLACEMENT_3D('',#74146,#58953,#58954);
#52097=AXIS2_PLACEMENT_3D('',#74148,#58955,#58956);
#52098=AXIS2_PLACEMENT_3D('',#74150,#58958,#58959);
#52099=AXIS2_PLACEMENT_3D('',#74152,#58961,#58962);
#52100=AXIS2_PLACEMENT_3D('',#74154,#58964,#58965);
#52101=AXIS2_PLACEMENT_3D('',#74156,#58967,#58968);
#52102=AXIS2_PLACEMENT_3D('',#74158,#58970,#58971);
#52103=AXIS2_PLACEMENT_3D('',#74160,#58973,#58974);
#52104=AXIS2_PLACEMENT_3D('',#74162,#58976,#58977);
#52105=AXIS2_PLACEMENT_3D('',#74164,#58979,#58980);
#52106=AXIS2_PLACEMENT_3D('',#74166,#58982,#58983);
#52107=AXIS2_PLACEMENT_3D('',#74168,#58985,#58986);
#52108=AXIS2_PLACEMENT_3D('',#74170,#58988,#58989);
#52109=AXIS2_PLACEMENT_3D('',#74172,#58991,#58992);
#52110=AXIS2_PLACEMENT_3D('',#74174,#58994,#58995);
#52111=AXIS2_PLACEMENT_3D('',#74176,#58997,#58998);
#52112=AXIS2_PLACEMENT_3D('',#74180,#58999,#59000);
#52113=AXIS2_PLACEMENT_3D('',#74184,#59003,#59004);
#52114=AXIS2_PLACEMENT_3D('',#74186,#59005,#59006);
#52115=AXIS2_PLACEMENT_3D('',#74188,#59008,#59009);
#52116=AXIS2_PLACEMENT_3D('',#74190,#59010,#59011);
#52117=AXIS2_PLACEMENT_3D('',#74192,#59013,#59014);
#52118=AXIS2_PLACEMENT_3D('',#74194,#59015,#59016);
#52119=AXIS2_PLACEMENT_3D('',#74196,#59018,#59019);
#52120=AXIS2_PLACEMENT_3D('',#74198,#59020,#59021);
#52121=AXIS2_PLACEMENT_3D('',#74200,#59023,#59024);
#52122=AXIS2_PLACEMENT_3D('',#74202,#59025,#59026);
#52123=AXIS2_PLACEMENT_3D('',#74204,#59028,#59029);
#52124=AXIS2_PLACEMENT_3D('',#74208,#59032,#59033);
#52125=AXIS2_PLACEMENT_3D('',#74210,#59034,#59035);
#52126=AXIS2_PLACEMENT_3D('',#74212,#59037,#59038);
#52127=AXIS2_PLACEMENT_3D('',#74214,#59039,#59040);
#52128=AXIS2_PLACEMENT_3D('',#74216,#59042,#59043);
#52129=AXIS2_PLACEMENT_3D('',#74218,#59044,#59045);
#52130=AXIS2_PLACEMENT_3D('',#74220,#59047,#59048);
#52131=AXIS2_PLACEMENT_3D('',#74222,#59049,#59050);
#52132=AXIS2_PLACEMENT_3D('',#74224,#59052,#59053);
#52133=AXIS2_PLACEMENT_3D('',#74226,#59054,#59055);
#52134=AXIS2_PLACEMENT_3D('',#74228,#59057,#59058);
#52135=AXIS2_PLACEMENT_3D('',#74230,#59060,#59061);
#52136=AXIS2_PLACEMENT_3D('',#74231,#59062,#59063);
#52137=AXIS2_PLACEMENT_3D('',#74233,#59064,#59065);
#52138=AXIS2_PLACEMENT_3D('',#74235,#59066,#59067);
#52139=AXIS2_PLACEMENT_3D('',#74239,#59069,#59070);
#52140=AXIS2_PLACEMENT_3D('',#74241,#59071,#59072);
#52141=AXIS2_PLACEMENT_3D('',#74243,#59073,#59074);
#52142=AXIS2_PLACEMENT_3D('',#74245,#59075,#59076);
#52143=AXIS2_PLACEMENT_3D('',#74247,#59077,#59078);
#52144=AXIS2_PLACEMENT_3D('',#74251,#59080,#59081);
#52145=AXIS2_PLACEMENT_3D('',#74253,#59082,#59083);
#52146=AXIS2_PLACEMENT_3D('',#74255,#59084,#59085);
#52147=AXIS2_PLACEMENT_3D('',#74257,#59086,#59087);
#52148=AXIS2_PLACEMENT_3D('',#74259,#59088,#59089);
#52149=AXIS2_PLACEMENT_3D('',#74261,#59091,#59092);
#52150=AXIS2_PLACEMENT_3D('',#74263,#59094,#59095);
#52151=AXIS2_PLACEMENT_3D('',#74265,#59097,#59098);
#52152=AXIS2_PLACEMENT_3D('',#74267,#59100,#59101);
#52153=AXIS2_PLACEMENT_3D('',#74269,#59103,#59104);
#52154=AXIS2_PLACEMENT_3D('',#74271,#59106,#59107);
#52155=AXIS2_PLACEMENT_3D('',#74273,#59109,#59110);
#52156=AXIS2_PLACEMENT_3D('',#74275,#59112,#59113);
#52157=AXIS2_PLACEMENT_3D('',#74277,#59115,#59116);
#52158=AXIS2_PLACEMENT_3D('',#74279,#59118,#59119);
#52159=AXIS2_PLACEMENT_3D('',#74281,#59121,#59122);
#52160=AXIS2_PLACEMENT_3D('',#74283,#59124,#59125);
#52161=AXIS2_PLACEMENT_3D('',#74285,#59127,#59128);
#52162=AXIS2_PLACEMENT_3D('',#74287,#59130,#59131);
#52163=AXIS2_PLACEMENT_3D('',#74291,#59132,#59133);
#52164=AXIS2_PLACEMENT_3D('',#74295,#59136,#59137);
#52165=AXIS2_PLACEMENT_3D('',#74297,#59138,#59139);
#52166=AXIS2_PLACEMENT_3D('',#74299,#59141,#59142);
#52167=AXIS2_PLACEMENT_3D('',#74301,#59143,#59144);
#52168=AXIS2_PLACEMENT_3D('',#74303,#59146,#59147);
#52169=AXIS2_PLACEMENT_3D('',#74305,#59148,#59149);
#52170=AXIS2_PLACEMENT_3D('',#74307,#59151,#59152);
#52171=AXIS2_PLACEMENT_3D('',#74309,#59153,#59154);
#52172=AXIS2_PLACEMENT_3D('',#74311,#59156,#59157);
#52173=AXIS2_PLACEMENT_3D('',#74313,#59158,#59159);
#52174=AXIS2_PLACEMENT_3D('',#74315,#59161,#59162);
#52175=AXIS2_PLACEMENT_3D('',#74319,#59165,#59166);
#52176=AXIS2_PLACEMENT_3D('',#74321,#59167,#59168);
#52177=AXIS2_PLACEMENT_3D('',#74323,#59170,#59171);
#52178=AXIS2_PLACEMENT_3D('',#74325,#59172,#59173);
#52179=AXIS2_PLACEMENT_3D('',#74327,#59175,#59176);
#52180=AXIS2_PLACEMENT_3D('',#74329,#59177,#59178);
#52181=AXIS2_PLACEMENT_3D('',#74331,#59180,#59181);
#52182=AXIS2_PLACEMENT_3D('',#74333,#59182,#59183);
#52183=AXIS2_PLACEMENT_3D('',#74335,#59185,#59186);
#52184=AXIS2_PLACEMENT_3D('',#74337,#59187,#59188);
#52185=AXIS2_PLACEMENT_3D('',#74339,#59190,#59191);
#52186=AXIS2_PLACEMENT_3D('',#74341,#59193,#59194);
#52187=AXIS2_PLACEMENT_3D('',#74342,#59195,#59196);
#52188=AXIS2_PLACEMENT_3D('',#74344,#59197,#59198);
#52189=AXIS2_PLACEMENT_3D('',#74346,#59199,#59200);
#52190=AXIS2_PLACEMENT_3D('',#74350,#59202,#59203);
#52191=AXIS2_PLACEMENT_3D('',#74352,#59204,#59205);
#52192=AXIS2_PLACEMENT_3D('',#74354,#59206,#59207);
#52193=AXIS2_PLACEMENT_3D('',#74356,#59208,#59209);
#52194=AXIS2_PLACEMENT_3D('',#74358,#59210,#59211);
#52195=AXIS2_PLACEMENT_3D('',#74362,#59213,#59214);
#52196=AXIS2_PLACEMENT_3D('',#74364,#59215,#59216);
#52197=AXIS2_PLACEMENT_3D('',#74366,#59217,#59218);
#52198=AXIS2_PLACEMENT_3D('',#74368,#59219,#59220);
#52199=AXIS2_PLACEMENT_3D('',#74370,#59221,#59222);
#52200=AXIS2_PLACEMENT_3D('',#74372,#59224,#59225);
#52201=AXIS2_PLACEMENT_3D('',#74374,#59227,#59228);
#52202=AXIS2_PLACEMENT_3D('',#74376,#59230,#59231);
#52203=AXIS2_PLACEMENT_3D('',#74378,#59233,#59234);
#52204=AXIS2_PLACEMENT_3D('',#74380,#59236,#59237);
#52205=AXIS2_PLACEMENT_3D('',#74382,#59239,#59240);
#52206=AXIS2_PLACEMENT_3D('',#74384,#59242,#59243);
#52207=AXIS2_PLACEMENT_3D('',#74386,#59245,#59246);
#52208=AXIS2_PLACEMENT_3D('',#74388,#59248,#59249);
#52209=AXIS2_PLACEMENT_3D('',#74390,#59251,#59252);
#52210=AXIS2_PLACEMENT_3D('',#74392,#59254,#59255);
#52211=AXIS2_PLACEMENT_3D('',#74394,#59257,#59258);
#52212=AXIS2_PLACEMENT_3D('',#74396,#59260,#59261);
#52213=AXIS2_PLACEMENT_3D('',#74398,#59263,#59264);
#52214=AXIS2_PLACEMENT_3D('',#74402,#59265,#59266);
#52215=AXIS2_PLACEMENT_3D('',#74406,#59269,#59270);
#52216=AXIS2_PLACEMENT_3D('',#74408,#59271,#59272);
#52217=AXIS2_PLACEMENT_3D('',#74410,#59274,#59275);
#52218=AXIS2_PLACEMENT_3D('',#74412,#59276,#59277);
#52219=AXIS2_PLACEMENT_3D('',#74414,#59279,#59280);
#52220=AXIS2_PLACEMENT_3D('',#74416,#59281,#59282);
#52221=AXIS2_PLACEMENT_3D('',#74418,#59284,#59285);
#52222=AXIS2_PLACEMENT_3D('',#74420,#59286,#59287);
#52223=AXIS2_PLACEMENT_3D('',#74422,#59289,#59290);
#52224=AXIS2_PLACEMENT_3D('',#74424,#59291,#59292);
#52225=AXIS2_PLACEMENT_3D('',#74426,#59294,#59295);
#52226=AXIS2_PLACEMENT_3D('',#74430,#59298,#59299);
#52227=AXIS2_PLACEMENT_3D('',#74432,#59300,#59301);
#52228=AXIS2_PLACEMENT_3D('',#74434,#59303,#59304);
#52229=AXIS2_PLACEMENT_3D('',#74436,#59305,#59306);
#52230=AXIS2_PLACEMENT_3D('',#74438,#59308,#59309);
#52231=AXIS2_PLACEMENT_3D('',#74440,#59310,#59311);
#52232=AXIS2_PLACEMENT_3D('',#74442,#59313,#59314);
#52233=AXIS2_PLACEMENT_3D('',#74444,#59315,#59316);
#52234=AXIS2_PLACEMENT_3D('',#74446,#59318,#59319);
#52235=AXIS2_PLACEMENT_3D('',#74448,#59320,#59321);
#52236=AXIS2_PLACEMENT_3D('',#74450,#59323,#59324);
#52237=AXIS2_PLACEMENT_3D('',#74452,#59326,#59327);
#52238=AXIS2_PLACEMENT_3D('',#74453,#59328,#59329);
#52239=AXIS2_PLACEMENT_3D('',#74455,#59330,#59331);
#52240=AXIS2_PLACEMENT_3D('',#74457,#59332,#59333);
#52241=AXIS2_PLACEMENT_3D('',#74461,#59335,#59336);
#52242=AXIS2_PLACEMENT_3D('',#74463,#59337,#59338);
#52243=AXIS2_PLACEMENT_3D('',#74465,#59339,#59340);
#52244=AXIS2_PLACEMENT_3D('',#74467,#59341,#59342);
#52245=AXIS2_PLACEMENT_3D('',#74469,#59343,#59344);
#52246=AXIS2_PLACEMENT_3D('',#74473,#59346,#59347);
#52247=AXIS2_PLACEMENT_3D('',#74475,#59348,#59349);
#52248=AXIS2_PLACEMENT_3D('',#74477,#59350,#59351);
#52249=AXIS2_PLACEMENT_3D('',#74479,#59352,#59353);
#52250=AXIS2_PLACEMENT_3D('',#74481,#59354,#59355);
#52251=AXIS2_PLACEMENT_3D('',#74483,#59357,#59358);
#52252=AXIS2_PLACEMENT_3D('',#74485,#59360,#59361);
#52253=AXIS2_PLACEMENT_3D('',#74487,#59363,#59364);
#52254=AXIS2_PLACEMENT_3D('',#74489,#59366,#59367);
#52255=AXIS2_PLACEMENT_3D('',#74491,#59369,#59370);
#52256=AXIS2_PLACEMENT_3D('',#74493,#59372,#59373);
#52257=AXIS2_PLACEMENT_3D('',#74495,#59375,#59376);
#52258=AXIS2_PLACEMENT_3D('',#74497,#59378,#59379);
#52259=AXIS2_PLACEMENT_3D('',#74499,#59381,#59382);
#52260=AXIS2_PLACEMENT_3D('',#74501,#59384,#59385);
#52261=AXIS2_PLACEMENT_3D('',#74503,#59387,#59388);
#52262=AXIS2_PLACEMENT_3D('',#74505,#59390,#59391);
#52263=AXIS2_PLACEMENT_3D('',#74507,#59393,#59394);
#52264=AXIS2_PLACEMENT_3D('',#74509,#59396,#59397);
#52265=AXIS2_PLACEMENT_3D('',#74513,#59398,#59399);
#52266=AXIS2_PLACEMENT_3D('',#74517,#59402,#59403);
#52267=AXIS2_PLACEMENT_3D('',#74519,#59404,#59405);
#52268=AXIS2_PLACEMENT_3D('',#74521,#59407,#59408);
#52269=AXIS2_PLACEMENT_3D('',#74523,#59409,#59410);
#52270=AXIS2_PLACEMENT_3D('',#74525,#59412,#59413);
#52271=AXIS2_PLACEMENT_3D('',#74527,#59414,#59415);
#52272=AXIS2_PLACEMENT_3D('',#74529,#59417,#59418);
#52273=AXIS2_PLACEMENT_3D('',#74531,#59419,#59420);
#52274=AXIS2_PLACEMENT_3D('',#74533,#59422,#59423);
#52275=AXIS2_PLACEMENT_3D('',#74535,#59424,#59425);
#52276=AXIS2_PLACEMENT_3D('',#74537,#59427,#59428);
#52277=AXIS2_PLACEMENT_3D('',#74541,#59431,#59432);
#52278=AXIS2_PLACEMENT_3D('',#74543,#59433,#59434);
#52279=AXIS2_PLACEMENT_3D('',#74545,#59436,#59437);
#52280=AXIS2_PLACEMENT_3D('',#74547,#59438,#59439);
#52281=AXIS2_PLACEMENT_3D('',#74549,#59441,#59442);
#52282=AXIS2_PLACEMENT_3D('',#74551,#59443,#59444);
#52283=AXIS2_PLACEMENT_3D('',#74553,#59446,#59447);
#52284=AXIS2_PLACEMENT_3D('',#74555,#59448,#59449);
#52285=AXIS2_PLACEMENT_3D('',#74557,#59451,#59452);
#52286=AXIS2_PLACEMENT_3D('',#74559,#59453,#59454);
#52287=AXIS2_PLACEMENT_3D('',#74561,#59456,#59457);
#52288=AXIS2_PLACEMENT_3D('',#74563,#59459,#59460);
#52289=AXIS2_PLACEMENT_3D('',#74564,#59461,#59462);
#52290=AXIS2_PLACEMENT_3D('',#74566,#59463,#59464);
#52291=AXIS2_PLACEMENT_3D('',#74568,#59465,#59466);
#52292=AXIS2_PLACEMENT_3D('',#74572,#59468,#59469);
#52293=AXIS2_PLACEMENT_3D('',#74574,#59470,#59471);
#52294=AXIS2_PLACEMENT_3D('',#74576,#59472,#59473);
#52295=AXIS2_PLACEMENT_3D('',#74578,#59474,#59475);
#52296=AXIS2_PLACEMENT_3D('',#74580,#59476,#59477);
#52297=AXIS2_PLACEMENT_3D('',#74584,#59479,#59480);
#52298=AXIS2_PLACEMENT_3D('',#74586,#59481,#59482);
#52299=AXIS2_PLACEMENT_3D('',#74588,#59483,#59484);
#52300=AXIS2_PLACEMENT_3D('',#74590,#59485,#59486);
#52301=AXIS2_PLACEMENT_3D('',#74592,#59487,#59488);
#52302=AXIS2_PLACEMENT_3D('',#74594,#59490,#59491);
#52303=AXIS2_PLACEMENT_3D('',#74596,#59493,#59494);
#52304=AXIS2_PLACEMENT_3D('',#74598,#59496,#59497);
#52305=AXIS2_PLACEMENT_3D('',#74600,#59499,#59500);
#52306=AXIS2_PLACEMENT_3D('',#74602,#59502,#59503);
#52307=AXIS2_PLACEMENT_3D('',#74604,#59505,#59506);
#52308=AXIS2_PLACEMENT_3D('',#74606,#59508,#59509);
#52309=AXIS2_PLACEMENT_3D('',#74608,#59511,#59512);
#52310=AXIS2_PLACEMENT_3D('',#74610,#59514,#59515);
#52311=AXIS2_PLACEMENT_3D('',#74612,#59517,#59518);
#52312=AXIS2_PLACEMENT_3D('',#74614,#59520,#59521);
#52313=AXIS2_PLACEMENT_3D('',#74616,#59523,#59524);
#52314=AXIS2_PLACEMENT_3D('',#74618,#59526,#59527);
#52315=AXIS2_PLACEMENT_3D('',#74620,#59529,#59530);
#52316=AXIS2_PLACEMENT_3D('',#74624,#59531,#59532);
#52317=AXIS2_PLACEMENT_3D('',#74628,#59535,#59536);
#52318=AXIS2_PLACEMENT_3D('',#74630,#59537,#59538);
#52319=AXIS2_PLACEMENT_3D('',#74632,#59540,#59541);
#52320=AXIS2_PLACEMENT_3D('',#74634,#59542,#59543);
#52321=AXIS2_PLACEMENT_3D('',#74636,#59545,#59546);
#52322=AXIS2_PLACEMENT_3D('',#74638,#59547,#59548);
#52323=AXIS2_PLACEMENT_3D('',#74640,#59550,#59551);
#52324=AXIS2_PLACEMENT_3D('',#74642,#59552,#59553);
#52325=AXIS2_PLACEMENT_3D('',#74644,#59555,#59556);
#52326=AXIS2_PLACEMENT_3D('',#74646,#59557,#59558);
#52327=AXIS2_PLACEMENT_3D('',#74648,#59560,#59561);
#52328=AXIS2_PLACEMENT_3D('',#74652,#59564,#59565);
#52329=AXIS2_PLACEMENT_3D('',#74654,#59566,#59567);
#52330=AXIS2_PLACEMENT_3D('',#74656,#59569,#59570);
#52331=AXIS2_PLACEMENT_3D('',#74658,#59571,#59572);
#52332=AXIS2_PLACEMENT_3D('',#74660,#59574,#59575);
#52333=AXIS2_PLACEMENT_3D('',#74662,#59576,#59577);
#52334=AXIS2_PLACEMENT_3D('',#74664,#59579,#59580);
#52335=AXIS2_PLACEMENT_3D('',#74666,#59581,#59582);
#52336=AXIS2_PLACEMENT_3D('',#74668,#59584,#59585);
#52337=AXIS2_PLACEMENT_3D('',#74670,#59586,#59587);
#52338=AXIS2_PLACEMENT_3D('',#74672,#59589,#59590);
#52339=AXIS2_PLACEMENT_3D('',#74674,#59592,#59593);
#52340=AXIS2_PLACEMENT_3D('',#74675,#59594,#59595);
#52341=AXIS2_PLACEMENT_3D('',#74677,#59596,#59597);
#52342=AXIS2_PLACEMENT_3D('',#74679,#59598,#59599);
#52343=AXIS2_PLACEMENT_3D('',#74683,#59601,#59602);
#52344=AXIS2_PLACEMENT_3D('',#74685,#59603,#59604);
#52345=AXIS2_PLACEMENT_3D('',#74687,#59605,#59606);
#52346=AXIS2_PLACEMENT_3D('',#74689,#59607,#59608);
#52347=AXIS2_PLACEMENT_3D('',#74691,#59609,#59610);
#52348=AXIS2_PLACEMENT_3D('',#74695,#59612,#59613);
#52349=AXIS2_PLACEMENT_3D('',#74697,#59614,#59615);
#52350=AXIS2_PLACEMENT_3D('',#74699,#59616,#59617);
#52351=AXIS2_PLACEMENT_3D('',#74701,#59618,#59619);
#52352=AXIS2_PLACEMENT_3D('',#74703,#59620,#59621);
#52353=AXIS2_PLACEMENT_3D('',#74705,#59623,#59624);
#52354=AXIS2_PLACEMENT_3D('',#74707,#59626,#59627);
#52355=AXIS2_PLACEMENT_3D('',#74709,#59629,#59630);
#52356=AXIS2_PLACEMENT_3D('',#74711,#59632,#59633);
#52357=AXIS2_PLACEMENT_3D('',#74713,#59635,#59636);
#52358=AXIS2_PLACEMENT_3D('',#74715,#59638,#59639);
#52359=AXIS2_PLACEMENT_3D('',#74717,#59641,#59642);
#52360=AXIS2_PLACEMENT_3D('',#74719,#59644,#59645);
#52361=AXIS2_PLACEMENT_3D('',#74721,#59647,#59648);
#52362=AXIS2_PLACEMENT_3D('',#74723,#59650,#59651);
#52363=AXIS2_PLACEMENT_3D('',#74725,#59653,#59654);
#52364=AXIS2_PLACEMENT_3D('',#74727,#59656,#59657);
#52365=AXIS2_PLACEMENT_3D('',#74729,#59659,#59660);
#52366=AXIS2_PLACEMENT_3D('',#74731,#59662,#59663);
#52367=AXIS2_PLACEMENT_3D('',#74735,#59664,#59665);
#52368=AXIS2_PLACEMENT_3D('',#74739,#59668,#59669);
#52369=AXIS2_PLACEMENT_3D('',#74741,#59670,#59671);
#52370=AXIS2_PLACEMENT_3D('',#74743,#59673,#59674);
#52371=AXIS2_PLACEMENT_3D('',#74745,#59675,#59676);
#52372=AXIS2_PLACEMENT_3D('',#74747,#59678,#59679);
#52373=AXIS2_PLACEMENT_3D('',#74749,#59680,#59681);
#52374=AXIS2_PLACEMENT_3D('',#74751,#59683,#59684);
#52375=AXIS2_PLACEMENT_3D('',#74753,#59685,#59686);
#52376=AXIS2_PLACEMENT_3D('',#74755,#59688,#59689);
#52377=AXIS2_PLACEMENT_3D('',#74757,#59690,#59691);
#52378=AXIS2_PLACEMENT_3D('',#74759,#59693,#59694);
#52379=AXIS2_PLACEMENT_3D('',#74763,#59697,#59698);
#52380=AXIS2_PLACEMENT_3D('',#74765,#59699,#59700);
#52381=AXIS2_PLACEMENT_3D('',#74767,#59702,#59703);
#52382=AXIS2_PLACEMENT_3D('',#74769,#59704,#59705);
#52383=AXIS2_PLACEMENT_3D('',#74771,#59707,#59708);
#52384=AXIS2_PLACEMENT_3D('',#74773,#59709,#59710);
#52385=AXIS2_PLACEMENT_3D('',#74775,#59712,#59713);
#52386=AXIS2_PLACEMENT_3D('',#74777,#59714,#59715);
#52387=AXIS2_PLACEMENT_3D('',#74779,#59717,#59718);
#52388=AXIS2_PLACEMENT_3D('',#74781,#59719,#59720);
#52389=AXIS2_PLACEMENT_3D('',#74783,#59722,#59723);
#52390=AXIS2_PLACEMENT_3D('',#74785,#59725,#59726);
#52391=AXIS2_PLACEMENT_3D('',#74786,#59727,#59728);
#52392=AXIS2_PLACEMENT_3D('',#74788,#59729,#59730);
#52393=AXIS2_PLACEMENT_3D('',#74790,#59731,#59732);
#52394=AXIS2_PLACEMENT_3D('',#74794,#59734,#59735);
#52395=AXIS2_PLACEMENT_3D('',#74796,#59736,#59737);
#52396=AXIS2_PLACEMENT_3D('',#74798,#59738,#59739);
#52397=AXIS2_PLACEMENT_3D('',#74800,#59740,#59741);
#52398=AXIS2_PLACEMENT_3D('',#74802,#59742,#59743);
#52399=AXIS2_PLACEMENT_3D('',#74806,#59745,#59746);
#52400=AXIS2_PLACEMENT_3D('',#74808,#59747,#59748);
#52401=AXIS2_PLACEMENT_3D('',#74810,#59749,#59750);
#52402=AXIS2_PLACEMENT_3D('',#74812,#59751,#59752);
#52403=AXIS2_PLACEMENT_3D('',#74814,#59753,#59754);
#52404=AXIS2_PLACEMENT_3D('',#74816,#59756,#59757);
#52405=AXIS2_PLACEMENT_3D('',#74818,#59759,#59760);
#52406=AXIS2_PLACEMENT_3D('',#74820,#59762,#59763);
#52407=AXIS2_PLACEMENT_3D('',#74822,#59765,#59766);
#52408=AXIS2_PLACEMENT_3D('',#74824,#59768,#59769);
#52409=AXIS2_PLACEMENT_3D('',#74826,#59771,#59772);
#52410=AXIS2_PLACEMENT_3D('',#74828,#59774,#59775);
#52411=AXIS2_PLACEMENT_3D('',#74830,#59777,#59778);
#52412=AXIS2_PLACEMENT_3D('',#74832,#59780,#59781);
#52413=AXIS2_PLACEMENT_3D('',#74834,#59783,#59784);
#52414=AXIS2_PLACEMENT_3D('',#74836,#59786,#59787);
#52415=AXIS2_PLACEMENT_3D('',#74838,#59789,#59790);
#52416=AXIS2_PLACEMENT_3D('',#74840,#59792,#59793);
#52417=AXIS2_PLACEMENT_3D('',#74842,#59795,#59796);
#52418=AXIS2_PLACEMENT_3D('',#74846,#59797,#59798);
#52419=AXIS2_PLACEMENT_3D('',#74850,#59801,#59802);
#52420=AXIS2_PLACEMENT_3D('',#74852,#59803,#59804);
#52421=AXIS2_PLACEMENT_3D('',#74854,#59806,#59807);
#52422=AXIS2_PLACEMENT_3D('',#74856,#59808,#59809);
#52423=AXIS2_PLACEMENT_3D('',#74858,#59811,#59812);
#52424=AXIS2_PLACEMENT_3D('',#74860,#59813,#59814);
#52425=AXIS2_PLACEMENT_3D('',#74862,#59816,#59817);
#52426=AXIS2_PLACEMENT_3D('',#74864,#59818,#59819);
#52427=AXIS2_PLACEMENT_3D('',#74866,#59821,#59822);
#52428=AXIS2_PLACEMENT_3D('',#74868,#59823,#59824);
#52429=AXIS2_PLACEMENT_3D('',#74870,#59826,#59827);
#52430=AXIS2_PLACEMENT_3D('',#74874,#59830,#59831);
#52431=AXIS2_PLACEMENT_3D('',#74876,#59832,#59833);
#52432=AXIS2_PLACEMENT_3D('',#74878,#59835,#59836);
#52433=AXIS2_PLACEMENT_3D('',#74880,#59837,#59838);
#52434=AXIS2_PLACEMENT_3D('',#74882,#59840,#59841);
#52435=AXIS2_PLACEMENT_3D('',#74884,#59842,#59843);
#52436=AXIS2_PLACEMENT_3D('',#74886,#59845,#59846);
#52437=AXIS2_PLACEMENT_3D('',#74888,#59847,#59848);
#52438=AXIS2_PLACEMENT_3D('',#74890,#59850,#59851);
#52439=AXIS2_PLACEMENT_3D('',#74892,#59852,#59853);
#52440=AXIS2_PLACEMENT_3D('',#74894,#59855,#59856);
#52441=AXIS2_PLACEMENT_3D('',#74896,#59858,#59859);
#52442=AXIS2_PLACEMENT_3D('',#74897,#59860,#59861);
#52443=AXIS2_PLACEMENT_3D('',#74899,#59862,#59863);
#52444=AXIS2_PLACEMENT_3D('',#74901,#59864,#59865);
#52445=AXIS2_PLACEMENT_3D('',#74905,#59867,#59868);
#52446=AXIS2_PLACEMENT_3D('',#74907,#59869,#59870);
#52447=AXIS2_PLACEMENT_3D('',#74909,#59871,#59872);
#52448=AXIS2_PLACEMENT_3D('',#74911,#59873,#59874);
#52449=AXIS2_PLACEMENT_3D('',#74913,#59875,#59876);
#52450=AXIS2_PLACEMENT_3D('',#74917,#59878,#59879);
#52451=AXIS2_PLACEMENT_3D('',#74919,#59880,#59881);
#52452=AXIS2_PLACEMENT_3D('',#74921,#59882,#59883);
#52453=AXIS2_PLACEMENT_3D('',#74923,#59884,#59885);
#52454=AXIS2_PLACEMENT_3D('',#74925,#59886,#59887);
#52455=AXIS2_PLACEMENT_3D('',#74927,#59889,#59890);
#52456=AXIS2_PLACEMENT_3D('',#74929,#59892,#59893);
#52457=AXIS2_PLACEMENT_3D('',#74931,#59895,#59896);
#52458=AXIS2_PLACEMENT_3D('',#74933,#59898,#59899);
#52459=AXIS2_PLACEMENT_3D('',#74935,#59901,#59902);
#52460=AXIS2_PLACEMENT_3D('',#74937,#59904,#59905);
#52461=AXIS2_PLACEMENT_3D('',#74939,#59907,#59908);
#52462=AXIS2_PLACEMENT_3D('',#74941,#59910,#59911);
#52463=AXIS2_PLACEMENT_3D('',#74943,#59913,#59914);
#52464=AXIS2_PLACEMENT_3D('',#74945,#59916,#59917);
#52465=AXIS2_PLACEMENT_3D('',#74947,#59919,#59920);
#52466=AXIS2_PLACEMENT_3D('',#74949,#59922,#59923);
#52467=AXIS2_PLACEMENT_3D('',#74951,#59925,#59926);
#52468=AXIS2_PLACEMENT_3D('',#74953,#59928,#59929);
#52469=AXIS2_PLACEMENT_3D('',#74957,#59930,#59931);
#52470=AXIS2_PLACEMENT_3D('',#74961,#59934,#59935);
#52471=AXIS2_PLACEMENT_3D('',#74963,#59936,#59937);
#52472=AXIS2_PLACEMENT_3D('',#74965,#59939,#59940);
#52473=AXIS2_PLACEMENT_3D('',#74967,#59941,#59942);
#52474=AXIS2_PLACEMENT_3D('',#74969,#59944,#59945);
#52475=AXIS2_PLACEMENT_3D('',#74971,#59946,#59947);
#52476=AXIS2_PLACEMENT_3D('',#74973,#59949,#59950);
#52477=AXIS2_PLACEMENT_3D('',#74975,#59951,#59952);
#52478=AXIS2_PLACEMENT_3D('',#74977,#59954,#59955);
#52479=AXIS2_PLACEMENT_3D('',#74979,#59956,#59957);
#52480=AXIS2_PLACEMENT_3D('',#74981,#59959,#59960);
#52481=AXIS2_PLACEMENT_3D('',#74985,#59963,#59964);
#52482=AXIS2_PLACEMENT_3D('',#74987,#59965,#59966);
#52483=AXIS2_PLACEMENT_3D('',#74989,#59968,#59969);
#52484=AXIS2_PLACEMENT_3D('',#74991,#59970,#59971);
#52485=AXIS2_PLACEMENT_3D('',#74993,#59973,#59974);
#52486=AXIS2_PLACEMENT_3D('',#74995,#59975,#59976);
#52487=AXIS2_PLACEMENT_3D('',#74997,#59978,#59979);
#52488=AXIS2_PLACEMENT_3D('',#74999,#59980,#59981);
#52489=AXIS2_PLACEMENT_3D('',#75001,#59983,#59984);
#52490=AXIS2_PLACEMENT_3D('',#75003,#59985,#59986);
#52491=AXIS2_PLACEMENT_3D('',#75005,#59988,#59989);
#52492=AXIS2_PLACEMENT_3D('',#75007,#59991,#59992);
#52493=AXIS2_PLACEMENT_3D('',#75008,#59993,#59994);
#52494=AXIS2_PLACEMENT_3D('',#75010,#59995,#59996);
#52495=AXIS2_PLACEMENT_3D('',#75012,#59997,#59998);
#52496=AXIS2_PLACEMENT_3D('',#75016,#60000,#60001);
#52497=AXIS2_PLACEMENT_3D('',#75018,#60002,#60003);
#52498=AXIS2_PLACEMENT_3D('',#75020,#60004,#60005);
#52499=AXIS2_PLACEMENT_3D('',#75022,#60006,#60007);
#52500=AXIS2_PLACEMENT_3D('',#75024,#60008,#60009);
#52501=AXIS2_PLACEMENT_3D('',#75028,#60011,#60012);
#52502=AXIS2_PLACEMENT_3D('',#75030,#60013,#60014);
#52503=AXIS2_PLACEMENT_3D('',#75032,#60015,#60016);
#52504=AXIS2_PLACEMENT_3D('',#75034,#60017,#60018);
#52505=AXIS2_PLACEMENT_3D('',#75036,#60019,#60020);
#52506=AXIS2_PLACEMENT_3D('',#75038,#60022,#60023);
#52507=AXIS2_PLACEMENT_3D('',#75040,#60025,#60026);
#52508=AXIS2_PLACEMENT_3D('',#75042,#60028,#60029);
#52509=AXIS2_PLACEMENT_3D('',#75044,#60031,#60032);
#52510=AXIS2_PLACEMENT_3D('',#75046,#60034,#60035);
#52511=AXIS2_PLACEMENT_3D('',#75048,#60037,#60038);
#52512=AXIS2_PLACEMENT_3D('',#75050,#60040,#60041);
#52513=AXIS2_PLACEMENT_3D('',#75052,#60043,#60044);
#52514=AXIS2_PLACEMENT_3D('',#75054,#60046,#60047);
#52515=AXIS2_PLACEMENT_3D('',#75056,#60049,#60050);
#52516=AXIS2_PLACEMENT_3D('',#75058,#60052,#60053);
#52517=AXIS2_PLACEMENT_3D('',#75060,#60055,#60056);
#52518=AXIS2_PLACEMENT_3D('',#75062,#60058,#60059);
#52519=AXIS2_PLACEMENT_3D('',#75064,#60061,#60062);
#52520=AXIS2_PLACEMENT_3D('',#75068,#60063,#60064);
#52521=AXIS2_PLACEMENT_3D('',#75072,#60067,#60068);
#52522=AXIS2_PLACEMENT_3D('',#75074,#60069,#60070);
#52523=AXIS2_PLACEMENT_3D('',#75076,#60072,#60073);
#52524=AXIS2_PLACEMENT_3D('',#75078,#60074,#60075);
#52525=AXIS2_PLACEMENT_3D('',#75080,#60077,#60078);
#52526=AXIS2_PLACEMENT_3D('',#75082,#60079,#60080);
#52527=AXIS2_PLACEMENT_3D('',#75084,#60082,#60083);
#52528=AXIS2_PLACEMENT_3D('',#75086,#60084,#60085);
#52529=AXIS2_PLACEMENT_3D('',#75088,#60087,#60088);
#52530=AXIS2_PLACEMENT_3D('',#75090,#60089,#60090);
#52531=AXIS2_PLACEMENT_3D('',#75092,#60092,#60093);
#52532=AXIS2_PLACEMENT_3D('',#75096,#60096,#60097);
#52533=AXIS2_PLACEMENT_3D('',#75098,#60098,#60099);
#52534=AXIS2_PLACEMENT_3D('',#75100,#60101,#60102);
#52535=AXIS2_PLACEMENT_3D('',#75102,#60103,#60104);
#52536=AXIS2_PLACEMENT_3D('',#75104,#60106,#60107);
#52537=AXIS2_PLACEMENT_3D('',#75106,#60108,#60109);
#52538=AXIS2_PLACEMENT_3D('',#75108,#60111,#60112);
#52539=AXIS2_PLACEMENT_3D('',#75110,#60113,#60114);
#52540=AXIS2_PLACEMENT_3D('',#75112,#60116,#60117);
#52541=AXIS2_PLACEMENT_3D('',#75114,#60118,#60119);
#52542=AXIS2_PLACEMENT_3D('',#75116,#60121,#60122);
#52543=AXIS2_PLACEMENT_3D('',#75118,#60124,#60125);
#52544=AXIS2_PLACEMENT_3D('',#75119,#60126,#60127);
#52545=AXIS2_PLACEMENT_3D('',#75121,#60128,#60129);
#52546=AXIS2_PLACEMENT_3D('',#75123,#60130,#60131);
#52547=AXIS2_PLACEMENT_3D('',#75127,#60133,#60134);
#52548=AXIS2_PLACEMENT_3D('',#75129,#60135,#60136);
#52549=AXIS2_PLACEMENT_3D('',#75131,#60137,#60138);
#52550=AXIS2_PLACEMENT_3D('',#75133,#60139,#60140);
#52551=AXIS2_PLACEMENT_3D('',#75135,#60141,#60142);
#52552=AXIS2_PLACEMENT_3D('',#75139,#60144,#60145);
#52553=AXIS2_PLACEMENT_3D('',#75141,#60146,#60147);
#52554=AXIS2_PLACEMENT_3D('',#75143,#60148,#60149);
#52555=AXIS2_PLACEMENT_3D('',#75145,#60150,#60151);
#52556=AXIS2_PLACEMENT_3D('',#75147,#60152,#60153);
#52557=AXIS2_PLACEMENT_3D('',#75149,#60155,#60156);
#52558=AXIS2_PLACEMENT_3D('',#75151,#60158,#60159);
#52559=AXIS2_PLACEMENT_3D('',#75153,#60161,#60162);
#52560=AXIS2_PLACEMENT_3D('',#75155,#60164,#60165);
#52561=AXIS2_PLACEMENT_3D('',#75157,#60167,#60168);
#52562=AXIS2_PLACEMENT_3D('',#75159,#60170,#60171);
#52563=AXIS2_PLACEMENT_3D('',#75161,#60173,#60174);
#52564=AXIS2_PLACEMENT_3D('',#75163,#60176,#60177);
#52565=AXIS2_PLACEMENT_3D('',#75165,#60179,#60180);
#52566=AXIS2_PLACEMENT_3D('',#75167,#60182,#60183);
#52567=AXIS2_PLACEMENT_3D('',#75169,#60185,#60186);
#52568=AXIS2_PLACEMENT_3D('',#75171,#60188,#60189);
#52569=AXIS2_PLACEMENT_3D('',#75173,#60191,#60192);
#52570=AXIS2_PLACEMENT_3D('',#75175,#60194,#60195);
#52571=AXIS2_PLACEMENT_3D('',#75179,#60196,#60197);
#52572=AXIS2_PLACEMENT_3D('',#75183,#60200,#60201);
#52573=AXIS2_PLACEMENT_3D('',#75185,#60202,#60203);
#52574=AXIS2_PLACEMENT_3D('',#75187,#60205,#60206);
#52575=AXIS2_PLACEMENT_3D('',#75189,#60207,#60208);
#52576=AXIS2_PLACEMENT_3D('',#75191,#60210,#60211);
#52577=AXIS2_PLACEMENT_3D('',#75193,#60212,#60213);
#52578=AXIS2_PLACEMENT_3D('',#75195,#60215,#60216);
#52579=AXIS2_PLACEMENT_3D('',#75197,#60217,#60218);
#52580=AXIS2_PLACEMENT_3D('',#75199,#60220,#60221);
#52581=AXIS2_PLACEMENT_3D('',#75201,#60222,#60223);
#52582=AXIS2_PLACEMENT_3D('',#75203,#60225,#60226);
#52583=AXIS2_PLACEMENT_3D('',#75207,#60229,#60230);
#52584=AXIS2_PLACEMENT_3D('',#75209,#60231,#60232);
#52585=AXIS2_PLACEMENT_3D('',#75211,#60234,#60235);
#52586=AXIS2_PLACEMENT_3D('',#75213,#60236,#60237);
#52587=AXIS2_PLACEMENT_3D('',#75215,#60239,#60240);
#52588=AXIS2_PLACEMENT_3D('',#75217,#60241,#60242);
#52589=AXIS2_PLACEMENT_3D('',#75219,#60244,#60245);
#52590=AXIS2_PLACEMENT_3D('',#75221,#60246,#60247);
#52591=AXIS2_PLACEMENT_3D('',#75223,#60249,#60250);
#52592=AXIS2_PLACEMENT_3D('',#75225,#60251,#60252);
#52593=AXIS2_PLACEMENT_3D('',#75227,#60254,#60255);
#52594=AXIS2_PLACEMENT_3D('',#75229,#60257,#60258);
#52595=AXIS2_PLACEMENT_3D('',#75230,#60259,#60260);
#52596=AXIS2_PLACEMENT_3D('',#75232,#60261,#60262);
#52597=AXIS2_PLACEMENT_3D('',#75234,#60263,#60264);
#52598=AXIS2_PLACEMENT_3D('',#75238,#60266,#60267);
#52599=AXIS2_PLACEMENT_3D('',#75240,#60268,#60269);
#52600=AXIS2_PLACEMENT_3D('',#75242,#60270,#60271);
#52601=AXIS2_PLACEMENT_3D('',#75244,#60272,#60273);
#52602=AXIS2_PLACEMENT_3D('',#75246,#60274,#60275);
#52603=AXIS2_PLACEMENT_3D('',#75250,#60277,#60278);
#52604=AXIS2_PLACEMENT_3D('',#75252,#60279,#60280);
#52605=AXIS2_PLACEMENT_3D('',#75254,#60281,#60282);
#52606=AXIS2_PLACEMENT_3D('',#75256,#60283,#60284);
#52607=AXIS2_PLACEMENT_3D('',#75258,#60285,#60286);
#52608=AXIS2_PLACEMENT_3D('',#75260,#60288,#60289);
#52609=AXIS2_PLACEMENT_3D('',#75262,#60291,#60292);
#52610=AXIS2_PLACEMENT_3D('',#75264,#60294,#60295);
#52611=AXIS2_PLACEMENT_3D('',#75266,#60297,#60298);
#52612=AXIS2_PLACEMENT_3D('',#75268,#60300,#60301);
#52613=AXIS2_PLACEMENT_3D('',#75270,#60303,#60304);
#52614=AXIS2_PLACEMENT_3D('',#75272,#60306,#60307);
#52615=AXIS2_PLACEMENT_3D('',#75274,#60309,#60310);
#52616=AXIS2_PLACEMENT_3D('',#75276,#60312,#60313);
#52617=AXIS2_PLACEMENT_3D('',#75278,#60315,#60316);
#52618=AXIS2_PLACEMENT_3D('',#75280,#60318,#60319);
#52619=AXIS2_PLACEMENT_3D('',#75282,#60321,#60322);
#52620=AXIS2_PLACEMENT_3D('',#75284,#60324,#60325);
#52621=AXIS2_PLACEMENT_3D('',#75286,#60327,#60328);
#52622=AXIS2_PLACEMENT_3D('',#75290,#60329,#60330);
#52623=AXIS2_PLACEMENT_3D('',#75294,#60333,#60334);
#52624=AXIS2_PLACEMENT_3D('',#75296,#60335,#60336);
#52625=AXIS2_PLACEMENT_3D('',#75298,#60338,#60339);
#52626=AXIS2_PLACEMENT_3D('',#75300,#60340,#60341);
#52627=AXIS2_PLACEMENT_3D('',#75302,#60343,#60344);
#52628=AXIS2_PLACEMENT_3D('',#75304,#60345,#60346);
#52629=AXIS2_PLACEMENT_3D('',#75306,#60348,#60349);
#52630=AXIS2_PLACEMENT_3D('',#75308,#60350,#60351);
#52631=AXIS2_PLACEMENT_3D('',#75310,#60353,#60354);
#52632=AXIS2_PLACEMENT_3D('',#75312,#60355,#60356);
#52633=AXIS2_PLACEMENT_3D('',#75314,#60358,#60359);
#52634=AXIS2_PLACEMENT_3D('',#75318,#60362,#60363);
#52635=AXIS2_PLACEMENT_3D('',#75320,#60364,#60365);
#52636=AXIS2_PLACEMENT_3D('',#75322,#60367,#60368);
#52637=AXIS2_PLACEMENT_3D('',#75324,#60369,#60370);
#52638=AXIS2_PLACEMENT_3D('',#75326,#60372,#60373);
#52639=AXIS2_PLACEMENT_3D('',#75328,#60374,#60375);
#52640=AXIS2_PLACEMENT_3D('',#75330,#60377,#60378);
#52641=AXIS2_PLACEMENT_3D('',#75332,#60379,#60380);
#52642=AXIS2_PLACEMENT_3D('',#75334,#60382,#60383);
#52643=AXIS2_PLACEMENT_3D('',#75336,#60384,#60385);
#52644=AXIS2_PLACEMENT_3D('',#75338,#60387,#60388);
#52645=AXIS2_PLACEMENT_3D('',#75340,#60390,#60391);
#52646=AXIS2_PLACEMENT_3D('',#75341,#60392,#60393);
#52647=AXIS2_PLACEMENT_3D('',#75343,#60394,#60395);
#52648=AXIS2_PLACEMENT_3D('',#75345,#60396,#60397);
#52649=AXIS2_PLACEMENT_3D('',#75349,#60399,#60400);
#52650=AXIS2_PLACEMENT_3D('',#75351,#60401,#60402);
#52651=AXIS2_PLACEMENT_3D('',#75353,#60403,#60404);
#52652=AXIS2_PLACEMENT_3D('',#75355,#60405,#60406);
#52653=AXIS2_PLACEMENT_3D('',#75357,#60407,#60408);
#52654=AXIS2_PLACEMENT_3D('',#75361,#60410,#60411);
#52655=AXIS2_PLACEMENT_3D('',#75363,#60412,#60413);
#52656=AXIS2_PLACEMENT_3D('',#75365,#60414,#60415);
#52657=AXIS2_PLACEMENT_3D('',#75367,#60416,#60417);
#52658=AXIS2_PLACEMENT_3D('',#75369,#60418,#60419);
#52659=AXIS2_PLACEMENT_3D('',#75371,#60421,#60422);
#52660=AXIS2_PLACEMENT_3D('',#75373,#60424,#60425);
#52661=AXIS2_PLACEMENT_3D('',#75375,#60427,#60428);
#52662=AXIS2_PLACEMENT_3D('',#75377,#60430,#60431);
#52663=AXIS2_PLACEMENT_3D('',#75379,#60433,#60434);
#52664=AXIS2_PLACEMENT_3D('',#75381,#60436,#60437);
#52665=AXIS2_PLACEMENT_3D('',#75383,#60439,#60440);
#52666=AXIS2_PLACEMENT_3D('',#75385,#60442,#60443);
#52667=AXIS2_PLACEMENT_3D('',#75387,#60445,#60446);
#52668=AXIS2_PLACEMENT_3D('',#75389,#60448,#60449);
#52669=AXIS2_PLACEMENT_3D('',#75391,#60451,#60452);
#52670=AXIS2_PLACEMENT_3D('',#75393,#60454,#60455);
#52671=AXIS2_PLACEMENT_3D('',#75395,#60457,#60458);
#52672=AXIS2_PLACEMENT_3D('',#75397,#60460,#60461);
#52673=AXIS2_PLACEMENT_3D('',#75401,#60462,#60463);
#52674=AXIS2_PLACEMENT_3D('',#75405,#60466,#60467);
#52675=AXIS2_PLACEMENT_3D('',#75407,#60468,#60469);
#52676=AXIS2_PLACEMENT_3D('',#75409,#60471,#60472);
#52677=AXIS2_PLACEMENT_3D('',#75411,#60473,#60474);
#52678=AXIS2_PLACEMENT_3D('',#75413,#60476,#60477);
#52679=AXIS2_PLACEMENT_3D('',#75415,#60478,#60479);
#52680=AXIS2_PLACEMENT_3D('',#75417,#60481,#60482);
#52681=AXIS2_PLACEMENT_3D('',#75419,#60483,#60484);
#52682=AXIS2_PLACEMENT_3D('',#75421,#60486,#60487);
#52683=AXIS2_PLACEMENT_3D('',#75423,#60488,#60489);
#52684=AXIS2_PLACEMENT_3D('',#75425,#60491,#60492);
#52685=AXIS2_PLACEMENT_3D('',#75429,#60495,#60496);
#52686=AXIS2_PLACEMENT_3D('',#75431,#60497,#60498);
#52687=AXIS2_PLACEMENT_3D('',#75433,#60500,#60501);
#52688=AXIS2_PLACEMENT_3D('',#75435,#60502,#60503);
#52689=AXIS2_PLACEMENT_3D('',#75437,#60505,#60506);
#52690=AXIS2_PLACEMENT_3D('',#75439,#60507,#60508);
#52691=AXIS2_PLACEMENT_3D('',#75441,#60510,#60511);
#52692=AXIS2_PLACEMENT_3D('',#75443,#60512,#60513);
#52693=AXIS2_PLACEMENT_3D('',#75445,#60515,#60516);
#52694=AXIS2_PLACEMENT_3D('',#75447,#60517,#60518);
#52695=AXIS2_PLACEMENT_3D('',#75449,#60520,#60521);
#52696=AXIS2_PLACEMENT_3D('',#75451,#60523,#60524);
#52697=AXIS2_PLACEMENT_3D('',#75452,#60525,#60526);
#52698=AXIS2_PLACEMENT_3D('',#75454,#60527,#60528);
#52699=AXIS2_PLACEMENT_3D('',#75456,#60529,#60530);
#52700=AXIS2_PLACEMENT_3D('',#75460,#60532,#60533);
#52701=AXIS2_PLACEMENT_3D('',#75462,#60534,#60535);
#52702=AXIS2_PLACEMENT_3D('',#75464,#60536,#60537);
#52703=AXIS2_PLACEMENT_3D('',#75466,#60538,#60539);
#52704=AXIS2_PLACEMENT_3D('',#75468,#60540,#60541);
#52705=AXIS2_PLACEMENT_3D('',#75472,#60543,#60544);
#52706=AXIS2_PLACEMENT_3D('',#75474,#60545,#60546);
#52707=AXIS2_PLACEMENT_3D('',#75476,#60547,#60548);
#52708=AXIS2_PLACEMENT_3D('',#75478,#60549,#60550);
#52709=AXIS2_PLACEMENT_3D('',#75480,#60551,#60552);
#52710=AXIS2_PLACEMENT_3D('',#75482,#60554,#60555);
#52711=AXIS2_PLACEMENT_3D('',#75484,#60557,#60558);
#52712=AXIS2_PLACEMENT_3D('',#75486,#60560,#60561);
#52713=AXIS2_PLACEMENT_3D('',#75488,#60563,#60564);
#52714=AXIS2_PLACEMENT_3D('',#75490,#60566,#60567);
#52715=AXIS2_PLACEMENT_3D('',#75492,#60569,#60570);
#52716=AXIS2_PLACEMENT_3D('',#75494,#60572,#60573);
#52717=AXIS2_PLACEMENT_3D('',#75496,#60575,#60576);
#52718=AXIS2_PLACEMENT_3D('',#75498,#60578,#60579);
#52719=AXIS2_PLACEMENT_3D('',#75500,#60581,#60582);
#52720=AXIS2_PLACEMENT_3D('',#75502,#60584,#60585);
#52721=AXIS2_PLACEMENT_3D('',#75504,#60587,#60588);
#52722=AXIS2_PLACEMENT_3D('',#75506,#60590,#60591);
#52723=AXIS2_PLACEMENT_3D('',#75508,#60593,#60594);
#52724=AXIS2_PLACEMENT_3D('',#75512,#60595,#60596);
#52725=AXIS2_PLACEMENT_3D('',#75516,#60599,#60600);
#52726=AXIS2_PLACEMENT_3D('',#75518,#60601,#60602);
#52727=AXIS2_PLACEMENT_3D('',#75520,#60604,#60605);
#52728=AXIS2_PLACEMENT_3D('',#75522,#60606,#60607);
#52729=AXIS2_PLACEMENT_3D('',#75524,#60609,#60610);
#52730=AXIS2_PLACEMENT_3D('',#75526,#60611,#60612);
#52731=AXIS2_PLACEMENT_3D('',#75528,#60614,#60615);
#52732=AXIS2_PLACEMENT_3D('',#75530,#60616,#60617);
#52733=AXIS2_PLACEMENT_3D('',#75532,#60619,#60620);
#52734=AXIS2_PLACEMENT_3D('',#75534,#60621,#60622);
#52735=AXIS2_PLACEMENT_3D('',#75536,#60624,#60625);
#52736=AXIS2_PLACEMENT_3D('',#75540,#60628,#60629);
#52737=AXIS2_PLACEMENT_3D('',#75542,#60630,#60631);
#52738=AXIS2_PLACEMENT_3D('',#75544,#60633,#60634);
#52739=AXIS2_PLACEMENT_3D('',#75546,#60635,#60636);
#52740=AXIS2_PLACEMENT_3D('',#75548,#60638,#60639);
#52741=AXIS2_PLACEMENT_3D('',#75550,#60640,#60641);
#52742=AXIS2_PLACEMENT_3D('',#75552,#60643,#60644);
#52743=AXIS2_PLACEMENT_3D('',#75554,#60645,#60646);
#52744=AXIS2_PLACEMENT_3D('',#75556,#60648,#60649);
#52745=AXIS2_PLACEMENT_3D('',#75558,#60650,#60651);
#52746=AXIS2_PLACEMENT_3D('',#75560,#60653,#60654);
#52747=AXIS2_PLACEMENT_3D('',#75562,#60656,#60657);
#52748=AXIS2_PLACEMENT_3D('',#75563,#60658,#60659);
#52749=AXIS2_PLACEMENT_3D('',#75565,#60660,#60661);
#52750=AXIS2_PLACEMENT_3D('',#75567,#60662,#60663);
#52751=AXIS2_PLACEMENT_3D('',#75571,#60665,#60666);
#52752=AXIS2_PLACEMENT_3D('',#75573,#60667,#60668);
#52753=AXIS2_PLACEMENT_3D('',#75575,#60669,#60670);
#52754=AXIS2_PLACEMENT_3D('',#75577,#60671,#60672);
#52755=AXIS2_PLACEMENT_3D('',#75579,#60673,#60674);
#52756=AXIS2_PLACEMENT_3D('',#75583,#60676,#60677);
#52757=AXIS2_PLACEMENT_3D('',#75585,#60678,#60679);
#52758=AXIS2_PLACEMENT_3D('',#75587,#60680,#60681);
#52759=AXIS2_PLACEMENT_3D('',#75589,#60682,#60683);
#52760=AXIS2_PLACEMENT_3D('',#75591,#60684,#60685);
#52761=AXIS2_PLACEMENT_3D('',#75593,#60687,#60688);
#52762=AXIS2_PLACEMENT_3D('',#75595,#60690,#60691);
#52763=AXIS2_PLACEMENT_3D('',#75597,#60693,#60694);
#52764=AXIS2_PLACEMENT_3D('',#75599,#60696,#60697);
#52765=AXIS2_PLACEMENT_3D('',#75601,#60699,#60700);
#52766=AXIS2_PLACEMENT_3D('',#75603,#60702,#60703);
#52767=AXIS2_PLACEMENT_3D('',#75605,#60705,#60706);
#52768=AXIS2_PLACEMENT_3D('',#75607,#60708,#60709);
#52769=AXIS2_PLACEMENT_3D('',#75609,#60711,#60712);
#52770=AXIS2_PLACEMENT_3D('',#75611,#60714,#60715);
#52771=AXIS2_PLACEMENT_3D('',#75613,#60717,#60718);
#52772=AXIS2_PLACEMENT_3D('',#75615,#60720,#60721);
#52773=AXIS2_PLACEMENT_3D('',#75617,#60723,#60724);
#52774=AXIS2_PLACEMENT_3D('',#75619,#60726,#60727);
#52775=AXIS2_PLACEMENT_3D('',#75623,#60728,#60729);
#52776=AXIS2_PLACEMENT_3D('',#75627,#60732,#60733);
#52777=AXIS2_PLACEMENT_3D('',#75629,#60734,#60735);
#52778=AXIS2_PLACEMENT_3D('',#75631,#60737,#60738);
#52779=AXIS2_PLACEMENT_3D('',#75633,#60739,#60740);
#52780=AXIS2_PLACEMENT_3D('',#75635,#60742,#60743);
#52781=AXIS2_PLACEMENT_3D('',#75637,#60744,#60745);
#52782=AXIS2_PLACEMENT_3D('',#75639,#60747,#60748);
#52783=AXIS2_PLACEMENT_3D('',#75641,#60749,#60750);
#52784=AXIS2_PLACEMENT_3D('',#75643,#60752,#60753);
#52785=AXIS2_PLACEMENT_3D('',#75645,#60754,#60755);
#52786=AXIS2_PLACEMENT_3D('',#75647,#60757,#60758);
#52787=AXIS2_PLACEMENT_3D('',#75651,#60761,#60762);
#52788=AXIS2_PLACEMENT_3D('',#75653,#60763,#60764);
#52789=AXIS2_PLACEMENT_3D('',#75655,#60766,#60767);
#52790=AXIS2_PLACEMENT_3D('',#75657,#60768,#60769);
#52791=AXIS2_PLACEMENT_3D('',#75659,#60771,#60772);
#52792=AXIS2_PLACEMENT_3D('',#75661,#60773,#60774);
#52793=AXIS2_PLACEMENT_3D('',#75663,#60776,#60777);
#52794=AXIS2_PLACEMENT_3D('',#75665,#60778,#60779);
#52795=AXIS2_PLACEMENT_3D('',#75667,#60781,#60782);
#52796=AXIS2_PLACEMENT_3D('',#75669,#60783,#60784);
#52797=AXIS2_PLACEMENT_3D('',#75671,#60786,#60787);
#52798=AXIS2_PLACEMENT_3D('',#75673,#60789,#60790);
#52799=AXIS2_PLACEMENT_3D('',#75674,#60791,#60792);
#52800=AXIS2_PLACEMENT_3D('',#75676,#60793,#60794);
#52801=AXIS2_PLACEMENT_3D('',#75678,#60795,#60796);
#52802=AXIS2_PLACEMENT_3D('',#75682,#60798,#60799);
#52803=AXIS2_PLACEMENT_3D('',#75684,#60800,#60801);
#52804=AXIS2_PLACEMENT_3D('',#75686,#60802,#60803);
#52805=AXIS2_PLACEMENT_3D('',#75688,#60804,#60805);
#52806=AXIS2_PLACEMENT_3D('',#75690,#60806,#60807);
#52807=AXIS2_PLACEMENT_3D('',#75694,#60809,#60810);
#52808=AXIS2_PLACEMENT_3D('',#75696,#60811,#60812);
#52809=AXIS2_PLACEMENT_3D('',#75698,#60813,#60814);
#52810=AXIS2_PLACEMENT_3D('',#75700,#60815,#60816);
#52811=AXIS2_PLACEMENT_3D('',#75702,#60817,#60818);
#52812=AXIS2_PLACEMENT_3D('',#75704,#60820,#60821);
#52813=AXIS2_PLACEMENT_3D('',#75706,#60823,#60824);
#52814=AXIS2_PLACEMENT_3D('',#75708,#60826,#60827);
#52815=AXIS2_PLACEMENT_3D('',#75710,#60829,#60830);
#52816=AXIS2_PLACEMENT_3D('',#75712,#60832,#60833);
#52817=AXIS2_PLACEMENT_3D('',#75714,#60835,#60836);
#52818=AXIS2_PLACEMENT_3D('',#75716,#60838,#60839);
#52819=AXIS2_PLACEMENT_3D('',#75718,#60841,#60842);
#52820=AXIS2_PLACEMENT_3D('',#75720,#60844,#60845);
#52821=AXIS2_PLACEMENT_3D('',#75722,#60847,#60848);
#52822=AXIS2_PLACEMENT_3D('',#75724,#60850,#60851);
#52823=AXIS2_PLACEMENT_3D('',#75726,#60853,#60854);
#52824=AXIS2_PLACEMENT_3D('',#75728,#60856,#60857);
#52825=AXIS2_PLACEMENT_3D('',#75730,#60859,#60860);
#52826=AXIS2_PLACEMENT_3D('',#75734,#60861,#60862);
#52827=AXIS2_PLACEMENT_3D('',#75738,#60865,#60866);
#52828=AXIS2_PLACEMENT_3D('',#75740,#60867,#60868);
#52829=AXIS2_PLACEMENT_3D('',#75742,#60870,#60871);
#52830=AXIS2_PLACEMENT_3D('',#75744,#60872,#60873);
#52831=AXIS2_PLACEMENT_3D('',#75746,#60875,#60876);
#52832=AXIS2_PLACEMENT_3D('',#75748,#60877,#60878);
#52833=AXIS2_PLACEMENT_3D('',#75750,#60880,#60881);
#52834=AXIS2_PLACEMENT_3D('',#75752,#60882,#60883);
#52835=AXIS2_PLACEMENT_3D('',#75754,#60885,#60886);
#52836=AXIS2_PLACEMENT_3D('',#75756,#60887,#60888);
#52837=AXIS2_PLACEMENT_3D('',#75758,#60890,#60891);
#52838=AXIS2_PLACEMENT_3D('',#75762,#60894,#60895);
#52839=AXIS2_PLACEMENT_3D('',#75764,#60896,#60897);
#52840=AXIS2_PLACEMENT_3D('',#75766,#60899,#60900);
#52841=AXIS2_PLACEMENT_3D('',#75768,#60901,#60902);
#52842=AXIS2_PLACEMENT_3D('',#75770,#60904,#60905);
#52843=AXIS2_PLACEMENT_3D('',#75772,#60906,#60907);
#52844=AXIS2_PLACEMENT_3D('',#75774,#60909,#60910);
#52845=AXIS2_PLACEMENT_3D('',#75776,#60911,#60912);
#52846=AXIS2_PLACEMENT_3D('',#75778,#60914,#60915);
#52847=AXIS2_PLACEMENT_3D('',#75780,#60916,#60917);
#52848=AXIS2_PLACEMENT_3D('',#75782,#60919,#60920);
#52849=AXIS2_PLACEMENT_3D('',#75784,#60922,#60923);
#52850=AXIS2_PLACEMENT_3D('',#75785,#60924,#60925);
#52851=AXIS2_PLACEMENT_3D('',#75787,#60926,#60927);
#52852=AXIS2_PLACEMENT_3D('',#75789,#60928,#60929);
#52853=AXIS2_PLACEMENT_3D('',#75793,#60931,#60932);
#52854=AXIS2_PLACEMENT_3D('',#75795,#60933,#60934);
#52855=AXIS2_PLACEMENT_3D('',#75797,#60935,#60936);
#52856=AXIS2_PLACEMENT_3D('',#75799,#60937,#60938);
#52857=AXIS2_PLACEMENT_3D('',#75801,#60939,#60940);
#52858=AXIS2_PLACEMENT_3D('',#75805,#60942,#60943);
#52859=AXIS2_PLACEMENT_3D('',#75807,#60944,#60945);
#52860=AXIS2_PLACEMENT_3D('',#75809,#60946,#60947);
#52861=AXIS2_PLACEMENT_3D('',#75811,#60948,#60949);
#52862=AXIS2_PLACEMENT_3D('',#75813,#60950,#60951);
#52863=AXIS2_PLACEMENT_3D('',#75815,#60953,#60954);
#52864=AXIS2_PLACEMENT_3D('',#75817,#60956,#60957);
#52865=AXIS2_PLACEMENT_3D('',#75819,#60959,#60960);
#52866=AXIS2_PLACEMENT_3D('',#75821,#60962,#60963);
#52867=AXIS2_PLACEMENT_3D('',#75823,#60965,#60966);
#52868=AXIS2_PLACEMENT_3D('',#75825,#60968,#60969);
#52869=AXIS2_PLACEMENT_3D('',#75827,#60971,#60972);
#52870=AXIS2_PLACEMENT_3D('',#75829,#60974,#60975);
#52871=AXIS2_PLACEMENT_3D('',#75831,#60977,#60978);
#52872=AXIS2_PLACEMENT_3D('',#75833,#60980,#60981);
#52873=AXIS2_PLACEMENT_3D('',#75835,#60983,#60984);
#52874=AXIS2_PLACEMENT_3D('',#75837,#60986,#60987);
#52875=AXIS2_PLACEMENT_3D('',#75839,#60989,#60990);
#52876=AXIS2_PLACEMENT_3D('',#75841,#60992,#60993);
#52877=AXIS2_PLACEMENT_3D('',#75845,#60994,#60995);
#52878=AXIS2_PLACEMENT_3D('',#75849,#60998,#60999);
#52879=AXIS2_PLACEMENT_3D('',#75851,#61000,#61001);
#52880=AXIS2_PLACEMENT_3D('',#75853,#61003,#61004);
#52881=AXIS2_PLACEMENT_3D('',#75855,#61005,#61006);
#52882=AXIS2_PLACEMENT_3D('',#75857,#61008,#61009);
#52883=AXIS2_PLACEMENT_3D('',#75859,#61010,#61011);
#52884=AXIS2_PLACEMENT_3D('',#75861,#61013,#61014);
#52885=AXIS2_PLACEMENT_3D('',#75863,#61015,#61016);
#52886=AXIS2_PLACEMENT_3D('',#75865,#61018,#61019);
#52887=AXIS2_PLACEMENT_3D('',#75867,#61020,#61021);
#52888=AXIS2_PLACEMENT_3D('',#75869,#61023,#61024);
#52889=AXIS2_PLACEMENT_3D('',#75873,#61027,#61028);
#52890=AXIS2_PLACEMENT_3D('',#75875,#61029,#61030);
#52891=AXIS2_PLACEMENT_3D('',#75877,#61032,#61033);
#52892=AXIS2_PLACEMENT_3D('',#75879,#61034,#61035);
#52893=AXIS2_PLACEMENT_3D('',#75881,#61037,#61038);
#52894=AXIS2_PLACEMENT_3D('',#75883,#61039,#61040);
#52895=AXIS2_PLACEMENT_3D('',#75885,#61042,#61043);
#52896=AXIS2_PLACEMENT_3D('',#75887,#61044,#61045);
#52897=AXIS2_PLACEMENT_3D('',#75889,#61047,#61048);
#52898=AXIS2_PLACEMENT_3D('',#75891,#61049,#61050);
#52899=AXIS2_PLACEMENT_3D('',#75893,#61052,#61053);
#52900=AXIS2_PLACEMENT_3D('',#75895,#61055,#61056);
#52901=AXIS2_PLACEMENT_3D('',#75896,#61057,#61058);
#52902=AXIS2_PLACEMENT_3D('',#75898,#61059,#61060);
#52903=AXIS2_PLACEMENT_3D('',#75900,#61061,#61062);
#52904=AXIS2_PLACEMENT_3D('',#75904,#61064,#61065);
#52905=AXIS2_PLACEMENT_3D('',#75906,#61066,#61067);
#52906=AXIS2_PLACEMENT_3D('',#75908,#61068,#61069);
#52907=AXIS2_PLACEMENT_3D('',#75910,#61070,#61071);
#52908=AXIS2_PLACEMENT_3D('',#75912,#61072,#61073);
#52909=AXIS2_PLACEMENT_3D('',#75916,#61075,#61076);
#52910=AXIS2_PLACEMENT_3D('',#75918,#61077,#61078);
#52911=AXIS2_PLACEMENT_3D('',#75920,#61079,#61080);
#52912=AXIS2_PLACEMENT_3D('',#75922,#61081,#61082);
#52913=AXIS2_PLACEMENT_3D('',#75924,#61083,#61084);
#52914=AXIS2_PLACEMENT_3D('',#75926,#61086,#61087);
#52915=AXIS2_PLACEMENT_3D('',#75928,#61089,#61090);
#52916=AXIS2_PLACEMENT_3D('',#75930,#61092,#61093);
#52917=AXIS2_PLACEMENT_3D('',#75932,#61095,#61096);
#52918=AXIS2_PLACEMENT_3D('',#75934,#61098,#61099);
#52919=AXIS2_PLACEMENT_3D('',#75936,#61101,#61102);
#52920=AXIS2_PLACEMENT_3D('',#75938,#61104,#61105);
#52921=AXIS2_PLACEMENT_3D('',#75940,#61107,#61108);
#52922=AXIS2_PLACEMENT_3D('',#75942,#61110,#61111);
#52923=AXIS2_PLACEMENT_3D('',#75944,#61113,#61114);
#52924=AXIS2_PLACEMENT_3D('',#75946,#61116,#61117);
#52925=AXIS2_PLACEMENT_3D('',#75948,#61119,#61120);
#52926=AXIS2_PLACEMENT_3D('',#75950,#61122,#61123);
#52927=AXIS2_PLACEMENT_3D('',#75952,#61125,#61126);
#52928=AXIS2_PLACEMENT_3D('',#75956,#61127,#61128);
#52929=AXIS2_PLACEMENT_3D('',#75960,#61131,#61132);
#52930=AXIS2_PLACEMENT_3D('',#75962,#61133,#61134);
#52931=AXIS2_PLACEMENT_3D('',#75964,#61136,#61137);
#52932=AXIS2_PLACEMENT_3D('',#75966,#61138,#61139);
#52933=AXIS2_PLACEMENT_3D('',#75968,#61141,#61142);
#52934=AXIS2_PLACEMENT_3D('',#75970,#61143,#61144);
#52935=AXIS2_PLACEMENT_3D('',#75972,#61146,#61147);
#52936=AXIS2_PLACEMENT_3D('',#75974,#61148,#61149);
#52937=AXIS2_PLACEMENT_3D('',#75976,#61151,#61152);
#52938=AXIS2_PLACEMENT_3D('',#75978,#61153,#61154);
#52939=AXIS2_PLACEMENT_3D('',#75980,#61156,#61157);
#52940=AXIS2_PLACEMENT_3D('',#75984,#61160,#61161);
#52941=AXIS2_PLACEMENT_3D('',#75986,#61162,#61163);
#52942=AXIS2_PLACEMENT_3D('',#75988,#61165,#61166);
#52943=AXIS2_PLACEMENT_3D('',#75990,#61167,#61168);
#52944=AXIS2_PLACEMENT_3D('',#75992,#61170,#61171);
#52945=AXIS2_PLACEMENT_3D('',#75994,#61172,#61173);
#52946=AXIS2_PLACEMENT_3D('',#75996,#61175,#61176);
#52947=AXIS2_PLACEMENT_3D('',#75998,#61177,#61178);
#52948=AXIS2_PLACEMENT_3D('',#76000,#61180,#61181);
#52949=AXIS2_PLACEMENT_3D('',#76002,#61182,#61183);
#52950=AXIS2_PLACEMENT_3D('',#76004,#61185,#61186);
#52951=AXIS2_PLACEMENT_3D('',#76006,#61188,#61189);
#52952=AXIS2_PLACEMENT_3D('',#76007,#61190,#61191);
#52953=AXIS2_PLACEMENT_3D('',#76009,#61192,#61193);
#52954=AXIS2_PLACEMENT_3D('',#76011,#61194,#61195);
#52955=AXIS2_PLACEMENT_3D('',#76015,#61197,#61198);
#52956=AXIS2_PLACEMENT_3D('',#76017,#61199,#61200);
#52957=AXIS2_PLACEMENT_3D('',#76019,#61201,#61202);
#52958=AXIS2_PLACEMENT_3D('',#76021,#61203,#61204);
#52959=AXIS2_PLACEMENT_3D('',#76023,#61205,#61206);
#52960=AXIS2_PLACEMENT_3D('',#76027,#61208,#61209);
#52961=AXIS2_PLACEMENT_3D('',#76029,#61210,#61211);
#52962=AXIS2_PLACEMENT_3D('',#76031,#61212,#61213);
#52963=AXIS2_PLACEMENT_3D('',#76033,#61214,#61215);
#52964=AXIS2_PLACEMENT_3D('',#76035,#61216,#61217);
#52965=AXIS2_PLACEMENT_3D('',#76037,#61219,#61220);
#52966=AXIS2_PLACEMENT_3D('',#76039,#61222,#61223);
#52967=AXIS2_PLACEMENT_3D('',#76041,#61225,#61226);
#52968=AXIS2_PLACEMENT_3D('',#76043,#61228,#61229);
#52969=AXIS2_PLACEMENT_3D('',#76045,#61231,#61232);
#52970=AXIS2_PLACEMENT_3D('',#76047,#61234,#61235);
#52971=AXIS2_PLACEMENT_3D('',#76049,#61237,#61238);
#52972=AXIS2_PLACEMENT_3D('',#76051,#61240,#61241);
#52973=AXIS2_PLACEMENT_3D('',#76053,#61243,#61244);
#52974=AXIS2_PLACEMENT_3D('',#76055,#61246,#61247);
#52975=AXIS2_PLACEMENT_3D('',#76057,#61249,#61250);
#52976=AXIS2_PLACEMENT_3D('',#76059,#61252,#61253);
#52977=AXIS2_PLACEMENT_3D('',#76061,#61255,#61256);
#52978=AXIS2_PLACEMENT_3D('',#76063,#61258,#61259);
#52979=AXIS2_PLACEMENT_3D('',#76067,#61260,#61261);
#52980=AXIS2_PLACEMENT_3D('',#76071,#61264,#61265);
#52981=AXIS2_PLACEMENT_3D('',#76073,#61266,#61267);
#52982=AXIS2_PLACEMENT_3D('',#76075,#61269,#61270);
#52983=AXIS2_PLACEMENT_3D('',#76077,#61271,#61272);
#52984=AXIS2_PLACEMENT_3D('',#76079,#61274,#61275);
#52985=AXIS2_PLACEMENT_3D('',#76081,#61276,#61277);
#52986=AXIS2_PLACEMENT_3D('',#76083,#61279,#61280);
#52987=AXIS2_PLACEMENT_3D('',#76085,#61281,#61282);
#52988=AXIS2_PLACEMENT_3D('',#76087,#61284,#61285);
#52989=AXIS2_PLACEMENT_3D('',#76089,#61286,#61287);
#52990=AXIS2_PLACEMENT_3D('',#76091,#61289,#61290);
#52991=AXIS2_PLACEMENT_3D('',#76095,#61293,#61294);
#52992=AXIS2_PLACEMENT_3D('',#76097,#61295,#61296);
#52993=AXIS2_PLACEMENT_3D('',#76099,#61298,#61299);
#52994=AXIS2_PLACEMENT_3D('',#76101,#61300,#61301);
#52995=AXIS2_PLACEMENT_3D('',#76103,#61303,#61304);
#52996=AXIS2_PLACEMENT_3D('',#76105,#61305,#61306);
#52997=AXIS2_PLACEMENT_3D('',#76107,#61308,#61309);
#52998=AXIS2_PLACEMENT_3D('',#76109,#61310,#61311);
#52999=AXIS2_PLACEMENT_3D('',#76111,#61313,#61314);
#53000=AXIS2_PLACEMENT_3D('',#76113,#61315,#61316);
#53001=AXIS2_PLACEMENT_3D('',#76115,#61318,#61319);
#53002=AXIS2_PLACEMENT_3D('',#76117,#61321,#61322);
#53003=AXIS2_PLACEMENT_3D('',#76118,#61323,#61324);
#53004=AXIS2_PLACEMENT_3D('',#76120,#61325,#61326);
#53005=AXIS2_PLACEMENT_3D('',#76122,#61327,#61328);
#53006=AXIS2_PLACEMENT_3D('',#76126,#61330,#61331);
#53007=AXIS2_PLACEMENT_3D('',#76128,#61332,#61333);
#53008=AXIS2_PLACEMENT_3D('',#76130,#61334,#61335);
#53009=AXIS2_PLACEMENT_3D('',#76132,#61336,#61337);
#53010=AXIS2_PLACEMENT_3D('',#76134,#61338,#61339);
#53011=AXIS2_PLACEMENT_3D('',#76138,#61341,#61342);
#53012=AXIS2_PLACEMENT_3D('',#76140,#61343,#61344);
#53013=AXIS2_PLACEMENT_3D('',#76142,#61345,#61346);
#53014=AXIS2_PLACEMENT_3D('',#76144,#61347,#61348);
#53015=AXIS2_PLACEMENT_3D('',#76146,#61349,#61350);
#53016=AXIS2_PLACEMENT_3D('',#76148,#61352,#61353);
#53017=AXIS2_PLACEMENT_3D('',#76150,#61355,#61356);
#53018=AXIS2_PLACEMENT_3D('',#76152,#61358,#61359);
#53019=AXIS2_PLACEMENT_3D('',#76154,#61361,#61362);
#53020=AXIS2_PLACEMENT_3D('',#76156,#61364,#61365);
#53021=AXIS2_PLACEMENT_3D('',#76158,#61367,#61368);
#53022=AXIS2_PLACEMENT_3D('',#76160,#61370,#61371);
#53023=AXIS2_PLACEMENT_3D('',#76162,#61373,#61374);
#53024=AXIS2_PLACEMENT_3D('',#76164,#61376,#61377);
#53025=AXIS2_PLACEMENT_3D('',#76166,#61379,#61380);
#53026=AXIS2_PLACEMENT_3D('',#76168,#61382,#61383);
#53027=AXIS2_PLACEMENT_3D('',#76170,#61385,#61386);
#53028=AXIS2_PLACEMENT_3D('',#76172,#61388,#61389);
#53029=AXIS2_PLACEMENT_3D('',#76174,#61391,#61392);
#53030=AXIS2_PLACEMENT_3D('',#76178,#61393,#61394);
#53031=AXIS2_PLACEMENT_3D('',#76182,#61397,#61398);
#53032=AXIS2_PLACEMENT_3D('',#76184,#61399,#61400);
#53033=AXIS2_PLACEMENT_3D('',#76186,#61402,#61403);
#53034=AXIS2_PLACEMENT_3D('',#76188,#61404,#61405);
#53035=AXIS2_PLACEMENT_3D('',#76190,#61407,#61408);
#53036=AXIS2_PLACEMENT_3D('',#76192,#61409,#61410);
#53037=AXIS2_PLACEMENT_3D('',#76194,#61412,#61413);
#53038=AXIS2_PLACEMENT_3D('',#76196,#61414,#61415);
#53039=AXIS2_PLACEMENT_3D('',#76198,#61417,#61418);
#53040=AXIS2_PLACEMENT_3D('',#76200,#61419,#61420);
#53041=AXIS2_PLACEMENT_3D('',#76202,#61422,#61423);
#53042=AXIS2_PLACEMENT_3D('',#76206,#61426,#61427);
#53043=AXIS2_PLACEMENT_3D('',#76208,#61428,#61429);
#53044=AXIS2_PLACEMENT_3D('',#76210,#61431,#61432);
#53045=AXIS2_PLACEMENT_3D('',#76212,#61433,#61434);
#53046=AXIS2_PLACEMENT_3D('',#76214,#61436,#61437);
#53047=AXIS2_PLACEMENT_3D('',#76216,#61438,#61439);
#53048=AXIS2_PLACEMENT_3D('',#76218,#61441,#61442);
#53049=AXIS2_PLACEMENT_3D('',#76220,#61443,#61444);
#53050=AXIS2_PLACEMENT_3D('',#76222,#61446,#61447);
#53051=AXIS2_PLACEMENT_3D('',#76224,#61448,#61449);
#53052=AXIS2_PLACEMENT_3D('',#76226,#61451,#61452);
#53053=AXIS2_PLACEMENT_3D('',#76228,#61454,#61455);
#53054=AXIS2_PLACEMENT_3D('',#76229,#61456,#61457);
#53055=AXIS2_PLACEMENT_3D('',#76231,#61458,#61459);
#53056=AXIS2_PLACEMENT_3D('',#76233,#61460,#61461);
#53057=AXIS2_PLACEMENT_3D('',#76237,#61463,#61464);
#53058=AXIS2_PLACEMENT_3D('',#76239,#61465,#61466);
#53059=AXIS2_PLACEMENT_3D('',#76241,#61467,#61468);
#53060=AXIS2_PLACEMENT_3D('',#76243,#61469,#61470);
#53061=AXIS2_PLACEMENT_3D('',#76245,#61471,#61472);
#53062=AXIS2_PLACEMENT_3D('',#76249,#61474,#61475);
#53063=AXIS2_PLACEMENT_3D('',#76251,#61476,#61477);
#53064=AXIS2_PLACEMENT_3D('',#76253,#61478,#61479);
#53065=AXIS2_PLACEMENT_3D('',#76255,#61480,#61481);
#53066=AXIS2_PLACEMENT_3D('',#76257,#61482,#61483);
#53067=AXIS2_PLACEMENT_3D('',#76259,#61485,#61486);
#53068=AXIS2_PLACEMENT_3D('',#76261,#61488,#61489);
#53069=AXIS2_PLACEMENT_3D('',#76263,#61491,#61492);
#53070=AXIS2_PLACEMENT_3D('',#76265,#61494,#61495);
#53071=AXIS2_PLACEMENT_3D('',#76267,#61497,#61498);
#53072=AXIS2_PLACEMENT_3D('',#76269,#61500,#61501);
#53073=AXIS2_PLACEMENT_3D('',#76271,#61503,#61504);
#53074=AXIS2_PLACEMENT_3D('',#76273,#61506,#61507);
#53075=AXIS2_PLACEMENT_3D('',#76275,#61509,#61510);
#53076=AXIS2_PLACEMENT_3D('',#76277,#61512,#61513);
#53077=AXIS2_PLACEMENT_3D('',#76279,#61515,#61516);
#53078=AXIS2_PLACEMENT_3D('',#76281,#61518,#61519);
#53079=AXIS2_PLACEMENT_3D('',#76283,#61521,#61522);
#53080=AXIS2_PLACEMENT_3D('',#76285,#61524,#61525);
#53081=AXIS2_PLACEMENT_3D('',#76289,#61526,#61527);
#53082=AXIS2_PLACEMENT_3D('',#76293,#61530,#61531);
#53083=AXIS2_PLACEMENT_3D('',#76295,#61532,#61533);
#53084=AXIS2_PLACEMENT_3D('',#76297,#61535,#61536);
#53085=AXIS2_PLACEMENT_3D('',#76299,#61537,#61538);
#53086=AXIS2_PLACEMENT_3D('',#76301,#61540,#61541);
#53087=AXIS2_PLACEMENT_3D('',#76303,#61542,#61543);
#53088=AXIS2_PLACEMENT_3D('',#76305,#61545,#61546);
#53089=AXIS2_PLACEMENT_3D('',#76307,#61547,#61548);
#53090=AXIS2_PLACEMENT_3D('',#76309,#61550,#61551);
#53091=AXIS2_PLACEMENT_3D('',#76311,#61552,#61553);
#53092=AXIS2_PLACEMENT_3D('',#76313,#61555,#61556);
#53093=AXIS2_PLACEMENT_3D('',#76317,#61559,#61560);
#53094=AXIS2_PLACEMENT_3D('',#76319,#61561,#61562);
#53095=AXIS2_PLACEMENT_3D('',#76321,#61564,#61565);
#53096=AXIS2_PLACEMENT_3D('',#76323,#61566,#61567);
#53097=AXIS2_PLACEMENT_3D('',#76325,#61569,#61570);
#53098=AXIS2_PLACEMENT_3D('',#76327,#61571,#61572);
#53099=AXIS2_PLACEMENT_3D('',#76329,#61574,#61575);
#53100=AXIS2_PLACEMENT_3D('',#76331,#61576,#61577);
#53101=AXIS2_PLACEMENT_3D('',#76333,#61579,#61580);
#53102=AXIS2_PLACEMENT_3D('',#76335,#61581,#61582);
#53103=AXIS2_PLACEMENT_3D('',#76337,#61584,#61585);
#53104=AXIS2_PLACEMENT_3D('',#76339,#61587,#61588);
#53105=AXIS2_PLACEMENT_3D('',#76340,#61589,#61590);
#53106=AXIS2_PLACEMENT_3D('',#76342,#61591,#61592);
#53107=AXIS2_PLACEMENT_3D('',#76344,#61593,#61594);
#53108=AXIS2_PLACEMENT_3D('',#76348,#61596,#61597);
#53109=AXIS2_PLACEMENT_3D('',#76350,#61598,#61599);
#53110=AXIS2_PLACEMENT_3D('',#76352,#61600,#61601);
#53111=AXIS2_PLACEMENT_3D('',#76354,#61602,#61603);
#53112=AXIS2_PLACEMENT_3D('',#76356,#61604,#61605);
#53113=AXIS2_PLACEMENT_3D('',#76360,#61607,#61608);
#53114=AXIS2_PLACEMENT_3D('',#76362,#61609,#61610);
#53115=AXIS2_PLACEMENT_3D('',#76364,#61611,#61612);
#53116=AXIS2_PLACEMENT_3D('',#76366,#61613,#61614);
#53117=AXIS2_PLACEMENT_3D('',#76368,#61615,#61616);
#53118=AXIS2_PLACEMENT_3D('',#76370,#61618,#61619);
#53119=AXIS2_PLACEMENT_3D('',#76372,#61621,#61622);
#53120=AXIS2_PLACEMENT_3D('',#76374,#61624,#61625);
#53121=AXIS2_PLACEMENT_3D('',#76376,#61627,#61628);
#53122=AXIS2_PLACEMENT_3D('',#76378,#61630,#61631);
#53123=AXIS2_PLACEMENT_3D('',#76380,#61633,#61634);
#53124=AXIS2_PLACEMENT_3D('',#76382,#61636,#61637);
#53125=AXIS2_PLACEMENT_3D('',#76384,#61639,#61640);
#53126=AXIS2_PLACEMENT_3D('',#76386,#61642,#61643);
#53127=AXIS2_PLACEMENT_3D('',#76388,#61645,#61646);
#53128=AXIS2_PLACEMENT_3D('',#76390,#61648,#61649);
#53129=AXIS2_PLACEMENT_3D('',#76392,#61651,#61652);
#53130=AXIS2_PLACEMENT_3D('',#76394,#61654,#61655);
#53131=AXIS2_PLACEMENT_3D('',#76396,#61657,#61658);
#53132=AXIS2_PLACEMENT_3D('',#76400,#61659,#61660);
#53133=AXIS2_PLACEMENT_3D('',#76404,#61663,#61664);
#53134=AXIS2_PLACEMENT_3D('',#76406,#61665,#61666);
#53135=AXIS2_PLACEMENT_3D('',#76408,#61668,#61669);
#53136=AXIS2_PLACEMENT_3D('',#76410,#61670,#61671);
#53137=AXIS2_PLACEMENT_3D('',#76412,#61673,#61674);
#53138=AXIS2_PLACEMENT_3D('',#76414,#61675,#61676);
#53139=AXIS2_PLACEMENT_3D('',#76416,#61678,#61679);
#53140=AXIS2_PLACEMENT_3D('',#76418,#61680,#61681);
#53141=AXIS2_PLACEMENT_3D('',#76420,#61683,#61684);
#53142=AXIS2_PLACEMENT_3D('',#76422,#61685,#61686);
#53143=AXIS2_PLACEMENT_3D('',#76424,#61688,#61689);
#53144=AXIS2_PLACEMENT_3D('',#76428,#61692,#61693);
#53145=AXIS2_PLACEMENT_3D('',#76430,#61694,#61695);
#53146=AXIS2_PLACEMENT_3D('',#76432,#61697,#61698);
#53147=AXIS2_PLACEMENT_3D('',#76434,#61699,#61700);
#53148=AXIS2_PLACEMENT_3D('',#76436,#61702,#61703);
#53149=AXIS2_PLACEMENT_3D('',#76438,#61704,#61705);
#53150=AXIS2_PLACEMENT_3D('',#76440,#61707,#61708);
#53151=AXIS2_PLACEMENT_3D('',#76442,#61709,#61710);
#53152=AXIS2_PLACEMENT_3D('',#76444,#61712,#61713);
#53153=AXIS2_PLACEMENT_3D('',#76446,#61714,#61715);
#53154=AXIS2_PLACEMENT_3D('',#76448,#61717,#61718);
#53155=AXIS2_PLACEMENT_3D('',#76450,#61720,#61721);
#53156=AXIS2_PLACEMENT_3D('',#76451,#61722,#61723);
#53157=AXIS2_PLACEMENT_3D('',#76453,#61724,#61725);
#53158=AXIS2_PLACEMENT_3D('',#76455,#61726,#61727);
#53159=AXIS2_PLACEMENT_3D('',#76459,#61729,#61730);
#53160=AXIS2_PLACEMENT_3D('',#76461,#61731,#61732);
#53161=AXIS2_PLACEMENT_3D('',#76463,#61733,#61734);
#53162=AXIS2_PLACEMENT_3D('',#76465,#61735,#61736);
#53163=AXIS2_PLACEMENT_3D('',#76467,#61737,#61738);
#53164=AXIS2_PLACEMENT_3D('',#76471,#61740,#61741);
#53165=AXIS2_PLACEMENT_3D('',#76473,#61742,#61743);
#53166=AXIS2_PLACEMENT_3D('',#76475,#61744,#61745);
#53167=AXIS2_PLACEMENT_3D('',#76477,#61746,#61747);
#53168=AXIS2_PLACEMENT_3D('',#76479,#61748,#61749);
#53169=AXIS2_PLACEMENT_3D('',#76481,#61751,#61752);
#53170=AXIS2_PLACEMENT_3D('',#76483,#61754,#61755);
#53171=AXIS2_PLACEMENT_3D('',#76485,#61757,#61758);
#53172=AXIS2_PLACEMENT_3D('',#76487,#61760,#61761);
#53173=AXIS2_PLACEMENT_3D('',#76489,#61763,#61764);
#53174=AXIS2_PLACEMENT_3D('',#76491,#61766,#61767);
#53175=AXIS2_PLACEMENT_3D('',#76493,#61769,#61770);
#53176=AXIS2_PLACEMENT_3D('',#76495,#61772,#61773);
#53177=AXIS2_PLACEMENT_3D('',#76497,#61775,#61776);
#53178=AXIS2_PLACEMENT_3D('',#76499,#61778,#61779);
#53179=AXIS2_PLACEMENT_3D('',#76501,#61781,#61782);
#53180=AXIS2_PLACEMENT_3D('',#76503,#61784,#61785);
#53181=AXIS2_PLACEMENT_3D('',#76505,#61787,#61788);
#53182=AXIS2_PLACEMENT_3D('',#76507,#61790,#61791);
#53183=AXIS2_PLACEMENT_3D('',#76511,#61792,#61793);
#53184=AXIS2_PLACEMENT_3D('',#76515,#61796,#61797);
#53185=AXIS2_PLACEMENT_3D('',#76517,#61798,#61799);
#53186=AXIS2_PLACEMENT_3D('',#76519,#61801,#61802);
#53187=AXIS2_PLACEMENT_3D('',#76521,#61803,#61804);
#53188=AXIS2_PLACEMENT_3D('',#76523,#61806,#61807);
#53189=AXIS2_PLACEMENT_3D('',#76525,#61808,#61809);
#53190=AXIS2_PLACEMENT_3D('',#76527,#61811,#61812);
#53191=AXIS2_PLACEMENT_3D('',#76529,#61813,#61814);
#53192=AXIS2_PLACEMENT_3D('',#76531,#61816,#61817);
#53193=AXIS2_PLACEMENT_3D('',#76533,#61818,#61819);
#53194=AXIS2_PLACEMENT_3D('',#76535,#61821,#61822);
#53195=AXIS2_PLACEMENT_3D('',#76539,#61825,#61826);
#53196=AXIS2_PLACEMENT_3D('',#76541,#61827,#61828);
#53197=AXIS2_PLACEMENT_3D('',#76543,#61830,#61831);
#53198=AXIS2_PLACEMENT_3D('',#76545,#61832,#61833);
#53199=AXIS2_PLACEMENT_3D('',#76547,#61835,#61836);
#53200=AXIS2_PLACEMENT_3D('',#76549,#61837,#61838);
#53201=AXIS2_PLACEMENT_3D('',#76551,#61840,#61841);
#53202=AXIS2_PLACEMENT_3D('',#76553,#61842,#61843);
#53203=AXIS2_PLACEMENT_3D('',#76555,#61845,#61846);
#53204=AXIS2_PLACEMENT_3D('',#76557,#61847,#61848);
#53205=AXIS2_PLACEMENT_3D('',#76559,#61850,#61851);
#53206=AXIS2_PLACEMENT_3D('',#76561,#61853,#61854);
#53207=AXIS2_PLACEMENT_3D('',#76562,#61855,#61856);
#53208=AXIS2_PLACEMENT_3D('',#76564,#61857,#61858);
#53209=AXIS2_PLACEMENT_3D('',#76566,#61859,#61860);
#53210=AXIS2_PLACEMENT_3D('',#76570,#61862,#61863);
#53211=AXIS2_PLACEMENT_3D('',#76572,#61864,#61865);
#53212=AXIS2_PLACEMENT_3D('',#76574,#61866,#61867);
#53213=AXIS2_PLACEMENT_3D('',#76576,#61868,#61869);
#53214=AXIS2_PLACEMENT_3D('',#76578,#61870,#61871);
#53215=AXIS2_PLACEMENT_3D('',#76582,#61873,#61874);
#53216=AXIS2_PLACEMENT_3D('',#76584,#61875,#61876);
#53217=AXIS2_PLACEMENT_3D('',#76586,#61877,#61878);
#53218=AXIS2_PLACEMENT_3D('',#76588,#61879,#61880);
#53219=AXIS2_PLACEMENT_3D('',#76590,#61881,#61882);
#53220=AXIS2_PLACEMENT_3D('',#76592,#61884,#61885);
#53221=AXIS2_PLACEMENT_3D('',#76594,#61887,#61888);
#53222=AXIS2_PLACEMENT_3D('',#76596,#61890,#61891);
#53223=AXIS2_PLACEMENT_3D('',#76598,#61893,#61894);
#53224=AXIS2_PLACEMENT_3D('',#76600,#61896,#61897);
#53225=AXIS2_PLACEMENT_3D('',#76602,#61899,#61900);
#53226=AXIS2_PLACEMENT_3D('',#76604,#61902,#61903);
#53227=AXIS2_PLACEMENT_3D('',#76606,#61905,#61906);
#53228=AXIS2_PLACEMENT_3D('',#76608,#61908,#61909);
#53229=AXIS2_PLACEMENT_3D('',#76610,#61911,#61912);
#53230=AXIS2_PLACEMENT_3D('',#76612,#61914,#61915);
#53231=AXIS2_PLACEMENT_3D('',#76614,#61917,#61918);
#53232=AXIS2_PLACEMENT_3D('',#76616,#61920,#61921);
#53233=AXIS2_PLACEMENT_3D('',#76618,#61923,#61924);
#53234=AXIS2_PLACEMENT_3D('',#76622,#61925,#61926);
#53235=AXIS2_PLACEMENT_3D('',#76626,#61929,#61930);
#53236=AXIS2_PLACEMENT_3D('',#76628,#61931,#61932);
#53237=AXIS2_PLACEMENT_3D('',#76630,#61934,#61935);
#53238=AXIS2_PLACEMENT_3D('',#76632,#61936,#61937);
#53239=AXIS2_PLACEMENT_3D('',#76634,#61939,#61940);
#53240=AXIS2_PLACEMENT_3D('',#76636,#61941,#61942);
#53241=AXIS2_PLACEMENT_3D('',#76638,#61944,#61945);
#53242=AXIS2_PLACEMENT_3D('',#76640,#61946,#61947);
#53243=AXIS2_PLACEMENT_3D('',#76642,#61949,#61950);
#53244=AXIS2_PLACEMENT_3D('',#76644,#61951,#61952);
#53245=AXIS2_PLACEMENT_3D('',#76646,#61954,#61955);
#53246=AXIS2_PLACEMENT_3D('',#76650,#61958,#61959);
#53247=AXIS2_PLACEMENT_3D('',#76652,#61960,#61961);
#53248=AXIS2_PLACEMENT_3D('',#76654,#61963,#61964);
#53249=AXIS2_PLACEMENT_3D('',#76656,#61965,#61966);
#53250=AXIS2_PLACEMENT_3D('',#76658,#61968,#61969);
#53251=AXIS2_PLACEMENT_3D('',#76660,#61970,#61971);
#53252=AXIS2_PLACEMENT_3D('',#76662,#61973,#61974);
#53253=AXIS2_PLACEMENT_3D('',#76664,#61975,#61976);
#53254=AXIS2_PLACEMENT_3D('',#76666,#61978,#61979);
#53255=AXIS2_PLACEMENT_3D('',#76668,#61980,#61981);
#53256=AXIS2_PLACEMENT_3D('',#76670,#61983,#61984);
#53257=AXIS2_PLACEMENT_3D('',#76672,#61986,#61987);
#53258=AXIS2_PLACEMENT_3D('',#76673,#61988,#61989);
#53259=AXIS2_PLACEMENT_3D('',#76675,#61990,#61991);
#53260=AXIS2_PLACEMENT_3D('',#76677,#61992,#61993);
#53261=AXIS2_PLACEMENT_3D('',#76681,#61995,#61996);
#53262=AXIS2_PLACEMENT_3D('',#76683,#61997,#61998);
#53263=AXIS2_PLACEMENT_3D('',#76685,#61999,#62000);
#53264=AXIS2_PLACEMENT_3D('',#76687,#62001,#62002);
#53265=AXIS2_PLACEMENT_3D('',#76689,#62003,#62004);
#53266=AXIS2_PLACEMENT_3D('',#76693,#62006,#62007);
#53267=AXIS2_PLACEMENT_3D('',#76695,#62008,#62009);
#53268=AXIS2_PLACEMENT_3D('',#76697,#62010,#62011);
#53269=AXIS2_PLACEMENT_3D('',#76699,#62012,#62013);
#53270=AXIS2_PLACEMENT_3D('',#76701,#62014,#62015);
#53271=AXIS2_PLACEMENT_3D('',#76703,#62017,#62018);
#53272=AXIS2_PLACEMENT_3D('',#76705,#62020,#62021);
#53273=AXIS2_PLACEMENT_3D('',#76707,#62023,#62024);
#53274=AXIS2_PLACEMENT_3D('',#76709,#62026,#62027);
#53275=AXIS2_PLACEMENT_3D('',#76711,#62029,#62030);
#53276=AXIS2_PLACEMENT_3D('',#76713,#62032,#62033);
#53277=AXIS2_PLACEMENT_3D('',#76715,#62035,#62036);
#53278=AXIS2_PLACEMENT_3D('',#76717,#62038,#62039);
#53279=AXIS2_PLACEMENT_3D('',#76719,#62041,#62042);
#53280=AXIS2_PLACEMENT_3D('',#76721,#62044,#62045);
#53281=AXIS2_PLACEMENT_3D('',#76723,#62047,#62048);
#53282=AXIS2_PLACEMENT_3D('',#76725,#62050,#62051);
#53283=AXIS2_PLACEMENT_3D('',#76727,#62053,#62054);
#53284=AXIS2_PLACEMENT_3D('',#76729,#62056,#62057);
#53285=AXIS2_PLACEMENT_3D('',#76733,#62058,#62059);
#53286=AXIS2_PLACEMENT_3D('',#76737,#62062,#62063);
#53287=AXIS2_PLACEMENT_3D('',#76739,#62064,#62065);
#53288=AXIS2_PLACEMENT_3D('',#76741,#62067,#62068);
#53289=AXIS2_PLACEMENT_3D('',#76743,#62069,#62070);
#53290=AXIS2_PLACEMENT_3D('',#76745,#62072,#62073);
#53291=AXIS2_PLACEMENT_3D('',#76747,#62074,#62075);
#53292=AXIS2_PLACEMENT_3D('',#76749,#62077,#62078);
#53293=AXIS2_PLACEMENT_3D('',#76751,#62079,#62080);
#53294=AXIS2_PLACEMENT_3D('',#76753,#62082,#62083);
#53295=AXIS2_PLACEMENT_3D('',#76755,#62084,#62085);
#53296=AXIS2_PLACEMENT_3D('',#76757,#62087,#62088);
#53297=AXIS2_PLACEMENT_3D('',#76761,#62091,#62092);
#53298=AXIS2_PLACEMENT_3D('',#76763,#62093,#62094);
#53299=AXIS2_PLACEMENT_3D('',#76765,#62096,#62097);
#53300=AXIS2_PLACEMENT_3D('',#76767,#62098,#62099);
#53301=AXIS2_PLACEMENT_3D('',#76769,#62101,#62102);
#53302=AXIS2_PLACEMENT_3D('',#76771,#62103,#62104);
#53303=AXIS2_PLACEMENT_3D('',#76773,#62106,#62107);
#53304=AXIS2_PLACEMENT_3D('',#76775,#62108,#62109);
#53305=AXIS2_PLACEMENT_3D('',#76777,#62111,#62112);
#53306=AXIS2_PLACEMENT_3D('',#76779,#62113,#62114);
#53307=AXIS2_PLACEMENT_3D('',#76781,#62116,#62117);
#53308=AXIS2_PLACEMENT_3D('',#76783,#62119,#62120);
#53309=AXIS2_PLACEMENT_3D('',#76784,#62121,#62122);
#53310=AXIS2_PLACEMENT_3D('',#76786,#62123,#62124);
#53311=AXIS2_PLACEMENT_3D('',#76788,#62125,#62126);
#53312=AXIS2_PLACEMENT_3D('',#76792,#62128,#62129);
#53313=AXIS2_PLACEMENT_3D('',#76794,#62130,#62131);
#53314=AXIS2_PLACEMENT_3D('',#76796,#62132,#62133);
#53315=AXIS2_PLACEMENT_3D('',#76798,#62134,#62135);
#53316=AXIS2_PLACEMENT_3D('',#76800,#62136,#62137);
#53317=AXIS2_PLACEMENT_3D('',#76804,#62139,#62140);
#53318=AXIS2_PLACEMENT_3D('',#76806,#62141,#62142);
#53319=AXIS2_PLACEMENT_3D('',#76808,#62143,#62144);
#53320=AXIS2_PLACEMENT_3D('',#76810,#62145,#62146);
#53321=AXIS2_PLACEMENT_3D('',#76812,#62147,#62148);
#53322=AXIS2_PLACEMENT_3D('',#76814,#62150,#62151);
#53323=AXIS2_PLACEMENT_3D('',#76816,#62153,#62154);
#53324=AXIS2_PLACEMENT_3D('',#76818,#62156,#62157);
#53325=AXIS2_PLACEMENT_3D('',#76820,#62159,#62160);
#53326=AXIS2_PLACEMENT_3D('',#76822,#62162,#62163);
#53327=AXIS2_PLACEMENT_3D('',#76824,#62165,#62166);
#53328=AXIS2_PLACEMENT_3D('',#76826,#62168,#62169);
#53329=AXIS2_PLACEMENT_3D('',#76828,#62171,#62172);
#53330=AXIS2_PLACEMENT_3D('',#76830,#62174,#62175);
#53331=AXIS2_PLACEMENT_3D('',#76832,#62177,#62178);
#53332=AXIS2_PLACEMENT_3D('',#76834,#62180,#62181);
#53333=AXIS2_PLACEMENT_3D('',#76836,#62183,#62184);
#53334=AXIS2_PLACEMENT_3D('',#76838,#62186,#62187);
#53335=AXIS2_PLACEMENT_3D('',#76840,#62189,#62190);
#53336=AXIS2_PLACEMENT_3D('',#76844,#62191,#62192);
#53337=AXIS2_PLACEMENT_3D('',#76848,#62195,#62196);
#53338=AXIS2_PLACEMENT_3D('',#76850,#62197,#62198);
#53339=AXIS2_PLACEMENT_3D('',#76852,#62200,#62201);
#53340=AXIS2_PLACEMENT_3D('',#76854,#62202,#62203);
#53341=AXIS2_PLACEMENT_3D('',#76856,#62205,#62206);
#53342=AXIS2_PLACEMENT_3D('',#76858,#62207,#62208);
#53343=AXIS2_PLACEMENT_3D('',#76860,#62210,#62211);
#53344=AXIS2_PLACEMENT_3D('',#76862,#62212,#62213);
#53345=AXIS2_PLACEMENT_3D('',#76864,#62215,#62216);
#53346=AXIS2_PLACEMENT_3D('',#76866,#62217,#62218);
#53347=AXIS2_PLACEMENT_3D('',#76868,#62220,#62221);
#53348=AXIS2_PLACEMENT_3D('',#76872,#62224,#62225);
#53349=AXIS2_PLACEMENT_3D('',#76874,#62226,#62227);
#53350=AXIS2_PLACEMENT_3D('',#76876,#62229,#62230);
#53351=AXIS2_PLACEMENT_3D('',#76878,#62231,#62232);
#53352=AXIS2_PLACEMENT_3D('',#76880,#62234,#62235);
#53353=AXIS2_PLACEMENT_3D('',#76882,#62236,#62237);
#53354=AXIS2_PLACEMENT_3D('',#76884,#62239,#62240);
#53355=AXIS2_PLACEMENT_3D('',#76886,#62241,#62242);
#53356=AXIS2_PLACEMENT_3D('',#76888,#62244,#62245);
#53357=AXIS2_PLACEMENT_3D('',#76890,#62246,#62247);
#53358=AXIS2_PLACEMENT_3D('',#76892,#62249,#62250);
#53359=AXIS2_PLACEMENT_3D('',#76894,#62252,#62253);
#53360=AXIS2_PLACEMENT_3D('',#76895,#62254,#62255);
#53361=AXIS2_PLACEMENT_3D('',#76897,#62256,#62257);
#53362=AXIS2_PLACEMENT_3D('',#76899,#62258,#62259);
#53363=AXIS2_PLACEMENT_3D('',#76903,#62261,#62262);
#53364=AXIS2_PLACEMENT_3D('',#76905,#62263,#62264);
#53365=AXIS2_PLACEMENT_3D('',#76907,#62265,#62266);
#53366=AXIS2_PLACEMENT_3D('',#76909,#62267,#62268);
#53367=AXIS2_PLACEMENT_3D('',#76911,#62269,#62270);
#53368=AXIS2_PLACEMENT_3D('',#76915,#62272,#62273);
#53369=AXIS2_PLACEMENT_3D('',#76917,#62274,#62275);
#53370=AXIS2_PLACEMENT_3D('',#76919,#62276,#62277);
#53371=AXIS2_PLACEMENT_3D('',#76921,#62278,#62279);
#53372=AXIS2_PLACEMENT_3D('',#76923,#62280,#62281);
#53373=AXIS2_PLACEMENT_3D('',#76925,#62283,#62284);
#53374=AXIS2_PLACEMENT_3D('',#76927,#62286,#62287);
#53375=AXIS2_PLACEMENT_3D('',#76929,#62289,#62290);
#53376=AXIS2_PLACEMENT_3D('',#76931,#62292,#62293);
#53377=AXIS2_PLACEMENT_3D('',#76933,#62295,#62296);
#53378=AXIS2_PLACEMENT_3D('',#76935,#62298,#62299);
#53379=AXIS2_PLACEMENT_3D('',#76937,#62301,#62302);
#53380=AXIS2_PLACEMENT_3D('',#76939,#62304,#62305);
#53381=AXIS2_PLACEMENT_3D('',#76941,#62307,#62308);
#53382=AXIS2_PLACEMENT_3D('',#76943,#62310,#62311);
#53383=AXIS2_PLACEMENT_3D('',#76945,#62313,#62314);
#53384=AXIS2_PLACEMENT_3D('',#76947,#62316,#62317);
#53385=AXIS2_PLACEMENT_3D('',#76949,#62319,#62320);
#53386=AXIS2_PLACEMENT_3D('',#76951,#62322,#62323);
#53387=AXIS2_PLACEMENT_3D('',#76955,#62324,#62325);
#53388=AXIS2_PLACEMENT_3D('',#76959,#62328,#62329);
#53389=AXIS2_PLACEMENT_3D('',#76961,#62330,#62331);
#53390=AXIS2_PLACEMENT_3D('',#76963,#62333,#62334);
#53391=AXIS2_PLACEMENT_3D('',#76965,#62335,#62336);
#53392=AXIS2_PLACEMENT_3D('',#76967,#62338,#62339);
#53393=AXIS2_PLACEMENT_3D('',#76969,#62340,#62341);
#53394=AXIS2_PLACEMENT_3D('',#76971,#62343,#62344);
#53395=AXIS2_PLACEMENT_3D('',#76973,#62345,#62346);
#53396=AXIS2_PLACEMENT_3D('',#76975,#62348,#62349);
#53397=AXIS2_PLACEMENT_3D('',#76977,#62350,#62351);
#53398=AXIS2_PLACEMENT_3D('',#76979,#62353,#62354);
#53399=AXIS2_PLACEMENT_3D('',#76983,#62357,#62358);
#53400=AXIS2_PLACEMENT_3D('',#76985,#62359,#62360);
#53401=AXIS2_PLACEMENT_3D('',#76987,#62362,#62363);
#53402=AXIS2_PLACEMENT_3D('',#76989,#62364,#62365);
#53403=AXIS2_PLACEMENT_3D('',#76991,#62367,#62368);
#53404=AXIS2_PLACEMENT_3D('',#76993,#62369,#62370);
#53405=AXIS2_PLACEMENT_3D('',#76995,#62372,#62373);
#53406=AXIS2_PLACEMENT_3D('',#76997,#62374,#62375);
#53407=AXIS2_PLACEMENT_3D('',#76999,#62377,#62378);
#53408=AXIS2_PLACEMENT_3D('',#77001,#62379,#62380);
#53409=AXIS2_PLACEMENT_3D('',#77003,#62382,#62383);
#53410=AXIS2_PLACEMENT_3D('',#77005,#62385,#62386);
#53411=AXIS2_PLACEMENT_3D('',#77006,#62387,#62388);
#53412=AXIS2_PLACEMENT_3D('',#77008,#62389,#62390);
#53413=AXIS2_PLACEMENT_3D('',#77010,#62391,#62392);
#53414=AXIS2_PLACEMENT_3D('',#77014,#62394,#62395);
#53415=AXIS2_PLACEMENT_3D('',#77016,#62396,#62397);
#53416=AXIS2_PLACEMENT_3D('',#77018,#62398,#62399);
#53417=AXIS2_PLACEMENT_3D('',#77020,#62400,#62401);
#53418=AXIS2_PLACEMENT_3D('',#77022,#62402,#62403);
#53419=AXIS2_PLACEMENT_3D('',#77026,#62405,#62406);
#53420=AXIS2_PLACEMENT_3D('',#77028,#62407,#62408);
#53421=AXIS2_PLACEMENT_3D('',#77030,#62409,#62410);
#53422=AXIS2_PLACEMENT_3D('',#77032,#62411,#62412);
#53423=AXIS2_PLACEMENT_3D('',#77034,#62413,#62414);
#53424=AXIS2_PLACEMENT_3D('',#77036,#62416,#62417);
#53425=AXIS2_PLACEMENT_3D('',#77038,#62419,#62420);
#53426=AXIS2_PLACEMENT_3D('',#77040,#62422,#62423);
#53427=AXIS2_PLACEMENT_3D('',#77042,#62425,#62426);
#53428=AXIS2_PLACEMENT_3D('',#77044,#62428,#62429);
#53429=AXIS2_PLACEMENT_3D('',#77046,#62431,#62432);
#53430=AXIS2_PLACEMENT_3D('',#77048,#62434,#62435);
#53431=AXIS2_PLACEMENT_3D('',#77050,#62437,#62438);
#53432=AXIS2_PLACEMENT_3D('',#77052,#62440,#62441);
#53433=AXIS2_PLACEMENT_3D('',#77054,#62443,#62444);
#53434=AXIS2_PLACEMENT_3D('',#77056,#62446,#62447);
#53435=AXIS2_PLACEMENT_3D('',#77058,#62449,#62450);
#53436=AXIS2_PLACEMENT_3D('',#77060,#62452,#62453);
#53437=AXIS2_PLACEMENT_3D('',#77062,#62455,#62456);
#53438=AXIS2_PLACEMENT_3D('',#77066,#62457,#62458);
#53439=AXIS2_PLACEMENT_3D('',#77070,#62461,#62462);
#53440=AXIS2_PLACEMENT_3D('',#77072,#62463,#62464);
#53441=AXIS2_PLACEMENT_3D('',#77074,#62466,#62467);
#53442=AXIS2_PLACEMENT_3D('',#77076,#62468,#62469);
#53443=AXIS2_PLACEMENT_3D('',#77078,#62471,#62472);
#53444=AXIS2_PLACEMENT_3D('',#77080,#62473,#62474);
#53445=AXIS2_PLACEMENT_3D('',#77082,#62476,#62477);
#53446=AXIS2_PLACEMENT_3D('',#77084,#62478,#62479);
#53447=AXIS2_PLACEMENT_3D('',#77086,#62481,#62482);
#53448=AXIS2_PLACEMENT_3D('',#77088,#62483,#62484);
#53449=AXIS2_PLACEMENT_3D('',#77090,#62486,#62487);
#53450=AXIS2_PLACEMENT_3D('',#77094,#62490,#62491);
#53451=AXIS2_PLACEMENT_3D('',#77096,#62492,#62493);
#53452=AXIS2_PLACEMENT_3D('',#77098,#62495,#62496);
#53453=AXIS2_PLACEMENT_3D('',#77100,#62497,#62498);
#53454=AXIS2_PLACEMENT_3D('',#77102,#62500,#62501);
#53455=AXIS2_PLACEMENT_3D('',#77104,#62502,#62503);
#53456=AXIS2_PLACEMENT_3D('',#77106,#62505,#62506);
#53457=AXIS2_PLACEMENT_3D('',#77108,#62507,#62508);
#53458=AXIS2_PLACEMENT_3D('',#77110,#62510,#62511);
#53459=AXIS2_PLACEMENT_3D('',#77112,#62512,#62513);
#53460=AXIS2_PLACEMENT_3D('',#77114,#62515,#62516);
#53461=AXIS2_PLACEMENT_3D('',#77116,#62518,#62519);
#53462=AXIS2_PLACEMENT_3D('',#77117,#62520,#62521);
#53463=AXIS2_PLACEMENT_3D('',#77119,#62522,#62523);
#53464=AXIS2_PLACEMENT_3D('',#77121,#62524,#62525);
#53465=AXIS2_PLACEMENT_3D('',#77125,#62527,#62528);
#53466=AXIS2_PLACEMENT_3D('',#77127,#62529,#62530);
#53467=AXIS2_PLACEMENT_3D('',#77129,#62531,#62532);
#53468=AXIS2_PLACEMENT_3D('',#77131,#62533,#62534);
#53469=AXIS2_PLACEMENT_3D('',#77133,#62535,#62536);
#53470=AXIS2_PLACEMENT_3D('',#77137,#62538,#62539);
#53471=AXIS2_PLACEMENT_3D('',#77139,#62540,#62541);
#53472=AXIS2_PLACEMENT_3D('',#77141,#62542,#62543);
#53473=AXIS2_PLACEMENT_3D('',#77143,#62544,#62545);
#53474=AXIS2_PLACEMENT_3D('',#77145,#62546,#62547);
#53475=AXIS2_PLACEMENT_3D('',#77147,#62549,#62550);
#53476=AXIS2_PLACEMENT_3D('',#77149,#62552,#62553);
#53477=AXIS2_PLACEMENT_3D('',#77151,#62555,#62556);
#53478=AXIS2_PLACEMENT_3D('',#77153,#62558,#62559);
#53479=AXIS2_PLACEMENT_3D('',#77155,#62561,#62562);
#53480=AXIS2_PLACEMENT_3D('',#77157,#62564,#62565);
#53481=AXIS2_PLACEMENT_3D('',#77159,#62567,#62568);
#53482=AXIS2_PLACEMENT_3D('',#77161,#62570,#62571);
#53483=AXIS2_PLACEMENT_3D('',#77163,#62573,#62574);
#53484=AXIS2_PLACEMENT_3D('',#77165,#62576,#62577);
#53485=AXIS2_PLACEMENT_3D('',#77167,#62579,#62580);
#53486=AXIS2_PLACEMENT_3D('',#77169,#62582,#62583);
#53487=AXIS2_PLACEMENT_3D('',#77171,#62585,#62586);
#53488=AXIS2_PLACEMENT_3D('',#77173,#62588,#62589);
#53489=AXIS2_PLACEMENT_3D('',#77177,#62590,#62591);
#53490=AXIS2_PLACEMENT_3D('',#77181,#62594,#62595);
#53491=AXIS2_PLACEMENT_3D('',#77183,#62596,#62597);
#53492=AXIS2_PLACEMENT_3D('',#77185,#62599,#62600);
#53493=AXIS2_PLACEMENT_3D('',#77187,#62601,#62602);
#53494=AXIS2_PLACEMENT_3D('',#77189,#62604,#62605);
#53495=AXIS2_PLACEMENT_3D('',#77191,#62606,#62607);
#53496=AXIS2_PLACEMENT_3D('',#77193,#62609,#62610);
#53497=AXIS2_PLACEMENT_3D('',#77195,#62611,#62612);
#53498=AXIS2_PLACEMENT_3D('',#77197,#62614,#62615);
#53499=AXIS2_PLACEMENT_3D('',#77199,#62616,#62617);
#53500=AXIS2_PLACEMENT_3D('',#77201,#62619,#62620);
#53501=AXIS2_PLACEMENT_3D('',#77205,#62623,#62624);
#53502=AXIS2_PLACEMENT_3D('',#77207,#62625,#62626);
#53503=AXIS2_PLACEMENT_3D('',#77209,#62628,#62629);
#53504=AXIS2_PLACEMENT_3D('',#77211,#62630,#62631);
#53505=AXIS2_PLACEMENT_3D('',#77213,#62633,#62634);
#53506=AXIS2_PLACEMENT_3D('',#77215,#62635,#62636);
#53507=AXIS2_PLACEMENT_3D('',#77217,#62638,#62639);
#53508=AXIS2_PLACEMENT_3D('',#77219,#62640,#62641);
#53509=AXIS2_PLACEMENT_3D('',#77221,#62643,#62644);
#53510=AXIS2_PLACEMENT_3D('',#77223,#62645,#62646);
#53511=AXIS2_PLACEMENT_3D('',#77225,#62648,#62649);
#53512=AXIS2_PLACEMENT_3D('',#77227,#62651,#62652);
#53513=AXIS2_PLACEMENT_3D('',#77228,#62653,#62654);
#53514=AXIS2_PLACEMENT_3D('',#77230,#62655,#62656);
#53515=AXIS2_PLACEMENT_3D('',#77232,#62657,#62658);
#53516=AXIS2_PLACEMENT_3D('',#77236,#62660,#62661);
#53517=AXIS2_PLACEMENT_3D('',#77238,#62662,#62663);
#53518=AXIS2_PLACEMENT_3D('',#77240,#62664,#62665);
#53519=AXIS2_PLACEMENT_3D('',#77242,#62666,#62667);
#53520=AXIS2_PLACEMENT_3D('',#77244,#62668,#62669);
#53521=AXIS2_PLACEMENT_3D('',#77248,#62671,#62672);
#53522=AXIS2_PLACEMENT_3D('',#77250,#62673,#62674);
#53523=AXIS2_PLACEMENT_3D('',#77252,#62675,#62676);
#53524=AXIS2_PLACEMENT_3D('',#77254,#62677,#62678);
#53525=AXIS2_PLACEMENT_3D('',#77256,#62679,#62680);
#53526=AXIS2_PLACEMENT_3D('',#77258,#62682,#62683);
#53527=AXIS2_PLACEMENT_3D('',#77262,#62686,#62687);
#53528=AXIS2_PLACEMENT_3D('',#77264,#62688,#62689);
#53529=AXIS2_PLACEMENT_3D('',#77266,#62691,#62692);
#53530=AXIS2_PLACEMENT_3D('',#77268,#62693,#62694);
#53531=AXIS2_PLACEMENT_3D('',#77270,#62696,#62697);
#53532=AXIS2_PLACEMENT_3D('',#77272,#62698,#62699);
#53533=AXIS2_PLACEMENT_3D('',#77274,#62701,#62702);
#53534=AXIS2_PLACEMENT_3D('',#77276,#62703,#62704);
#53535=AXIS2_PLACEMENT_3D('',#77278,#62706,#62707);
#53536=AXIS2_PLACEMENT_3D('',#77280,#62708,#62709);
#53537=AXIS2_PLACEMENT_3D('',#77282,#62711,#62712);
#53538=AXIS2_PLACEMENT_3D('',#77286,#62715,#62716);
#53539=AXIS2_PLACEMENT_3D('',#77288,#62717,#62718);
#53540=AXIS2_PLACEMENT_3D('',#77290,#62720,#62721);
#53541=AXIS2_PLACEMENT_3D('',#77292,#62722,#62723);
#53542=AXIS2_PLACEMENT_3D('',#77294,#62725,#62726);
#53543=AXIS2_PLACEMENT_3D('',#77296,#62727,#62728);
#53544=AXIS2_PLACEMENT_3D('',#77298,#62730,#62731);
#53545=AXIS2_PLACEMENT_3D('',#77300,#62732,#62733);
#53546=AXIS2_PLACEMENT_3D('',#77302,#62735,#62736);
#53547=AXIS2_PLACEMENT_3D('',#77304,#62737,#62738);
#53548=AXIS2_PLACEMENT_3D('',#77306,#62740,#62741);
#53549=AXIS2_PLACEMENT_3D('',#77310,#62744,#62745);
#53550=AXIS2_PLACEMENT_3D('',#77311,#62746,#62747);
#53551=AXIS2_PLACEMENT_3D('',#77312,#62748,#62749);
#53552=AXIS2_PLACEMENT_3D('',#77314,#62751,#62752);
#53553=AXIS2_PLACEMENT_3D('',#77316,#62754,#62755);
#53554=AXIS2_PLACEMENT_3D('',#77318,#62757,#62758);
#53555=AXIS2_PLACEMENT_3D('',#77320,#62760,#62761);
#53556=AXIS2_PLACEMENT_3D('',#77322,#62763,#62764);
#53557=AXIS2_PLACEMENT_3D('',#77324,#62766,#62767);
#53558=AXIS2_PLACEMENT_3D('',#77326,#62769,#62770);
#53559=AXIS2_PLACEMENT_3D('',#77328,#62772,#62773);
#53560=AXIS2_PLACEMENT_3D('',#77330,#62775,#62776);
#53561=AXIS2_PLACEMENT_3D('',#77332,#62778,#62779);
#53562=AXIS2_PLACEMENT_3D('',#77334,#62781,#62782);
#53563=AXIS2_PLACEMENT_3D('',#77336,#62784,#62785);
#53564=AXIS2_PLACEMENT_3D('',#77338,#62787,#62788);
#53565=AXIS2_PLACEMENT_3D('',#77342,#62789,#62790);
#53566=AXIS2_PLACEMENT_3D('',#77343,#62791,#62792);
#53567=AXIS2_PLACEMENT_3D('',#77346,#62794,#62795);
#53568=AXIS2_PLACEMENT_3D('',#77347,#62796,#62797);
#53569=AXIS2_PLACEMENT_3D('',#77349,#62798,#62799);
#53570=AXIS2_PLACEMENT_3D('',#77353,#62801,#62802);
#53571=AXIS2_PLACEMENT_3D('',#77354,#62803,#62804);
#53572=AXIS2_PLACEMENT_3D('',#77355,#62805,#62806);
#53573=AXIS2_PLACEMENT_3D('',#77359,#62808,#62809);
#53574=AXIS2_PLACEMENT_3D('',#77360,#62810,#62811);
#53575=AXIS2_PLACEMENT_3D('',#77361,#62812,#62813);
#53576=AXIS2_PLACEMENT_3D('',#77362,#62814,#62815);
#53577=AXIS2_PLACEMENT_3D('',#77364,#62816,#62817);
#53578=AXIS2_PLACEMENT_3D('',#77366,#62818,#62819);
#53579=AXIS2_PLACEMENT_3D('',#77367,#62820,#62821);
#53580=AXIS2_PLACEMENT_3D('',#77368,#62822,#62823);
#53581=AXIS2_PLACEMENT_3D('',#77371,#62825,#62826);
#53582=AXIS2_PLACEMENT_3D('',#77372,#62827,#62828);
#53583=AXIS2_PLACEMENT_3D('',#77375,#62829,#62830);
#53584=AXIS2_PLACEMENT_3D('',#77377,#62831,#62832);
#53585=AXIS2_PLACEMENT_3D('',#77378,#62833,#62834);
#53586=AXIS2_PLACEMENT_3D('',#77379,#62835,#62836);
#53587=AXIS2_PLACEMENT_3D('',#77380,#62837,#62838);
#53588=AXIS2_PLACEMENT_3D('',#77384,#62840,#62841);
#53589=AXIS2_PLACEMENT_3D('',#77385,#62842,#62843);
#53590=AXIS2_PLACEMENT_3D('',#77386,#62844,#62845);
#53591=AXIS2_PLACEMENT_3D('',#77388,#62846,#62847);
#53592=AXIS2_PLACEMENT_3D('',#77389,#62848,#62849);
#53593=AXIS2_PLACEMENT_3D('',#77391,#62850,#62851);
#53594=AXIS2_PLACEMENT_3D('',#77392,#62852,#62853);
#53595=AXIS2_PLACEMENT_3D('',#77393,#62854,#62855);
#53596=AXIS2_PLACEMENT_3D('',#77395,#62856,#62857);
#53597=AXIS2_PLACEMENT_3D('',#77396,#62858,#62859);
#53598=AXIS2_PLACEMENT_3D('',#77397,#62860,#62861);
#53599=AXIS2_PLACEMENT_3D('',#77399,#62862,#62863);
#53600=AXIS2_PLACEMENT_3D('',#77400,#62864,#62865);
#53601=AXIS2_PLACEMENT_3D('',#77402,#62866,#62867);
#53602=AXIS2_PLACEMENT_3D('',#77404,#62869,#62870);
#53603=AXIS2_PLACEMENT_3D('',#77406,#62871,#62872);
#53604=AXIS2_PLACEMENT_3D('',#77408,#62874,#62875);
#53605=AXIS2_PLACEMENT_3D('',#77410,#62877,#62878);
#53606=AXIS2_PLACEMENT_3D('',#77412,#62879,#62880);
#53607=AXIS2_PLACEMENT_3D('',#77414,#62882,#62883);
#55370=DIRECTION('axis',(0.,0.,1.));
#55371=DIRECTION('refdir',(1.,0.,0.));
#55372=DIRECTION('center_axis',(1.,0.,0.));
#55373=DIRECTION('ref_axis',(0.,1.,0.));
#55374=DIRECTION('center_axis',(-1.,0.,0.));
#55375=DIRECTION('ref_axis',(0.,1.,0.));
#55376=DIRECTION('center_axis',(1.,0.,0.));
#55377=DIRECTION('ref_axis',(0.,1.,0.));
#55378=DIRECTION('center_axis',(-1.,0.,0.));
#55379=DIRECTION('ref_axis',(0.,1.,0.));
#55380=DIRECTION('center_axis',(1.,0.,0.));
#55381=DIRECTION('ref_axis',(0.,1.,0.));
#55382=DIRECTION('center_axis',(-1.,0.,0.));
#55383=DIRECTION('ref_axis',(0.,1.,0.));
#55384=DIRECTION('center_axis',(1.,0.,0.));
#55385=DIRECTION('ref_axis',(0.,1.,0.));
#55386=DIRECTION('center_axis',(-1.,0.,0.));
#55387=DIRECTION('ref_axis',(0.,1.,0.));
#55388=DIRECTION('center_axis',(1.,0.,0.));
#55389=DIRECTION('ref_axis',(0.,1.,0.));
#55390=DIRECTION('center_axis',(-1.,0.,0.));
#55391=DIRECTION('ref_axis',(0.,1.,0.));
#55392=DIRECTION('center_axis',(1.,0.,0.));
#55393=DIRECTION('ref_axis',(0.,1.,0.));
#55394=DIRECTION('center_axis',(-1.,0.,0.));
#55395=DIRECTION('ref_axis',(0.,1.,0.));
#55396=DIRECTION('center_axis',(1.,0.,0.));
#55397=DIRECTION('ref_axis',(0.,1.,0.));
#55398=DIRECTION('center_axis',(-1.,0.,0.));
#55399=DIRECTION('ref_axis',(0.,1.,0.));
#55400=DIRECTION('center_axis',(1.,0.,0.));
#55401=DIRECTION('ref_axis',(0.,1.,0.));
#55402=DIRECTION('center_axis',(-1.,0.,0.));
#55403=DIRECTION('ref_axis',(0.,1.,0.));
#55404=DIRECTION('center_axis',(1.,0.,0.));
#55405=DIRECTION('ref_axis',(0.,1.,0.));
#55406=DIRECTION('center_axis',(-1.,0.,0.));
#55407=DIRECTION('ref_axis',(0.,1.,0.));
#55408=DIRECTION('center_axis',(1.,0.,0.));
#55409=DIRECTION('ref_axis',(0.,1.,0.));
#55410=DIRECTION('center_axis',(-1.,0.,0.));
#55411=DIRECTION('ref_axis',(0.,1.,0.));
#55412=DIRECTION('center_axis',(1.,0.,0.));
#55413=DIRECTION('ref_axis',(0.,1.,0.));
#55414=DIRECTION('center_axis',(-1.,0.,0.));
#55415=DIRECTION('ref_axis',(0.,1.,0.));
#55416=DIRECTION('center_axis',(1.,0.,0.));
#55417=DIRECTION('ref_axis',(0.,1.,0.));
#55418=DIRECTION('center_axis',(-1.,0.,0.));
#55419=DIRECTION('ref_axis',(0.,1.,0.));
#55420=DIRECTION('center_axis',(1.,0.,0.));
#55421=DIRECTION('ref_axis',(0.,1.,0.));
#55422=DIRECTION('center_axis',(-1.,0.,0.));
#55423=DIRECTION('ref_axis',(0.,1.,0.));
#55424=DIRECTION('center_axis',(1.,0.,0.));
#55425=DIRECTION('ref_axis',(0.,1.,0.));
#55426=DIRECTION('center_axis',(-1.,0.,0.));
#55427=DIRECTION('ref_axis',(0.,1.,0.));
#55428=DIRECTION('center_axis',(1.,0.,0.));
#55429=DIRECTION('ref_axis',(0.,1.,0.));
#55430=DIRECTION('center_axis',(-1.,0.,0.));
#55431=DIRECTION('ref_axis',(0.,1.,0.));
#55432=DIRECTION('center_axis',(1.,0.,0.));
#55433=DIRECTION('ref_axis',(0.,1.,0.));
#55434=DIRECTION('center_axis',(-1.,0.,0.));
#55435=DIRECTION('ref_axis',(0.,1.,0.));
#55436=DIRECTION('center_axis',(1.,0.,0.));
#55437=DIRECTION('ref_axis',(0.,1.,0.));
#55438=DIRECTION('center_axis',(-1.,0.,0.));
#55439=DIRECTION('ref_axis',(0.,1.,0.));
#55440=DIRECTION('center_axis',(1.,0.,0.));
#55441=DIRECTION('ref_axis',(0.,-1.,1.22464679914735E-16));
#55442=DIRECTION('center_axis',(-1.,0.,0.));
#55443=DIRECTION('ref_axis',(0.,1.,0.));
#55444=DIRECTION('center_axis',(1.,0.,0.));
#55445=DIRECTION('ref_axis',(0.,1.,0.));
#55446=DIRECTION('center_axis',(-1.,0.,0.));
#55447=DIRECTION('ref_axis',(0.,1.,0.));
#55448=DIRECTION('center_axis',(1.,0.,0.));
#55449=DIRECTION('ref_axis',(0.,1.,0.));
#55450=DIRECTION('center_axis',(-1.,0.,0.));
#55451=DIRECTION('ref_axis',(0.,1.,0.));
#55452=DIRECTION('center_axis',(1.,0.,0.));
#55453=DIRECTION('ref_axis',(0.,1.,0.));
#55454=DIRECTION('center_axis',(-1.,0.,0.));
#55455=DIRECTION('ref_axis',(0.,1.,0.));
#55456=DIRECTION('center_axis',(1.,0.,0.));
#55457=DIRECTION('ref_axis',(0.,1.,0.));
#55458=DIRECTION('center_axis',(-1.,0.,0.));
#55459=DIRECTION('ref_axis',(0.,1.,0.));
#55460=DIRECTION('center_axis',(1.,0.,0.));
#55461=DIRECTION('ref_axis',(0.,1.,0.));
#55462=DIRECTION('center_axis',(-1.,0.,0.));
#55463=DIRECTION('ref_axis',(0.,1.,0.));
#55464=DIRECTION('center_axis',(1.,0.,0.));
#55465=DIRECTION('ref_axis',(0.,1.,0.));
#55466=DIRECTION('center_axis',(-1.,0.,0.));
#55467=DIRECTION('ref_axis',(0.,1.,0.));
#55468=DIRECTION('center_axis',(1.,0.,0.));
#55469=DIRECTION('ref_axis',(0.,1.,0.));
#55470=DIRECTION('center_axis',(-1.,0.,0.));
#55471=DIRECTION('ref_axis',(0.,1.,0.));
#55472=DIRECTION('center_axis',(1.,0.,0.));
#55473=DIRECTION('ref_axis',(0.,1.,0.));
#55474=DIRECTION('center_axis',(-1.,0.,0.));
#55475=DIRECTION('ref_axis',(0.,1.,0.));
#55476=DIRECTION('center_axis',(1.,0.,0.));
#55477=DIRECTION('ref_axis',(0.,1.,0.));
#55478=DIRECTION('center_axis',(-1.,0.,0.));
#55479=DIRECTION('ref_axis',(0.,1.,0.));
#55480=DIRECTION('center_axis',(1.,0.,0.));
#55481=DIRECTION('ref_axis',(0.,1.,0.));
#55482=DIRECTION('center_axis',(-1.,0.,0.));
#55483=DIRECTION('ref_axis',(0.,1.,0.));
#55484=DIRECTION('center_axis',(1.,0.,0.));
#55485=DIRECTION('ref_axis',(0.,1.,0.));
#55486=DIRECTION('center_axis',(-1.,0.,0.));
#55487=DIRECTION('ref_axis',(0.,1.,0.));
#55488=DIRECTION('center_axis',(1.,0.,0.));
#55489=DIRECTION('ref_axis',(0.,1.,0.));
#55490=DIRECTION('center_axis',(-1.,0.,0.));
#55491=DIRECTION('ref_axis',(0.,1.,0.));
#55492=DIRECTION('center_axis',(1.,0.,0.));
#55493=DIRECTION('ref_axis',(0.,1.,0.));
#55494=DIRECTION('center_axis',(-1.,0.,0.));
#55495=DIRECTION('ref_axis',(0.,1.,0.));
#55496=DIRECTION('center_axis',(1.,0.,0.));
#55497=DIRECTION('ref_axis',(0.,1.,0.));
#55498=DIRECTION('center_axis',(-1.,0.,0.));
#55499=DIRECTION('ref_axis',(0.,1.,0.));
#55500=DIRECTION('center_axis',(1.,0.,0.));
#55501=DIRECTION('ref_axis',(0.,1.,0.));
#55502=DIRECTION('center_axis',(-1.,0.,0.));
#55503=DIRECTION('ref_axis',(0.,1.,0.));
#55504=DIRECTION('center_axis',(1.,0.,0.));
#55505=DIRECTION('ref_axis',(0.,1.,0.));
#55506=DIRECTION('center_axis',(-1.,0.,0.));
#55507=DIRECTION('ref_axis',(0.,1.,0.));
#55508=DIRECTION('center_axis',(1.,0.,0.));
#55509=DIRECTION('ref_axis',(0.,1.,0.));
#55510=DIRECTION('center_axis',(-1.,0.,0.));
#55511=DIRECTION('ref_axis',(0.,1.,0.));
#55512=DIRECTION('center_axis',(1.,0.,0.));
#55513=DIRECTION('ref_axis',(0.,1.,0.));
#55514=DIRECTION('center_axis',(-1.,0.,0.));
#55515=DIRECTION('ref_axis',(0.,1.,0.));
#55516=DIRECTION('center_axis',(0.,1.,0.));
#55517=DIRECTION('ref_axis',(1.,0.,0.));
#55518=DIRECTION('',(0.755033118392644,0.,-0.655686655446243));
#55519=DIRECTION('',(1.,0.,0.));
#55520=DIRECTION('',(0.,0.,1.));
#55521=DIRECTION('',(0.998052578482888,0.,0.0623782861551806));
#55522=DIRECTION('',(0.957826285221151,0.,-0.287347885566345));
#55523=DIRECTION('',(0.86824314212446,0.,-0.496138938356832));
#55524=DIRECTION('',(0.948683298050513,0.,-0.31622776601684));
#55525=DIRECTION('',(1.,0.,0.));
#55526=DIRECTION('',(0.948683298050514,0.,0.316227766016839));
#55527=DIRECTION('',(0.868243142124459,0.,0.496138938356833));
#55528=DIRECTION('',(0.957826285221151,0.,0.287347885566346));
#55529=DIRECTION('',(0.998052578482888,0.,-0.0623782861551805));
#55530=DIRECTION('',(0.,0.,-1.));
#55531=DIRECTION('',(1.,0.,0.));
#55532=DIRECTION('',(0.755033118392644,0.,0.655686655446243));
#55533=DIRECTION('',(-0.755033118392644,0.,0.655686655446243));
#55534=DIRECTION('',(-1.,0.,0.));
#55535=DIRECTION('',(0.,0.,-1.));
#55536=DIRECTION('',(-0.998052578482888,0.,-0.0623782861551805));
#55537=DIRECTION('',(-0.957826285221151,0.,0.287347885566346));
#55538=DIRECTION('',(-0.868243142124459,0.,0.496138938356833));
#55539=DIRECTION('',(-0.948683298050514,0.,0.316227766016839));
#55540=DIRECTION('',(-1.,0.,0.));
#55541=DIRECTION('',(-0.948683298050513,0.,-0.31622776601684));
#55542=DIRECTION('',(-0.86824314212446,0.,-0.496138938356832));
#55543=DIRECTION('',(-0.957826285221151,0.,-0.287347885566345));
#55544=DIRECTION('',(-0.998052578482888,0.,0.0623782861551806));
#55545=DIRECTION('',(0.,0.,1.));
#55546=DIRECTION('',(-1.,0.,0.));
#55547=DIRECTION('',(-0.755033118392644,0.,-0.655686655446243));
#55548=DIRECTION('center_axis',(0.649305557988371,-0.139173100960065,0.747685187986608));
#55549=DIRECTION('ref_axis',(0.755033118392643,0.,-0.655686655446243));
#55550=DIRECTION('',(0.,0.983113759331517,0.182995454077559));
#55551=DIRECTION('',(-0.755033118392644,0.,0.655686655446243));
#55552=DIRECTION('center_axis',(-0.649305557988371,0.139173100960065,-0.747685187986608));
#55553=DIRECTION('ref_axis',(0.760527640763576,0.118819965419165,-0.638341228068795));
#55554=DIRECTION('',(0.0519254248777275,0.98893216263388,0.138985351600607));
#55555=DIRECTION('center_axis',(0.,0.984807753012208,0.17364817766693));
#55556=DIRECTION('ref_axis',(1.,0.,0.));
#55557=DIRECTION('',(0.755033118392643,0.113858792838765,-0.645725301830105));
#55558=DIRECTION('',(1.,0.,0.));
#55559=DIRECTION('',(0.,-0.17364817766693,0.984807753012208));
#55560=DIRECTION('',(0.998052578482888,-0.0108318757168334,0.0614306198252359));
#55561=DIRECTION('',(0.957826285221151,0.0498974366850415,-0.282982425517402));
#55562=DIRECTION('',(0.86824314212446,0.0861536225152694,-0.488601473065054));
#55563=DIRECTION('',(0.948683298050513,0.0549123752965087,-0.311423555691114));
#55564=DIRECTION('',(1.,0.,0.));
#55565=DIRECTION('',(0.948683298050514,-0.0549123752965085,0.311423555691113));
#55566=DIRECTION('',(0.868243142124459,-0.0861536225152696,0.488601473065055));
#55567=DIRECTION('',(0.957826285221151,-0.0498974366850416,0.282982425517402));
#55568=DIRECTION('',(0.998052578482888,0.0108318757168334,-0.0614306198252359));
#55569=DIRECTION('',(0.,0.17364817766693,-0.984807753012208));
#55570=DIRECTION('',(1.,0.,0.));
#55571=DIRECTION('',(0.755033118392644,-0.113858792838765,0.645725301830105));
#55572=DIRECTION('',(-0.755033118392644,-0.113858792838765,0.645725301830105));
#55573=DIRECTION('',(-1.,0.,0.));
#55574=DIRECTION('',(0.,0.17364817766693,-0.984807753012208));
#55575=DIRECTION('',(-0.998052578482888,0.0108318757168334,-0.0614306198252359));
#55576=DIRECTION('',(-0.957826285221151,-0.0498974366850416,0.282982425517402));
#55577=DIRECTION('',(-0.868243142124459,-0.0861536225152696,0.488601473065055));
#55578=DIRECTION('',(-0.948683298050514,-0.0549123752965085,0.311423555691113));
#55579=DIRECTION('',(-1.,0.,0.));
#55580=DIRECTION('',(-0.948683298050513,0.0549123752965087,-0.311423555691114));
#55581=DIRECTION('',(-0.86824314212446,0.0861536225152694,-0.488601473065054));
#55582=DIRECTION('',(-0.957826285221151,0.0498974366850415,-0.282982425517402));
#55583=DIRECTION('',(-0.998052578482888,-0.0108318757168334,0.0614306198252359));
#55584=DIRECTION('',(0.,-0.17364817766693,0.984807753012208));
#55585=DIRECTION('',(-1.,0.,0.));
#55586=DIRECTION('',(-0.755033118392643,0.113858792838765,-0.645725301830105));
#55587=DIRECTION('center_axis',(0.649305557988371,-0.266892919198654,0.712159014579631));
#55588=DIRECTION('ref_axis',(0.755033118392643,0.113858792838765,-0.645725301830105));
#55589=DIRECTION('',(0.,0.936401225160756,0.350931254688773));
#55590=DIRECTION('',(-0.755033118392643,-0.113858792838765,0.645725301830105));
#55591=DIRECTION('center_axis',(-0.649305557988371,0.266892919198654,-0.712159014579631));
#55592=DIRECTION('ref_axis',(0.760527640763576,0.227861614141253,-0.608010520003998));
#55593=DIRECTION('',(0.0519254248777275,0.949773507937132,0.308600119688995));
#55594=DIRECTION('center_axis',(0.,0.939692620785908,0.342020143325669));
#55595=DIRECTION('ref_axis',(1.,0.,0.));
#55596=DIRECTION('',(0.755033118392644,0.224258043872452,-0.616143911670627));
#55597=DIRECTION('',(1.,0.,0.));
#55598=DIRECTION('',(0.,-0.342020143325669,0.939692620785908));
#55599=DIRECTION('',(0.998052578482888,-0.0213346303712044,0.058616415197295));
#55600=DIRECTION('',(0.957826285221151,0.0982787650057293,-0.270018687665128));
#55601=DIRECTION('',(0.86824314212446,0.169689510806249,-0.46621809925847));
#55602=DIRECTION('',(0.948683298050513,0.108156265856636,-0.297156898213637));
#55603=DIRECTION('',(1.,0.,0.));
#55604=DIRECTION('',(0.948683298050514,-0.108156265856635,0.297156898213636));
#55605=DIRECTION('',(0.868243142124459,-0.169689510806249,0.466218099258471));
#55606=DIRECTION('',(0.957826285221151,-0.0982787650057295,0.270018687665129));
#55607=DIRECTION('',(0.998052578482888,0.0213346303712044,-0.0586164151972949));
#55608=DIRECTION('',(0.,0.342020143325669,-0.939692620785908));
#55609=DIRECTION('',(1.,0.,0.));
#55610=DIRECTION('',(0.755033118392644,-0.224258043872452,0.616143911670627));
#55611=DIRECTION('',(-0.755033118392644,-0.224258043872452,0.616143911670627));
#55612=DIRECTION('',(-1.,0.,0.));
#55613=DIRECTION('',(0.,0.342020143325669,-0.939692620785908));
#55614=DIRECTION('',(-0.998052578482888,0.0213346303712044,-0.0586164151972949));
#55615=DIRECTION('',(-0.957826285221151,-0.0982787650057295,0.270018687665129));
#55616=DIRECTION('',(-0.868243142124459,-0.169689510806249,0.466218099258471));
#55617=DIRECTION('',(-0.948683298050514,-0.108156265856635,0.297156898213636));
#55618=DIRECTION('',(-1.,0.,0.));
#55619=DIRECTION('',(-0.948683298050513,0.108156265856636,-0.297156898213637));
#55620=DIRECTION('',(-0.86824314212446,0.169689510806249,-0.46621809925847));
#55621=DIRECTION('',(-0.957826285221151,0.0982787650057293,-0.270018687665128));
#55622=DIRECTION('',(-0.998052578482888,-0.0213346303712044,0.058616415197295));
#55623=DIRECTION('',(0.,-0.342020143325669,0.939692620785908));
#55624=DIRECTION('',(-1.,0.,0.));
#55625=DIRECTION('',(-0.755033118392644,0.224258043872452,-0.616143911670627));
#55626=DIRECTION('center_axis',(0.649305557988371,-0.386503331141725,0.654994249884502));
#55627=DIRECTION('ref_axis',(0.755033118392643,0.224258043872452,-0.616143911670627));
#55628=DIRECTION('',(0.,0.861236613605368,0.508204186706051));
#55629=DIRECTION('',(-0.755033118392644,-0.224258043872452,0.616143911670627));
#55630=DIRECTION('center_axis',(-0.649305557988371,0.386503331141725,-0.654994249884502));
#55631=DIRECTION('ref_axis',(0.760527640763576,0.329979803021199,-0.559205719957048));
#55632=DIRECTION('',(0.0519254248777275,0.881756465810299,0.468838229299828));
#55633=DIRECTION('center_axis',(0.,0.866025403784439,0.5));
#55634=DIRECTION('ref_axis',(1.,0.,0.));
#55635=DIRECTION('',(0.755033118392644,0.327843327723122,-0.567841300538901));
#55636=DIRECTION('',(1.,0.,0.));
#55637=DIRECTION('',(0.,-0.5,0.866025403784439));
#55638=DIRECTION('',(0.998052578482888,-0.0311891430775903,0.0540211804549215));
#55639=DIRECTION('',(0.957826285221151,0.143673942783173,-0.248850568624199));
#55640=DIRECTION('',(0.86824314212446,0.248069469178416,-0.429668924423658));
#55641=DIRECTION('',(0.948683298050513,0.15811388300842,-0.273861278752585));
#55642=DIRECTION('',(1.,0.,0.));
#55643=DIRECTION('',(0.948683298050514,-0.158113883008419,0.273861278752584));
#55644=DIRECTION('',(0.868243142124459,-0.248069469178417,0.429668924423659));
#55645=DIRECTION('',(0.957826285221151,-0.143673942783173,0.248850568624199));
#55646=DIRECTION('',(0.998052578482888,0.0311891430775903,-0.0540211804549215));
#55647=DIRECTION('',(0.,0.5,-0.866025403784439));
#55648=DIRECTION('',(1.,0.,0.));
#55649=DIRECTION('',(0.755033118392644,-0.327843327723121,0.567841300538901));
#55650=DIRECTION('',(-0.755033118392644,-0.327843327723121,0.567841300538901));
#55651=DIRECTION('',(-1.,0.,0.));
#55652=DIRECTION('',(0.,0.5,-0.866025403784439));
#55653=DIRECTION('',(-0.998052578482888,0.0311891430775903,-0.0540211804549215));
#55654=DIRECTION('',(-0.957826285221151,-0.143673942783173,0.248850568624199));
#55655=DIRECTION('',(-0.868243142124459,-0.248069469178417,0.429668924423659));
#55656=DIRECTION('',(-0.948683298050514,-0.158113883008419,0.273861278752584));
#55657=DIRECTION('',(-1.,0.,0.));
#55658=DIRECTION('',(-0.948683298050513,0.15811388300842,-0.273861278752585));
#55659=DIRECTION('',(-0.86824314212446,0.248069469178416,-0.429668924423658));
#55660=DIRECTION('',(-0.957826285221151,0.143673942783173,-0.248850568624199));
#55661=DIRECTION('',(-0.998052578482888,-0.0311891430775903,0.0540211804549215));
#55662=DIRECTION('',(0.,-0.5,0.866025403784439));
#55663=DIRECTION('',(-1.,0.,0.));
#55664=DIRECTION('',(-0.755033118392644,0.327843327723122,-0.567841300538901));
#55665=DIRECTION('center_axis',(0.649305557988371,-0.494370034948177,0.577927816349714));
#55666=DIRECTION('ref_axis',(0.755033118392643,0.327843327723122,-0.567841300538901));
#55667=DIRECTION('',(0.,0.759903763352335,0.650035591673993));
#55668=DIRECTION('',(-0.755033118392644,-0.327843327723122,0.567841300538901));
#55669=DIRECTION('center_axis',(-0.649305557988371,0.494370034948177,-0.577927816349714));
#55670=DIRECTION('ref_axis',(0.760527640763576,0.422071722564183,-0.493409737080951));
#55671=DIRECTION('',(0.0519254248777275,0.786947699660121,0.614830926556978));
#55672=DIRECTION('center_axis',(0.,0.766044443118978,0.642787609686539));
#55673=DIRECTION('ref_axis',(1.,0.,0.));
#55674=DIRECTION('',(0.755033118392644,0.421467257957652,-0.502285118831863));
#55675=DIRECTION('',(1.,0.,0.));
#55676=DIRECTION('',(0.,-0.642787609686539,0.766044443118978));
#55677=DIRECTION('',(0.998052578482888,-0.0400959894540315,0.0477845394804616));
#55678=DIRECTION('',(0.957826285221151,0.184703660511672,-0.220121250980087));
#55679=DIRECTION('',(0.86824314212446,0.318911962258805,-0.3800644767432));
#55680=DIRECTION('',(0.948683298050513,0.203267289834479,-0.242244522917128));
#55681=DIRECTION('',(1.,0.,0.));
#55682=DIRECTION('',(0.948683298050514,-0.203267289834478,0.242244522917128));
#55683=DIRECTION('',(0.868243142124459,-0.318911962258806,0.380064476743201));
#55684=DIRECTION('',(0.957826285221151,-0.184703660511673,0.220121250980087));
#55685=DIRECTION('',(0.998052578482888,0.0400959894540314,-0.0477845394804615));
#55686=DIRECTION('',(0.,0.642787609686539,-0.766044443118978));
#55687=DIRECTION('',(1.,0.,0.));
#55688=DIRECTION('',(0.755033118392644,-0.421467257957652,0.502285118831862));
#55689=DIRECTION('',(-0.755033118392644,-0.421467257957652,0.502285118831862));
#55690=DIRECTION('',(-1.,0.,0.));
#55691=DIRECTION('',(0.,0.642787609686539,-0.766044443118978));
#55692=DIRECTION('',(-0.998052578482888,0.0400959894540314,-0.0477845394804615));
#55693=DIRECTION('',(-0.957826285221151,-0.184703660511673,0.220121250980087));
#55694=DIRECTION('',(-0.868243142124459,-0.318911962258806,0.380064476743201));
#55695=DIRECTION('',(-0.948683298050514,-0.203267289834478,0.242244522917128));
#55696=DIRECTION('',(-1.,0.,0.));
#55697=DIRECTION('',(-0.948683298050513,0.203267289834479,-0.242244522917128));
#55698=DIRECTION('',(-0.86824314212446,0.318911962258805,-0.3800644767432));
#55699=DIRECTION('',(-0.957826285221151,0.184703660511672,-0.220121250980087));
#55700=DIRECTION('',(-0.998052578482888,-0.0400959894540315,0.0477845394804616));
#55701=DIRECTION('',(0.,-0.642787609686539,0.766044443118978));
#55702=DIRECTION('',(-1.,0.,0.));
#55703=DIRECTION('',(-0.755033118392644,0.421467257957652,-0.502285118831863));
#55704=DIRECTION('center_axis',(0.649305557988371,-0.587215555406037,0.483301338560726));
#55705=DIRECTION('ref_axis',(0.755033118392643,0.421467257957652,-0.502285118831863));
#55706=DIRECTION('',(0.,0.6354816217797,0.772115994122802));
#55707=DIRECTION('',(-0.755033118392644,-0.421467257957652,0.502285118831863));
#55708=DIRECTION('center_axis',(-0.649305557988371,0.587215555406037,-0.483301338560726));
#55709=DIRECTION('ref_axis',(0.760527640763576,0.501339206395651,-0.412621749021023));
#55710=DIRECTION('',(0.0519254248777275,0.66822792587052,0.742142297230154));
#55711=DIRECTION('center_axis',(0.,0.642787609686539,0.766044443118978));
#55712=DIRECTION('ref_axis',(1.,0.,0.));
#55713=DIRECTION('',(0.755033118392644,0.502285118831863,-0.421467257957652));
#55714=DIRECTION('',(1.,0.,0.));
#55715=DIRECTION('',(0.,-0.766044443118978,0.642787609686539));
#55716=DIRECTION('',(0.998052578482888,-0.0477845394804615,0.0400959894540315));
#55717=DIRECTION('',(0.957826285221151,0.220121250980087,-0.184703660511672));
#55718=DIRECTION('',(0.86824314212446,0.3800644767432,-0.318911962258805));
#55719=DIRECTION('',(0.948683298050513,0.242244522917128,-0.203267289834479));
#55720=DIRECTION('',(1.,0.,0.));
#55721=DIRECTION('',(0.948683298050513,-0.242244522917128,0.203267289834478));
#55722=DIRECTION('',(0.868243142124459,-0.380064476743201,0.318911962258806));
#55723=DIRECTION('',(0.957826285221151,-0.220121250980087,0.184703660511673));
#55724=DIRECTION('',(0.998052578482888,0.0477845394804615,-0.0400959894540314));
#55725=DIRECTION('',(0.,0.766044443118978,-0.642787609686539));
#55726=DIRECTION('',(1.,0.,0.));
#55727=DIRECTION('',(0.755033118392644,-0.502285118831862,0.421467257957652));
#55728=DIRECTION('',(-0.755033118392644,-0.502285118831862,0.421467257957652));
#55729=DIRECTION('',(-1.,0.,0.));
#55730=DIRECTION('',(0.,0.766044443118978,-0.642787609686539));
#55731=DIRECTION('',(-0.998052578482888,0.0477845394804615,-0.0400959894540314));
#55732=DIRECTION('',(-0.957826285221151,-0.220121250980087,0.184703660511673));
#55733=DIRECTION('',(-0.868243142124459,-0.380064476743201,0.318911962258806));
#55734=DIRECTION('',(-0.948683298050513,-0.242244522917128,0.203267289834478));
#55735=DIRECTION('',(-1.,0.,0.));
#55736=DIRECTION('',(-0.948683298050513,0.242244522917128,-0.203267289834479));
#55737=DIRECTION('',(-0.86824314212446,0.3800644767432,-0.318911962258805));
#55738=DIRECTION('',(-0.957826285221151,0.220121250980087,-0.184703660511672));
#55739=DIRECTION('',(-0.998052578482888,-0.0477845394804615,0.0400959894540315));
#55740=DIRECTION('',(0.,-0.766044443118978,0.642787609686539));
#55741=DIRECTION('',(-1.,0.,0.));
#55742=DIRECTION('',(-0.755033118392644,0.502285118831863,-0.421467257957652));
#55743=DIRECTION('center_axis',(0.649305557988371,-0.662218828358294,0.373989994161848));
#55744=DIRECTION('ref_axis',(0.755033118392643,0.502285118831863,-0.421467257957652));
#55745=DIRECTION('',(0.,0.491750692698505,0.870736042799734));
#55746=DIRECTION('',(-0.755033118392644,-0.502285118831863,0.421467257957652));
#55747=DIRECTION('center_axis',(-0.649305557988371,0.662218828358294,-0.373989994161848));
#55748=DIRECTION('ref_axis',(0.760527640763576,0.565373752130667,-0.319296457913771));
#55749=DIRECTION('',(0.0519254248777275,0.52920438469299,0.846904049744115));
#55750=DIRECTION('center_axis',(0.,0.5,0.866025403784439));
#55751=DIRECTION('ref_axis',(1.,0.,0.));
#55752=DIRECTION('',(0.755033118392644,0.567841300538901,-0.327843327723122));
#55753=DIRECTION('',(1.,0.,0.));
#55754=DIRECTION('',(0.,-0.866025403784439,0.5));
#55755=DIRECTION('',(0.998052578482888,-0.0540211804549215,0.0311891430775903));
#55756=DIRECTION('',(0.957826285221151,0.248850568624199,-0.143673942783173));
#55757=DIRECTION('',(0.86824314212446,0.429668924423658,-0.248069469178416));
#55758=DIRECTION('',(0.948683298050513,0.273861278752585,-0.15811388300842));
#55759=DIRECTION('',(1.,0.,0.));
#55760=DIRECTION('',(0.948683298050514,-0.273861278752584,0.158113883008419));
#55761=DIRECTION('',(0.868243142124459,-0.429668924423659,0.248069469178417));
#55762=DIRECTION('',(0.957826285221151,-0.248850568624199,0.143673942783173));
#55763=DIRECTION('',(0.998052578482888,0.0540211804549215,-0.0311891430775903));
#55764=DIRECTION('',(0.,0.866025403784439,-0.5));
#55765=DIRECTION('',(1.,0.,0.));
#55766=DIRECTION('',(0.755033118392644,-0.567841300538901,0.327843327723122));
#55767=DIRECTION('',(-0.755033118392644,-0.567841300538901,0.327843327723122));
#55768=DIRECTION('',(-1.,0.,0.));
#55769=DIRECTION('',(0.,0.866025403784439,-0.5));
#55770=DIRECTION('',(-0.998052578482888,0.0540211804549215,-0.0311891430775903));
#55771=DIRECTION('',(-0.957826285221151,-0.248850568624199,0.143673942783173));
#55772=DIRECTION('',(-0.868243142124459,-0.429668924423659,0.248069469178417));
#55773=DIRECTION('',(-0.948683298050514,-0.273861278752584,0.158113883008419));
#55774=DIRECTION('',(-1.,0.,0.));
#55775=DIRECTION('',(-0.948683298050513,0.273861278752585,-0.15811388300842));
#55776=DIRECTION('',(-0.86824314212446,0.429668924423658,-0.248069469178416));
#55777=DIRECTION('',(-0.957826285221151,0.248850568624199,-0.143673942783173));
#55778=DIRECTION('',(-0.998052578482888,-0.0540211804549215,0.0311891430775903));
#55779=DIRECTION('',(0.,-0.866025403784439,0.5));
#55780=DIRECTION('',(-1.,0.,0.));
#55781=DIRECTION('',(-0.755033118392644,0.567841300538901,-0.327843327723122));
#55782=DIRECTION('center_axis',(0.649305557988371,-0.717100917309779,0.253315153038431));
#55783=DIRECTION('ref_axis',(0.755033118392643,0.567841300538901,-0.327843327723122));
#55784=DIRECTION('',(0.,0.333078167657524,0.942899217429894));
#55785=DIRECTION('',(-0.755033118392644,-0.567841300538901,0.327843327723122));
#55786=DIRECTION('center_axis',(-0.649305557988371,0.717100917309779,-0.253315153038431));
#55787=DIRECTION('ref_axis',(0.760527640763576,0.612229702500115,-0.216269505504613));
#55788=DIRECTION('',(0.0519254248777275,0.374101236076903,0.925933051260728));
#55789=DIRECTION('center_axis',(0.,0.342020143325669,0.939692620785908));
#55790=DIRECTION('ref_axis',(1.,0.,0.));
#55791=DIRECTION('',(0.755033118392644,0.616143911670627,-0.224258043872453));
#55792=DIRECTION('',(1.,0.,0.));
#55793=DIRECTION('',(0.,-0.939692620785908,0.342020143325669));
#55794=DIRECTION('',(0.998052578482888,-0.058616415197295,0.0213346303712044));
#55795=DIRECTION('',(0.957826285221151,0.270018687665128,-0.0982787650057293));
#55796=DIRECTION('',(0.86824314212446,0.46621809925847,-0.169689510806249));
#55797=DIRECTION('',(0.948683298050513,0.297156898213637,-0.108156265856636));
#55798=DIRECTION('',(1.,0.,0.));
#55799=DIRECTION('',(0.948683298050514,-0.297156898213636,0.108156265856635));
#55800=DIRECTION('',(0.868243142124459,-0.466218099258471,0.169689510806249));
#55801=DIRECTION('',(0.957826285221151,-0.270018687665129,0.0982787650057295));
#55802=DIRECTION('',(0.998052578482888,0.0586164151972949,-0.0213346303712044));
#55803=DIRECTION('',(0.,0.939692620785908,-0.342020143325669));
#55804=DIRECTION('',(1.,0.,0.));
#55805=DIRECTION('',(0.755033118392644,-0.616143911670627,0.224258043872453));
#55806=DIRECTION('',(-0.755033118392644,-0.616143911670627,0.224258043872453));
#55807=DIRECTION('',(-1.,0.,0.));
#55808=DIRECTION('',(0.,0.939692620785908,-0.342020143325669));
#55809=DIRECTION('',(-0.998052578482888,0.0586164151972949,-0.0213346303712044));
#55810=DIRECTION('',(-0.957826285221151,-0.270018687665129,0.0982787650057295));
#55811=DIRECTION('',(-0.868243142124459,-0.466218099258471,0.169689510806249));
#55812=DIRECTION('',(-0.948683298050514,-0.297156898213636,0.108156265856635));
#55813=DIRECTION('',(-1.,0.,0.));
#55814=DIRECTION('',(-0.948683298050513,0.297156898213637,-0.108156265856636));
#55815=DIRECTION('',(-0.86824314212446,0.46621809925847,-0.169689510806249));
#55816=DIRECTION('',(-0.957826285221151,0.270018687665128,-0.0982787650057293));
#55817=DIRECTION('',(-0.998052578482888,-0.058616415197295,0.0213346303712044));
#55818=DIRECTION('',(0.,-0.939692620785908,0.342020143325669));
#55819=DIRECTION('',(-1.,0.,0.));
#55820=DIRECTION('',(-0.755033118392644,0.616143911670627,-0.224258043872453));
#55821=DIRECTION('center_axis',(0.649305557988371,-0.75019425775938,0.124943459173594));
#55822=DIRECTION('ref_axis',(0.755033118392643,0.616143911670627,-0.224258043872453));
#55823=DIRECTION('',(0.,0.164285231037954,0.986412876468473));
#55824=DIRECTION('',(-0.755033118392644,-0.616143911670627,0.224258043872453));
#55825=DIRECTION('center_axis',(-0.649305557988371,0.75019425775938,-0.124943459173594));
#55826=DIRECTION('ref_axis',(0.760527640763576,0.640483363162275,-0.106671313608347));
#55827=DIRECTION('',(0.0519254248777275,0.207631210706978,0.976828045559515));
#55828=DIRECTION('center_axis',(0.,0.17364817766693,0.984807753012208));
#55829=DIRECTION('ref_axis',(1.,0.,0.));
#55830=DIRECTION('',(0.755033118392643,0.645725301830105,-0.113858792838765));
#55831=DIRECTION('',(1.,0.,0.));
#55832=DIRECTION('',(0.,-0.984807753012208,0.17364817766693));
#55833=DIRECTION('',(0.998052578482888,-0.0614306198252359,0.0108318757168334));
#55834=DIRECTION('',(0.957826285221151,0.282982425517402,-0.0498974366850415));
#55835=DIRECTION('',(0.86824314212446,0.488601473065054,-0.0861536225152694));
#55836=DIRECTION('',(0.948683298050513,0.311423555691114,-0.0549123752965087));
#55837=DIRECTION('',(1.,0.,0.));
#55838=DIRECTION('',(0.948683298050514,-0.311423555691113,0.0549123752965085));
#55839=DIRECTION('',(0.868243142124459,-0.488601473065055,0.0861536225152696));
#55840=DIRECTION('',(0.957826285221151,-0.282982425517402,0.0498974366850416));
#55841=DIRECTION('',(0.998052578482888,0.0614306198252359,-0.0108318757168334));
#55842=DIRECTION('',(0.,0.984807753012208,-0.17364817766693));
#55843=DIRECTION('',(1.,0.,0.));
#55844=DIRECTION('',(0.755033118392644,-0.645725301830105,0.113858792838765));
#55845=DIRECTION('',(-0.755033118392644,-0.645725301830105,0.113858792838765));
#55846=DIRECTION('',(-1.,0.,0.));
#55847=DIRECTION('',(0.,0.984807753012208,-0.17364817766693));
#55848=DIRECTION('',(-0.998052578482888,0.0614306198252359,-0.0108318757168334));
#55849=DIRECTION('',(-0.957826285221151,-0.282982425517402,0.0498974366850416));
#55850=DIRECTION('',(-0.868243142124459,-0.488601473065055,0.0861536225152696));
#55851=DIRECTION('',(-0.948683298050514,-0.311423555691113,0.0549123752965085));
#55852=DIRECTION('',(-1.,0.,0.));
#55853=DIRECTION('',(-0.948683298050513,0.311423555691114,-0.0549123752965087));
#55854=DIRECTION('',(-0.86824314212446,0.488601473065054,-0.0861536225152694));
#55855=DIRECTION('',(-0.957826285221151,0.282982425517402,-0.0498974366850415));
#55856=DIRECTION('',(-0.998052578482888,-0.0614306198252359,0.0108318757168334));
#55857=DIRECTION('',(0.,-0.984807753012208,0.17364817766693));
#55858=DIRECTION('',(-1.,0.,0.));
#55859=DIRECTION('',(-0.755033118392643,0.645725301830105,-0.113858792838765));
#55860=DIRECTION('center_axis',(0.649305557988371,-0.760493325303573,-0.00722457847379221));
#55861=DIRECTION('ref_axis',(0.755033118392643,0.645725301830105,-0.113858792838765));
#55862=DIRECTION('',(0.,-0.00949942919436652,0.999954879404557));
#55863=DIRECTION('',(-0.755033118392643,-0.645725301830105,0.113858792838765));
#55864=DIRECTION('center_axis',(-0.649305557988371,0.760493325303573,0.00722457847379221));
#55865=DIRECTION('ref_axis',(0.760527640763576,0.64927626093497,0.00616803217361917));
#55866=DIRECTION('',(0.0519254248777275,0.0348524160661845,0.998042613992818));
#55867=DIRECTION('center_axis',(0.,6.12323399573677E-17,1.));
#55868=DIRECTION('ref_axis',(1.,0.,0.));
#55869=DIRECTION('',(0.755033118392644,0.655686655446243,-4.01492281917938E-17));
#55870=DIRECTION('',(1.,0.,0.));
#55871=DIRECTION('',(0.,-1.,6.12323399573677E-17));
#55872=DIRECTION('',(0.998052578482888,-0.0623782861551806,3.81956842381198E-18));
#55873=DIRECTION('',(0.957826285221151,0.287347885566345,-1.75949834150292E-17));
#55874=DIRECTION('',(0.86824314212446,0.496138938356832,-3.0379748139553E-17));
#55875=DIRECTION('',(0.948683298050513,0.31622776601684,-1.9363366072702E-17));
#55876=DIRECTION('',(1.,0.,0.));
#55877=DIRECTION('',(0.948683298050514,-0.316227766016839,1.9363366072702E-17));
#55878=DIRECTION('',(0.868243142124459,-0.496138938356833,3.03797481395531E-17));
#55879=DIRECTION('',(0.957826285221151,-0.287347885566346,1.75949834150293E-17));
#55880=DIRECTION('',(0.998052578482888,0.0623782861551805,-3.81956842381197E-18));
#55881=DIRECTION('',(0.,1.,-6.12323399573677E-17));
#55882=DIRECTION('',(1.,0.,0.));
#55883=DIRECTION('',(0.755033118392644,-0.655686655446243,4.01492281917938E-17));
#55884=DIRECTION('',(-0.755033118392644,-0.655686655446243,4.01492281917938E-17));
#55885=DIRECTION('',(-1.,0.,0.));
#55886=DIRECTION('',(0.,1.,-6.12323399573677E-17));
#55887=DIRECTION('',(-0.998052578482888,0.0623782861551805,-3.81956842381197E-18));
#55888=DIRECTION('',(-0.957826285221151,-0.287347885566346,1.75949834150293E-17));
#55889=DIRECTION('',(-0.868243142124459,-0.496138938356833,3.03797481395531E-17));
#55890=DIRECTION('',(-0.948683298050514,-0.316227766016839,1.9363366072702E-17));
#55891=DIRECTION('',(-1.,0.,0.));
#55892=DIRECTION('',(-0.948683298050513,0.31622776601684,-1.9363366072702E-17));
#55893=DIRECTION('',(-0.86824314212446,0.496138938356832,-3.0379748139553E-17));
#55894=DIRECTION('',(-0.957826285221151,0.287347885566345,-1.75949834150292E-17));
#55895=DIRECTION('',(-0.998052578482888,-0.0623782861551806,3.81956842381198E-18));
#55896=DIRECTION('',(0.,-1.,6.12323399573677E-17));
#55897=DIRECTION('',(-1.,0.,0.));
#55898=DIRECTION('',(-0.755033118392644,0.655686655446243,-4.01492281917938E-17));
#55899=DIRECTION('center_axis',(0.649305557988371,-0.747685187986608,-0.139173100960065));
#55900=DIRECTION('ref_axis',(0.755033118392643,0.655686655446243,-4.01492281917938E-17));
#55901=DIRECTION('',(0.,-0.182995454077559,0.983113759331517));
#55902=DIRECTION('',(-0.755033118392644,-0.655686655446243,4.01492281917938E-17));
#55903=DIRECTION('center_axis',(-0.649305557988371,0.747685187986608,0.139173100960065));
#55904=DIRECTION('ref_axis',(0.760527640763576,0.638341228068795,0.118819965419165));
#55905=DIRECTION('',(0.0519254248777275,-0.138985351600607,0.98893216263388));
#55906=DIRECTION('center_axis',(0.,-0.17364817766693,0.984807753012208));
#55907=DIRECTION('ref_axis',(1.,0.,0.));
#55908=DIRECTION('',(0.755033118392643,0.645725301830105,0.113858792838765));
#55909=DIRECTION('',(1.,0.,0.));
#55910=DIRECTION('',(0.,-0.984807753012208,-0.17364817766693));
#55911=DIRECTION('',(0.998052578482888,-0.0614306198252359,-0.0108318757168334));
#55912=DIRECTION('',(0.957826285221151,0.282982425517402,0.0498974366850415));
#55913=DIRECTION('',(0.86824314212446,0.488601473065054,0.0861536225152694));
#55914=DIRECTION('',(0.948683298050513,0.311423555691114,0.0549123752965087));
#55915=DIRECTION('',(1.,0.,0.));
#55916=DIRECTION('',(0.948683298050514,-0.311423555691113,-0.0549123752965085));
#55917=DIRECTION('',(0.868243142124459,-0.488601473065055,-0.0861536225152696));
#55918=DIRECTION('',(0.957826285221151,-0.282982425517402,-0.0498974366850416));
#55919=DIRECTION('',(0.998052578482888,0.0614306198252359,0.0108318757168334));
#55920=DIRECTION('',(0.,0.984807753012208,0.17364817766693));
#55921=DIRECTION('',(1.,0.,0.));
#55922=DIRECTION('',(0.755033118392644,-0.645725301830105,-0.113858792838765));
#55923=DIRECTION('',(-0.755033118392644,-0.645725301830105,-0.113858792838765));
#55924=DIRECTION('',(-1.,0.,0.));
#55925=DIRECTION('',(0.,0.984807753012208,0.17364817766693));
#55926=DIRECTION('',(-0.998052578482888,0.0614306198252359,0.0108318757168334));
#55927=DIRECTION('',(-0.957826285221151,-0.282982425517402,-0.0498974366850416));
#55928=DIRECTION('',(-0.868243142124459,-0.488601473065055,-0.0861536225152696));
#55929=DIRECTION('',(-0.948683298050514,-0.311423555691113,-0.0549123752965085));
#55930=DIRECTION('',(-1.,0.,0.));
#55931=DIRECTION('',(-0.948683298050513,0.311423555691114,0.0549123752965087));
#55932=DIRECTION('',(-0.86824314212446,0.488601473065054,0.0861536225152694));
#55933=DIRECTION('',(-0.957826285221151,0.282982425517402,0.0498974366850415));
#55934=DIRECTION('',(-0.998052578482888,-0.0614306198252359,-0.0108318757168334));
#55935=DIRECTION('',(0.,-0.984807753012208,-0.17364817766693));
#55936=DIRECTION('',(-1.,0.,0.));
#55937=DIRECTION('',(-0.755033118392643,0.645725301830105,0.113858792838765));
#55938=DIRECTION('center_axis',(0.649305557988371,-0.712159014579631,-0.266892919198654));
#55939=DIRECTION('ref_axis',(0.755033118392643,0.645725301830105,0.113858792838765));
#55940=DIRECTION('',(0.,-0.350931254688773,0.936401225160756));
#55941=DIRECTION('',(-0.755033118392643,-0.645725301830105,-0.113858792838765));
#55942=DIRECTION('center_axis',(-0.649305557988371,0.712159014579631,0.266892919198654));
#55943=DIRECTION('ref_axis',(0.760527640763576,0.608010520003998,0.227861614141253));
#55944=DIRECTION('',(0.0519254248777275,-0.308600119688995,0.949773507937132));
#55945=DIRECTION('center_axis',(0.,-0.342020143325669,0.939692620785908));
#55946=DIRECTION('ref_axis',(1.,0.,0.));
#55947=DIRECTION('',(0.755033118392644,0.616143911670627,0.224258043872452));
#55948=DIRECTION('',(1.,0.,0.));
#55949=DIRECTION('',(0.,-0.939692620785908,-0.342020143325669));
#55950=DIRECTION('',(0.998052578482888,-0.058616415197295,-0.0213346303712044));
#55951=DIRECTION('',(0.957826285221151,0.270018687665128,0.0982787650057293));
#55952=DIRECTION('',(0.86824314212446,0.46621809925847,0.169689510806249));
#55953=DIRECTION('',(0.948683298050513,0.297156898213637,0.108156265856636));
#55954=DIRECTION('',(1.,0.,0.));
#55955=DIRECTION('',(0.948683298050514,-0.297156898213636,-0.108156265856635));
#55956=DIRECTION('',(0.868243142124459,-0.466218099258471,-0.169689510806249));
#55957=DIRECTION('',(0.957826285221151,-0.270018687665129,-0.0982787650057295));
#55958=DIRECTION('',(0.998052578482888,0.0586164151972949,0.0213346303712044));
#55959=DIRECTION('',(0.,0.939692620785908,0.342020143325669));
#55960=DIRECTION('',(1.,0.,0.));
#55961=DIRECTION('',(0.755033118392644,-0.616143911670627,-0.224258043872452));
#55962=DIRECTION('',(-0.755033118392644,-0.616143911670627,-0.224258043872452));
#55963=DIRECTION('',(-1.,0.,0.));
#55964=DIRECTION('',(0.,0.939692620785908,0.342020143325669));
#55965=DIRECTION('',(-0.998052578482888,0.0586164151972949,0.0213346303712044));
#55966=DIRECTION('',(-0.957826285221151,-0.270018687665129,-0.0982787650057295));
#55967=DIRECTION('',(-0.868243142124459,-0.466218099258471,-0.169689510806249));
#55968=DIRECTION('',(-0.948683298050514,-0.297156898213636,-0.108156265856635));
#55969=DIRECTION('',(-1.,0.,0.));
#55970=DIRECTION('',(-0.948683298050513,0.297156898213637,0.108156265856636));
#55971=DIRECTION('',(-0.86824314212446,0.46621809925847,0.169689510806249));
#55972=DIRECTION('',(-0.957826285221151,0.270018687665128,0.0982787650057293));
#55973=DIRECTION('',(-0.998052578482888,-0.058616415197295,-0.0213346303712044));
#55974=DIRECTION('',(0.,-0.939692620785908,-0.342020143325669));
#55975=DIRECTION('',(-1.,0.,0.));
#55976=DIRECTION('',(-0.755033118392644,0.616143911670627,0.224258043872452));
#55977=DIRECTION('center_axis',(0.649305557988371,-0.654994249884502,-0.386503331141725));
#55978=DIRECTION('ref_axis',(0.755033118392643,0.616143911670627,0.224258043872452));
#55979=DIRECTION('',(0.,-0.508204186706051,0.861236613605368));
#55980=DIRECTION('',(-0.755033118392644,-0.616143911670627,-0.224258043872452));
#55981=DIRECTION('center_axis',(-0.649305557988371,0.654994249884502,0.386503331141725));
#55982=DIRECTION('ref_axis',(0.760527640763576,0.559205719957048,0.329979803021199));
#55983=DIRECTION('',(0.0519254248777275,-0.468838229299828,0.881756465810299));
#55984=DIRECTION('center_axis',(0.,-0.5,0.866025403784439));
#55985=DIRECTION('ref_axis',(1.,0.,0.));
#55986=DIRECTION('',(0.755033118392644,0.567841300538901,0.327843327723121));
#55987=DIRECTION('',(1.,0.,0.));
#55988=DIRECTION('',(0.,-0.866025403784439,-0.5));
#55989=DIRECTION('',(0.998052578482888,-0.0540211804549215,-0.0311891430775903));
#55990=DIRECTION('',(0.957826285221151,0.248850568624199,0.143673942783173));
#55991=DIRECTION('',(0.86824314212446,0.429668924423658,0.248069469178416));
#55992=DIRECTION('',(0.948683298050513,0.273861278752585,0.15811388300842));
#55993=DIRECTION('',(1.,0.,0.));
#55994=DIRECTION('',(0.948683298050513,-0.273861278752584,-0.158113883008419));
#55995=DIRECTION('',(0.868243142124459,-0.429668924423659,-0.248069469178417));
#55996=DIRECTION('',(0.957826285221151,-0.248850568624199,-0.143673942783173));
#55997=DIRECTION('',(0.998052578482888,0.0540211804549215,0.0311891430775902));
#55998=DIRECTION('',(0.,0.866025403784439,0.5));
#55999=DIRECTION('',(1.,0.,0.));
#56000=DIRECTION('',(0.755033118392644,-0.567841300538901,-0.327843327723121));
#56001=DIRECTION('',(-0.755033118392644,-0.567841300538901,-0.327843327723121));
#56002=DIRECTION('',(-1.,0.,0.));
#56003=DIRECTION('',(0.,0.866025403784439,0.5));
#56004=DIRECTION('',(-0.998052578482888,0.0540211804549215,0.0311891430775902));
#56005=DIRECTION('',(-0.957826285221151,-0.248850568624199,-0.143673942783173));
#56006=DIRECTION('',(-0.868243142124459,-0.429668924423659,-0.248069469178417));
#56007=DIRECTION('',(-0.948683298050513,-0.273861278752584,-0.158113883008419));
#56008=DIRECTION('',(-1.,0.,0.));
#56009=DIRECTION('',(-0.948683298050513,0.273861278752585,0.15811388300842));
#56010=DIRECTION('',(-0.86824314212446,0.429668924423658,0.248069469178416));
#56011=DIRECTION('',(-0.957826285221151,0.248850568624199,0.143673942783173));
#56012=DIRECTION('',(-0.998052578482888,-0.0540211804549215,-0.0311891430775903));
#56013=DIRECTION('',(0.,-0.866025403784439,-0.5));
#56014=DIRECTION('',(-1.,0.,0.));
#56015=DIRECTION('',(-0.755033118392644,0.567841300538901,0.327843327723121));
#56016=DIRECTION('center_axis',(0.649305557988371,-0.577927816349714,-0.494370034948177));
#56017=DIRECTION('ref_axis',(0.755033118392643,0.567841300538901,0.327843327723121));
#56018=DIRECTION('',(0.,-0.650035591673993,0.759903763352335));
#56019=DIRECTION('',(-0.755033118392644,-0.567841300538901,-0.327843327723121));
#56020=DIRECTION('center_axis',(-0.649305557988371,0.577927816349714,0.494370034948177));
#56021=DIRECTION('ref_axis',(0.760527640763576,0.493409737080951,0.422071722564183));
#56022=DIRECTION('',(0.0519254248777275,-0.614830926556978,0.786947699660121));
#56023=DIRECTION('center_axis',(0.,-0.642787609686539,0.766044443118978));
#56024=DIRECTION('ref_axis',(1.,0.,0.));
#56025=DIRECTION('',(0.755033118392644,0.502285118831863,0.421467257957652));
#56026=DIRECTION('',(1.,0.,0.));
#56027=DIRECTION('',(0.,-0.766044443118978,-0.642787609686539));
#56028=DIRECTION('',(0.998052578482888,-0.0477845394804615,-0.0400959894540315));
#56029=DIRECTION('',(0.957826285221151,0.220121250980087,0.184703660511672));
#56030=DIRECTION('',(0.86824314212446,0.3800644767432,0.318911962258805));
#56031=DIRECTION('',(0.948683298050513,0.242244522917128,0.203267289834479));
#56032=DIRECTION('',(1.,0.,0.));
#56033=DIRECTION('',(0.948683298050513,-0.242244522917128,-0.203267289834478));
#56034=DIRECTION('',(0.868243142124459,-0.380064476743201,-0.318911962258806));
#56035=DIRECTION('',(0.957826285221151,-0.220121250980087,-0.184703660511673));
#56036=DIRECTION('',(0.998052578482888,0.0477845394804615,0.0400959894540314));
#56037=DIRECTION('',(0.,0.766044443118978,0.642787609686539));
#56038=DIRECTION('',(1.,0.,0.));
#56039=DIRECTION('',(0.755033118392644,-0.502285118831862,-0.421467257957652));
#56040=DIRECTION('',(-0.755033118392644,-0.502285118831862,-0.421467257957652));
#56041=DIRECTION('',(-1.,0.,0.));
#56042=DIRECTION('',(0.,0.766044443118978,0.642787609686539));
#56043=DIRECTION('',(-0.998052578482888,0.0477845394804615,0.0400959894540314));
#56044=DIRECTION('',(-0.957826285221151,-0.220121250980087,-0.184703660511673));
#56045=DIRECTION('',(-0.868243142124459,-0.380064476743201,-0.318911962258806));
#56046=DIRECTION('',(-0.948683298050513,-0.242244522917128,-0.203267289834478));
#56047=DIRECTION('',(-1.,0.,0.));
#56048=DIRECTION('',(-0.948683298050513,0.242244522917128,0.203267289834479));
#56049=DIRECTION('',(-0.86824314212446,0.3800644767432,0.318911962258805));
#56050=DIRECTION('',(-0.957826285221151,0.220121250980087,0.184703660511672));
#56051=DIRECTION('',(-0.998052578482888,-0.0477845394804615,-0.0400959894540315));
#56052=DIRECTION('',(0.,-0.766044443118978,-0.642787609686539));
#56053=DIRECTION('',(-1.,0.,0.));
#56054=DIRECTION('',(-0.755033118392644,0.502285118831863,0.421467257957652));
#56055=DIRECTION('center_axis',(0.649305557988371,-0.483301338560726,-0.587215555406037));
#56056=DIRECTION('ref_axis',(0.755033118392643,0.502285118831863,0.421467257957652));
#56057=DIRECTION('',(0.,-0.772115994122802,0.6354816217797));
#56058=DIRECTION('',(-0.755033118392644,-0.502285118831863,-0.421467257957652));
#56059=DIRECTION('center_axis',(-0.649305557988371,0.483301338560726,0.587215555406037));
#56060=DIRECTION('ref_axis',(0.760527640763576,0.412621749021023,0.501339206395652));
#56061=DIRECTION('',(0.0519254248777275,-0.742142297230154,0.66822792587052));
#56062=DIRECTION('center_axis',(0.,-0.766044443118978,0.642787609686539));
#56063=DIRECTION('ref_axis',(1.,0.,0.));
#56064=DIRECTION('',(0.755033118392644,0.421467257957652,0.502285118831862));
#56065=DIRECTION('',(1.,0.,0.));
#56066=DIRECTION('',(0.,-0.642787609686539,-0.766044443118978));
#56067=DIRECTION('',(0.998052578482888,-0.0400959894540315,-0.0477845394804615));
#56068=DIRECTION('',(0.957826285221151,0.184703660511672,0.220121250980087));
#56069=DIRECTION('',(0.86824314212446,0.318911962258805,0.3800644767432));
#56070=DIRECTION('',(0.948683298050513,0.203267289834479,0.242244522917128));
#56071=DIRECTION('',(1.,0.,0.));
#56072=DIRECTION('',(0.948683298050514,-0.203267289834478,-0.242244522917128));
#56073=DIRECTION('',(0.868243142124459,-0.318911962258806,-0.380064476743201));
#56074=DIRECTION('',(0.957826285221151,-0.184703660511673,-0.220121250980087));
#56075=DIRECTION('',(0.998052578482888,0.0400959894540314,0.0477845394804615));
#56076=DIRECTION('',(0.,0.642787609686539,0.766044443118978));
#56077=DIRECTION('',(1.,0.,0.));
#56078=DIRECTION('',(0.755033118392644,-0.421467257957652,-0.502285118831862));
#56079=DIRECTION('',(-0.755033118392644,-0.421467257957652,-0.502285118831862));
#56080=DIRECTION('',(-1.,0.,0.));
#56081=DIRECTION('',(0.,0.642787609686539,0.766044443118978));
#56082=DIRECTION('',(-0.998052578482888,0.0400959894540314,0.0477845394804615));
#56083=DIRECTION('',(-0.957826285221151,-0.184703660511673,-0.220121250980087));
#56084=DIRECTION('',(-0.868243142124459,-0.318911962258806,-0.380064476743201));
#56085=DIRECTION('',(-0.948683298050514,-0.203267289834478,-0.242244522917128));
#56086=DIRECTION('',(-1.,0.,0.));
#56087=DIRECTION('',(-0.948683298050513,0.203267289834479,0.242244522917128));
#56088=DIRECTION('',(-0.86824314212446,0.318911962258805,0.3800644767432));
#56089=DIRECTION('',(-0.957826285221151,0.184703660511672,0.220121250980087));
#56090=DIRECTION('',(-0.998052578482888,-0.0400959894540315,-0.0477845394804615));
#56091=DIRECTION('',(0.,-0.642787609686539,-0.766044443118978));
#56092=DIRECTION('',(-1.,0.,0.));
#56093=DIRECTION('',(-0.755033118392644,0.421467257957652,0.502285118831862));
#56094=DIRECTION('center_axis',(0.649305557988371,-0.373989994161848,-0.662218828358294));
#56095=DIRECTION('ref_axis',(0.755033118392644,0.421467257957652,0.502285118831862));
#56096=DIRECTION('',(0.,-0.870736042799734,0.491750692698505));
#56097=DIRECTION('',(-0.755033118392644,-0.421467257957652,-0.502285118831862));
#56098=DIRECTION('center_axis',(-0.649305557988371,0.373989994161848,0.662218828358294));
#56099=DIRECTION('ref_axis',(0.760527640763576,0.319296457913771,0.565373752130667));
#56100=DIRECTION('',(0.0519254248777275,-0.846904049744115,0.52920438469299));
#56101=DIRECTION('center_axis',(0.,-0.866025403784439,0.5));
#56102=DIRECTION('ref_axis',(1.,0.,0.));
#56103=DIRECTION('',(0.755033118392644,0.327843327723122,0.567841300538901));
#56104=DIRECTION('',(1.,0.,0.));
#56105=DIRECTION('',(0.,-0.5,-0.866025403784439));
#56106=DIRECTION('',(0.998052578482888,-0.0311891430775903,-0.0540211804549215));
#56107=DIRECTION('',(0.957826285221151,0.143673942783173,0.248850568624199));
#56108=DIRECTION('',(0.86824314212446,0.248069469178416,0.429668924423658));
#56109=DIRECTION('',(0.948683298050513,0.15811388300842,0.273861278752585));
#56110=DIRECTION('',(1.,0.,0.));
#56111=DIRECTION('',(0.948683298050514,-0.158113883008419,-0.273861278752584));
#56112=DIRECTION('',(0.868243142124459,-0.248069469178417,-0.429668924423659));
#56113=DIRECTION('',(0.957826285221151,-0.143673942783173,-0.248850568624199));
#56114=DIRECTION('',(0.998052578482888,0.0311891430775903,0.0540211804549215));
#56115=DIRECTION('',(0.,0.5,0.866025403784439));
#56116=DIRECTION('',(1.,0.,0.));
#56117=DIRECTION('',(0.755033118392644,-0.327843327723121,-0.567841300538901));
#56118=DIRECTION('',(-0.755033118392644,-0.327843327723121,-0.567841300538901));
#56119=DIRECTION('',(-1.,0.,0.));
#56120=DIRECTION('',(0.,0.5,0.866025403784439));
#56121=DIRECTION('',(-0.998052578482888,0.0311891430775903,0.0540211804549215));
#56122=DIRECTION('',(-0.957826285221151,-0.143673942783173,-0.248850568624199));
#56123=DIRECTION('',(-0.868243142124459,-0.248069469178417,-0.429668924423659));
#56124=DIRECTION('',(-0.948683298050514,-0.158113883008419,-0.273861278752584));
#56125=DIRECTION('',(-1.,0.,0.));
#56126=DIRECTION('',(-0.948683298050513,0.15811388300842,0.273861278752585));
#56127=DIRECTION('',(-0.86824314212446,0.248069469178416,0.429668924423658));
#56128=DIRECTION('',(-0.957826285221151,0.143673942783173,0.248850568624199));
#56129=DIRECTION('',(-0.998052578482888,-0.0311891430775903,-0.0540211804549215));
#56130=DIRECTION('',(0.,-0.5,-0.866025403784439));
#56131=DIRECTION('',(-1.,0.,0.));
#56132=DIRECTION('',(-0.755033118392644,0.327843327723122,0.567841300538901));
#56133=DIRECTION('center_axis',(0.649305557988371,-0.253315153038431,-0.717100917309779));
#56134=DIRECTION('ref_axis',(0.755033118392643,0.327843327723122,0.567841300538901));
#56135=DIRECTION('',(0.,-0.942899217429894,0.333078167657524));
#56136=DIRECTION('',(-0.755033118392644,-0.327843327723122,-0.567841300538901));
#56137=DIRECTION('center_axis',(-0.649305557988371,0.253315153038431,0.717100917309779));
#56138=DIRECTION('ref_axis',(0.760527640763576,0.216269505504613,0.612229702500115));
#56139=DIRECTION('',(0.0519254248777275,-0.925933051260728,0.374101236076902));
#56140=DIRECTION('center_axis',(0.,-0.939692620785908,0.342020143325669));
#56141=DIRECTION('ref_axis',(1.,0.,0.));
#56142=DIRECTION('',(0.755033118392643,0.224258043872453,0.616143911670627));
#56143=DIRECTION('',(1.,0.,0.));
#56144=DIRECTION('',(0.,-0.342020143325669,-0.939692620785908));
#56145=DIRECTION('',(0.998052578482888,-0.0213346303712044,-0.058616415197295));
#56146=DIRECTION('',(0.957826285221151,0.0982787650057294,0.270018687665128));
#56147=DIRECTION('',(0.86824314212446,0.169689510806249,0.46621809925847));
#56148=DIRECTION('',(0.948683298050513,0.108156265856636,0.297156898213637));
#56149=DIRECTION('',(1.,0.,0.));
#56150=DIRECTION('',(0.948683298050514,-0.108156265856635,-0.297156898213636));
#56151=DIRECTION('',(0.868243142124459,-0.169689510806249,-0.466218099258471));
#56152=DIRECTION('',(0.957826285221151,-0.0982787650057295,-0.270018687665129));
#56153=DIRECTION('',(0.998052578482888,0.0213346303712044,0.0586164151972949));
#56154=DIRECTION('',(0.,0.342020143325669,0.939692620785908));
#56155=DIRECTION('',(1.,0.,0.));
#56156=DIRECTION('',(0.755033118392644,-0.224258043872452,-0.616143911670627));
#56157=DIRECTION('',(-0.755033118392644,-0.224258043872452,-0.616143911670627));
#56158=DIRECTION('',(-1.,0.,0.));
#56159=DIRECTION('',(0.,0.342020143325669,0.939692620785908));
#56160=DIRECTION('',(-0.998052578482888,0.0213346303712044,0.0586164151972949));
#56161=DIRECTION('',(-0.957826285221151,-0.0982787650057295,-0.270018687665129));
#56162=DIRECTION('',(-0.868243142124459,-0.169689510806249,-0.466218099258471));
#56163=DIRECTION('',(-0.948683298050514,-0.108156265856635,-0.297156898213636));
#56164=DIRECTION('',(-1.,0.,0.));
#56165=DIRECTION('',(-0.948683298050513,0.108156265856636,0.297156898213637));
#56166=DIRECTION('',(-0.86824314212446,0.169689510806249,0.46621809925847));
#56167=DIRECTION('',(-0.957826285221151,0.0982787650057294,0.270018687665128));
#56168=DIRECTION('',(-0.998052578482888,-0.0213346303712044,-0.058616415197295));
#56169=DIRECTION('',(0.,-0.342020143325669,-0.939692620785908));
#56170=DIRECTION('',(-1.,0.,0.));
#56171=DIRECTION('',(-0.755033118392643,0.224258043872453,0.616143911670627));
#56172=DIRECTION('center_axis',(0.649305557988371,-0.124943459173594,-0.75019425775938));
#56173=DIRECTION('ref_axis',(0.755033118392643,0.224258043872453,0.616143911670627));
#56174=DIRECTION('',(0.,-0.986412876468473,0.164285231037954));
#56175=DIRECTION('',(-0.755033118392643,-0.224258043872453,-0.616143911670627));
#56176=DIRECTION('center_axis',(-0.649305557988371,0.124943459173594,0.75019425775938));
#56177=DIRECTION('ref_axis',(0.760527640763576,0.106671313608347,0.640483363162275));
#56178=DIRECTION('',(0.0519254248777275,-0.976828045559515,0.207631210706978));
#56179=DIRECTION('center_axis',(0.,-0.984807753012208,0.173648177666931));
#56180=DIRECTION('ref_axis',(1.,0.,0.));
#56181=DIRECTION('',(0.755033118392644,0.113858792838765,0.645725301830105));
#56182=DIRECTION('',(1.,0.,0.));
#56183=DIRECTION('',(0.,-0.173648177666931,-0.984807753012208));
#56184=DIRECTION('',(0.998052578482888,-0.0108318757168334,-0.0614306198252359));
#56185=DIRECTION('',(0.957826285221151,0.0498974366850416,0.282982425517402));
#56186=DIRECTION('',(0.86824314212446,0.0861536225152695,0.488601473065054));
#56187=DIRECTION('',(0.948683298050513,0.0549123752965088,0.311423555691114));
#56188=DIRECTION('',(1.,0.,0.));
#56189=DIRECTION('',(0.948683298050514,-0.0549123752965086,-0.311423555691113));
#56190=DIRECTION('',(0.868243142124459,-0.0861536225152698,-0.488601473065055));
#56191=DIRECTION('',(0.957826285221151,-0.0498974366850417,-0.282982425517402));
#56192=DIRECTION('',(0.998052578482888,0.0108318757168334,0.0614306198252358));
#56193=DIRECTION('',(0.,0.173648177666931,0.984807753012208));
#56194=DIRECTION('',(1.,0.,0.));
#56195=DIRECTION('',(0.755033118392644,-0.113858792838765,-0.645725301830104));
#56196=DIRECTION('',(-0.755033118392644,-0.113858792838765,-0.645725301830104));
#56197=DIRECTION('',(-1.,0.,0.));
#56198=DIRECTION('',(0.,0.173648177666931,0.984807753012208));
#56199=DIRECTION('',(-0.998052578482888,0.0108318757168334,0.0614306198252358));
#56200=DIRECTION('',(-0.957826285221151,-0.0498974366850417,-0.282982425517402));
#56201=DIRECTION('',(-0.868243142124459,-0.0861536225152698,-0.488601473065055));
#56202=DIRECTION('',(-0.948683298050514,-0.0549123752965086,-0.311423555691113));
#56203=DIRECTION('',(-1.,0.,0.));
#56204=DIRECTION('',(-0.948683298050513,0.0549123752965088,0.311423555691114));
#56205=DIRECTION('',(-0.86824314212446,0.0861536225152695,0.488601473065054));
#56206=DIRECTION('',(-0.957826285221151,0.0498974366850416,0.282982425517402));
#56207=DIRECTION('',(-0.998052578482888,-0.0108318757168334,-0.0614306198252359));
#56208=DIRECTION('',(0.,-0.173648177666931,-0.984807753012208));
#56209=DIRECTION('',(-1.,0.,0.));
#56210=DIRECTION('',(-0.755033118392644,0.113858792838765,0.645725301830105));
#56211=DIRECTION('center_axis',(0.649305557988371,0.00722457847379199,-0.760493325303573));
#56212=DIRECTION('ref_axis',(0.755033118392643,0.113858792838765,0.645725301830105));
#56213=DIRECTION('',(0.,-0.999954879404557,-0.00949942919436624));
#56214=DIRECTION('',(-0.755033118392644,-0.113858792838765,-0.645725301830105));
#56215=DIRECTION('center_axis',(-0.649305557988371,-0.00722457847379199,
0.760493325303573));
#56216=DIRECTION('ref_axis',(-0.760527640763576,0.00616803217361895,-0.64927626093497));
#56217=DIRECTION('',(0.0519254248777275,-0.998042613992818,0.0348524160661848));
#56218=DIRECTION('center_axis',(0.,-1.,1.22464679914735E-16));
#56219=DIRECTION('ref_axis',(1.,0.,0.));
#56220=DIRECTION('',(0.755033118392644,8.02984563835875E-17,0.655686655446243));
#56221=DIRECTION('',(1.,0.,0.));
#56222=DIRECTION('',(0.,-1.22464679914735E-16,-1.));
#56223=DIRECTION('',(0.998052578482888,-7.63913684762395E-18,-0.0623782861551806));
#56224=DIRECTION('',(0.957826285221151,3.51899668300585E-17,0.287347885566345));
#56225=DIRECTION('',(0.86824314212446,6.0759496279106E-17,0.496138938356832));
#56226=DIRECTION('',(0.948683298050513,3.87267321454041E-17,0.31622776601684));
#56227=DIRECTION('',(1.,0.,0.));
#56228=DIRECTION('',(0.948683298050514,-3.8726732145404E-17,-0.316227766016839));
#56229=DIRECTION('',(0.868243142124459,-6.07594962791062E-17,-0.496138938356833));
#56230=DIRECTION('',(0.957826285221151,-3.51899668300585E-17,-0.287347885566346));
#56231=DIRECTION('',(0.998052578482888,7.63913684762395E-18,0.0623782861551805));
#56232=DIRECTION('',(0.,1.22464679914735E-16,1.));
#56233=DIRECTION('',(1.,0.,0.));
#56234=DIRECTION('',(0.755033118392644,-8.02984563835875E-17,-0.655686655446243));
#56235=DIRECTION('',(-0.755033118392644,-8.02984563835875E-17,-0.655686655446243));
#56236=DIRECTION('',(-1.,0.,0.));
#56237=DIRECTION('',(0.,1.22464679914735E-16,1.));
#56238=DIRECTION('',(-0.998052578482888,7.63913684762395E-18,0.0623782861551805));
#56239=DIRECTION('',(-0.957826285221151,-3.51899668300585E-17,-0.287347885566346));
#56240=DIRECTION('',(-0.868243142124459,-6.07594962791062E-17,-0.496138938356833));
#56241=DIRECTION('',(-0.948683298050514,-3.8726732145404E-17,-0.316227766016839));
#56242=DIRECTION('',(-1.,0.,0.));
#56243=DIRECTION('',(-0.948683298050513,3.87267321454041E-17,0.31622776601684));
#56244=DIRECTION('',(-0.86824314212446,6.0759496279106E-17,0.496138938356832));
#56245=DIRECTION('',(-0.957826285221151,3.51899668300585E-17,0.287347885566345));
#56246=DIRECTION('',(-0.998052578482888,-7.63913684762395E-18,-0.0623782861551806));
#56247=DIRECTION('',(0.,-1.22464679914735E-16,-1.));
#56248=DIRECTION('',(-1.,0.,0.));
#56249=DIRECTION('',(-0.755033118392644,8.02984563835875E-17,0.655686655446243));
#56250=DIRECTION('center_axis',(0.649305557988371,0.139173100960065,-0.747685187986608));
#56251=DIRECTION('ref_axis',(0.755033118392643,8.02984563835875E-17,0.655686655446243));
#56252=DIRECTION('',(0.,-0.983113759331517,-0.182995454077559));
#56253=DIRECTION('',(-0.755033118392644,-8.02984563835875E-17,-0.655686655446243));
#56254=DIRECTION('center_axis',(-0.649305557988371,-0.139173100960065,0.747685187986608));
#56255=DIRECTION('ref_axis',(-0.760527640763576,0.118819965419165,-0.638341228068795));
#56256=DIRECTION('',(0.0519254248777275,-0.98893216263388,-0.138985351600607));
#56257=DIRECTION('center_axis',(0.,-0.984807753012208,-0.17364817766693));
#56258=DIRECTION('ref_axis',(1.,0.,0.));
#56259=DIRECTION('',(0.755033118392643,-0.113858792838764,0.645725301830105));
#56260=DIRECTION('',(1.,0.,0.));
#56261=DIRECTION('',(0.,0.17364817766693,-0.984807753012208));
#56262=DIRECTION('',(0.998052578482888,0.0108318757168334,-0.0614306198252359));
#56263=DIRECTION('',(0.957826285221151,-0.0498974366850414,0.282982425517402));
#56264=DIRECTION('',(0.86824314212446,-0.0861536225152693,0.488601473065054));
#56265=DIRECTION('',(0.948683298050513,-0.0549123752965086,0.311423555691114));
#56266=DIRECTION('',(1.,0.,0.));
#56267=DIRECTION('',(0.948683298050514,0.0549123752965084,-0.311423555691113));
#56268=DIRECTION('',(0.868243142124459,0.0861536225152694,-0.488601473065055));
#56269=DIRECTION('',(0.957826285221151,0.0498974366850415,-0.282982425517402));
#56270=DIRECTION('',(0.998052578482888,-0.0108318757168334,0.0614306198252359));
#56271=DIRECTION('',(0.,-0.17364817766693,0.984807753012208));
#56272=DIRECTION('',(1.,0.,0.));
#56273=DIRECTION('',(0.755033118392644,0.113858792838764,-0.645725301830105));
#56274=DIRECTION('',(-0.755033118392644,0.113858792838764,-0.645725301830105));
#56275=DIRECTION('',(-1.,0.,0.));
#56276=DIRECTION('',(0.,-0.17364817766693,0.984807753012208));
#56277=DIRECTION('',(-0.998052578482888,-0.0108318757168334,0.0614306198252359));
#56278=DIRECTION('',(-0.957826285221151,0.0498974366850415,-0.282982425517402));
#56279=DIRECTION('',(-0.868243142124459,0.0861536225152694,-0.488601473065055));
#56280=DIRECTION('',(-0.948683298050514,0.0549123752965084,-0.311423555691113));
#56281=DIRECTION('',(-1.,0.,0.));
#56282=DIRECTION('',(-0.948683298050513,-0.0549123752965086,0.311423555691114));
#56283=DIRECTION('',(-0.86824314212446,-0.0861536225152693,0.488601473065054));
#56284=DIRECTION('',(-0.957826285221151,-0.0498974366850414,0.282982425517402));
#56285=DIRECTION('',(-0.998052578482888,0.0108318757168334,-0.0614306198252359));
#56286=DIRECTION('',(0.,0.17364817766693,-0.984807753012208));
#56287=DIRECTION('',(-1.,0.,0.));
#56288=DIRECTION('',(-0.755033118392643,-0.113858792838764,0.645725301830105));
#56289=DIRECTION('center_axis',(0.649305557988371,0.266892919198654,-0.712159014579631));
#56290=DIRECTION('ref_axis',(0.755033118392643,-0.113858792838764,0.645725301830105));
#56291=DIRECTION('',(0.,-0.936401225160756,-0.350931254688773));
#56292=DIRECTION('',(-0.755033118392643,0.113858792838764,-0.645725301830105));
#56293=DIRECTION('center_axis',(-0.649305557988371,-0.266892919198654,0.712159014579631));
#56294=DIRECTION('ref_axis',(-0.760527640763576,0.227861614141253,-0.608010520003998));
#56295=DIRECTION('',(0.0519254248777275,-0.949773507937132,-0.308600119688995));
#56296=DIRECTION('center_axis',(0.,-0.939692620785908,-0.342020143325669));
#56297=DIRECTION('ref_axis',(1.,0.,0.));
#56298=DIRECTION('',(0.755033118392644,-0.224258043872452,0.616143911670627));
#56299=DIRECTION('',(1.,0.,0.));
#56300=DIRECTION('',(0.,0.342020143325669,-0.939692620785909));
#56301=DIRECTION('',(0.998052578482888,0.0213346303712044,-0.058616415197295));
#56302=DIRECTION('',(0.957826285221151,-0.0982787650057293,0.270018687665128));
#56303=DIRECTION('',(0.86824314212446,-0.169689510806249,0.46621809925847));
#56304=DIRECTION('',(0.948683298050513,-0.108156265856636,0.297156898213637));
#56305=DIRECTION('',(1.,0.,0.));
#56306=DIRECTION('',(0.948683298050514,0.108156265856635,-0.297156898213636));
#56307=DIRECTION('',(0.868243142124459,0.169689510806249,-0.466218099258471));
#56308=DIRECTION('',(0.957826285221151,0.0982787650057294,-0.270018687665129));
#56309=DIRECTION('',(0.998052578482888,-0.0213346303712044,0.0586164151972949));
#56310=DIRECTION('',(0.,-0.342020143325669,0.939692620785909));
#56311=DIRECTION('',(1.,0.,0.));
#56312=DIRECTION('',(0.755033118392644,0.224258043872452,-0.616143911670627));
#56313=DIRECTION('',(-0.755033118392644,0.224258043872452,-0.616143911670627));
#56314=DIRECTION('',(-1.,0.,0.));
#56315=DIRECTION('',(0.,-0.342020143325669,0.939692620785909));
#56316=DIRECTION('',(-0.998052578482888,-0.0213346303712044,0.0586164151972949));
#56317=DIRECTION('',(-0.957826285221151,0.0982787650057294,-0.270018687665129));
#56318=DIRECTION('',(-0.868243142124459,0.169689510806249,-0.466218099258471));
#56319=DIRECTION('',(-0.948683298050514,0.108156265856635,-0.297156898213636));
#56320=DIRECTION('',(-1.,0.,0.));
#56321=DIRECTION('',(-0.948683298050513,-0.108156265856636,0.297156898213637));
#56322=DIRECTION('',(-0.86824314212446,-0.169689510806249,0.46621809925847));
#56323=DIRECTION('',(-0.957826285221151,-0.0982787650057293,0.270018687665128));
#56324=DIRECTION('',(-0.998052578482888,0.0213346303712044,-0.058616415197295));
#56325=DIRECTION('',(0.,0.342020143325669,-0.939692620785909));
#56326=DIRECTION('',(-1.,0.,0.));
#56327=DIRECTION('',(-0.755033118392644,-0.224258043872452,0.616143911670627));
#56328=DIRECTION('center_axis',(0.649305557988371,0.386503331141725,-0.654994249884502));
#56329=DIRECTION('ref_axis',(0.755033118392643,-0.224258043872452,0.616143911670627));
#56330=DIRECTION('',(0.,-0.861236613605368,-0.508204186706051));
#56331=DIRECTION('',(-0.755033118392644,0.224258043872452,-0.616143911670627));
#56332=DIRECTION('center_axis',(-0.649305557988371,-0.386503331141725,0.654994249884502));
#56333=DIRECTION('ref_axis',(-0.760527640763576,0.329979803021199,-0.559205719957048));
#56334=DIRECTION('',(0.0519254248777275,-0.881756465810299,-0.468838229299828));
#56335=DIRECTION('center_axis',(0.,-0.866025403784439,-0.5));
#56336=DIRECTION('ref_axis',(1.,0.,0.));
#56337=DIRECTION('',(0.755033118392644,-0.327843327723121,0.567841300538901));
#56338=DIRECTION('',(1.,0.,0.));
#56339=DIRECTION('',(0.,0.5,-0.866025403784439));
#56340=DIRECTION('',(0.998052578482888,0.0311891430775903,-0.0540211804549215));
#56341=DIRECTION('',(0.957826285221151,-0.143673942783173,0.248850568624199));
#56342=DIRECTION('',(0.86824314212446,-0.248069469178416,0.429668924423658));
#56343=DIRECTION('',(0.948683298050513,-0.15811388300842,0.273861278752585));
#56344=DIRECTION('',(1.,0.,0.));
#56345=DIRECTION('',(0.948683298050513,0.158113883008419,-0.273861278752584));
#56346=DIRECTION('',(0.868243142124459,0.248069469178416,-0.429668924423659));
#56347=DIRECTION('',(0.957826285221151,0.143673942783173,-0.248850568624199));
#56348=DIRECTION('',(0.998052578482888,-0.0311891430775902,0.0540211804549215));
#56349=DIRECTION('',(0.,-0.5,0.866025403784439));
#56350=DIRECTION('',(1.,0.,0.));
#56351=DIRECTION('',(0.755033118392644,0.327843327723121,-0.567841300538901));
#56352=DIRECTION('',(-0.755033118392644,0.327843327723121,-0.567841300538901));
#56353=DIRECTION('',(-1.,0.,0.));
#56354=DIRECTION('',(0.,-0.5,0.866025403784439));
#56355=DIRECTION('',(-0.998052578482888,-0.0311891430775902,0.0540211804549215));
#56356=DIRECTION('',(-0.957826285221151,0.143673942783173,-0.248850568624199));
#56357=DIRECTION('',(-0.868243142124459,0.248069469178416,-0.429668924423659));
#56358=DIRECTION('',(-0.948683298050513,0.158113883008419,-0.273861278752584));
#56359=DIRECTION('',(-1.,0.,0.));
#56360=DIRECTION('',(-0.948683298050513,-0.15811388300842,0.273861278752585));
#56361=DIRECTION('',(-0.86824314212446,-0.248069469178416,0.429668924423658));
#56362=DIRECTION('',(-0.957826285221151,-0.143673942783173,0.248850568624199));
#56363=DIRECTION('',(-0.998052578482888,0.0311891430775903,-0.0540211804549215));
#56364=DIRECTION('',(0.,0.5,-0.866025403784439));
#56365=DIRECTION('',(-1.,0.,0.));
#56366=DIRECTION('',(-0.755033118392644,-0.327843327723121,0.567841300538901));
#56367=DIRECTION('center_axis',(0.649305557988371,0.494370034948177,-0.577927816349714));
#56368=DIRECTION('ref_axis',(0.755033118392643,-0.327843327723121,0.567841300538901));
#56369=DIRECTION('',(0.,-0.759903763352335,-0.650035591673993));
#56370=DIRECTION('',(-0.755033118392644,0.327843327723121,-0.567841300538901));
#56371=DIRECTION('center_axis',(-0.649305557988371,-0.494370034948177,0.577927816349714));
#56372=DIRECTION('ref_axis',(-0.760527640763576,0.422071722564183,-0.493409737080951));
#56373=DIRECTION('',(0.0519254248777275,-0.786947699660121,-0.614830926556978));
#56374=DIRECTION('center_axis',(0.,-0.766044443118978,-0.642787609686539));
#56375=DIRECTION('ref_axis',(1.,0.,0.));
#56376=DIRECTION('',(0.755033118392644,-0.421467257957652,0.502285118831863));
#56377=DIRECTION('',(1.,0.,0.));
#56378=DIRECTION('',(0.,0.642787609686539,-0.766044443118978));
#56379=DIRECTION('',(0.998052578482888,0.0400959894540315,-0.0477845394804616));
#56380=DIRECTION('',(0.957826285221151,-0.184703660511672,0.220121250980087));
#56381=DIRECTION('',(0.86824314212446,-0.318911962258805,0.3800644767432));
#56382=DIRECTION('',(0.948683298050513,-0.203267289834479,0.242244522917128));
#56383=DIRECTION('',(1.,0.,0.));
#56384=DIRECTION('',(0.948683298050514,0.203267289834478,-0.242244522917128));
#56385=DIRECTION('',(0.868243142124459,0.318911962258806,-0.380064476743201));
#56386=DIRECTION('',(0.957826285221151,0.184703660511673,-0.220121250980087));
#56387=DIRECTION('',(0.998052578482888,-0.0400959894540314,0.0477845394804615));
#56388=DIRECTION('',(0.,-0.642787609686539,0.766044443118978));
#56389=DIRECTION('',(1.,0.,0.));
#56390=DIRECTION('',(0.755033118392644,0.421467257957652,-0.502285118831862));
#56391=DIRECTION('',(-0.755033118392644,0.421467257957652,-0.502285118831862));
#56392=DIRECTION('',(-1.,0.,0.));
#56393=DIRECTION('',(0.,-0.642787609686539,0.766044443118978));
#56394=DIRECTION('',(-0.998052578482888,-0.0400959894540314,0.0477845394804615));
#56395=DIRECTION('',(-0.957826285221151,0.184703660511673,-0.220121250980087));
#56396=DIRECTION('',(-0.868243142124459,0.318911962258806,-0.380064476743201));
#56397=DIRECTION('',(-0.948683298050514,0.203267289834478,-0.242244522917128));
#56398=DIRECTION('',(-1.,0.,0.));
#56399=DIRECTION('',(-0.948683298050513,-0.203267289834479,0.242244522917128));
#56400=DIRECTION('',(-0.86824314212446,-0.318911962258805,0.3800644767432));
#56401=DIRECTION('',(-0.957826285221151,-0.184703660511672,0.220121250980087));
#56402=DIRECTION('',(-0.998052578482888,0.0400959894540315,-0.0477845394804616));
#56403=DIRECTION('',(0.,0.642787609686539,-0.766044443118978));
#56404=DIRECTION('',(-1.,0.,0.));
#56405=DIRECTION('',(-0.755033118392644,-0.421467257957652,0.502285118831863));
#56406=DIRECTION('center_axis',(0.649305557988371,0.587215555406037,-0.483301338560726));
#56407=DIRECTION('ref_axis',(0.755033118392643,-0.421467257957652,0.502285118831863));
#56408=DIRECTION('',(0.,-0.6354816217797,-0.772115994122802));
#56409=DIRECTION('',(-0.755033118392644,0.421467257957652,-0.502285118831863));
#56410=DIRECTION('center_axis',(-0.649305557988371,-0.587215555406037,0.483301338560726));
#56411=DIRECTION('ref_axis',(-0.760527640763576,0.501339206395651,-0.412621749021023));
#56412=DIRECTION('',(0.0519254248777275,-0.66822792587052,-0.742142297230154));
#56413=DIRECTION('center_axis',(0.,-0.642787609686539,-0.766044443118978));
#56414=DIRECTION('ref_axis',(1.,0.,0.));
#56415=DIRECTION('',(0.755033118392644,-0.502285118831862,0.421467257957652));
#56416=DIRECTION('',(1.,0.,0.));
#56417=DIRECTION('',(0.,0.766044443118978,-0.642787609686539));
#56418=DIRECTION('',(0.998052578482888,0.0477845394804615,-0.0400959894540315));
#56419=DIRECTION('',(0.957826285221151,-0.220121250980087,0.184703660511672));
#56420=DIRECTION('',(0.86824314212446,-0.3800644767432,0.318911962258805));
#56421=DIRECTION('',(0.948683298050513,-0.242244522917128,0.203267289834479));
#56422=DIRECTION('',(1.,0.,0.));
#56423=DIRECTION('',(0.948683298050514,0.242244522917128,-0.203267289834478));
#56424=DIRECTION('',(0.86824314212446,0.380064476743201,-0.318911962258806));
#56425=DIRECTION('',(0.957826285221151,0.220121250980087,-0.184703660511673));
#56426=DIRECTION('',(0.998052578482888,-0.0477845394804615,0.0400959894540314));
#56427=DIRECTION('',(0.,-0.766044443118978,0.642787609686539));
#56428=DIRECTION('',(1.,0.,0.));
#56429=DIRECTION('',(0.755033118392644,0.502285118831862,-0.421467257957652));
#56430=DIRECTION('',(-0.755033118392644,0.502285118831862,-0.421467257957652));
#56431=DIRECTION('',(-1.,0.,0.));
#56432=DIRECTION('',(0.,-0.766044443118978,0.642787609686539));
#56433=DIRECTION('',(-0.998052578482888,-0.0477845394804615,0.0400959894540314));
#56434=DIRECTION('',(-0.957826285221151,0.220121250980087,-0.184703660511673));
#56435=DIRECTION('',(-0.86824314212446,0.380064476743201,-0.318911962258806));
#56436=DIRECTION('',(-0.948683298050514,0.242244522917128,-0.203267289834478));
#56437=DIRECTION('',(-1.,0.,0.));
#56438=DIRECTION('',(-0.948683298050513,-0.242244522917128,0.203267289834479));
#56439=DIRECTION('',(-0.86824314212446,-0.3800644767432,0.318911962258805));
#56440=DIRECTION('',(-0.957826285221151,-0.220121250980087,0.184703660511672));
#56441=DIRECTION('',(-0.998052578482888,0.0477845394804615,-0.0400959894540315));
#56442=DIRECTION('',(0.,0.766044443118978,-0.642787609686539));
#56443=DIRECTION('',(-1.,0.,0.));
#56444=DIRECTION('',(-0.755033118392644,-0.502285118831862,0.421467257957652));
#56445=DIRECTION('center_axis',(0.649305557988371,0.662218828358294,-0.373989994161848));
#56446=DIRECTION('ref_axis',(0.755033118392643,-0.502285118831862,0.421467257957652));
#56447=DIRECTION('',(0.,-0.491750692698505,-0.870736042799734));
#56448=DIRECTION('',(-0.755033118392644,0.502285118831862,-0.421467257957652));
#56449=DIRECTION('center_axis',(-0.649305557988371,-0.662218828358294,0.373989994161848));
#56450=DIRECTION('ref_axis',(-0.760527640763576,0.565373752130667,-0.319296457913771));
#56451=DIRECTION('',(0.0519254248777275,-0.52920438469299,-0.846904049744115));
#56452=DIRECTION('center_axis',(0.,-0.5,-0.866025403784438));
#56453=DIRECTION('ref_axis',(1.,0.,0.));
#56454=DIRECTION('',(0.755033118392644,-0.567841300538901,0.327843327723122));
#56455=DIRECTION('',(1.,0.,0.));
#56456=DIRECTION('',(0.,0.866025403784438,-0.5));
#56457=DIRECTION('',(0.998052578482888,0.0540211804549215,-0.0311891430775903));
#56458=DIRECTION('',(0.957826285221151,-0.248850568624199,0.143673942783173));
#56459=DIRECTION('',(0.86824314212446,-0.429668924423658,0.248069469178416));
#56460=DIRECTION('',(0.948683298050513,-0.273861278752584,0.15811388300842));
#56461=DIRECTION('',(1.,0.,0.));
#56462=DIRECTION('',(0.948683298050514,0.273861278752584,-0.158113883008419));
#56463=DIRECTION('',(0.86824314212446,0.429668924423659,-0.248069469178417));
#56464=DIRECTION('',(0.957826285221151,0.248850568624199,-0.143673942783173));
#56465=DIRECTION('',(0.998052578482888,-0.0540211804549214,0.0311891430775903));
#56466=DIRECTION('',(0.,-0.866025403784438,0.5));
#56467=DIRECTION('',(1.,0.,0.));
#56468=DIRECTION('',(0.755033118392644,0.567841300538901,-0.327843327723122));
#56469=DIRECTION('',(-0.755033118392644,0.567841300538901,-0.327843327723122));
#56470=DIRECTION('',(-1.,0.,0.));
#56471=DIRECTION('',(0.,-0.866025403784438,0.5));
#56472=DIRECTION('',(-0.998052578482888,-0.0540211804549214,0.0311891430775903));
#56473=DIRECTION('',(-0.957826285221151,0.248850568624199,-0.143673942783173));
#56474=DIRECTION('',(-0.86824314212446,0.429668924423659,-0.248069469178417));
#56475=DIRECTION('',(-0.948683298050514,0.273861278752584,-0.158113883008419));
#56476=DIRECTION('',(-1.,0.,0.));
#56477=DIRECTION('',(-0.948683298050513,-0.273861278752584,0.15811388300842));
#56478=DIRECTION('',(-0.86824314212446,-0.429668924423658,0.248069469178416));
#56479=DIRECTION('',(-0.957826285221151,-0.248850568624199,0.143673942783173));
#56480=DIRECTION('',(-0.998052578482888,0.0540211804549215,-0.0311891430775903));
#56481=DIRECTION('',(0.,0.866025403784438,-0.5));
#56482=DIRECTION('',(-1.,0.,0.));
#56483=DIRECTION('',(-0.755033118392644,-0.567841300538901,0.327843327723122));
#56484=DIRECTION('center_axis',(0.649305557988371,0.717100917309779,-0.253315153038432));
#56485=DIRECTION('ref_axis',(0.755033118392643,-0.567841300538901,0.327843327723122));
#56486=DIRECTION('',(0.,-0.333078167657524,-0.942899217429894));
#56487=DIRECTION('',(-0.755033118392644,0.567841300538901,-0.327843327723122));
#56488=DIRECTION('center_axis',(-0.649305557988371,-0.717100917309779,0.253315153038432));
#56489=DIRECTION('ref_axis',(-0.760527640763576,0.612229702500115,-0.216269505504613));
#56490=DIRECTION('',(0.0519254248777275,-0.374101236076903,-0.925933051260727));
#56491=DIRECTION('center_axis',(0.,-0.342020143325669,-0.939692620785908));
#56492=DIRECTION('ref_axis',(1.,0.,0.));
#56493=DIRECTION('',(0.755033118392644,-0.616143911670627,0.224258043872453));
#56494=DIRECTION('',(1.,0.,0.));
#56495=DIRECTION('',(0.,0.939692620785908,-0.342020143325669));
#56496=DIRECTION('',(0.998052578482888,0.0586164151972949,-0.0213346303712045));
#56497=DIRECTION('',(0.957826285221151,-0.270018687665128,0.0982787650057295));
#56498=DIRECTION('',(0.86824314212446,-0.46621809925847,0.169689510806249));
#56499=DIRECTION('',(0.948683298050513,-0.297156898213637,0.108156265856636));
#56500=DIRECTION('',(1.,0.,0.));
#56501=DIRECTION('',(0.948683298050514,0.297156898213636,-0.108156265856635));
#56502=DIRECTION('',(0.868243142124459,0.466218099258471,-0.16968951080625));
#56503=DIRECTION('',(0.957826285221151,0.270018687665129,-0.0982787650057297));
#56504=DIRECTION('',(0.998052578482888,-0.0586164151972949,0.0213346303712045));
#56505=DIRECTION('',(0.,-0.939692620785908,0.342020143325669));
#56506=DIRECTION('',(1.,0.,0.));
#56507=DIRECTION('',(0.755033118392644,0.616143911670627,-0.224258043872453));
#56508=DIRECTION('',(-0.755033118392644,0.616143911670627,-0.224258043872453));
#56509=DIRECTION('',(-1.,0.,0.));
#56510=DIRECTION('',(0.,-0.939692620785908,0.342020143325669));
#56511=DIRECTION('',(-0.998052578482888,-0.0586164151972949,0.0213346303712045));
#56512=DIRECTION('',(-0.957826285221151,0.270018687665129,-0.0982787650057297));
#56513=DIRECTION('',(-0.868243142124459,0.466218099258471,-0.16968951080625));
#56514=DIRECTION('',(-0.948683298050514,0.297156898213636,-0.108156265856635));
#56515=DIRECTION('',(-1.,0.,0.));
#56516=DIRECTION('',(-0.948683298050513,-0.297156898213637,0.108156265856636));
#56517=DIRECTION('',(-0.86824314212446,-0.46621809925847,0.169689510806249));
#56518=DIRECTION('',(-0.957826285221151,-0.270018687665128,0.0982787650057295));
#56519=DIRECTION('',(-0.998052578482888,0.0586164151972949,-0.0213346303712045));
#56520=DIRECTION('',(0.,0.939692620785908,-0.342020143325669));
#56521=DIRECTION('',(-1.,0.,0.));
#56522=DIRECTION('',(-0.755033118392644,-0.616143911670627,0.224258043872453));
#56523=DIRECTION('center_axis',(0.649305557988371,0.75019425775938,-0.124943459173594));
#56524=DIRECTION('ref_axis',(0.755033118392643,-0.616143911670627,0.224258043872453));
#56525=DIRECTION('',(0.,-0.164285231037954,-0.986412876468473));
#56526=DIRECTION('',(-0.755033118392644,0.616143911670627,-0.224258043872453));
#56527=DIRECTION('center_axis',(-0.649305557988371,-0.75019425775938,0.124943459173594));
#56528=DIRECTION('ref_axis',(-0.760527640763576,0.640483363162275,-0.106671313608347));
#56529=DIRECTION('',(0.0519254248777275,-0.207631210706979,-0.976828045559515));
#56530=DIRECTION('center_axis',(0.,-0.17364817766693,-0.984807753012208));
#56531=DIRECTION('ref_axis',(1.,0.,0.));
#56532=DIRECTION('',(0.755033118392643,-0.645725301830105,0.113858792838765));
#56533=DIRECTION('',(1.,0.,0.));
#56534=DIRECTION('',(0.,0.984807753012208,-0.17364817766693));
#56535=DIRECTION('',(0.998052578482888,0.0614306198252359,-0.0108318757168334));
#56536=DIRECTION('',(0.957826285221151,-0.282982425517402,0.0498974366850415));
#56537=DIRECTION('',(0.86824314212446,-0.488601473065054,0.0861536225152694));
#56538=DIRECTION('',(0.948683298050513,-0.311423555691114,0.0549123752965087));
#56539=DIRECTION('',(1.,0.,0.));
#56540=DIRECTION('',(0.948683298050514,0.311423555691113,-0.0549123752965085));
#56541=DIRECTION('',(0.868243142124459,0.488601473065055,-0.0861536225152696));
#56542=DIRECTION('',(0.957826285221151,0.282982425517402,-0.0498974366850416));
#56543=DIRECTION('',(0.998052578482888,-0.0614306198252359,0.0108318757168334));
#56544=DIRECTION('',(0.,-0.984807753012208,0.17364817766693));
#56545=DIRECTION('',(1.,0.,0.));
#56546=DIRECTION('',(0.755033118392644,0.645725301830105,-0.113858792838765));
#56547=DIRECTION('',(-0.755033118392644,0.645725301830105,-0.113858792838765));
#56548=DIRECTION('',(-1.,0.,0.));
#56549=DIRECTION('',(0.,-0.984807753012208,0.17364817766693));
#56550=DIRECTION('',(-0.998052578482888,-0.0614306198252359,0.0108318757168334));
#56551=DIRECTION('',(-0.957826285221151,0.282982425517402,-0.0498974366850416));
#56552=DIRECTION('',(-0.868243142124459,0.488601473065055,-0.0861536225152696));
#56553=DIRECTION('',(-0.948683298050514,0.311423555691113,-0.0549123752965085));
#56554=DIRECTION('',(-1.,0.,0.));
#56555=DIRECTION('',(-0.948683298050513,-0.311423555691114,0.0549123752965087));
#56556=DIRECTION('',(-0.86824314212446,-0.488601473065054,0.0861536225152694));
#56557=DIRECTION('',(-0.957826285221151,-0.282982425517402,0.0498974366850415));
#56558=DIRECTION('',(-0.998052578482888,0.0614306198252359,-0.0108318757168334));
#56559=DIRECTION('',(0.,0.984807753012208,-0.17364817766693));
#56560=DIRECTION('',(-1.,0.,0.));
#56561=DIRECTION('',(-0.755033118392643,-0.645725301830105,0.113858792838765));
#56562=DIRECTION('center_axis',(0.649305557988371,0.760493325303573,0.00722457847379226));
#56563=DIRECTION('ref_axis',(0.755033118392643,-0.645725301830105,0.113858792838765));
#56564=DIRECTION('',(0.,0.0094994291943666,-0.999954879404557));
#56565=DIRECTION('',(-0.755033118392643,0.645725301830105,-0.113858792838765));
#56566=DIRECTION('center_axis',(-0.649305557988371,-0.760493325303573,-0.00722457847379226));
#56567=DIRECTION('ref_axis',(-0.760527640763576,0.64927626093497,0.00616803217361923));
#56568=DIRECTION('',(0.0519254248777275,-0.0348524160661844,-0.998042613992818));
#56569=DIRECTION('center_axis',(0.,-1.83697019872103E-16,-1.));
#56570=DIRECTION('ref_axis',(1.,0.,0.));
#56571=DIRECTION('',(0.755033118392644,-0.655686655446243,1.20447684575381E-16));
#56572=DIRECTION('',(1.,0.,0.));
#56573=DIRECTION('',(0.,1.,-1.83697019872103E-16));
#56574=DIRECTION('',(0.998052578482888,0.0623782861551806,-1.14587052714359E-17));
#56575=DIRECTION('',(0.957826285221151,-0.287347885566345,5.27849502450877E-17));
#56576=DIRECTION('',(0.86824314212446,-0.496138938356832,9.11392444186591E-17));
#56577=DIRECTION('',(0.948683298050513,-0.31622776601684,5.80900982181061E-17));
#56578=DIRECTION('',(1.,0.,0.));
#56579=DIRECTION('',(0.948683298050514,0.316227766016839,-5.80900982181059E-17));
#56580=DIRECTION('',(0.868243142124459,0.496138938356833,-9.11392444186592E-17));
#56581=DIRECTION('',(0.957826285221151,0.287347885566346,-5.27849502450878E-17));
#56582=DIRECTION('',(0.998052578482888,-0.0623782861551805,1.14587052714359E-17));
#56583=DIRECTION('',(0.,-1.,1.83697019872103E-16));
#56584=DIRECTION('',(1.,0.,0.));
#56585=DIRECTION('',(0.755033118392644,0.655686655446243,-1.20447684575381E-16));
#56586=DIRECTION('',(-0.755033118392644,0.655686655446243,-1.20447684575381E-16));
#56587=DIRECTION('',(-1.,0.,0.));
#56588=DIRECTION('',(0.,-1.,1.83697019872103E-16));
#56589=DIRECTION('',(-0.998052578482888,-0.0623782861551805,1.14587052714359E-17));
#56590=DIRECTION('',(-0.957826285221151,0.287347885566346,-5.27849502450878E-17));
#56591=DIRECTION('',(-0.868243142124459,0.496138938356833,-9.11392444186592E-17));
#56592=DIRECTION('',(-0.948683298050514,0.316227766016839,-5.80900982181059E-17));
#56593=DIRECTION('',(-1.,0.,0.));
#56594=DIRECTION('',(-0.948683298050513,-0.31622776601684,5.80900982181061E-17));
#56595=DIRECTION('',(-0.86824314212446,-0.496138938356832,9.11392444186591E-17));
#56596=DIRECTION('',(-0.957826285221151,-0.287347885566345,5.27849502450877E-17));
#56597=DIRECTION('',(-0.998052578482888,0.0623782861551806,-1.14587052714359E-17));
#56598=DIRECTION('',(0.,1.,-1.83697019872103E-16));
#56599=DIRECTION('',(-1.,0.,0.));
#56600=DIRECTION('',(-0.755033118392644,-0.655686655446243,1.20447684575381E-16));
#56601=DIRECTION('center_axis',(0.649305557988371,0.747685187986609,0.139173100960065));
#56602=DIRECTION('ref_axis',(0.755033118392643,-0.655686655446243,1.20447684575381E-16));
#56603=DIRECTION('',(0.,0.182995454077559,-0.983113759331517));
#56604=DIRECTION('',(-0.755033118392644,0.655686655446243,-1.20447684575381E-16));
#56605=DIRECTION('center_axis',(-0.649305557988371,-0.747685187986609,-0.139173100960065));
#56606=DIRECTION('ref_axis',(-0.760527640763576,0.638341228068795,0.118819965419165));
#56607=DIRECTION('',(0.0519254248777275,0.138985351600607,-0.98893216263388));
#56608=DIRECTION('center_axis',(0.,0.17364817766693,-0.984807753012208));
#56609=DIRECTION('ref_axis',(1.,0.,0.));
#56610=DIRECTION('',(0.755033118392643,-0.645725301830105,-0.113858792838764));
#56611=DIRECTION('',(1.,0.,0.));
#56612=DIRECTION('',(0.,0.984807753012208,0.17364817766693));
#56613=DIRECTION('',(0.998052578482888,0.0614306198252359,0.0108318757168334));
#56614=DIRECTION('',(0.957826285221151,-0.282982425517402,-0.0498974366850414));
#56615=DIRECTION('',(0.86824314212446,-0.488601473065054,-0.0861536225152692));
#56616=DIRECTION('',(0.948683298050513,-0.311423555691114,-0.0549123752965085));
#56617=DIRECTION('',(1.,0.,0.));
#56618=DIRECTION('',(0.948683298050514,0.311423555691113,0.0549123752965084));
#56619=DIRECTION('',(0.86824314212446,0.488601473065055,0.0861536225152694));
#56620=DIRECTION('',(0.957826285221151,0.282982425517402,0.0498974366850415));
#56621=DIRECTION('',(0.998052578482888,-0.0614306198252359,-0.0108318757168334));
#56622=DIRECTION('',(0.,-0.984807753012208,-0.17364817766693));
#56623=DIRECTION('',(1.,0.,0.));
#56624=DIRECTION('',(0.755033118392644,0.645725301830105,0.113858792838764));
#56625=DIRECTION('',(-0.755033118392644,0.645725301830105,0.113858792838764));
#56626=DIRECTION('',(-1.,0.,0.));
#56627=DIRECTION('',(0.,-0.984807753012208,-0.17364817766693));
#56628=DIRECTION('',(-0.998052578482888,-0.0614306198252359,-0.0108318757168334));
#56629=DIRECTION('',(-0.957826285221151,0.282982425517402,0.0498974366850415));
#56630=DIRECTION('',(-0.86824314212446,0.488601473065055,0.0861536225152694));
#56631=DIRECTION('',(-0.948683298050514,0.311423555691113,0.0549123752965084));
#56632=DIRECTION('',(-1.,0.,0.));
#56633=DIRECTION('',(-0.948683298050513,-0.311423555691114,-0.0549123752965085));
#56634=DIRECTION('',(-0.86824314212446,-0.488601473065054,-0.0861536225152692));
#56635=DIRECTION('',(-0.957826285221151,-0.282982425517402,-0.0498974366850414));
#56636=DIRECTION('',(-0.998052578482888,0.0614306198252359,0.0108318757168334));
#56637=DIRECTION('',(0.,0.984807753012208,0.17364817766693));
#56638=DIRECTION('',(-1.,0.,0.));
#56639=DIRECTION('',(-0.755033118392643,-0.645725301830105,-0.113858792838764));
#56640=DIRECTION('center_axis',(0.649305557988371,0.712159014579631,0.266892919198654));
#56641=DIRECTION('ref_axis',(0.755033118392643,-0.645725301830105,-0.113858792838764));
#56642=DIRECTION('',(0.,0.350931254688772,-0.936401225160756));
#56643=DIRECTION('',(-0.755033118392643,0.645725301830105,0.113858792838764));
#56644=DIRECTION('center_axis',(-0.649305557988371,-0.712159014579631,-0.266892919198654));
#56645=DIRECTION('ref_axis',(-0.760527640763576,0.608010520003999,0.227861614141252));
#56646=DIRECTION('',(0.0519254248777275,0.308600119688995,-0.949773507937132));
#56647=DIRECTION('center_axis',(0.,0.342020143325668,-0.939692620785909));
#56648=DIRECTION('ref_axis',(1.,0.,0.));
#56649=DIRECTION('',(0.755033118392643,-0.616143911670627,-0.224258043872452));
#56650=DIRECTION('',(1.,0.,0.));
#56651=DIRECTION('',(0.,0.939692620785909,0.342020143325668));
#56652=DIRECTION('',(0.998052578482888,0.058616415197295,0.0213346303712044));
#56653=DIRECTION('',(0.957826285221151,-0.270018687665128,-0.0982787650057291));
#56654=DIRECTION('',(0.86824314212446,-0.46621809925847,-0.169689510806249));
#56655=DIRECTION('',(0.948683298050513,-0.297156898213637,-0.108156265856635));
#56656=DIRECTION('',(1.,0.,0.));
#56657=DIRECTION('',(0.948683298050514,0.297156898213636,0.108156265856635));
#56658=DIRECTION('',(0.868243142124459,0.466218099258471,0.169689510806249));
#56659=DIRECTION('',(0.957826285221151,0.270018687665129,0.0982787650057293));
#56660=DIRECTION('',(0.998052578482888,-0.0586164151972949,-0.0213346303712044));
#56661=DIRECTION('',(0.,-0.939692620785909,-0.342020143325668));
#56662=DIRECTION('',(1.,0.,0.));
#56663=DIRECTION('',(0.755033118392644,0.616143911670627,0.224258043872452));
#56664=DIRECTION('',(-0.755033118392644,0.616143911670627,0.224258043872452));
#56665=DIRECTION('',(-1.,0.,0.));
#56666=DIRECTION('',(0.,-0.939692620785909,-0.342020143325668));
#56667=DIRECTION('',(-0.998052578482888,-0.0586164151972949,-0.0213346303712044));
#56668=DIRECTION('',(-0.957826285221151,0.270018687665129,0.0982787650057293));
#56669=DIRECTION('',(-0.868243142124459,0.466218099258471,0.169689510806249));
#56670=DIRECTION('',(-0.948683298050514,0.297156898213636,0.108156265856635));
#56671=DIRECTION('',(-1.,0.,0.));
#56672=DIRECTION('',(-0.948683298050513,-0.297156898213637,-0.108156265856635));
#56673=DIRECTION('',(-0.86824314212446,-0.46621809925847,-0.169689510806249));
#56674=DIRECTION('',(-0.957826285221151,-0.270018687665128,-0.0982787650057291));
#56675=DIRECTION('',(-0.998052578482888,0.058616415197295,0.0213346303712044));
#56676=DIRECTION('',(0.,0.939692620785909,0.342020143325668));
#56677=DIRECTION('',(-1.,0.,0.));
#56678=DIRECTION('',(-0.755033118392643,-0.616143911670627,-0.224258043872452));
#56679=DIRECTION('center_axis',(0.649305557988371,0.654994249884502,0.386503331141725));
#56680=DIRECTION('ref_axis',(0.755033118392643,-0.616143911670627,-0.224258043872452));
#56681=DIRECTION('',(0.,0.508204186706051,-0.861236613605368));
#56682=DIRECTION('',(-0.755033118392643,0.616143911670627,0.224258043872452));
#56683=DIRECTION('center_axis',(-0.649305557988371,-0.654994249884502,-0.386503331141725));
#56684=DIRECTION('ref_axis',(-0.760527640763576,0.559205719957048,0.329979803021198));
#56685=DIRECTION('',(0.0519254248777275,0.468838229299828,-0.881756465810299));
#56686=DIRECTION('center_axis',(0.,0.5,-0.866025403784439));
#56687=DIRECTION('ref_axis',(1.,0.,0.));
#56688=DIRECTION('',(0.755033118392644,-0.567841300538901,-0.327843327723122));
#56689=DIRECTION('',(1.,0.,0.));
#56690=DIRECTION('',(0.,0.866025403784439,0.5));
#56691=DIRECTION('',(0.998052578482888,0.0540211804549215,0.0311891430775903));
#56692=DIRECTION('',(0.957826285221151,-0.248850568624199,-0.143673942783173));
#56693=DIRECTION('',(0.86824314212446,-0.429668924423658,-0.248069469178416));
#56694=DIRECTION('',(0.948683298050513,-0.273861278752585,-0.15811388300842));
#56695=DIRECTION('',(1.,0.,0.));
#56696=DIRECTION('',(0.948683298050514,0.273861278752584,0.158113883008419));
#56697=DIRECTION('',(0.868243142124459,0.429668924423659,0.248069469178417));
#56698=DIRECTION('',(0.957826285221151,0.248850568624199,0.143673942783173));
#56699=DIRECTION('',(0.998052578482888,-0.0540211804549215,-0.0311891430775903));
#56700=DIRECTION('',(0.,-0.866025403784439,-0.5));
#56701=DIRECTION('',(1.,0.,0.));
#56702=DIRECTION('',(0.755033118392644,0.567841300538901,0.327843327723122));
#56703=DIRECTION('',(-0.755033118392644,0.567841300538901,0.327843327723122));
#56704=DIRECTION('',(-1.,0.,0.));
#56705=DIRECTION('',(0.,-0.866025403784439,-0.5));
#56706=DIRECTION('',(-0.998052578482888,-0.0540211804549215,-0.0311891430775903));
#56707=DIRECTION('',(-0.957826285221151,0.248850568624199,0.143673942783173));
#56708=DIRECTION('',(-0.868243142124459,0.429668924423659,0.248069469178417));
#56709=DIRECTION('',(-0.948683298050514,0.273861278752584,0.158113883008419));
#56710=DIRECTION('',(-1.,0.,0.));
#56711=DIRECTION('',(-0.948683298050513,-0.273861278752585,-0.15811388300842));
#56712=DIRECTION('',(-0.86824314212446,-0.429668924423658,-0.248069469178416));
#56713=DIRECTION('',(-0.957826285221151,-0.248850568624199,-0.143673942783173));
#56714=DIRECTION('',(-0.998052578482888,0.0540211804549215,0.0311891430775903));
#56715=DIRECTION('',(0.,0.866025403784439,0.5));
#56716=DIRECTION('',(-1.,0.,0.));
#56717=DIRECTION('',(-0.755033118392644,-0.567841300538901,-0.327843327723122));
#56718=DIRECTION('center_axis',(0.649305557988371,0.577927816349714,0.494370034948177));
#56719=DIRECTION('ref_axis',(0.755033118392643,-0.567841300538901,-0.327843327723122));
#56720=DIRECTION('',(0.,0.650035591673993,-0.759903763352335));
#56721=DIRECTION('',(-0.755033118392644,0.567841300538901,0.327843327723122));
#56722=DIRECTION('center_axis',(-0.649305557988371,-0.577927816349714,-0.494370034948177));
#56723=DIRECTION('ref_axis',(-0.760527640763576,0.493409737080951,0.422071722564183));
#56724=DIRECTION('',(0.0519254248777275,0.614830926556978,-0.786947699660121));
#56725=DIRECTION('center_axis',(0.,0.642787609686539,-0.766044443118978));
#56726=DIRECTION('ref_axis',(1.,0.,0.));
#56727=DIRECTION('',(0.755033118392644,-0.502285118831863,-0.421467257957652));
#56728=DIRECTION('',(1.,0.,0.));
#56729=DIRECTION('',(0.,0.766044443118978,0.642787609686539));
#56730=DIRECTION('',(0.998052578482888,0.0477845394804616,0.0400959894540314));
#56731=DIRECTION('',(0.957826285221151,-0.220121250980087,-0.184703660511672));
#56732=DIRECTION('',(0.86824314212446,-0.3800644767432,-0.318911962258805));
#56733=DIRECTION('',(0.948683298050513,-0.242244522917128,-0.203267289834479));
#56734=DIRECTION('',(1.,0.,0.));
#56735=DIRECTION('',(0.948683298050514,0.242244522917128,0.203267289834478));
#56736=DIRECTION('',(0.868243142124459,0.380064476743201,0.318911962258806));
#56737=DIRECTION('',(0.957826285221151,0.220121250980087,0.184703660511673));
#56738=DIRECTION('',(0.998052578482888,-0.0477845394804615,-0.0400959894540314));
#56739=DIRECTION('',(0.,-0.766044443118978,-0.642787609686539));
#56740=DIRECTION('',(1.,0.,0.));
#56741=DIRECTION('',(0.755033118392644,0.502285118831863,0.421467257957652));
#56742=DIRECTION('',(-0.755033118392644,0.502285118831863,0.421467257957652));
#56743=DIRECTION('',(-1.,0.,0.));
#56744=DIRECTION('',(0.,-0.766044443118978,-0.642787609686539));
#56745=DIRECTION('',(-0.998052578482888,-0.0477845394804615,-0.0400959894540314));
#56746=DIRECTION('',(-0.957826285221151,0.220121250980087,0.184703660511673));
#56747=DIRECTION('',(-0.868243142124459,0.380064476743201,0.318911962258806));
#56748=DIRECTION('',(-0.948683298050514,0.242244522917128,0.203267289834478));
#56749=DIRECTION('',(-1.,0.,0.));
#56750=DIRECTION('',(-0.948683298050513,-0.242244522917128,-0.203267289834479));
#56751=DIRECTION('',(-0.86824314212446,-0.3800644767432,-0.318911962258805));
#56752=DIRECTION('',(-0.957826285221151,-0.220121250980087,-0.184703660511672));
#56753=DIRECTION('',(-0.998052578482888,0.0477845394804616,0.0400959894540314));
#56754=DIRECTION('',(0.,0.766044443118978,0.642787609686539));
#56755=DIRECTION('',(-1.,0.,0.));
#56756=DIRECTION('',(-0.755033118392644,-0.502285118831863,-0.421467257957652));
#56757=DIRECTION('center_axis',(0.649305557988371,0.483301338560726,0.587215555406037));
#56758=DIRECTION('ref_axis',(0.755033118392643,-0.502285118831863,-0.421467257957652));
#56759=DIRECTION('',(0.,0.772115994122802,-0.6354816217797));
#56760=DIRECTION('',(-0.755033118392644,0.502285118831863,0.421467257957652));
#56761=DIRECTION('center_axis',(-0.649305557988371,-0.483301338560726,-0.587215555406037));
#56762=DIRECTION('ref_axis',(-0.760527640763576,0.412621749021023,0.501339206395651));
#56763=DIRECTION('',(0.0519254248777275,0.742142297230154,-0.66822792587052));
#56764=DIRECTION('center_axis',(0.,0.766044443118978,-0.64278760968654));
#56765=DIRECTION('ref_axis',(1.,0.,0.));
#56766=DIRECTION('',(0.755033118392644,-0.421467257957652,-0.502285118831862));
#56767=DIRECTION('',(1.,0.,0.));
#56768=DIRECTION('',(0.,0.64278760968654,0.766044443118978));
#56769=DIRECTION('',(0.998052578482888,0.0400959894540315,0.0477845394804615));
#56770=DIRECTION('',(0.957826285221151,-0.184703660511672,-0.220121250980087));
#56771=DIRECTION('',(0.86824314212446,-0.318911962258806,-0.3800644767432));
#56772=DIRECTION('',(0.948683298050513,-0.203267289834479,-0.242244522917128));
#56773=DIRECTION('',(1.,0.,0.));
#56774=DIRECTION('',(0.948683298050514,0.203267289834478,0.242244522917128));
#56775=DIRECTION('',(0.86824314212446,0.318911962258806,0.380064476743201));
#56776=DIRECTION('',(0.957826285221151,0.184703660511673,0.220121250980087));
#56777=DIRECTION('',(0.998052578482888,-0.0400959894540314,-0.0477845394804615));
#56778=DIRECTION('',(0.,-0.64278760968654,-0.766044443118978));
#56779=DIRECTION('',(1.,0.,0.));
#56780=DIRECTION('',(0.755033118392644,0.421467257957652,0.502285118831862));
#56781=DIRECTION('',(-0.755033118392644,0.421467257957652,0.502285118831862));
#56782=DIRECTION('',(-1.,0.,0.));
#56783=DIRECTION('',(0.,-0.64278760968654,-0.766044443118978));
#56784=DIRECTION('',(-0.998052578482888,-0.0400959894540314,-0.0477845394804615));
#56785=DIRECTION('',(-0.957826285221151,0.184703660511673,0.220121250980087));
#56786=DIRECTION('',(-0.86824314212446,0.318911962258806,0.380064476743201));
#56787=DIRECTION('',(-0.948683298050514,0.203267289834478,0.242244522917128));
#56788=DIRECTION('',(-1.,0.,0.));
#56789=DIRECTION('',(-0.948683298050513,-0.203267289834479,-0.242244522917128));
#56790=DIRECTION('',(-0.86824314212446,-0.318911962258806,-0.3800644767432));
#56791=DIRECTION('',(-0.957826285221151,-0.184703660511672,-0.220121250980087));
#56792=DIRECTION('',(-0.998052578482888,0.0400959894540315,0.0477845394804615));
#56793=DIRECTION('',(0.,0.64278760968654,0.766044443118978));
#56794=DIRECTION('',(-1.,0.,0.));
#56795=DIRECTION('',(-0.755033118392644,-0.421467257957652,-0.502285118831862));
#56796=DIRECTION('center_axis',(0.649305557988371,0.373989994161849,0.662218828358293));
#56797=DIRECTION('ref_axis',(0.755033118392644,-0.421467257957652,-0.502285118831862));
#56798=DIRECTION('',(0.,0.870736042799734,-0.491750692698506));
#56799=DIRECTION('',(-0.755033118392644,0.421467257957652,0.502285118831862));
#56800=DIRECTION('center_axis',(-0.649305557988371,-0.373989994161849,-0.662218828358293));
#56801=DIRECTION('ref_axis',(-0.760527640763576,0.319296457913771,0.565373752130667));
#56802=DIRECTION('',(0.0519254248777275,0.846904049744114,-0.52920438469299));
#56803=DIRECTION('center_axis',(0.,0.866025403784438,-0.5));
#56804=DIRECTION('ref_axis',(1.,0.,0.));
#56805=DIRECTION('',(0.755033118392644,-0.327843327723122,-0.567841300538901));
#56806=DIRECTION('',(1.,0.,0.));
#56807=DIRECTION('',(0.,0.5,0.866025403784438));
#56808=DIRECTION('',(0.998052578482888,0.0311891430775903,0.0540211804549215));
#56809=DIRECTION('',(0.957826285221151,-0.143673942783173,-0.248850568624199));
#56810=DIRECTION('',(0.86824314212446,-0.248069469178416,-0.429668924423658));
#56811=DIRECTION('',(0.948683298050513,-0.15811388300842,-0.273861278752584));
#56812=DIRECTION('',(1.,0.,0.));
#56813=DIRECTION('',(0.948683298050514,0.158113883008419,0.273861278752584));
#56814=DIRECTION('',(0.86824314212446,0.248069469178417,0.429668924423659));
#56815=DIRECTION('',(0.957826285221151,0.143673942783173,0.248850568624199));
#56816=DIRECTION('',(0.998052578482888,-0.0311891430775903,-0.0540211804549214));
#56817=DIRECTION('',(0.,-0.5,-0.866025403784438));
#56818=DIRECTION('',(1.,0.,0.));
#56819=DIRECTION('',(0.755033118392644,0.327843327723122,0.567841300538901));
#56820=DIRECTION('',(-0.755033118392644,0.327843327723122,0.567841300538901));
#56821=DIRECTION('',(-1.,0.,0.));
#56822=DIRECTION('',(0.,-0.5,-0.866025403784438));
#56823=DIRECTION('',(-0.998052578482888,-0.0311891430775903,-0.0540211804549214));
#56824=DIRECTION('',(-0.957826285221151,0.143673942783173,0.248850568624199));
#56825=DIRECTION('',(-0.86824314212446,0.248069469178417,0.429668924423659));
#56826=DIRECTION('',(-0.948683298050514,0.158113883008419,0.273861278752584));
#56827=DIRECTION('',(-1.,0.,0.));
#56828=DIRECTION('',(-0.948683298050513,-0.15811388300842,-0.273861278752584));
#56829=DIRECTION('',(-0.86824314212446,-0.248069469178416,-0.429668924423658));
#56830=DIRECTION('',(-0.957826285221151,-0.143673942783173,-0.248850568624199));
#56831=DIRECTION('',(-0.998052578482888,0.0311891430775903,0.0540211804549215));
#56832=DIRECTION('',(0.,0.5,0.866025403784438));
#56833=DIRECTION('',(-1.,0.,0.));
#56834=DIRECTION('',(-0.755033118392644,-0.327843327723122,-0.567841300538901));
#56835=DIRECTION('center_axis',(0.649305557988371,0.253315153038432,0.717100917309779));
#56836=DIRECTION('ref_axis',(0.755033118392643,-0.327843327723122,-0.567841300538901));
#56837=DIRECTION('',(0.,0.942899217429894,-0.333078167657524));
#56838=DIRECTION('',(-0.755033118392644,0.327843327723122,0.567841300538901));
#56839=DIRECTION('center_axis',(-0.649305557988371,-0.253315153038432,-0.717100917309779));
#56840=DIRECTION('ref_axis',(-0.760527640763576,0.216269505504613,0.612229702500115));
#56841=DIRECTION('',(0.0519254248777275,0.925933051260727,-0.374101236076903));
#56842=DIRECTION('center_axis',(0.,0.939692620785908,-0.342020143325669));
#56843=DIRECTION('ref_axis',(1.,0.,0.));
#56844=DIRECTION('',(0.755033118392644,-0.224258043872453,-0.616143911670627));
#56845=DIRECTION('',(1.,0.,0.));
#56846=DIRECTION('',(0.,0.342020143325669,0.939692620785908));
#56847=DIRECTION('',(0.998052578482888,0.0213346303712045,0.0586164151972949));
#56848=DIRECTION('',(0.957826285221151,-0.0982787650057295,-0.270018687665128));
#56849=DIRECTION('',(0.86824314212446,-0.169689510806249,-0.46621809925847));
#56850=DIRECTION('',(0.948683298050513,-0.108156265856636,-0.297156898213637));
#56851=DIRECTION('',(1.,0.,0.));
#56852=DIRECTION('',(0.948683298050514,0.108156265856635,0.297156898213636));
#56853=DIRECTION('',(0.868243142124459,0.16968951080625,0.466218099258471));
#56854=DIRECTION('',(0.957826285221151,0.0982787650057297,0.270018687665129));
#56855=DIRECTION('',(0.998052578482888,-0.0213346303712045,-0.0586164151972949));
#56856=DIRECTION('',(0.,-0.342020143325669,-0.939692620785908));
#56857=DIRECTION('',(1.,0.,0.));
#56858=DIRECTION('',(0.755033118392644,0.224258043872453,0.616143911670627));
#56859=DIRECTION('',(-0.755033118392644,0.224258043872453,0.616143911670627));
#56860=DIRECTION('',(-1.,0.,0.));
#56861=DIRECTION('',(0.,-0.342020143325669,-0.939692620785908));
#56862=DIRECTION('',(-0.998052578482888,-0.0213346303712045,-0.0586164151972949));
#56863=DIRECTION('',(-0.957826285221151,0.0982787650057297,0.270018687665129));
#56864=DIRECTION('',(-0.868243142124459,0.16968951080625,0.466218099258471));
#56865=DIRECTION('',(-0.948683298050514,0.108156265856635,0.297156898213636));
#56866=DIRECTION('',(-1.,0.,0.));
#56867=DIRECTION('',(-0.948683298050513,-0.108156265856636,-0.297156898213637));
#56868=DIRECTION('',(-0.86824314212446,-0.169689510806249,-0.46621809925847));
#56869=DIRECTION('',(-0.957826285221151,-0.0982787650057295,-0.270018687665128));
#56870=DIRECTION('',(-0.998052578482888,0.0213346303712045,0.0586164151972949));
#56871=DIRECTION('',(0.,0.342020143325669,0.939692620785908));
#56872=DIRECTION('',(-1.,0.,0.));
#56873=DIRECTION('',(-0.755033118392644,-0.224258043872453,-0.616143911670627));
#56874=DIRECTION('center_axis',(0.649305557988371,0.124943459173594,0.75019425775938));
#56875=DIRECTION('ref_axis',(0.755033118392643,-0.224258043872453,-0.616143911670627));
#56876=DIRECTION('',(0.,0.986412876468473,-0.164285231037954));
#56877=DIRECTION('',(-0.755033118392644,0.224258043872453,0.616143911670627));
#56878=DIRECTION('center_axis',(-0.649305557988371,-0.124943459173594,-0.75019425775938));
#56879=DIRECTION('ref_axis',(-0.760527640763576,0.106671313608347,0.640483363162275));
#56880=DIRECTION('',(0.0519254248777275,0.976828045559515,-0.207631210706979));
#56881=DIRECTION('center_axis',(0.,0.984807753012208,-0.17364817766693));
#56882=DIRECTION('ref_axis',(1.,0.,0.));
#56883=DIRECTION('',(0.755033118392643,-0.113858792838765,-0.645725301830105));
#56884=DIRECTION('',(1.,0.,0.));
#56885=DIRECTION('',(0.,0.17364817766693,0.984807753012208));
#56886=DIRECTION('',(0.998052578482888,0.0108318757168334,0.0614306198252359));
#56887=DIRECTION('',(0.957826285221151,-0.0498974366850415,-0.282982425517402));
#56888=DIRECTION('',(0.86824314212446,-0.0861536225152694,-0.488601473065054));
#56889=DIRECTION('',(0.948683298050513,-0.0549123752965087,-0.311423555691114));
#56890=DIRECTION('',(1.,0.,0.));
#56891=DIRECTION('',(0.948683298050514,0.0549123752965085,0.311423555691113));
#56892=DIRECTION('',(0.868243142124459,0.0861536225152696,0.488601473065055));
#56893=DIRECTION('',(0.957826285221151,0.0498974366850416,0.282982425517402));
#56894=DIRECTION('',(0.998052578482888,-0.0108318757168334,-0.0614306198252359));
#56895=DIRECTION('',(0.,-0.17364817766693,-0.984807753012208));
#56896=DIRECTION('',(1.,0.,0.));
#56897=DIRECTION('',(0.755033118392644,0.113858792838765,0.645725301830104));
#56898=DIRECTION('',(-0.755033118392644,0.113858792838765,0.645725301830104));
#56899=DIRECTION('',(-1.,0.,0.));
#56900=DIRECTION('',(0.,-0.17364817766693,-0.984807753012208));
#56901=DIRECTION('',(-0.998052578482888,-0.0108318757168334,-0.0614306198252359));
#56902=DIRECTION('',(-0.957826285221151,0.0498974366850416,0.282982425517402));
#56903=DIRECTION('',(-0.868243142124459,0.0861536225152696,0.488601473065055));
#56904=DIRECTION('',(-0.948683298050514,0.0549123752965085,0.311423555691113));
#56905=DIRECTION('',(-1.,0.,0.));
#56906=DIRECTION('',(-0.948683298050513,-0.0549123752965087,-0.311423555691114));
#56907=DIRECTION('',(-0.86824314212446,-0.0861536225152694,-0.488601473065054));
#56908=DIRECTION('',(-0.957826285221151,-0.0498974366850415,-0.282982425517402));
#56909=DIRECTION('',(-0.998052578482888,0.0108318757168334,0.0614306198252359));
#56910=DIRECTION('',(0.,0.17364817766693,0.984807753012208));
#56911=DIRECTION('',(-1.,0.,0.));
#56912=DIRECTION('',(-0.755033118392643,-0.113858792838765,-0.645725301830105));
#56913=DIRECTION('center_axis',(0.649305557988371,-0.00722457847379224,
0.760493325303573));
#56914=DIRECTION('ref_axis',(0.755033118392643,-0.113858792838765,-0.645725301830105));
#56915=DIRECTION('',(0.,0.999954879404557,0.00949942919436656));
#56916=DIRECTION('',(-0.755033118392643,0.113858792838765,0.645725301830105));
#56917=DIRECTION('center_axis',(-0.649305557988371,0.00722457847379224,
-0.760493325303573));
#56918=DIRECTION('ref_axis',(0.760527640763576,0.00616803217361924,-0.64927626093497));
#56919=DIRECTION('',(0.0519254248777275,0.998042613992818,-0.0348524160661844));
#56920=DIRECTION('center_axis',(-1.,0.,0.));
#56921=DIRECTION('ref_axis',(0.,1.,0.));
#56922=DIRECTION('center_axis',(1.,0.,0.));
#56923=DIRECTION('ref_axis',(0.,1.,0.));
#56924=DIRECTION('center_axis',(-1.,0.,0.));
#56925=DIRECTION('ref_axis',(0.,1.,0.));
#56926=DIRECTION('center_axis',(1.,0.,0.));
#56927=DIRECTION('ref_axis',(0.,1.,0.));
#56928=DIRECTION('center_axis',(-1.,0.,0.));
#56929=DIRECTION('ref_axis',(0.,1.,0.));
#56930=DIRECTION('center_axis',(1.,0.,0.));
#56931=DIRECTION('ref_axis',(0.,1.,0.));
#56932=DIRECTION('center_axis',(-1.,0.,0.));
#56933=DIRECTION('ref_axis',(0.,1.,0.));
#56934=DIRECTION('center_axis',(1.,0.,0.));
#56935=DIRECTION('ref_axis',(0.,1.,0.));
#56936=DIRECTION('center_axis',(-1.,0.,0.));
#56937=DIRECTION('ref_axis',(0.,1.,0.));
#56938=DIRECTION('center_axis',(1.,0.,0.));
#56939=DIRECTION('ref_axis',(0.,1.,0.));
#56940=DIRECTION('center_axis',(-1.,0.,0.));
#56941=DIRECTION('ref_axis',(0.,1.,0.));
#56942=DIRECTION('center_axis',(1.,0.,0.));
#56943=DIRECTION('ref_axis',(0.,1.,0.));
#56944=DIRECTION('center_axis',(-1.,0.,0.));
#56945=DIRECTION('ref_axis',(0.,1.,0.));
#56946=DIRECTION('center_axis',(1.,0.,0.));
#56947=DIRECTION('ref_axis',(0.,1.,0.));
#56948=DIRECTION('center_axis',(-1.,0.,0.));
#56949=DIRECTION('ref_axis',(0.,1.,0.));
#56950=DIRECTION('center_axis',(1.,0.,0.));
#56951=DIRECTION('ref_axis',(0.,1.,0.));
#56952=DIRECTION('center_axis',(-1.,0.,0.));
#56953=DIRECTION('ref_axis',(0.,1.,0.));
#56954=DIRECTION('center_axis',(1.,0.,0.));
#56955=DIRECTION('ref_axis',(0.,1.,0.));
#56956=DIRECTION('center_axis',(-1.,0.,0.));
#56957=DIRECTION('ref_axis',(0.,1.,0.));
#56958=DIRECTION('center_axis',(1.,0.,0.));
#56959=DIRECTION('ref_axis',(0.,1.,0.));
#56960=DIRECTION('center_axis',(-1.,0.,0.));
#56961=DIRECTION('ref_axis',(0.,1.,0.));
#56962=DIRECTION('center_axis',(1.,0.,0.));
#56963=DIRECTION('ref_axis',(0.,1.,0.));
#56964=DIRECTION('center_axis',(-1.,0.,0.));
#56965=DIRECTION('ref_axis',(0.,1.,0.));
#56966=DIRECTION('center_axis',(1.,0.,0.));
#56967=DIRECTION('ref_axis',(0.,1.,0.));
#56968=DIRECTION('center_axis',(-1.,0.,0.));
#56969=DIRECTION('ref_axis',(0.,1.,0.));
#56970=DIRECTION('center_axis',(1.,0.,0.));
#56971=DIRECTION('ref_axis',(0.,1.,0.));
#56972=DIRECTION('center_axis',(-1.,0.,0.));
#56973=DIRECTION('ref_axis',(0.,1.,0.));
#56974=DIRECTION('center_axis',(1.,0.,0.));
#56975=DIRECTION('ref_axis',(0.,1.,0.));
#56976=DIRECTION('center_axis',(-1.,0.,0.));
#56977=DIRECTION('ref_axis',(0.,1.,0.));
#56978=DIRECTION('center_axis',(1.,0.,0.));
#56979=DIRECTION('ref_axis',(0.,1.,0.));
#56980=DIRECTION('center_axis',(-1.,0.,0.));
#56981=DIRECTION('ref_axis',(0.,1.,0.));
#56982=DIRECTION('center_axis',(1.,0.,0.));
#56983=DIRECTION('ref_axis',(0.,1.,0.));
#56984=DIRECTION('center_axis',(-1.,0.,0.));
#56985=DIRECTION('ref_axis',(0.,1.,0.));
#56986=DIRECTION('center_axis',(1.,0.,0.));
#56987=DIRECTION('ref_axis',(0.,1.,0.));
#56988=DIRECTION('center_axis',(-1.,0.,0.));
#56989=DIRECTION('ref_axis',(0.,-1.,5.66553889764798E-16));
#56990=DIRECTION('center_axis',(1.,0.,0.));
#56991=DIRECTION('ref_axis',(0.,1.,0.));
#56992=DIRECTION('center_axis',(-1.,0.,0.));
#56993=DIRECTION('ref_axis',(0.,1.,0.));
#56994=DIRECTION('center_axis',(1.,0.,0.));
#56995=DIRECTION('ref_axis',(0.,1.,0.));
#56996=DIRECTION('center_axis',(-1.,0.,0.));
#56997=DIRECTION('ref_axis',(0.,1.,0.));
#56998=DIRECTION('center_axis',(1.,0.,0.));
#56999=DIRECTION('ref_axis',(0.,1.,0.));
#57000=DIRECTION('center_axis',(-1.,0.,0.));
#57001=DIRECTION('ref_axis',(0.,1.,0.));
#57002=DIRECTION('center_axis',(1.,0.,0.));
#57003=DIRECTION('ref_axis',(0.,1.,0.));
#57004=DIRECTION('center_axis',(-1.,0.,0.));
#57005=DIRECTION('ref_axis',(0.,1.,0.));
#57006=DIRECTION('center_axis',(1.,0.,0.));
#57007=DIRECTION('ref_axis',(0.,1.,0.));
#57008=DIRECTION('center_axis',(-1.,0.,0.));
#57009=DIRECTION('ref_axis',(0.,1.,0.));
#57010=DIRECTION('center_axis',(1.,0.,0.));
#57011=DIRECTION('ref_axis',(0.,1.,0.));
#57012=DIRECTION('center_axis',(-1.,0.,0.));
#57013=DIRECTION('ref_axis',(0.,1.,0.));
#57014=DIRECTION('center_axis',(1.,0.,0.));
#57015=DIRECTION('ref_axis',(0.,1.,0.));
#57016=DIRECTION('center_axis',(-1.,0.,0.));
#57017=DIRECTION('ref_axis',(0.,1.,0.));
#57018=DIRECTION('center_axis',(1.,0.,0.));
#57019=DIRECTION('ref_axis',(0.,1.,0.));
#57020=DIRECTION('center_axis',(-1.,0.,0.));
#57021=DIRECTION('ref_axis',(0.,1.,0.));
#57022=DIRECTION('center_axis',(1.,0.,0.));
#57023=DIRECTION('ref_axis',(0.,1.,0.));
#57024=DIRECTION('center_axis',(-1.,0.,0.));
#57025=DIRECTION('ref_axis',(0.,1.,0.));
#57026=DIRECTION('center_axis',(1.,0.,0.));
#57027=DIRECTION('ref_axis',(0.,1.,0.));
#57028=DIRECTION('center_axis',(-1.,0.,0.));
#57029=DIRECTION('ref_axis',(0.,1.,0.));
#57030=DIRECTION('center_axis',(1.,0.,0.));
#57031=DIRECTION('ref_axis',(0.,1.,0.));
#57032=DIRECTION('center_axis',(-1.,0.,0.));
#57033=DIRECTION('ref_axis',(0.,1.,0.));
#57034=DIRECTION('center_axis',(1.,0.,0.));
#57035=DIRECTION('ref_axis',(0.,1.,0.));
#57036=DIRECTION('center_axis',(-1.,0.,0.));
#57037=DIRECTION('ref_axis',(0.,1.,0.));
#57038=DIRECTION('center_axis',(1.,0.,0.));
#57039=DIRECTION('ref_axis',(0.,1.,0.));
#57040=DIRECTION('center_axis',(-1.,0.,0.));
#57041=DIRECTION('ref_axis',(0.,1.,0.));
#57042=DIRECTION('center_axis',(1.,0.,0.));
#57043=DIRECTION('ref_axis',(0.,1.,0.));
#57044=DIRECTION('center_axis',(-1.,0.,0.));
#57045=DIRECTION('ref_axis',(0.,1.,0.));
#57046=DIRECTION('center_axis',(1.,0.,0.));
#57047=DIRECTION('ref_axis',(0.,1.,0.));
#57048=DIRECTION('center_axis',(-1.,0.,0.));
#57049=DIRECTION('ref_axis',(0.,1.,0.));
#57050=DIRECTION('center_axis',(1.,0.,0.));
#57051=DIRECTION('ref_axis',(0.,1.,0.));
#57052=DIRECTION('center_axis',(-1.,0.,0.));
#57053=DIRECTION('ref_axis',(0.,1.,0.));
#57054=DIRECTION('center_axis',(1.,0.,0.));
#57055=DIRECTION('ref_axis',(0.,1.,0.));
#57056=DIRECTION('center_axis',(-1.,0.,0.));
#57057=DIRECTION('ref_axis',(0.,1.,0.));
#57058=DIRECTION('center_axis',(1.,0.,0.));
#57059=DIRECTION('ref_axis',(0.,1.,0.));
#57060=DIRECTION('center_axis',(-1.,0.,0.));
#57061=DIRECTION('ref_axis',(0.,1.,0.));
#57062=DIRECTION('center_axis',(1.,0.,0.));
#57063=DIRECTION('ref_axis',(0.,1.,0.));
#57064=DIRECTION('center_axis',(-0.649305557988371,-0.139173100960066,-0.747685187986609));
#57065=DIRECTION('ref_axis',(-0.755033118392644,0.,0.655686655446243));
#57066=DIRECTION('',(0.,0.983113759331517,-0.182995454077559));
#57067=DIRECTION('',(0.755033118392644,0.,-0.655686655446243));
#57068=DIRECTION('center_axis',(0.649305557988371,0.139173100960066,0.747685187986609));
#57069=DIRECTION('ref_axis',(-0.760527640763576,0.118819965419165,0.638341228068795));
#57070=DIRECTION('',(-0.0519254248777281,0.98893216263388,-0.138985351600607));
#57071=DIRECTION('center_axis',(-0.649305557988371,-0.00722457847379249,
-0.760493325303573));
#57072=DIRECTION('ref_axis',(-0.755033118392644,-0.113858792838765,0.645725301830105));
#57073=DIRECTION('',(0.,0.999954879404557,-0.00949942919436689));
#57074=DIRECTION('',(0.755033118392644,0.113858792838765,-0.645725301830105));
#57075=DIRECTION('center_axis',(0.649305557988371,0.00722457847379249,0.760493325303573));
#57076=DIRECTION('ref_axis',(-0.760527640763576,0.00616803217361938,0.649276260934969));
#57077=DIRECTION('',(-0.0519254248777281,0.998042613992818,0.0348524160661846));
#57078=DIRECTION('center_axis',(-0.649305557988371,0.124943459173594,-0.75019425775938));
#57079=DIRECTION('ref_axis',(-0.755033118392644,-0.224258043872452,0.616143911670627));
#57080=DIRECTION('',(0.,0.986412876468473,0.164285231037953));
#57081=DIRECTION('',(0.755033118392644,0.224258043872452,-0.616143911670627));
#57082=DIRECTION('center_axis',(0.649305557988371,-0.124943459173594,0.75019425775938));
#57083=DIRECTION('ref_axis',(0.760527640763576,0.106671313608347,-0.640483363162275));
#57084=DIRECTION('',(-0.0519254248777281,0.976828045559515,0.207631210706978));
#57085=DIRECTION('center_axis',(-0.649305557988371,0.253315153038431,-0.717100917309779));
#57086=DIRECTION('ref_axis',(-0.755033118392644,-0.327843327723121,0.567841300538901));
#57087=DIRECTION('',(0.,0.942899217429894,0.333078167657523));
#57088=DIRECTION('',(0.755033118392644,0.327843327723121,-0.567841300538901));
#57089=DIRECTION('center_axis',(0.649305557988371,-0.253315153038431,0.717100917309779));
#57090=DIRECTION('ref_axis',(0.760527640763576,0.216269505504612,-0.612229702500115));
#57091=DIRECTION('',(-0.0519254248777281,0.925933051260728,0.374101236076903));
#57092=DIRECTION('center_axis',(-0.649305557988371,0.373989994161848,-0.662218828358294));
#57093=DIRECTION('ref_axis',(-0.755033118392644,-0.421467257957652,0.502285118831862));
#57094=DIRECTION('',(0.,0.870736042799734,0.491750692698505));
#57095=DIRECTION('',(0.755033118392644,0.421467257957652,-0.502285118831862));
#57096=DIRECTION('center_axis',(0.649305557988371,-0.373989994161848,0.662218828358294));
#57097=DIRECTION('ref_axis',(0.760527640763576,0.31929645791377,-0.565373752130667));
#57098=DIRECTION('',(-0.0519254248777281,0.846904049744115,0.52920438469299));
#57099=DIRECTION('center_axis',(-0.649305557988371,0.483301338560726,-0.587215555406038));
#57100=DIRECTION('ref_axis',(-0.755033118392644,-0.502285118831862,0.421467257957652));
#57101=DIRECTION('',(0.,0.772115994122802,0.6354816217797));
#57102=DIRECTION('',(0.755033118392644,0.502285118831862,-0.421467257957652));
#57103=DIRECTION('center_axis',(0.649305557988371,-0.483301338560726,0.587215555406038));
#57104=DIRECTION('ref_axis',(0.760527640763576,0.412621749021022,-0.501339206395651));
#57105=DIRECTION('',(-0.0519254248777281,0.742142297230154,0.66822792587052));
#57106=DIRECTION('center_axis',(-0.649305557988371,0.577927816349714,-0.494370034948178));
#57107=DIRECTION('ref_axis',(-0.755033118392644,-0.567841300538901,0.327843327723122));
#57108=DIRECTION('',(0.,0.650035591673994,0.759903763352335));
#57109=DIRECTION('',(0.755033118392644,0.567841300538901,-0.327843327723122));
#57110=DIRECTION('center_axis',(0.649305557988371,-0.577927816349714,0.494370034948178));
#57111=DIRECTION('ref_axis',(0.760527640763576,0.49340973708095,-0.422071722564183));
#57112=DIRECTION('',(-0.0519254248777281,0.614830926556978,0.786947699660121));
#57113=DIRECTION('center_axis',(-0.649305557988371,0.654994249884502,-0.386503331141725));
#57114=DIRECTION('ref_axis',(-0.755033118392644,-0.616143911670627,0.224258043872453));
#57115=DIRECTION('',(0.,0.508204186706052,0.861236613605367));
#57116=DIRECTION('',(0.755033118392644,0.616143911670627,-0.224258043872453));
#57117=DIRECTION('center_axis',(0.649305557988371,-0.654994249884502,0.386503331141725));
#57118=DIRECTION('ref_axis',(0.760527640763576,0.559205719957048,-0.329979803021199));
#57119=DIRECTION('',(-0.0519254248777281,0.468838229299828,0.881756465810299));
#57120=DIRECTION('center_axis',(-0.649305557988371,0.712159014579631,-0.266892919198654));
#57121=DIRECTION('ref_axis',(-0.755033118392644,-0.645725301830105,0.113858792838765));
#57122=DIRECTION('',(0.,0.350931254688773,0.936401225160755));
#57123=DIRECTION('',(0.755033118392644,0.645725301830105,-0.113858792838765));
#57124=DIRECTION('center_axis',(0.649305557988371,-0.712159014579631,0.266892919198654));
#57125=DIRECTION('ref_axis',(0.760527640763576,0.608010520003998,-0.227861614141253));
#57126=DIRECTION('',(-0.0519254248777281,0.308600119688995,0.949773507937132));
#57127=DIRECTION('center_axis',(-0.649305557988371,0.747685187986609,-0.139173100960066));
#57128=DIRECTION('ref_axis',(-0.755033118392644,-0.655686655446243,4.01492281917938E-17));
#57129=DIRECTION('',(0.,0.182995454077559,0.983113759331517));
#57130=DIRECTION('',(0.755033118392644,0.655686655446243,-4.01492281917938E-17));
#57131=DIRECTION('center_axis',(0.649305557988371,-0.747685187986609,0.139173100960066));
#57132=DIRECTION('ref_axis',(0.760527640763576,0.638341228068795,-0.118819965419165));
#57133=DIRECTION('',(-0.0519254248777281,0.138985351600607,0.98893216263388));
#57134=DIRECTION('center_axis',(-0.649305557988371,0.760493325303573,-0.00722457847379251));
#57135=DIRECTION('ref_axis',(-0.755033118392644,-0.645725301830105,-0.113858792838765));
#57136=DIRECTION('',(0.,0.00949942919436693,0.999954879404557));
#57137=DIRECTION('',(0.755033118392644,0.645725301830105,0.113858792838765));
#57138=DIRECTION('center_axis',(0.649305557988371,-0.760493325303573,0.00722457847379251));
#57139=DIRECTION('ref_axis',(0.760527640763576,0.649276260934969,-0.00616803217361943));
#57140=DIRECTION('',(-0.0519254248777281,-0.0348524160661846,0.998042613992818));
#57141=DIRECTION('center_axis',(-0.649305557988371,0.75019425775938,0.124943459173594));
#57142=DIRECTION('ref_axis',(-0.755033118392644,-0.616143911670627,-0.224258043872452));
#57143=DIRECTION('',(0.,-0.164285231037953,0.986412876468473));
#57144=DIRECTION('',(0.755033118392644,0.616143911670627,0.224258043872452));
#57145=DIRECTION('center_axis',(0.649305557988371,-0.75019425775938,-0.124943459173594));
#57146=DIRECTION('ref_axis',(0.760527640763576,0.640483363162275,0.106671313608347));
#57147=DIRECTION('',(-0.0519254248777281,-0.207631210706978,0.976828045559515));
#57148=DIRECTION('center_axis',(-0.649305557988371,0.717100917309779,0.253315153038431));
#57149=DIRECTION('ref_axis',(-0.755033118392644,-0.567841300538901,-0.327843327723121));
#57150=DIRECTION('',(0.,-0.333078167657523,0.942899217429894));
#57151=DIRECTION('',(0.755033118392644,0.567841300538901,0.327843327723121));
#57152=DIRECTION('center_axis',(0.649305557988371,-0.717100917309779,-0.253315153038431));
#57153=DIRECTION('ref_axis',(0.760527640763576,0.612229702500115,0.216269505504612));
#57154=DIRECTION('',(-0.0519254248777281,-0.374101236076902,0.925933051260728));
#57155=DIRECTION('center_axis',(-0.649305557988371,0.662218828358294,0.373989994161848));
#57156=DIRECTION('ref_axis',(-0.755033118392644,-0.502285118831862,-0.421467257957652));
#57157=DIRECTION('',(0.,-0.491750692698505,0.870736042799734));
#57158=DIRECTION('',(0.755033118392644,0.502285118831862,0.421467257957652));
#57159=DIRECTION('center_axis',(0.649305557988371,-0.662218828358294,-0.373989994161848));
#57160=DIRECTION('ref_axis',(0.760527640763576,0.565373752130667,0.31929645791377));
#57161=DIRECTION('',(-0.0519254248777281,-0.52920438469299,0.846904049744114));
#57162=DIRECTION('center_axis',(-0.649305557988371,0.587215555406038,0.483301338560726));
#57163=DIRECTION('ref_axis',(-0.755033118392644,-0.421467257957652,-0.502285118831862));
#57164=DIRECTION('',(0.,-0.6354816217797,0.772115994122802));
#57165=DIRECTION('',(0.755033118392644,0.421467257957652,0.502285118831862));
#57166=DIRECTION('center_axis',(0.649305557988371,-0.587215555406038,-0.483301338560726));
#57167=DIRECTION('ref_axis',(0.760527640763576,0.501339206395651,0.412621749021022));
#57168=DIRECTION('',(-0.0519254248777281,-0.66822792587052,0.742142297230154));
#57169=DIRECTION('center_axis',(-0.649305557988371,0.494370034948177,0.577927816349714));
#57170=DIRECTION('ref_axis',(-0.755033118392644,-0.327843327723121,-0.567841300538901));
#57171=DIRECTION('',(0.,-0.759903763352335,0.650035591673993));
#57172=DIRECTION('',(0.755033118392644,0.327843327723121,0.567841300538901));
#57173=DIRECTION('center_axis',(0.649305557988371,-0.494370034948177,-0.577927816349714));
#57174=DIRECTION('ref_axis',(0.760527640763576,0.422071722564183,0.49340973708095));
#57175=DIRECTION('',(-0.0519254248777281,-0.786947699660121,0.614830926556977));
#57176=DIRECTION('center_axis',(-0.649305557988371,0.386503331141725,0.654994249884501));
#57177=DIRECTION('ref_axis',(-0.755033118392644,-0.224258043872452,-0.616143911670627));
#57178=DIRECTION('',(0.,-0.861236613605367,0.508204186706052));
#57179=DIRECTION('',(0.755033118392644,0.224258043872452,0.616143911670627));
#57180=DIRECTION('center_axis',(0.649305557988371,-0.386503331141725,-0.654994249884501));
#57181=DIRECTION('ref_axis',(0.760527640763576,0.329979803021199,0.559205719957048));
#57182=DIRECTION('',(-0.0519254248777281,-0.881756465810299,0.468838229299828));
#57183=DIRECTION('center_axis',(-0.649305557988371,0.266892919198654,0.712159014579631));
#57184=DIRECTION('ref_axis',(-0.755033118392644,-0.113858792838765,-0.645725301830104));
#57185=DIRECTION('',(0.,-0.936401225160755,0.350931254688773));
#57186=DIRECTION('',(0.755033118392644,0.113858792838765,0.645725301830104));
#57187=DIRECTION('center_axis',(0.649305557988371,-0.266892919198654,-0.712159014579631));
#57188=DIRECTION('ref_axis',(0.760527640763576,0.227861614141253,0.608010520003998));
#57189=DIRECTION('',(-0.0519254248777281,-0.949773507937132,0.308600119688995));
#57190=DIRECTION('center_axis',(-0.649305557988371,0.139173100960066,0.747685187986609));
#57191=DIRECTION('ref_axis',(-0.755033118392644,-8.02984563835875E-17,-0.655686655446243));
#57192=DIRECTION('',(0.,-0.983113759331517,0.182995454077559));
#57193=DIRECTION('',(0.755033118392644,8.02984563835875E-17,0.655686655446243));
#57194=DIRECTION('center_axis',(0.649305557988371,-0.139173100960066,-0.747685187986609));
#57195=DIRECTION('ref_axis',(0.760527640763576,0.118819965419165,0.638341228068795));
#57196=DIRECTION('',(-0.0519254248777281,-0.98893216263388,0.138985351600607));
#57197=DIRECTION('center_axis',(-0.649305557988371,0.00722457847379274,
0.760493325303573));
#57198=DIRECTION('ref_axis',(-0.755033118392644,0.113858792838764,-0.645725301830105));
#57199=DIRECTION('',(0.,-0.999954879404557,0.00949942919436722));
#57200=DIRECTION('',(0.755033118392644,-0.113858792838764,0.645725301830105));
#57201=DIRECTION('center_axis',(0.649305557988371,-0.00722457847379274,
-0.760493325303573));
#57202=DIRECTION('ref_axis',(0.760527640763576,0.00616803217361967,0.64927626093497));
#57203=DIRECTION('',(-0.0519254248777282,-0.998042613992818,-0.0348524160661843));
#57204=DIRECTION('center_axis',(-0.649305557988371,-0.124943459173594,0.75019425775938));
#57205=DIRECTION('ref_axis',(-0.755033118392644,0.224258043872452,-0.616143911670627));
#57206=DIRECTION('',(0.,-0.986412876468473,-0.164285231037953));
#57207=DIRECTION('',(0.755033118392644,-0.224258043872452,0.616143911670627));
#57208=DIRECTION('center_axis',(0.649305557988371,0.124943459173594,-0.75019425775938));
#57209=DIRECTION('ref_axis',(-0.760527640763576,0.106671313608347,-0.640483363162275));
#57210=DIRECTION('',(-0.0519254248777281,-0.976828045559515,-0.207631210706978));
#57211=DIRECTION('center_axis',(-0.649305557988371,-0.253315153038431,0.717100917309779));
#57212=DIRECTION('ref_axis',(-0.755033118392644,0.327843327723121,-0.567841300538901));
#57213=DIRECTION('',(0.,-0.942899217429894,-0.333078167657523));
#57214=DIRECTION('',(0.755033118392644,-0.327843327723121,0.567841300538901));
#57215=DIRECTION('center_axis',(0.649305557988371,0.253315153038431,-0.717100917309779));
#57216=DIRECTION('ref_axis',(-0.760527640763576,0.216269505504612,-0.612229702500115));
#57217=DIRECTION('',(-0.0519254248777281,-0.925933051260728,-0.374101236076902));
#57218=DIRECTION('center_axis',(-0.649305557988371,-0.373989994161848,0.662218828358294));
#57219=DIRECTION('ref_axis',(-0.755033118392644,0.421467257957652,-0.502285118831862));
#57220=DIRECTION('',(0.,-0.870736042799734,-0.491750692698505));
#57221=DIRECTION('',(0.755033118392644,-0.421467257957652,0.502285118831862));
#57222=DIRECTION('center_axis',(0.649305557988371,0.373989994161848,-0.662218828358294));
#57223=DIRECTION('ref_axis',(-0.760527640763576,0.31929645791377,-0.565373752130667));
#57224=DIRECTION('',(-0.0519254248777281,-0.846904049744115,-0.52920438469299));
#57225=DIRECTION('center_axis',(-0.649305557988371,-0.483301338560726,0.587215555406038));
#57226=DIRECTION('ref_axis',(-0.755033118392644,0.502285118831862,-0.421467257957652));
#57227=DIRECTION('',(0.,-0.772115994122802,-0.6354816217797));
#57228=DIRECTION('',(0.755033118392644,-0.502285118831862,0.421467257957652));
#57229=DIRECTION('center_axis',(0.649305557988371,0.483301338560726,-0.587215555406038));
#57230=DIRECTION('ref_axis',(-0.760527640763576,0.412621749021022,-0.501339206395651));
#57231=DIRECTION('',(-0.0519254248777281,-0.742142297230154,-0.66822792587052));
#57232=DIRECTION('center_axis',(-0.649305557988371,-0.577927816349714,0.494370034948178));
#57233=DIRECTION('ref_axis',(-0.755033118392644,0.567841300538901,-0.327843327723122));
#57234=DIRECTION('',(0.,-0.650035591673994,-0.759903763352334));
#57235=DIRECTION('',(0.755033118392644,-0.567841300538901,0.327843327723122));
#57236=DIRECTION('center_axis',(0.649305557988371,0.577927816349714,-0.494370034948178));
#57237=DIRECTION('ref_axis',(-0.760527640763576,0.49340973708095,-0.422071722564183));
#57238=DIRECTION('',(-0.0519254248777281,-0.614830926556978,-0.786947699660121));
#57239=DIRECTION('center_axis',(-0.649305557988371,-0.654994249884501,0.386503331141726));
#57240=DIRECTION('ref_axis',(-0.755033118392644,0.616143911670627,-0.224258043872453));
#57241=DIRECTION('',(0.,-0.508204186706052,-0.861236613605367));
#57242=DIRECTION('',(0.755033118392644,-0.616143911670627,0.224258043872453));
#57243=DIRECTION('center_axis',(0.649305557988371,0.654994249884501,-0.386503331141726));
#57244=DIRECTION('ref_axis',(-0.760527640763576,0.559205719957047,-0.329979803021199));
#57245=DIRECTION('',(-0.0519254248777281,-0.468838229299829,-0.881756465810299));
#57246=DIRECTION('center_axis',(-0.649305557988371,-0.712159014579631,0.266892919198654));
#57247=DIRECTION('ref_axis',(-0.755033118392644,0.645725301830105,-0.113858792838765));
#57248=DIRECTION('',(0.,-0.350931254688773,-0.936401225160755));
#57249=DIRECTION('',(0.755033118392644,-0.645725301830105,0.113858792838765));
#57250=DIRECTION('center_axis',(0.649305557988371,0.712159014579631,-0.266892919198654));
#57251=DIRECTION('ref_axis',(-0.760527640763576,0.608010520003998,-0.227861614141253));
#57252=DIRECTION('',(-0.0519254248777281,-0.308600119688995,-0.949773507937132));
#57253=DIRECTION('center_axis',(-0.649305557988371,-0.747685187986609,0.139173100960066));
#57254=DIRECTION('ref_axis',(-0.755033118392644,0.655686655446243,-1.20447684575381E-16));
#57255=DIRECTION('',(0.,-0.18299545407756,-0.983113759331517));
#57256=DIRECTION('',(0.755033118392644,-0.655686655446243,1.20447684575381E-16));
#57257=DIRECTION('center_axis',(0.649305557988371,0.747685187986609,-0.139173100960066));
#57258=DIRECTION('ref_axis',(-0.760527640763576,0.638341228068795,-0.118819965419165));
#57259=DIRECTION('',(-0.0519254248777281,-0.138985351600607,-0.98893216263388));
#57260=DIRECTION('center_axis',(-0.649305557988371,-0.760493325303573,0.00722457847379279));
#57261=DIRECTION('ref_axis',(-0.755033118392644,0.645725301830105,0.113858792838764));
#57262=DIRECTION('',(0.,-0.00949942919436729,-0.999954879404557));
#57263=DIRECTION('',(0.755033118392644,-0.645725301830105,-0.113858792838764));
#57264=DIRECTION('center_axis',(0.649305557988371,0.760493325303573,-0.00722457847379279));
#57265=DIRECTION('ref_axis',(-0.760527640763576,0.649276260934969,-0.00616803217361967));
#57266=DIRECTION('',(-0.0519254248777282,0.0348524160661842,-0.998042613992818));
#57267=DIRECTION('center_axis',(-0.649305557988371,-0.75019425775938,-0.124943459173593));
#57268=DIRECTION('ref_axis',(-0.755033118392644,0.616143911670627,0.224258043872452));
#57269=DIRECTION('',(0.,0.164285231037953,-0.986412876468473));
#57270=DIRECTION('',(0.755033118392644,-0.616143911670627,-0.224258043872452));
#57271=DIRECTION('center_axis',(0.649305557988371,0.75019425775938,0.124943459173593));
#57272=DIRECTION('ref_axis',(-0.760527640763576,0.640483363162275,0.106671313608346));
#57273=DIRECTION('',(-0.0519254248777281,0.207631210706978,-0.976828045559515));
#57274=DIRECTION('center_axis',(-0.649305557988371,-0.717100917309779,-0.253315153038431));
#57275=DIRECTION('ref_axis',(-0.755033118392644,0.567841300538901,0.327843327723122));
#57276=DIRECTION('',(0.,0.333078167657524,-0.942899217429894));
#57277=DIRECTION('',(0.755033118392644,-0.567841300538901,-0.327843327723122));
#57278=DIRECTION('center_axis',(0.649305557988371,0.717100917309779,0.253315153038431));
#57279=DIRECTION('ref_axis',(-0.760527640763576,0.612229702500115,0.216269505504612));
#57280=DIRECTION('',(-0.0519254248777281,0.374101236076903,-0.925933051260727));
#57281=DIRECTION('center_axis',(-0.649305557988371,-0.662218828358294,-0.373989994161848));
#57282=DIRECTION('ref_axis',(-0.755033118392644,0.502285118831863,0.421467257957652));
#57283=DIRECTION('',(0.,0.491750692698505,-0.870736042799734));
#57284=DIRECTION('',(0.755033118392644,-0.502285118831863,-0.421467257957652));
#57285=DIRECTION('center_axis',(0.649305557988371,0.662218828358294,0.373989994161848));
#57286=DIRECTION('ref_axis',(-0.760527640763576,0.565373752130667,0.31929645791377));
#57287=DIRECTION('',(-0.0519254248777281,0.52920438469299,-0.846904049744115));
#57288=DIRECTION('center_axis',(-0.649305557988371,-0.587215555406038,-0.483301338560726));
#57289=DIRECTION('ref_axis',(-0.755033118392644,0.421467257957652,0.502285118831862));
#57290=DIRECTION('',(0.,0.635481621779699,-0.772115994122802));
#57291=DIRECTION('',(0.755033118392644,-0.421467257957652,-0.502285118831862));
#57292=DIRECTION('center_axis',(0.649305557988371,0.587215555406038,0.483301338560726));
#57293=DIRECTION('ref_axis',(-0.760527640763576,0.501339206395651,0.412621749021022));
#57294=DIRECTION('',(-0.0519254248777281,0.66822792587052,-0.742142297230154));
#57295=DIRECTION('center_axis',(-0.649305557988371,-0.494370034948178,-0.577927816349714));
#57296=DIRECTION('ref_axis',(-0.755033118392644,0.327843327723122,0.567841300538901));
#57297=DIRECTION('',(0.,0.759903763352334,-0.650035591673994));
#57298=DIRECTION('',(0.755033118392644,-0.327843327723122,-0.567841300538901));
#57299=DIRECTION('center_axis',(0.649305557988371,0.494370034948178,0.577927816349714));
#57300=DIRECTION('ref_axis',(-0.760527640763576,0.422071722564183,0.49340973708095));
#57301=DIRECTION('',(-0.0519254248777281,0.786947699660121,-0.614830926556978));
#57302=DIRECTION('center_axis',(-0.649305557988371,-0.386503331141726,-0.654994249884501));
#57303=DIRECTION('ref_axis',(-0.755033118392644,0.224258043872453,0.616143911670627));
#57304=DIRECTION('',(0.,0.861236613605367,-0.508204186706052));
#57305=DIRECTION('',(0.755033118392644,-0.224258043872453,-0.616143911670627));
#57306=DIRECTION('center_axis',(0.649305557988371,0.386503331141726,0.654994249884501));
#57307=DIRECTION('ref_axis',(-0.760527640763576,0.329979803021199,0.559205719957047));
#57308=DIRECTION('',(-0.0519254248777281,0.881756465810299,-0.468838229299829));
#57309=DIRECTION('center_axis',(-0.649305557988371,-0.266892919198654,-0.712159014579631));
#57310=DIRECTION('ref_axis',(-0.755033118392644,0.113858792838765,0.645725301830104));
#57311=DIRECTION('',(0.,0.936401225160755,-0.350931254688773));
#57312=DIRECTION('',(0.755033118392644,-0.113858792838765,-0.645725301830104));
#57313=DIRECTION('center_axis',(0.649305557988371,0.266892919198654,0.712159014579631));
#57314=DIRECTION('ref_axis',(-0.760527640763576,0.227861614141253,0.608010520003998));
#57315=DIRECTION('',(-0.0519254248777281,0.949773507937132,-0.308600119688995));
#57316=DIRECTION('center_axis',(-1.,0.,0.));
#57317=DIRECTION('ref_axis',(0.,0.,1.));
#57318=DIRECTION('',(0.,-0.983113759331517,0.182995454077559));
#57319=DIRECTION('',(0.,0.,-1.));
#57320=DIRECTION('center_axis',(-1.,0.,0.));
#57321=DIRECTION('ref_axis',(0.,0.,1.));
#57322=DIRECTION('',(0.,-0.999954879404557,0.00949942919436634));
#57323=DIRECTION('',(0.,0.17364817766693,-0.984807753012208));
#57324=DIRECTION('center_axis',(-1.,0.,0.));
#57325=DIRECTION('ref_axis',(0.,0.,1.));
#57326=DIRECTION('',(0.,-0.986412876468473,-0.164285231037954));
#57327=DIRECTION('',(0.,0.342020143325669,-0.939692620785908));
#57328=DIRECTION('center_axis',(-1.,0.,0.));
#57329=DIRECTION('ref_axis',(0.,0.,1.));
#57330=DIRECTION('',(0.,-0.942899217429894,-0.333078167657524));
#57331=DIRECTION('',(0.,0.5,-0.866025403784439));
#57332=DIRECTION('center_axis',(-1.,0.,0.));
#57333=DIRECTION('ref_axis',(0.,0.,1.));
#57334=DIRECTION('',(0.,-0.870736042799734,-0.491750692698505));
#57335=DIRECTION('',(0.,0.642787609686539,-0.766044443118978));
#57336=DIRECTION('center_axis',(-1.,0.,0.));
#57337=DIRECTION('ref_axis',(0.,0.,1.));
#57338=DIRECTION('',(0.,-0.772115994122802,-0.6354816217797));
#57339=DIRECTION('',(0.,0.766044443118978,-0.642787609686539));
#57340=DIRECTION('center_axis',(-1.,0.,0.));
#57341=DIRECTION('ref_axis',(0.,0.,1.));
#57342=DIRECTION('',(0.,-0.650035591673993,-0.759903763352335));
#57343=DIRECTION('',(0.,0.866025403784439,-0.5));
#57344=DIRECTION('center_axis',(-1.,0.,0.));
#57345=DIRECTION('ref_axis',(0.,0.,1.));
#57346=DIRECTION('',(0.,-0.508204186706051,-0.861236613605368));
#57347=DIRECTION('',(0.,0.939692620785908,-0.342020143325669));
#57348=DIRECTION('center_axis',(-1.,0.,0.));
#57349=DIRECTION('ref_axis',(0.,0.,1.));
#57350=DIRECTION('',(0.,-0.350931254688773,-0.936401225160756));
#57351=DIRECTION('',(0.,0.984807753012208,-0.17364817766693));
#57352=DIRECTION('center_axis',(-1.,0.,0.));
#57353=DIRECTION('ref_axis',(0.,0.,1.));
#57354=DIRECTION('',(0.,-0.182995454077559,-0.983113759331517));
#57355=DIRECTION('',(0.,1.,-6.12323399573677E-17));
#57356=DIRECTION('center_axis',(-1.,0.,0.));
#57357=DIRECTION('ref_axis',(0.,0.,1.));
#57358=DIRECTION('',(0.,-0.00949942919436638,-0.999954879404557));
#57359=DIRECTION('',(0.,0.984807753012208,0.17364817766693));
#57360=DIRECTION('center_axis',(-1.,0.,0.));
#57361=DIRECTION('ref_axis',(0.,0.,1.));
#57362=DIRECTION('',(0.,0.164285231037954,-0.986412876468473));
#57363=DIRECTION('',(0.,0.939692620785908,0.342020143325669));
#57364=DIRECTION('center_axis',(-1.,0.,0.));
#57365=DIRECTION('ref_axis',(0.,0.,1.));
#57366=DIRECTION('',(0.,0.333078167657524,-0.942899217429894));
#57367=DIRECTION('',(0.,0.866025403784439,0.5));
#57368=DIRECTION('center_axis',(-1.,0.,0.));
#57369=DIRECTION('ref_axis',(0.,0.,1.));
#57370=DIRECTION('',(0.,0.491750692698505,-0.870736042799734));
#57371=DIRECTION('',(0.,0.766044443118978,0.642787609686539));
#57372=DIRECTION('center_axis',(-1.,0.,0.));
#57373=DIRECTION('ref_axis',(0.,0.,1.));
#57374=DIRECTION('',(0.,0.6354816217797,-0.772115994122802));
#57375=DIRECTION('',(0.,0.642787609686539,0.766044443118978));
#57376=DIRECTION('center_axis',(-1.,0.,0.));
#57377=DIRECTION('ref_axis',(0.,0.,1.));
#57378=DIRECTION('',(0.,0.759903763352335,-0.650035591673993));
#57379=DIRECTION('',(0.,0.5,0.866025403784439));
#57380=DIRECTION('center_axis',(-1.,0.,0.));
#57381=DIRECTION('ref_axis',(0.,0.,1.));
#57382=DIRECTION('',(0.,0.861236613605368,-0.508204186706051));
#57383=DIRECTION('',(0.,0.342020143325669,0.939692620785908));
#57384=DIRECTION('center_axis',(-1.,0.,0.));
#57385=DIRECTION('ref_axis',(0.,0.,1.));
#57386=DIRECTION('',(0.,0.936401225160755,-0.350931254688773));
#57387=DIRECTION('',(0.,0.173648177666931,0.984807753012208));
#57388=DIRECTION('center_axis',(-1.,0.,0.));
#57389=DIRECTION('ref_axis',(0.,0.,1.));
#57390=DIRECTION('',(0.,0.983113759331517,-0.182995454077559));
#57391=DIRECTION('',(0.,1.22464679914735E-16,1.));
#57392=DIRECTION('center_axis',(-1.,0.,0.));
#57393=DIRECTION('ref_axis',(0.,0.,1.));
#57394=DIRECTION('',(0.,0.999954879404557,-0.00949942919436667));
#57395=DIRECTION('',(0.,-0.17364817766693,0.984807753012208));
#57396=DIRECTION('center_axis',(-1.,0.,0.));
#57397=DIRECTION('ref_axis',(0.,0.,1.));
#57398=DIRECTION('',(0.,0.986412876468473,0.164285231037954));
#57399=DIRECTION('',(0.,-0.342020143325669,0.939692620785909));
#57400=DIRECTION('center_axis',(-1.,0.,0.));
#57401=DIRECTION('ref_axis',(0.,0.,1.));
#57402=DIRECTION('',(0.,0.942899217429894,0.333078167657524));
#57403=DIRECTION('',(0.,-0.5,0.866025403784439));
#57404=DIRECTION('center_axis',(-1.,0.,0.));
#57405=DIRECTION('ref_axis',(0.,0.,1.));
#57406=DIRECTION('',(0.,0.870736042799734,0.491750692698505));
#57407=DIRECTION('',(0.,-0.642787609686539,0.766044443118978));
#57408=DIRECTION('center_axis',(-1.,0.,0.));
#57409=DIRECTION('ref_axis',(0.,0.,1.));
#57410=DIRECTION('',(0.,0.772115994122802,0.6354816217797));
#57411=DIRECTION('',(0.,-0.766044443118978,0.642787609686539));
#57412=DIRECTION('center_axis',(-1.,0.,0.));
#57413=DIRECTION('ref_axis',(0.,0.,1.));
#57414=DIRECTION('',(0.,0.650035591673993,0.759903763352335));
#57415=DIRECTION('',(0.,-0.866025403784438,0.5));
#57416=DIRECTION('center_axis',(-1.,0.,0.));
#57417=DIRECTION('ref_axis',(0.,0.,1.));
#57418=DIRECTION('',(0.,0.508204186706052,0.861236613605367));
#57419=DIRECTION('',(0.,-0.939692620785908,0.342020143325669));
#57420=DIRECTION('center_axis',(-1.,0.,0.));
#57421=DIRECTION('ref_axis',(0.,0.,1.));
#57422=DIRECTION('',(0.,0.350931254688773,0.936401225160756));
#57423=DIRECTION('',(0.,-0.984807753012208,0.17364817766693));
#57424=DIRECTION('center_axis',(-1.,0.,0.));
#57425=DIRECTION('ref_axis',(0.,0.,1.));
#57426=DIRECTION('',(0.,0.182995454077559,0.983113759331517));
#57427=DIRECTION('',(0.,-1.,1.83697019872103E-16));
#57428=DIRECTION('center_axis',(-1.,0.,0.));
#57429=DIRECTION('ref_axis',(0.,0.,1.));
#57430=DIRECTION('',(0.,0.00949942919436674,0.999954879404557));
#57431=DIRECTION('',(0.,-0.984807753012208,-0.17364817766693));
#57432=DIRECTION('center_axis',(-1.,0.,0.));
#57433=DIRECTION('ref_axis',(0.,0.,1.));
#57434=DIRECTION('',(0.,-0.164285231037953,0.986412876468473));
#57435=DIRECTION('',(0.,-0.939692620785909,-0.342020143325668));
#57436=DIRECTION('center_axis',(-1.,0.,0.));
#57437=DIRECTION('ref_axis',(0.,0.,1.));
#57438=DIRECTION('',(0.,-0.333078167657524,0.942899217429894));
#57439=DIRECTION('',(0.,-0.866025403784439,-0.5));
#57440=DIRECTION('center_axis',(-1.,0.,0.));
#57441=DIRECTION('ref_axis',(0.,0.,1.));
#57442=DIRECTION('',(0.,-0.491750692698505,0.870736042799734));
#57443=DIRECTION('',(0.,-0.766044443118978,-0.642787609686539));
#57444=DIRECTION('center_axis',(-1.,0.,0.));
#57445=DIRECTION('ref_axis',(0.,0.,1.));
#57446=DIRECTION('',(0.,-0.6354816217797,0.772115994122802));
#57447=DIRECTION('',(0.,-0.64278760968654,-0.766044443118978));
#57448=DIRECTION('center_axis',(-1.,0.,0.));
#57449=DIRECTION('ref_axis',(0.,0.,1.));
#57450=DIRECTION('',(0.,-0.759903763352335,0.650035591673993));
#57451=DIRECTION('',(0.,-0.5,-0.866025403784438));
#57452=DIRECTION('center_axis',(-1.,0.,0.));
#57453=DIRECTION('ref_axis',(0.,0.,1.));
#57454=DIRECTION('',(0.,-0.861236613605367,0.508204186706052));
#57455=DIRECTION('',(0.,-0.342020143325669,-0.939692620785908));
#57456=DIRECTION('center_axis',(-1.,0.,0.));
#57457=DIRECTION('ref_axis',(0.,0.,1.));
#57458=DIRECTION('',(0.,-0.936401225160756,0.350931254688773));
#57459=DIRECTION('',(0.,-0.17364817766693,-0.984807753012208));
#57460=DIRECTION('center_axis',(0.649305557988371,-0.266892919198654,-0.712159014579631));
#57461=DIRECTION('ref_axis',(-0.755033118392643,-0.113858792838765,-0.645725301830105));
#57462=DIRECTION('',(0.0519254248777275,0.949773507937132,-0.308600119688995));
#57463=DIRECTION('center_axis',(-0.649305557988371,0.266892919198654,0.712159014579631));
#57464=DIRECTION('ref_axis',(0.760527640763576,0.227861614141253,0.608010520003998));
#57465=DIRECTION('',(0.755033118392643,0.113858792838765,0.645725301830105));
#57466=DIRECTION('center_axis',(0.649305557988371,-0.386503331141725,-0.654994249884501));
#57467=DIRECTION('ref_axis',(-0.755033118392643,-0.224258043872453,-0.616143911670627));
#57468=DIRECTION('',(0.0519254248777275,0.881756465810299,-0.468838229299829));
#57469=DIRECTION('center_axis',(-0.649305557988371,0.386503331141725,0.654994249884501));
#57470=DIRECTION('ref_axis',(0.760527640763576,0.329979803021199,0.559205719957048));
#57471=DIRECTION('',(0.755033118392644,0.224258043872453,0.616143911670627));
#57472=DIRECTION('center_axis',(0.649305557988371,-0.494370034948177,-0.577927816349714));
#57473=DIRECTION('ref_axis',(-0.755033118392643,-0.327843327723122,-0.567841300538901));
#57474=DIRECTION('',(0.0519254248777275,0.78694769966012,-0.614830926556978));
#57475=DIRECTION('center_axis',(-0.649305557988371,0.494370034948177,0.577927816349714));
#57476=DIRECTION('ref_axis',(0.760527640763576,0.422071722564183,0.49340973708095));
#57477=DIRECTION('',(0.755033118392644,0.327843327723122,0.567841300538901));
#57478=DIRECTION('center_axis',(0.649305557988371,-0.587215555406037,-0.483301338560726));
#57479=DIRECTION('ref_axis',(-0.755033118392644,-0.421467257957652,-0.502285118831862));
#57480=DIRECTION('',(0.0519254248777275,0.66822792587052,-0.742142297230154));
#57481=DIRECTION('center_axis',(-0.649305557988371,0.587215555406037,0.483301338560726));
#57482=DIRECTION('ref_axis',(0.760527640763576,0.501339206395651,0.412621749021023));
#57483=DIRECTION('',(0.755033118392644,0.421467257957652,0.502285118831862));
#57484=DIRECTION('center_axis',(0.649305557988371,-0.662218828358294,-0.373989994161848));
#57485=DIRECTION('ref_axis',(-0.755033118392643,-0.502285118831863,-0.421467257957652));
#57486=DIRECTION('',(0.0519254248777275,0.52920438469299,-0.846904049744115));
#57487=DIRECTION('center_axis',(-0.649305557988371,0.662218828358294,0.373989994161848));
#57488=DIRECTION('ref_axis',(0.760527640763576,0.565373752130667,0.319296457913771));
#57489=DIRECTION('',(0.755033118392644,0.502285118831863,0.421467257957652));
#57490=DIRECTION('center_axis',(0.649305557988371,-0.717100917309779,-0.253315153038431));
#57491=DIRECTION('ref_axis',(-0.755033118392643,-0.567841300538901,-0.327843327723122));
#57492=DIRECTION('',(0.0519254248777275,0.374101236076903,-0.925933051260727));
#57493=DIRECTION('center_axis',(-0.649305557988371,0.717100917309779,0.253315153038431));
#57494=DIRECTION('ref_axis',(0.760527640763576,0.612229702500115,0.216269505504613));
#57495=DIRECTION('',(0.755033118392644,0.567841300538901,0.327843327723122));
#57496=DIRECTION('center_axis',(0.649305557988371,-0.75019425775938,-0.124943459173594));
#57497=DIRECTION('ref_axis',(-0.755033118392643,-0.616143911670627,-0.224258043872452));
#57498=DIRECTION('',(0.0519254248777275,0.207631210706978,-0.976828045559515));
#57499=DIRECTION('center_axis',(-0.649305557988371,0.75019425775938,0.124943459173594));
#57500=DIRECTION('ref_axis',(0.760527640763576,0.640483363162275,0.106671313608347));
#57501=DIRECTION('',(0.755033118392643,0.616143911670627,0.224258043872452));
#57502=DIRECTION('center_axis',(0.649305557988371,-0.760493325303573,0.00722457847379238));
#57503=DIRECTION('ref_axis',(-0.755033118392643,-0.645725301830105,-0.113858792838764));
#57504=DIRECTION('',(0.0519254248777275,0.0348524160661842,-0.998042613992818));
#57505=DIRECTION('center_axis',(-0.649305557988371,0.760493325303573,-0.00722457847379238));
#57506=DIRECTION('ref_axis',(0.760527640763576,0.64927626093497,-0.00616803217361932));
#57507=DIRECTION('',(0.755033118392643,0.645725301830105,0.113858792838764));
#57508=DIRECTION('center_axis',(0.649305557988371,-0.747685187986609,0.139173100960065));
#57509=DIRECTION('ref_axis',(-0.755033118392643,-0.655686655446243,1.20447684575381E-16));
#57510=DIRECTION('',(0.0519254248777275,-0.138985351600607,-0.98893216263388));
#57511=DIRECTION('center_axis',(-0.649305557988371,0.747685187986609,-0.139173100960065));
#57512=DIRECTION('ref_axis',(0.760527640763576,0.638341228068795,-0.118819965419165));
#57513=DIRECTION('',(0.755033118392644,0.655686655446243,-1.20447684575381E-16));
#57514=DIRECTION('center_axis',(0.649305557988371,-0.712159014579631,0.266892919198654));
#57515=DIRECTION('ref_axis',(-0.755033118392643,-0.645725301830105,0.113858792838765));
#57516=DIRECTION('',(0.0519254248777275,-0.308600119688995,-0.949773507937132));
#57517=DIRECTION('center_axis',(-0.649305557988371,0.712159014579631,-0.266892919198654));
#57518=DIRECTION('ref_axis',(0.760527640763576,0.608010520003998,-0.227861614141252));
#57519=DIRECTION('',(0.755033118392643,0.645725301830105,-0.113858792838765));
#57520=DIRECTION('center_axis',(0.649305557988371,-0.654994249884501,0.386503331141725));
#57521=DIRECTION('ref_axis',(-0.755033118392643,-0.616143911670627,0.224258043872453));
#57522=DIRECTION('',(0.0519254248777275,-0.468838229299829,-0.881756465810299));
#57523=DIRECTION('center_axis',(-0.649305557988371,0.654994249884501,-0.386503331141725));
#57524=DIRECTION('ref_axis',(0.760527640763576,0.559205719957048,-0.329979803021199));
#57525=DIRECTION('',(0.755033118392644,0.616143911670627,-0.224258043872453));
#57526=DIRECTION('center_axis',(0.649305557988371,-0.577927816349714,0.494370034948177));
#57527=DIRECTION('ref_axis',(-0.755033118392643,-0.567841300538901,0.327843327723122));
#57528=DIRECTION('',(0.0519254248777275,-0.614830926556978,-0.78694769966012));
#57529=DIRECTION('center_axis',(-0.649305557988371,0.577927816349714,-0.494370034948177));
#57530=DIRECTION('ref_axis',(0.760527640763576,0.493409737080951,-0.422071722564183));
#57531=DIRECTION('',(0.755033118392644,0.567841300538901,-0.327843327723122));
#57532=DIRECTION('center_axis',(0.649305557988371,-0.483301338560726,0.587215555406037));
#57533=DIRECTION('ref_axis',(-0.755033118392643,-0.502285118831862,0.421467257957652));
#57534=DIRECTION('',(0.0519254248777275,-0.742142297230154,-0.66822792587052));
#57535=DIRECTION('center_axis',(-0.649305557988371,0.483301338560726,-0.587215555406037));
#57536=DIRECTION('ref_axis',(0.760527640763576,0.412621749021023,-0.501339206395651));
#57537=DIRECTION('',(0.755033118392644,0.502285118831862,-0.421467257957652));
#57538=DIRECTION('center_axis',(0.649305557988371,-0.373989994161849,0.662218828358294));
#57539=DIRECTION('ref_axis',(-0.755033118392643,-0.421467257957652,0.502285118831863));
#57540=DIRECTION('',(0.0519254248777275,-0.846904049744115,-0.52920438469299));
#57541=DIRECTION('center_axis',(-0.649305557988371,0.373989994161849,-0.662218828358294));
#57542=DIRECTION('ref_axis',(0.760527640763576,0.319296457913771,-0.565373752130667));
#57543=DIRECTION('',(0.755033118392644,0.421467257957652,-0.502285118831863));
#57544=DIRECTION('center_axis',(0.649305557988371,-0.253315153038431,0.717100917309779));
#57545=DIRECTION('ref_axis',(-0.755033118392643,-0.327843327723121,0.567841300538901));
#57546=DIRECTION('',(0.0519254248777275,-0.925933051260728,-0.374101236076902));
#57547=DIRECTION('center_axis',(-0.649305557988371,0.253315153038431,-0.717100917309779));
#57548=DIRECTION('ref_axis',(0.760527640763576,0.216269505504612,-0.612229702500115));
#57549=DIRECTION('',(0.755033118392644,0.327843327723121,-0.567841300538901));
#57550=DIRECTION('center_axis',(0.649305557988371,-0.124943459173594,0.75019425775938));
#57551=DIRECTION('ref_axis',(-0.755033118392643,-0.224258043872452,0.616143911670627));
#57552=DIRECTION('',(0.0519254248777275,-0.976828045559515,-0.207631210706978));
#57553=DIRECTION('center_axis',(-0.649305557988371,0.124943459173594,-0.75019425775938));
#57554=DIRECTION('ref_axis',(0.760527640763576,0.106671313608347,-0.640483363162275));
#57555=DIRECTION('',(0.755033118392644,0.224258043872452,-0.616143911670627));
#57556=DIRECTION('center_axis',(0.649305557988371,0.00722457847379232,0.760493325303573));
#57557=DIRECTION('ref_axis',(-0.755033118392643,-0.113858792838764,0.645725301830105));
#57558=DIRECTION('',(0.0519254248777275,-0.998042613992818,-0.0348524160661842));
#57559=DIRECTION('center_axis',(-0.649305557988371,-0.00722457847379232,
-0.760493325303573));
#57560=DIRECTION('ref_axis',(-0.760527640763576,0.00616803217361924,0.64927626093497));
#57561=DIRECTION('',(0.755033118392643,0.113858792838764,-0.645725301830105));
#57562=DIRECTION('center_axis',(0.649305557988371,0.139173100960065,0.747685187986609));
#57563=DIRECTION('ref_axis',(-0.755033118392643,8.02984563835875E-17,0.655686655446243));
#57564=DIRECTION('',(0.0519254248777275,-0.98893216263388,0.138985351600607));
#57565=DIRECTION('center_axis',(-0.649305557988371,-0.139173100960065,-0.747685187986609));
#57566=DIRECTION('ref_axis',(-0.760527640763576,0.118819965419165,0.638341228068795));
#57567=DIRECTION('',(0.755033118392644,-8.02984563835875E-17,-0.655686655446243));
#57568=DIRECTION('center_axis',(0.649305557988371,0.266892919198654,0.712159014579631));
#57569=DIRECTION('ref_axis',(-0.755033118392643,0.113858792838765,0.645725301830105));
#57570=DIRECTION('',(0.0519254248777275,-0.949773507937132,0.308600119688995));
#57571=DIRECTION('center_axis',(-0.649305557988371,-0.266892919198654,-0.712159014579631));
#57572=DIRECTION('ref_axis',(-0.760527640763576,0.227861614141253,0.608010520003998));
#57573=DIRECTION('',(0.755033118392644,-0.113858792838765,-0.645725301830105));
#57574=DIRECTION('center_axis',(0.649305557988371,0.386503331141725,0.654994249884502));
#57575=DIRECTION('ref_axis',(-0.755033118392643,0.224258043872453,0.616143911670627));
#57576=DIRECTION('',(0.0519254248777275,-0.881756465810299,0.468838229299828));
#57577=DIRECTION('center_axis',(-0.649305557988371,-0.386503331141725,-0.654994249884502));
#57578=DIRECTION('ref_axis',(-0.760527640763576,0.329979803021199,0.559205719957048));
#57579=DIRECTION('',(0.755033118392643,-0.224258043872453,-0.616143911670627));
#57580=DIRECTION('center_axis',(0.649305557988371,0.494370034948177,0.577927816349714));
#57581=DIRECTION('ref_axis',(-0.755033118392643,0.327843327723122,0.567841300538901));
#57582=DIRECTION('',(0.0519254248777275,-0.786947699660121,0.614830926556978));
#57583=DIRECTION('center_axis',(-0.649305557988371,-0.494370034948177,-0.577927816349714));
#57584=DIRECTION('ref_axis',(-0.760527640763576,0.422071722564183,0.493409737080951));
#57585=DIRECTION('',(0.755033118392644,-0.327843327723122,-0.567841300538901));
#57586=DIRECTION('center_axis',(0.649305557988371,0.587215555406037,0.483301338560726));
#57587=DIRECTION('ref_axis',(-0.755033118392644,0.421467257957652,0.502285118831862));
#57588=DIRECTION('',(0.0519254248777275,-0.66822792587052,0.742142297230154));
#57589=DIRECTION('center_axis',(-0.649305557988371,-0.587215555406037,-0.483301338560726));
#57590=DIRECTION('ref_axis',(-0.760527640763576,0.501339206395651,0.412621749021023));
#57591=DIRECTION('',(0.755033118392644,-0.421467257957652,-0.502285118831862));
#57592=DIRECTION('center_axis',(0.649305557988371,0.662218828358294,0.373989994161849));
#57593=DIRECTION('ref_axis',(-0.755033118392643,0.502285118831863,0.421467257957652));
#57594=DIRECTION('',(0.0519254248777275,-0.52920438469299,0.846904049744115));
#57595=DIRECTION('center_axis',(-0.649305557988371,-0.662218828358294,-0.373989994161849));
#57596=DIRECTION('ref_axis',(-0.760527640763576,0.565373752130667,0.319296457913771));
#57597=DIRECTION('',(0.755033118392644,-0.502285118831863,-0.421467257957652));
#57598=DIRECTION('center_axis',(0.649305557988371,0.717100917309779,0.253315153038431));
#57599=DIRECTION('ref_axis',(-0.755033118392643,0.567841300538901,0.327843327723121));
#57600=DIRECTION('',(0.0519254248777275,-0.374101236076902,0.925933051260728));
#57601=DIRECTION('center_axis',(-0.649305557988371,-0.717100917309779,-0.253315153038431));
#57602=DIRECTION('ref_axis',(-0.760527640763576,0.612229702500115,0.216269505504613));
#57603=DIRECTION('',(0.755033118392644,-0.567841300538901,-0.327843327723121));
#57604=DIRECTION('center_axis',(0.649305557988371,0.75019425775938,0.124943459173594));
#57605=DIRECTION('ref_axis',(-0.755033118392643,0.616143911670627,0.224258043872452));
#57606=DIRECTION('',(0.0519254248777275,-0.207631210706978,0.976828045559515));
#57607=DIRECTION('center_axis',(-0.649305557988371,-0.75019425775938,-0.124943459173594));
#57608=DIRECTION('ref_axis',(-0.760527640763576,0.640483363162275,0.106671313608347));
#57609=DIRECTION('',(0.755033118392644,-0.616143911670627,-0.224258043872452));
#57610=DIRECTION('center_axis',(0.649305557988371,0.760493325303573,-0.0072245784737921));
#57611=DIRECTION('ref_axis',(-0.755033118392643,0.645725301830105,0.113858792838765));
#57612=DIRECTION('',(0.0519254248777275,-0.0348524160661845,0.998042613992818));
#57613=DIRECTION('center_axis',(-0.649305557988371,-0.760493325303573,0.0072245784737921));
#57614=DIRECTION('ref_axis',(-0.760527640763576,0.64927626093497,-0.00616803217361908));
#57615=DIRECTION('',(0.755033118392643,-0.645725301830105,-0.113858792838765));
#57616=DIRECTION('center_axis',(0.649305557988371,0.747685187986609,-0.139173100960065));
#57617=DIRECTION('ref_axis',(-0.755033118392643,0.655686655446243,-4.01492281917938E-17));
#57618=DIRECTION('',(0.0519254248777275,0.138985351600607,0.98893216263388));
#57619=DIRECTION('center_axis',(-0.649305557988371,-0.747685187986609,0.139173100960065));
#57620=DIRECTION('ref_axis',(-0.760527640763576,0.638341228068795,-0.118819965419165));
#57621=DIRECTION('',(0.755033118392644,-0.655686655446243,4.01492281917938E-17));
#57622=DIRECTION('center_axis',(0.649305557988371,0.712159014579631,-0.266892919198654));
#57623=DIRECTION('ref_axis',(-0.755033118392643,0.645725301830105,-0.113858792838765));
#57624=DIRECTION('',(0.0519254248777275,0.308600119688995,0.949773507937132));
#57625=DIRECTION('center_axis',(-0.649305557988371,-0.712159014579631,0.266892919198654));
#57626=DIRECTION('ref_axis',(-0.760527640763576,0.608010520003998,-0.227861614141252));
#57627=DIRECTION('',(0.755033118392643,-0.645725301830105,0.113858792838765));
#57628=DIRECTION('center_axis',(0.649305557988371,0.654994249884502,-0.386503331141725));
#57629=DIRECTION('ref_axis',(-0.755033118392643,0.616143911670627,-0.224258043872453));
#57630=DIRECTION('',(0.0519254248777275,0.468838229299828,0.881756465810299));
#57631=DIRECTION('center_axis',(-0.649305557988371,-0.654994249884502,0.386503331141725));
#57632=DIRECTION('ref_axis',(-0.760527640763576,0.559205719957048,-0.329979803021199));
#57633=DIRECTION('',(0.755033118392644,-0.616143911670627,0.224258043872453));
#57634=DIRECTION('center_axis',(0.649305557988371,0.577927816349714,-0.494370034948177));
#57635=DIRECTION('ref_axis',(-0.755033118392643,0.567841300538901,-0.327843327723122));
#57636=DIRECTION('',(0.0519254248777275,0.614830926556978,0.786947699660121));
#57637=DIRECTION('center_axis',(-0.649305557988371,-0.577927816349714,0.494370034948177));
#57638=DIRECTION('ref_axis',(-0.760527640763576,0.493409737080951,-0.422071722564183));
#57639=DIRECTION('',(0.755033118392644,-0.567841300538901,0.327843327723122));
#57640=DIRECTION('center_axis',(0.649305557988371,0.483301338560726,-0.587215555406037));
#57641=DIRECTION('ref_axis',(-0.755033118392643,0.502285118831863,-0.421467257957652));
#57642=DIRECTION('',(0.0519254248777275,0.742142297230154,0.66822792587052));
#57643=DIRECTION('center_axis',(-0.649305557988371,-0.483301338560726,0.587215555406037));
#57644=DIRECTION('ref_axis',(-0.760527640763576,0.412621749021023,-0.501339206395651));
#57645=DIRECTION('',(0.755033118392644,-0.502285118831863,0.421467257957652));
#57646=DIRECTION('center_axis',(0.649305557988371,0.373989994161849,-0.662218828358294));
#57647=DIRECTION('ref_axis',(-0.755033118392643,0.421467257957652,-0.502285118831863));
#57648=DIRECTION('',(0.0519254248777275,0.846904049744115,0.52920438469299));
#57649=DIRECTION('center_axis',(-0.649305557988371,-0.373989994161849,0.662218828358294));
#57650=DIRECTION('ref_axis',(-0.760527640763576,0.319296457913771,-0.565373752130667));
#57651=DIRECTION('',(0.755033118392644,-0.421467257957652,0.502285118831863));
#57652=DIRECTION('center_axis',(0.649305557988371,0.253315153038431,-0.717100917309779));
#57653=DIRECTION('ref_axis',(-0.755033118392643,0.327843327723122,-0.567841300538901));
#57654=DIRECTION('',(0.0519254248777275,0.925933051260728,0.374101236076902));
#57655=DIRECTION('center_axis',(-0.649305557988371,-0.253315153038431,0.717100917309779));
#57656=DIRECTION('ref_axis',(-0.760527640763576,0.216269505504613,-0.612229702500115));
#57657=DIRECTION('',(0.755033118392644,-0.327843327723122,0.567841300538901));
#57658=DIRECTION('center_axis',(0.649305557988371,0.124943459173594,-0.75019425775938));
#57659=DIRECTION('ref_axis',(-0.755033118392643,0.224258043872452,-0.616143911670627));
#57660=DIRECTION('',(0.0519254248777275,0.976828045559515,0.207631210706978));
#57661=DIRECTION('center_axis',(-0.649305557988371,-0.124943459173594,0.75019425775938));
#57662=DIRECTION('ref_axis',(-0.760527640763576,0.106671313608347,-0.640483363162275));
#57663=DIRECTION('',(0.755033118392644,-0.224258043872452,0.616143911670627));
#57664=DIRECTION('center_axis',(0.649305557988371,-0.00722457847379207,
-0.760493325303573));
#57665=DIRECTION('ref_axis',(-0.755033118392643,0.113858792838765,-0.645725301830105));
#57666=DIRECTION('',(0.0519254248777275,0.998042613992818,0.0348524160661846));
#57667=DIRECTION('center_axis',(-0.649305557988371,0.00722457847379207,
0.760493325303573));
#57668=DIRECTION('ref_axis',(0.760527640763576,0.0061680321736191,0.64927626093497));
#57669=DIRECTION('',(0.755033118392643,-0.113858792838765,0.645725301830105));
#57670=DIRECTION('center_axis',(0.,1.,0.));
#57671=DIRECTION('ref_axis',(1.,0.,0.));
#57672=DIRECTION('',(0.755033118392644,0.,0.655686655446243));
#57673=DIRECTION('center_axis',(1.,0.,0.));
#57674=DIRECTION('ref_axis',(0.,0.,-1.));
#57675=DIRECTION('',(0.,-0.983113759331517,-0.182995454077559));
#57676=DIRECTION('',(0.,0.,1.));
#57677=DIRECTION('center_axis',(1.,0.,0.));
#57678=DIRECTION('ref_axis',(0.,0.,-1.));
#57679=DIRECTION('',(0.,-0.936401225160755,-0.350931254688773));
#57680=DIRECTION('',(0.,-0.17364817766693,0.984807753012208));
#57681=DIRECTION('center_axis',(1.,0.,0.));
#57682=DIRECTION('ref_axis',(0.,0.,-1.));
#57683=DIRECTION('',(0.,-0.861236613605367,-0.508204186706051));
#57684=DIRECTION('',(0.,-0.342020143325669,0.939692620785908));
#57685=DIRECTION('center_axis',(1.,0.,0.));
#57686=DIRECTION('ref_axis',(0.,0.,-1.));
#57687=DIRECTION('',(0.,-0.759903763352335,-0.650035591673993));
#57688=DIRECTION('',(0.,-0.5,0.866025403784439));
#57689=DIRECTION('center_axis',(1.,0.,0.));
#57690=DIRECTION('ref_axis',(0.,0.,-1.));
#57691=DIRECTION('',(0.,-0.6354816217797,-0.772115994122802));
#57692=DIRECTION('',(0.,-0.642787609686539,0.766044443118978));
#57693=DIRECTION('center_axis',(1.,0.,0.));
#57694=DIRECTION('ref_axis',(0.,0.,-1.));
#57695=DIRECTION('',(0.,-0.491750692698505,-0.870736042799734));
#57696=DIRECTION('',(0.,-0.766044443118978,0.642787609686539));
#57697=DIRECTION('center_axis',(1.,0.,0.));
#57698=DIRECTION('ref_axis',(0.,0.,-1.));
#57699=DIRECTION('',(0.,-0.333078167657524,-0.942899217429894));
#57700=DIRECTION('',(0.,-0.866025403784439,0.5));
#57701=DIRECTION('center_axis',(1.,0.,0.));
#57702=DIRECTION('ref_axis',(0.,0.,-1.));
#57703=DIRECTION('',(0.,-0.164285231037954,-0.986412876468473));
#57704=DIRECTION('',(0.,-0.939692620785908,0.342020143325669));
#57705=DIRECTION('center_axis',(1.,0.,0.));
#57706=DIRECTION('ref_axis',(0.,0.,-1.));
#57707=DIRECTION('',(0.,0.00949942919436663,-0.999954879404557));
#57708=DIRECTION('',(0.,-0.984807753012208,0.17364817766693));
#57709=DIRECTION('center_axis',(1.,0.,0.));
#57710=DIRECTION('ref_axis',(0.,0.,-1.));
#57711=DIRECTION('',(0.,0.182995454077559,-0.983113759331517));
#57712=DIRECTION('',(0.,-1.,6.12323399573677E-17));
#57713=DIRECTION('center_axis',(1.,0.,0.));
#57714=DIRECTION('ref_axis',(0.,0.,-1.));
#57715=DIRECTION('',(0.,0.350931254688773,-0.936401225160755));
#57716=DIRECTION('',(0.,-0.984807753012208,-0.17364817766693));
#57717=DIRECTION('center_axis',(1.,0.,0.));
#57718=DIRECTION('ref_axis',(0.,0.,-1.));
#57719=DIRECTION('',(0.,0.508204186706051,-0.861236613605367));
#57720=DIRECTION('',(0.,-0.939692620785908,-0.342020143325669));
#57721=DIRECTION('center_axis',(1.,0.,0.));
#57722=DIRECTION('ref_axis',(0.,0.,-1.));
#57723=DIRECTION('',(0.,0.650035591673993,-0.759903763352335));
#57724=DIRECTION('',(0.,-0.866025403784439,-0.5));
#57725=DIRECTION('center_axis',(1.,0.,0.));
#57726=DIRECTION('ref_axis',(0.,0.,-1.));
#57727=DIRECTION('',(0.,0.772115994122802,-0.6354816217797));
#57728=DIRECTION('',(0.,-0.766044443118978,-0.642787609686539));
#57729=DIRECTION('center_axis',(1.,0.,0.));
#57730=DIRECTION('ref_axis',(0.,0.,-1.));
#57731=DIRECTION('',(0.,0.870736042799734,-0.491750692698505));
#57732=DIRECTION('',(0.,-0.642787609686539,-0.766044443118978));
#57733=DIRECTION('center_axis',(1.,0.,0.));
#57734=DIRECTION('ref_axis',(0.,0.,-1.));
#57735=DIRECTION('',(0.,0.942899217429894,-0.333078167657523));
#57736=DIRECTION('',(0.,-0.5,-0.866025403784439));
#57737=DIRECTION('center_axis',(1.,0.,0.));
#57738=DIRECTION('ref_axis',(0.,0.,-1.));
#57739=DIRECTION('',(0.,0.986412876468473,-0.164285231037954));
#57740=DIRECTION('',(0.,-0.342020143325669,-0.939692620785908));
#57741=DIRECTION('center_axis',(1.,0.,0.));
#57742=DIRECTION('ref_axis',(0.,0.,-1.));
#57743=DIRECTION('',(0.,0.999954879404557,0.00949942919436638));
#57744=DIRECTION('',(0.,-0.173648177666931,-0.984807753012208));
#57745=DIRECTION('center_axis',(1.,0.,0.));
#57746=DIRECTION('ref_axis',(0.,0.,-1.));
#57747=DIRECTION('',(0.,0.983113759331517,0.182995454077559));
#57748=DIRECTION('',(0.,-1.22464679914735E-16,-1.));
#57749=DIRECTION('center_axis',(1.,0.,0.));
#57750=DIRECTION('ref_axis',(0.,0.,-1.));
#57751=DIRECTION('',(0.,0.936401225160756,0.350931254688773));
#57752=DIRECTION('',(0.,0.17364817766693,-0.984807753012208));
#57753=DIRECTION('center_axis',(1.,0.,0.));
#57754=DIRECTION('ref_axis',(0.,0.,-1.));
#57755=DIRECTION('',(0.,0.861236613605368,0.508204186706051));
#57756=DIRECTION('',(0.,0.342020143325669,-0.939692620785909));
#57757=DIRECTION('center_axis',(1.,0.,0.));
#57758=DIRECTION('ref_axis',(0.,0.,-1.));
#57759=DIRECTION('',(0.,0.759903763352335,0.650035591673993));
#57760=DIRECTION('',(0.,0.5,-0.866025403784439));
#57761=DIRECTION('center_axis',(1.,0.,0.));
#57762=DIRECTION('ref_axis',(0.,0.,-1.));
#57763=DIRECTION('',(0.,0.6354816217797,0.772115994122802));
#57764=DIRECTION('',(0.,0.642787609686539,-0.766044443118978));
#57765=DIRECTION('center_axis',(1.,0.,0.));
#57766=DIRECTION('ref_axis',(0.,0.,-1.));
#57767=DIRECTION('',(0.,0.491750692698505,0.870736042799734));
#57768=DIRECTION('',(0.,0.766044443118978,-0.642787609686539));
#57769=DIRECTION('center_axis',(1.,0.,0.));
#57770=DIRECTION('ref_axis',(0.,0.,-1.));
#57771=DIRECTION('',(0.,0.333078167657524,0.942899217429894));
#57772=DIRECTION('',(0.,0.866025403784438,-0.5));
#57773=DIRECTION('center_axis',(1.,0.,0.));
#57774=DIRECTION('ref_axis',(0.,0.,-1.));
#57775=DIRECTION('',(0.,0.164285231037954,0.986412876468473));
#57776=DIRECTION('',(0.,0.939692620785908,-0.342020143325669));
#57777=DIRECTION('center_axis',(1.,0.,0.));
#57778=DIRECTION('ref_axis',(0.,0.,-1.));
#57779=DIRECTION('',(0.,-0.00949942919436674,0.999954879404557));
#57780=DIRECTION('',(0.,0.984807753012208,-0.17364817766693));
#57781=DIRECTION('center_axis',(1.,0.,0.));
#57782=DIRECTION('ref_axis',(0.,0.,-1.));
#57783=DIRECTION('',(0.,-0.182995454077559,0.983113759331517));
#57784=DIRECTION('',(0.,1.,-1.83697019872103E-16));
#57785=DIRECTION('center_axis',(1.,0.,0.));
#57786=DIRECTION('ref_axis',(0.,0.,-1.));
#57787=DIRECTION('',(0.,-0.350931254688773,0.936401225160756));
#57788=DIRECTION('',(0.,0.984807753012208,0.17364817766693));
#57789=DIRECTION('center_axis',(1.,0.,0.));
#57790=DIRECTION('ref_axis',(0.,0.,-1.));
#57791=DIRECTION('',(0.,-0.508204186706051,0.861236613605368));
#57792=DIRECTION('',(0.,0.939692620785909,0.342020143325668));
#57793=DIRECTION('center_axis',(1.,0.,0.));
#57794=DIRECTION('ref_axis',(0.,0.,-1.));
#57795=DIRECTION('',(0.,-0.650035591673993,0.759903763352335));
#57796=DIRECTION('',(0.,0.866025403784439,0.5));
#57797=DIRECTION('center_axis',(1.,0.,0.));
#57798=DIRECTION('ref_axis',(0.,0.,-1.));
#57799=DIRECTION('',(0.,-0.772115994122802,0.6354816217797));
#57800=DIRECTION('',(0.,0.766044443118978,0.642787609686539));
#57801=DIRECTION('center_axis',(1.,0.,0.));
#57802=DIRECTION('ref_axis',(0.,0.,-1.));
#57803=DIRECTION('',(0.,-0.870736042799734,0.491750692698505));
#57804=DIRECTION('',(0.,0.64278760968654,0.766044443118978));
#57805=DIRECTION('center_axis',(1.,0.,0.));
#57806=DIRECTION('ref_axis',(0.,0.,-1.));
#57807=DIRECTION('',(0.,-0.942899217429894,0.333078167657524));
#57808=DIRECTION('',(0.,0.5,0.866025403784438));
#57809=DIRECTION('center_axis',(1.,0.,0.));
#57810=DIRECTION('ref_axis',(0.,0.,-1.));
#57811=DIRECTION('',(0.,-0.986412876468473,0.164285231037954));
#57812=DIRECTION('',(0.,0.342020143325669,0.939692620785908));
#57813=DIRECTION('center_axis',(1.,0.,0.));
#57814=DIRECTION('ref_axis',(0.,0.,-1.));
#57815=DIRECTION('',(0.,-0.999954879404557,-0.00949942919436667));
#57816=DIRECTION('',(0.,0.17364817766693,0.984807753012208));
#57817=DIRECTION('center_axis',(0.,0.984807753012208,-0.17364817766693));
#57818=DIRECTION('ref_axis',(1.,0.,0.));
#57819=DIRECTION('',(-0.755033118392644,-0.113858792838765,-0.645725301830104));
#57820=DIRECTION('center_axis',(0.,0.939692620785908,-0.342020143325669));
#57821=DIRECTION('ref_axis',(1.,0.,0.));
#57822=DIRECTION('',(-0.755033118392644,-0.224258043872453,-0.616143911670627));
#57823=DIRECTION('center_axis',(0.,0.866025403784438,-0.5));
#57824=DIRECTION('ref_axis',(1.,0.,0.));
#57825=DIRECTION('',(-0.755033118392644,-0.327843327723122,-0.567841300538901));
#57826=DIRECTION('center_axis',(0.,0.766044443118978,-0.64278760968654));
#57827=DIRECTION('ref_axis',(1.,0.,0.));
#57828=DIRECTION('',(-0.755033118392644,-0.421467257957652,-0.502285118831862));
#57829=DIRECTION('center_axis',(0.,0.642787609686539,-0.766044443118978));
#57830=DIRECTION('ref_axis',(1.,0.,0.));
#57831=DIRECTION('',(-0.755033118392644,-0.502285118831863,-0.421467257957652));
#57832=DIRECTION('center_axis',(0.,0.5,-0.866025403784439));
#57833=DIRECTION('ref_axis',(1.,0.,0.));
#57834=DIRECTION('',(-0.755033118392644,-0.567841300538901,-0.327843327723122));
#57835=DIRECTION('center_axis',(0.,0.342020143325668,-0.939692620785909));
#57836=DIRECTION('ref_axis',(1.,0.,0.));
#57837=DIRECTION('',(-0.755033118392644,-0.616143911670627,-0.224258043872452));
#57838=DIRECTION('center_axis',(0.,0.17364817766693,-0.984807753012208));
#57839=DIRECTION('ref_axis',(1.,0.,0.));
#57840=DIRECTION('',(-0.755033118392644,-0.645725301830105,-0.113858792838764));
#57841=DIRECTION('center_axis',(0.,-1.83697019872103E-16,-1.));
#57842=DIRECTION('ref_axis',(1.,0.,0.));
#57843=DIRECTION('',(-0.755033118392644,-0.655686655446243,1.20447684575381E-16));
#57844=DIRECTION('center_axis',(0.,-0.17364817766693,-0.984807753012208));
#57845=DIRECTION('ref_axis',(1.,0.,0.));
#57846=DIRECTION('',(-0.755033118392644,-0.645725301830105,0.113858792838765));
#57847=DIRECTION('center_axis',(0.,-0.342020143325669,-0.939692620785908));
#57848=DIRECTION('ref_axis',(1.,0.,0.));
#57849=DIRECTION('',(-0.755033118392644,-0.616143911670627,0.224258043872453));
#57850=DIRECTION('center_axis',(0.,-0.5,-0.866025403784438));
#57851=DIRECTION('ref_axis',(1.,0.,0.));
#57852=DIRECTION('',(-0.755033118392644,-0.567841300538901,0.327843327723122));
#57853=DIRECTION('center_axis',(0.,-0.642787609686539,-0.766044443118978));
#57854=DIRECTION('ref_axis',(1.,0.,0.));
#57855=DIRECTION('',(-0.755033118392644,-0.502285118831862,0.421467257957652));
#57856=DIRECTION('center_axis',(0.,-0.766044443118978,-0.642787609686539));
#57857=DIRECTION('ref_axis',(1.,0.,0.));
#57858=DIRECTION('',(-0.755033118392644,-0.421467257957652,0.502285118831862));
#57859=DIRECTION('center_axis',(0.,-0.866025403784439,-0.5));
#57860=DIRECTION('ref_axis',(1.,0.,0.));
#57861=DIRECTION('',(-0.755033118392644,-0.327843327723121,0.567841300538901));
#57862=DIRECTION('center_axis',(0.,-0.939692620785908,-0.342020143325669));
#57863=DIRECTION('ref_axis',(1.,0.,0.));
#57864=DIRECTION('',(-0.755033118392644,-0.224258043872452,0.616143911670627));
#57865=DIRECTION('center_axis',(0.,-0.984807753012208,-0.17364817766693));
#57866=DIRECTION('ref_axis',(1.,0.,0.));
#57867=DIRECTION('',(-0.755033118392644,-0.113858792838764,0.645725301830105));
#57868=DIRECTION('center_axis',(0.,-1.,1.22464679914735E-16));
#57869=DIRECTION('ref_axis',(1.,0.,0.));
#57870=DIRECTION('',(-0.755033118392644,8.02984563835875E-17,0.655686655446243));
#57871=DIRECTION('center_axis',(0.,-0.984807753012208,0.173648177666931));
#57872=DIRECTION('ref_axis',(1.,0.,0.));
#57873=DIRECTION('',(-0.755033118392644,0.113858792838765,0.645725301830104));
#57874=DIRECTION('center_axis',(0.,-0.939692620785908,0.342020143325669));
#57875=DIRECTION('ref_axis',(1.,0.,0.));
#57876=DIRECTION('',(-0.755033118392644,0.224258043872452,0.616143911670627));
#57877=DIRECTION('center_axis',(0.,-0.866025403784439,0.5));
#57878=DIRECTION('ref_axis',(1.,0.,0.));
#57879=DIRECTION('',(-0.755033118392644,0.327843327723121,0.567841300538901));
#57880=DIRECTION('center_axis',(0.,-0.766044443118978,0.642787609686539));
#57881=DIRECTION('ref_axis',(1.,0.,0.));
#57882=DIRECTION('',(-0.755033118392644,0.421467257957652,0.502285118831862));
#57883=DIRECTION('center_axis',(0.,-0.642787609686539,0.766044443118978));
#57884=DIRECTION('ref_axis',(1.,0.,0.));
#57885=DIRECTION('',(-0.755033118392644,0.502285118831862,0.421467257957652));
#57886=DIRECTION('center_axis',(0.,-0.5,0.866025403784439));
#57887=DIRECTION('ref_axis',(1.,0.,0.));
#57888=DIRECTION('',(-0.755033118392644,0.567841300538901,0.327843327723121));
#57889=DIRECTION('center_axis',(0.,-0.342020143325669,0.939692620785908));
#57890=DIRECTION('ref_axis',(1.,0.,0.));
#57891=DIRECTION('',(-0.755033118392644,0.616143911670627,0.224258043872452));
#57892=DIRECTION('center_axis',(0.,-0.17364817766693,0.984807753012208));
#57893=DIRECTION('ref_axis',(1.,0.,0.));
#57894=DIRECTION('',(-0.755033118392644,0.645725301830105,0.113858792838765));
#57895=DIRECTION('center_axis',(0.,6.12323399573677E-17,1.));
#57896=DIRECTION('ref_axis',(1.,0.,0.));
#57897=DIRECTION('',(-0.755033118392644,0.655686655446243,-4.01492281917938E-17));
#57898=DIRECTION('center_axis',(0.,0.17364817766693,0.984807753012208));
#57899=DIRECTION('ref_axis',(1.,0.,0.));
#57900=DIRECTION('',(-0.755033118392644,0.645725301830105,-0.113858792838765));
#57901=DIRECTION('center_axis',(0.,0.342020143325669,0.939692620785908));
#57902=DIRECTION('ref_axis',(1.,0.,0.));
#57903=DIRECTION('',(-0.755033118392644,0.616143911670627,-0.224258043872453));
#57904=DIRECTION('center_axis',(0.,0.5,0.866025403784439));
#57905=DIRECTION('ref_axis',(1.,0.,0.));
#57906=DIRECTION('',(-0.755033118392644,0.567841300538901,-0.327843327723122));
#57907=DIRECTION('center_axis',(0.,0.642787609686539,0.766044443118978));
#57908=DIRECTION('ref_axis',(1.,0.,0.));
#57909=DIRECTION('',(-0.755033118392644,0.502285118831862,-0.421467257957652));
#57910=DIRECTION('center_axis',(0.,0.766044443118978,0.642787609686539));
#57911=DIRECTION('ref_axis',(1.,0.,0.));
#57912=DIRECTION('',(-0.755033118392644,0.421467257957652,-0.502285118831862));
#57913=DIRECTION('center_axis',(0.,0.866025403784439,0.5));
#57914=DIRECTION('ref_axis',(1.,0.,0.));
#57915=DIRECTION('',(-0.755033118392644,0.327843327723121,-0.567841300538901));
#57916=DIRECTION('center_axis',(0.,0.939692620785908,0.342020143325669));
#57917=DIRECTION('ref_axis',(1.,0.,0.));
#57918=DIRECTION('',(-0.755033118392644,0.224258043872452,-0.616143911670627));
#57919=DIRECTION('center_axis',(0.,0.984807753012208,0.17364817766693));
#57920=DIRECTION('ref_axis',(1.,0.,0.));
#57921=DIRECTION('',(-0.755033118392644,0.113858792838765,-0.645725301830105));
#57922=DIRECTION('center_axis',(0.,1.,0.));
#57923=DIRECTION('ref_axis',(1.,0.,0.));
#57924=DIRECTION('',(-0.755033118392644,0.,-0.655686655446243));
#57925=DIRECTION('center_axis',(0.,0.0348994967025008,0.999390827019096));
#57926=DIRECTION('ref_axis',(1.,0.,0.));
#57927=DIRECTION('',(1.,0.,0.));
#57928=DIRECTION('',(-0.137844537491629,0.989850519773593,-0.0345663418323002));
#57929=DIRECTION('center_axis',(-0.99026806874157,-0.137058748836224,0.0241671553619711));
#57930=DIRECTION('ref_axis',(0.,0.17364817766693,0.984807753012208));
#57931=DIRECTION('center_axis',(0.99026806874157,0.137058748836224,-0.0241671553619711));
#57932=DIRECTION('ref_axis',(-0.139173100960066,0.975223671657125,-0.171958245538724));
#57933=DIRECTION('',(-0.137998583506848,0.989505769153514,-0.0428336755604259));
#57934=DIRECTION('center_axis',(-0.0617712249622997,0.0345646215150942,
0.997491655456914));
#57935=DIRECTION('ref_axis',(0.998052578482889,0.0108318757168334,0.0614306198252359));
#57936=DIRECTION('center_axis',(0.0617712249622997,-0.0345646215150942,
-0.997491655456914));
#57937=DIRECTION('ref_axis',(0.998090334472114,0.00213918413755091,0.061734173069449));
#57938=DIRECTION('',(0.0161503784824051,0.999303943318151,-0.0336272827279997));
#57939=DIRECTION('center_axis',(0.284551435696759,0.0276473787012797,0.958262022045047));
#57940=DIRECTION('ref_axis',(0.957826285221151,-0.0498974366850415,-0.282982425517402));
#57941=DIRECTION('center_axis',(-0.284551435696759,-0.0276473787012797,
-0.958262022045047));
#57942=DIRECTION('ref_axis',(-0.958660774436356,0.00820634526047714,0.284433077286297));
#57943=DIRECTION('',(0.0552259184163645,0.997451314500147,-0.0451771306857534));
#57944=DIRECTION('center_axis',(0.491310548314113,0.012242818584528,0.870898420315706));
#57945=DIRECTION('ref_axis',(0.86824314212446,-0.0861536225152694,-0.488601473065054));
#57946=DIRECTION('center_axis',(-0.491310548314113,-0.012242818584528,-0.870898420315706));
#57947=DIRECTION('ref_axis',(-0.870984468928858,0.00690600823120527,0.491262009456283));
#57948=DIRECTION('',(0.057078643955053,0.997299213951626,-0.0462201931597181));
#57949=DIRECTION('center_axis',(0.313150259135957,0.0260751666684335,0.949345564526583));
#57950=DIRECTION('ref_axis',(0.948683298050513,-0.0549123752965087,-0.311423555691114));
#57951=DIRECTION('center_axis',(-0.313150259135957,-0.0260751666684335,
-0.949345564526583));
#57952=DIRECTION('ref_axis',(-0.949703593340092,0.00859788807423112,0.313032204601348));
#57953=DIRECTION('',(0.0225789275220278,0.999136045839184,-0.0348905995476465));
#57954=DIRECTION('center_axis',(0.,0.034899496702501,0.999390827019096));
#57955=DIRECTION('ref_axis',(1.,0.,0.));
#57956=DIRECTION('',(1.,0.,0.));
#57957=DIRECTION('',(-0.0225789275220274,0.999136045839184,-0.0348905995476465));
#57958=DIRECTION('center_axis',(-0.313150259135956,0.0260751666684337,0.949345564526583));
#57959=DIRECTION('ref_axis',(0.948683298050514,0.0549123752965085,0.311423555691113));
#57960=DIRECTION('center_axis',(0.313150259135956,-0.0260751666684337,-0.949345564526583));
#57961=DIRECTION('ref_axis',(0.949703593340092,0.00859788807423116,0.313032204601347));
#57962=DIRECTION('',(-0.0570786439550527,0.997299213951626,-0.046220193159718));
#57963=DIRECTION('center_axis',(-0.491310548314114,0.0122428185845281,0.870898420315705));
#57964=DIRECTION('ref_axis',(0.868243142124459,0.0861536225152696,0.488601473065055));
#57965=DIRECTION('center_axis',(0.491310548314114,-0.0122428185845281,-0.870898420315705));
#57966=DIRECTION('ref_axis',(0.870984468928858,0.0069060082312054,0.491262009456284));
#57967=DIRECTION('',(-0.0552259184163635,0.997451314500147,-0.045177130685753));
#57968=DIRECTION('center_axis',(-0.284551435696759,0.0276473787012796,0.958262022045047));
#57969=DIRECTION('ref_axis',(0.957826285221151,0.0498974366850416,0.282982425517402));
#57970=DIRECTION('center_axis',(0.284551435696759,-0.0276473787012796,-0.958262022045047));
#57971=DIRECTION('ref_axis',(0.958660774436356,0.00820634526047709,0.284433077286297));
#57972=DIRECTION('',(-0.0161503784824052,0.999303943318151,-0.0336272827279996));
#57973=DIRECTION('center_axis',(0.0617712249622996,0.0345646215150941,0.997491655456914));
#57974=DIRECTION('ref_axis',(0.998052578482889,-0.0108318757168334,-0.0614306198252359));
#57975=DIRECTION('center_axis',(-0.0617712249622996,-0.0345646215150941,
-0.997491655456914));
#57976=DIRECTION('ref_axis',(-0.998090334472114,0.0021391841375509,0.061734173069449));
#57977=DIRECTION('',(0.137998583506848,0.989505769153514,-0.0428336755604258));
#57978=DIRECTION('center_axis',(0.99026806874157,-0.137058748836223,0.0241671553619711));
#57979=DIRECTION('ref_axis',(0.,-0.17364817766693,-0.984807753012208));
#57980=DIRECTION('center_axis',(-0.99026806874157,0.137058748836223,-0.0241671553619711));
#57981=DIRECTION('ref_axis',(0.139173100960065,0.975223671657125,-0.171958245538723));
#57982=DIRECTION('',(0.137844537491629,0.989850519773593,-0.0345663418323004));
#57983=DIRECTION('center_axis',(0.,0.034899496702501,0.999390827019096));
#57984=DIRECTION('ref_axis',(1.,0.,0.));
#57985=DIRECTION('',(1.,0.,0.));
#57986=DIRECTION('',(-0.051925424877728,0.998042613992818,-0.0348524160661846));
#57987=DIRECTION('center_axis',(-0.64930555798837,-0.00722457847379232,
0.760493325303574));
#57988=DIRECTION('ref_axis',(0.755033118392644,0.113858792838765,0.645725301830104));
#57989=DIRECTION('center_axis',(0.64930555798837,0.00722457847379232,-0.760493325303574));
#57990=DIRECTION('ref_axis',(-0.760527640763576,0.00616803217361924,-0.649276260934969));
#57991=DIRECTION('center_axis',(0.,-0.309016994374947,-0.951056516295154));
#57992=DIRECTION('ref_axis',(-1.,0.,0.));
#57993=DIRECTION('',(-1.,0.,0.));
#57994=DIRECTION('',(0.137844537491629,0.941977614300068,-0.306067080296576));
#57995=DIRECTION('center_axis',(0.99026806874157,-0.137058748836223,0.0241671553619711));
#57996=DIRECTION('ref_axis',(0.,-0.17364817766693,-0.984807753012208));
#57997=DIRECTION('center_axis',(-0.99026806874157,0.137058748836223,-0.0241671553619711));
#57998=DIRECTION('ref_axis',(0.139173100960065,0.975223671657125,-0.171958245538723));
#57999=DIRECTION('',(0.137998583506848,0.944481249352984,-0.298180416142191));
#58000=DIRECTION('center_axis',(0.0617712249622996,-0.308682119187541,-0.949157344732972));
#58001=DIRECTION('ref_axis',(-0.998052578482889,-0.0108318757168334,-0.0614306198252359));
#58002=DIRECTION('center_axis',(-0.0617712249622996,0.308682119187541,0.949157344732972));
#58003=DIRECTION('ref_axis',(0.998090334472114,0.0191041551727457,0.0587427909490065));
#58004=DIRECTION('',(-0.0161503784824054,0.950539749516609,-0.310182768482997));
#58005=DIRECTION('center_axis',(-0.284551435696759,-0.301764876373726,-0.909927711321104));
#58006=DIRECTION('ref_axis',(-0.957826285221151,0.0498974366850416,0.282982425517402));
#58007=DIRECTION('center_axis',(0.284551435696759,0.301764876373726,0.909927711321104));
#58008=DIRECTION('ref_axis',(-0.958660774436356,0.0895703997751286,0.27008639921553));
#58009=DIRECTION('',(-0.0552259184163638,0.952749128541176,-0.298695825212034));
#58010=DIRECTION('center_axis',(-0.491310548314114,-0.286360316256975,-0.822564109591763));
#58011=DIRECTION('ref_axis',(-0.868243142124459,0.0861536225152696,0.488601473065055));
#58012=DIRECTION('center_axis',(0.491310548314114,0.286360316256975,0.822564109591763));
#58013=DIRECTION('ref_axis',(-0.870984468928858,0.161531977910744,0.463997279083572));
#58014=DIRECTION('',(-0.0570786439550532,0.952962949154956,-0.297663645650825));
#58015=DIRECTION('center_axis',(-0.313150259135956,-0.30019266434088,-0.901011253802641));
#58016=DIRECTION('ref_axis',(-0.948683298050514,0.0549123752965085,0.311423555691113));
#58017=DIRECTION('center_axis',(0.313150259135956,0.30019266434088,0.901011253802641));
#58018=DIRECTION('ref_axis',(-0.949703593340092,0.0989839475056044,0.297094703643677));
#58019=DIRECTION('',(-0.0225789275220273,0.950814057294297,-0.30893821467004));
#58020=DIRECTION('center_axis',(0.,-0.309016994374947,-0.951056516295154));
#58021=DIRECTION('ref_axis',(-1.,0.,0.));
#58022=DIRECTION('',(-1.,0.,0.));
#58023=DIRECTION('',(0.0225789275220281,0.950814057294297,-0.30893821467004));
#58024=DIRECTION('center_axis',(0.313150259135957,-0.30019266434088,-0.901011253802641));
#58025=DIRECTION('ref_axis',(-0.948683298050513,-0.0549123752965087,-0.311423555691114));
#58026=DIRECTION('center_axis',(-0.313150259135957,0.30019266434088,0.901011253802641));
#58027=DIRECTION('ref_axis',(0.949703593340092,0.0989839475056049,0.297094703643678));
#58028=DIRECTION('',(0.0570786439550533,0.952962949154956,-0.297663645650825));
#58029=DIRECTION('center_axis',(0.491310548314113,-0.286360316256975,-0.822564109591764));
#58030=DIRECTION('ref_axis',(-0.86824314212446,-0.0861536225152694,-0.488601473065054));
#58031=DIRECTION('center_axis',(-0.491310548314113,0.286360316256975,0.822564109591764));
#58032=DIRECTION('ref_axis',(0.870984468928858,0.161531977910744,0.463997279083571));
#58033=DIRECTION('',(0.0552259184163649,0.952749128541176,-0.298695825212034));
#58034=DIRECTION('center_axis',(0.284551435696759,-0.301764876373726,-0.909927711321105));
#58035=DIRECTION('ref_axis',(-0.957826285221151,-0.0498974366850415,-0.282982425517402));
#58036=DIRECTION('center_axis',(-0.284551435696759,0.301764876373726,0.909927711321105));
#58037=DIRECTION('ref_axis',(0.958660774436356,0.0895703997751284,0.270086399215529));
#58038=DIRECTION('',(0.0161503784824051,0.950539749516609,-0.310182768482997));
#58039=DIRECTION('center_axis',(-0.0617712249622997,-0.308682119187541,
-0.949157344732972));
#58040=DIRECTION('ref_axis',(-0.998052578482889,0.0108318757168334,0.0614306198252359));
#58041=DIRECTION('center_axis',(0.0617712249622997,0.308682119187541,0.949157344732972));
#58042=DIRECTION('ref_axis',(-0.998090334472114,0.0191041551727457,0.0587427909490066));
#58043=DIRECTION('',(-0.137998583506848,0.944481249352984,-0.298180416142191));
#58044=DIRECTION('center_axis',(-0.99026806874157,-0.137058748836224,0.0241671553619711));
#58045=DIRECTION('ref_axis',(0.,0.17364817766693,0.984807753012208));
#58046=DIRECTION('center_axis',(0.99026806874157,0.137058748836224,-0.0241671553619711));
#58047=DIRECTION('ref_axis',(-0.139173100960066,0.975223671657125,-0.171958245538724));
#58048=DIRECTION('',(-0.137844537491629,0.941977614300068,-0.306067080296576));
#58049=DIRECTION('center_axis',(0.,-0.309016994374948,-0.951056516295154));
#58050=DIRECTION('ref_axis',(-1.,0.,0.));
#58051=DIRECTION('',(-1.,0.,0.));
#58052=DIRECTION('center_axis',(0.,0.984807753012208,-0.17364817766693));
#58053=DIRECTION('ref_axis',(1.,0.,0.));
#58054=DIRECTION('center_axis',(1.,0.,0.));
#58055=DIRECTION('ref_axis',(0.,1.,0.));
#58056=DIRECTION('center_axis',(1.,0.,0.));
#58057=DIRECTION('ref_axis',(0.,0.,-1.));
#58058=DIRECTION('',(-0.707106781186545,0.70710678118655,8.65956056235496E-17));
#58059=DIRECTION('center_axis',(1.,0.,0.));
#58060=DIRECTION('ref_axis',(0.,0.,-1.));
#58061=DIRECTION('center_axis',(1.,0.,0.));
#58062=DIRECTION('ref_axis',(0.,0.,-1.));
#58063=DIRECTION('center_axis',(1.,0.,0.));
#58064=DIRECTION('ref_axis',(0.,0.,-1.));
#58065=DIRECTION('center_axis',(1.,0.,0.));
#58066=DIRECTION('ref_axis',(0.,0.,-1.));
#58067=DIRECTION('center_axis',(1.,0.,0.));
#58068=DIRECTION('ref_axis',(0.,0.,-1.));
#58069=DIRECTION('center_axis',(1.,0.,0.));
#58070=DIRECTION('ref_axis',(0.,0.,-1.));
#58071=DIRECTION('center_axis',(1.,0.,0.));
#58072=DIRECTION('ref_axis',(0.,0.,-1.));
#58073=DIRECTION('center_axis',(1.,0.,0.));
#58074=DIRECTION('ref_axis',(0.,0.,-1.));
#58075=DIRECTION('center_axis',(1.,0.,0.));
#58076=DIRECTION('ref_axis',(0.,0.,-1.));
#58077=DIRECTION('center_axis',(1.,0.,0.));
#58078=DIRECTION('ref_axis',(0.,0.,-1.));
#58079=DIRECTION('center_axis',(1.,0.,0.));
#58080=DIRECTION('ref_axis',(0.,0.,-1.));
#58081=DIRECTION('center_axis',(1.,0.,0.));
#58082=DIRECTION('ref_axis',(0.,0.,-1.));
#58083=DIRECTION('center_axis',(1.,0.,0.));
#58084=DIRECTION('ref_axis',(0.,0.,-1.));
#58085=DIRECTION('center_axis',(1.,0.,0.));
#58086=DIRECTION('ref_axis',(0.,0.,-1.));
#58087=DIRECTION('center_axis',(1.,0.,0.));
#58088=DIRECTION('ref_axis',(0.,0.,-1.));
#58089=DIRECTION('center_axis',(1.,0.,0.));
#58090=DIRECTION('ref_axis',(0.,0.,-1.));
#58091=DIRECTION('center_axis',(1.,0.,0.));
#58092=DIRECTION('ref_axis',(0.,0.,-1.));
#58093=DIRECTION('center_axis',(1.,0.,0.));
#58094=DIRECTION('ref_axis',(0.,0.,-1.));
#58095=DIRECTION('center_axis',(1.,0.,0.));
#58096=DIRECTION('ref_axis',(0.,0.,-1.));
#58097=DIRECTION('center_axis',(1.,0.,0.));
#58098=DIRECTION('ref_axis',(0.,0.,-1.));
#58099=DIRECTION('center_axis',(1.,0.,0.));
#58100=DIRECTION('ref_axis',(0.,0.,-1.));
#58101=DIRECTION('center_axis',(1.,0.,0.));
#58102=DIRECTION('ref_axis',(0.,0.,-1.));
#58103=DIRECTION('center_axis',(1.,0.,0.));
#58104=DIRECTION('ref_axis',(0.,0.,-1.));
#58105=DIRECTION('center_axis',(1.,0.,0.));
#58106=DIRECTION('ref_axis',(0.,0.,-1.));
#58107=DIRECTION('center_axis',(1.,0.,0.));
#58108=DIRECTION('ref_axis',(0.,0.,-1.));
#58109=DIRECTION('center_axis',(1.,0.,0.));
#58110=DIRECTION('ref_axis',(0.,0.,-1.));
#58111=DIRECTION('center_axis',(1.,0.,0.));
#58112=DIRECTION('ref_axis',(0.,0.,-1.));
#58113=DIRECTION('center_axis',(1.,0.,0.));
#58114=DIRECTION('ref_axis',(0.,0.,-1.));
#58115=DIRECTION('center_axis',(1.,0.,0.));
#58116=DIRECTION('ref_axis',(0.,0.,-1.));
#58117=DIRECTION('center_axis',(1.,0.,0.));
#58118=DIRECTION('ref_axis',(0.,0.,-1.));
#58119=DIRECTION('center_axis',(1.,0.,0.));
#58120=DIRECTION('ref_axis',(0.,0.,-1.));
#58121=DIRECTION('center_axis',(1.,0.,0.));
#58122=DIRECTION('ref_axis',(0.,0.,-1.));
#58123=DIRECTION('center_axis',(1.,0.,0.));
#58124=DIRECTION('ref_axis',(0.,0.,-1.));
#58125=DIRECTION('center_axis',(1.,0.,0.));
#58126=DIRECTION('ref_axis',(0.,0.,-1.));
#58127=DIRECTION('center_axis',(1.,0.,0.));
#58128=DIRECTION('ref_axis',(0.,0.,-1.));
#58129=DIRECTION('center_axis',(1.,0.,0.));
#58130=DIRECTION('ref_axis',(0.,0.,-1.));
#58131=DIRECTION('center_axis',(1.,0.,0.));
#58132=DIRECTION('ref_axis',(0.,1.,0.));
#58133=DIRECTION('center_axis',(1.,0.,0.));
#58134=DIRECTION('ref_axis',(0.,0.,-1.));
#58135=DIRECTION('center_axis',(0.649305557988371,-0.124943459173594,-0.75019425775938));
#58136=DIRECTION('ref_axis',(0.760527640763576,0.106671313608347,0.640483363162275));
#58137=DIRECTION('',(1.,0.,0.));
#58138=DIRECTION('center_axis',(-0.99026806874157,0.130779935984066,-0.0476000039374394));
#58139=DIRECTION('ref_axis',(0.139173100960065,0.930547596796367,-0.338691626801824));
#58140=DIRECTION('center_axis',(-0.0617712249622996,-0.207252115456061,
-0.976335432321108));
#58141=DIRECTION('ref_axis',(-0.998090334472114,0.0128267117770656,0.0604248268374111));
#58142=DIRECTION('center_axis',(0.284551435696759,-0.193627806751036,-0.938902951798372));
#58143=DIRECTION('ref_axis',(0.958660774436356,0.0574729579753757,0.278686882824878));
#58144=DIRECTION('center_axis',(0.491310548314114,-0.163286746281596,-0.855541573276281));
#58145=DIRECTION('ref_axis',(0.870984468928858,0.0921078431475356,0.482599419928604));
#58146=DIRECTION('center_axis',(0.313150259135956,-0.190531153552384,-0.930394967059196));
#58147=DIRECTION('ref_axis',(0.949703593340092,0.0628247387151198,0.306783534438035));
#58148=DIRECTION('',(1.,0.,0.));
#58149=DIRECTION('center_axis',(-0.313150259135957,-0.190531153552384,-0.930394967059195));
#58150=DIRECTION('ref_axis',(-0.949703593340092,0.0628247387151199,0.306783534438037));
#58151=DIRECTION('center_axis',(-0.491310548314113,-0.163286746281596,-0.855541573276282));
#58152=DIRECTION('ref_axis',(-0.870984468928858,0.0921078431475352,0.482599419928602));
#58153=DIRECTION('center_axis',(-0.284551435696759,-0.193627806751036,-0.938902951798373));
#58154=DIRECTION('ref_axis',(-0.958660774436356,0.0574729579753756,0.278686882824878));
#58155=DIRECTION('center_axis',(0.0617712249622997,-0.207252115456061,-0.976335432321108));
#58156=DIRECTION('ref_axis',(0.998090334472114,0.0128267117770656,0.0604248268374111));
#58157=DIRECTION('center_axis',(0.99026806874157,0.130779935984066,-0.0476000039374395));
#58158=DIRECTION('ref_axis',(-0.139173100960066,0.930547596796366,-0.338691626801825));
#58159=DIRECTION('',(1.,0.,0.));
#58160=DIRECTION('center_axis',(0.,0.20791169081776,0.978147600733805));
#58161=DIRECTION('ref_axis',(1.,0.,0.));
#58162=DIRECTION('',(-0.137844537491629,0.968810083928407,-0.205926940351068));
#58163=DIRECTION('center_axis',(-0.99026806874157,-0.130779935984066,0.0476000039374395));
#58164=DIRECTION('ref_axis',(0.,0.342020143325669,0.939692620785908));
#58165=DIRECTION('',(-0.137998583506848,0.967034963408844,-0.21400880938634));
#58166=DIRECTION('center_axis',(-0.0617712249622997,0.207252115456061,0.976335432321108));
#58167=DIRECTION('ref_axis',(0.998052578482889,0.0213346303712045,0.0586164151972949));
#58168=DIRECTION('',(0.0161503784824051,0.978282954629779,-0.206643717435843));
#58169=DIRECTION('center_axis',(0.284551435696759,0.193627806751036,0.938902951798373));
#58170=DIRECTION('ref_axis',(0.957826285221151,-0.0982787650057295,-0.270018687665128));
#58171=DIRECTION('',(0.0552259184163645,0.974452861356161,-0.217696391632611));
#58172=DIRECTION('center_axis',(0.491310548314113,0.163286746281596,0.855541573276282));
#58173=DIRECTION('ref_axis',(0.86824314212446,-0.169689510806249,-0.46621809925847));
#58174=DIRECTION('',(0.057078643955053,0.974121945658943,-0.218697195660775));
#58175=DIRECTION('center_axis',(0.313150259135957,0.190531153552384,0.930394967059195));
#58176=DIRECTION('ref_axis',(0.948683298050513,-0.108156265856636,-0.297156898213637));
#58177=DIRECTION('',(0.0225789275220278,0.977898235227234,-0.207858686543084));
#58178=DIRECTION('center_axis',(0.,0.20791169081776,0.978147600733805));
#58179=DIRECTION('ref_axis',(1.,0.,0.));
#58180=DIRECTION('',(-0.0225789275220274,0.977898235227234,-0.207858686543084));
#58181=DIRECTION('center_axis',(-0.313150259135956,0.190531153552384,0.930394967059196));
#58182=DIRECTION('ref_axis',(0.948683298050514,0.108156265856635,0.297156898213636));
#58183=DIRECTION('',(-0.0570786439550527,0.974121945658943,-0.218697195660775));
#58184=DIRECTION('center_axis',(-0.491310548314114,0.163286746281596,0.855541573276281));
#58185=DIRECTION('ref_axis',(0.868243142124459,0.16968951080625,0.466218099258471));
#58186=DIRECTION('',(-0.0552259184163635,0.974452861356161,-0.217696391632611));
#58187=DIRECTION('center_axis',(-0.284551435696759,0.193627806751036,0.938902951798372));
#58188=DIRECTION('ref_axis',(0.957826285221151,0.0982787650057297,0.270018687665129));
#58189=DIRECTION('',(-0.0161503784824052,0.978282954629779,-0.206643717435843));
#58190=DIRECTION('center_axis',(0.0617712249622996,0.207252115456061,0.976335432321108));
#58191=DIRECTION('ref_axis',(0.998052578482889,-0.0213346303712045,-0.0586164151972949));
#58192=DIRECTION('',(0.137998583506848,0.967034963408844,-0.21400880938634));
#58193=DIRECTION('center_axis',(0.99026806874157,-0.130779935984066,0.0476000039374394));
#58194=DIRECTION('ref_axis',(0.,-0.342020143325669,-0.939692620785908));
#58195=DIRECTION('',(0.137844537491629,0.968810083928407,-0.205926940351068));
#58196=DIRECTION('center_axis',(0.,0.20791169081776,0.978147600733805));
#58197=DIRECTION('ref_axis',(1.,0.,0.));
#58198=DIRECTION('',(-0.0519254248777279,0.976828045559515,-0.207631210706979));
#58199=DIRECTION('center_axis',(-0.649305557988371,0.124943459173594,0.75019425775938));
#58200=DIRECTION('ref_axis',(0.755033118392644,0.224258043872453,0.616143911670627));
#58201=DIRECTION('center_axis',(0.,-0.469471562785891,-0.882947592858927));
#58202=DIRECTION('ref_axis',(-1.,0.,0.));
#58203=DIRECTION('',(-1.,0.,0.));
#58204=DIRECTION('',(0.137844537491629,0.874518866989312,-0.464989929744128));
#58205=DIRECTION('center_axis',(0.99026806874157,-0.130779935984066,0.0476000039374394));
#58206=DIRECTION('ref_axis',(0.,-0.342020143325669,-0.939692620785908));
#58207=DIRECTION('center_axis',(-0.99026806874157,0.130779935984066,-0.0476000039374394));
#58208=DIRECTION('ref_axis',(0.139173100960065,0.930547596796367,-0.338691626801824));
#58209=DIRECTION('',(0.137998583506848,0.878353971058416,-0.457657833403968));
#58210=DIRECTION('center_axis',(0.0617712249622996,-0.468811987424192,-0.881135424446229));
#58211=DIRECTION('ref_axis',(-0.998052578482889,-0.0213346303712045,-0.0586164151972949));
#58212=DIRECTION('center_axis',(-0.0617712249622996,0.468811987424192,0.881135424446229));
#58213=DIRECTION('ref_axis',(0.998090334472114,0.0290144987282327,0.0545329542285434));
#58214=DIRECTION('',(-0.0161503784824054,0.882236242379483,-0.470529890556387));
#58215=DIRECTION('center_axis',(-0.284551435696759,-0.455187678719167,-0.843702943923493));
#58216=DIRECTION('ref_axis',(-0.957826285221151,0.0982787650057297,0.270018687665129));
#58217=DIRECTION('center_axis',(0.284551435696759,0.455187678719167,0.843702943923493));
#58218=DIRECTION('ref_axis',(-0.958660774436356,0.13510963517535,0.250429443236754));
#58219=DIRECTION('',(-0.0552259184163638,0.886406742738185,-0.459601114406123));
#58220=DIRECTION('center_axis',(-0.491310548314114,-0.424846618249728,-0.760341565401402));
#58221=DIRECTION('ref_axis',(-0.868243142124459,0.16968951080625,0.466218099258471));
#58222=DIRECTION('center_axis',(0.491310548314114,0.424846618249728,0.760341565401402));
#58223=DIRECTION('ref_axis',(-0.870984468928858,0.239650226161174,0.428898384218936));
#58224=DIRECTION('',(-0.0570786439550532,0.886796551036219,-0.458621745531674));
#58225=DIRECTION('center_axis',(-0.313150259135956,-0.452091025520515,-0.835194959184317));
#58226=DIRECTION('ref_axis',(-0.948683298050514,0.108156265856635,0.297156898213636));
#58227=DIRECTION('center_axis',(0.313150259135956,0.452091025520515,0.835194959184317));
#58228=DIRECTION('ref_axis',(-0.949703593340092,0.149070112809494,0.27539278542453));
#58229=DIRECTION('',(-0.0225789275220273,0.88272249730729,-0.469351877358061));
#58230=DIRECTION('center_axis',(0.,-0.469471562785891,-0.882947592858927));
#58231=DIRECTION('ref_axis',(-1.,0.,0.));
#58232=DIRECTION('',(-1.,0.,0.));
#58233=DIRECTION('',(0.0225789275220281,0.88272249730729,-0.469351877358061));
#58234=DIRECTION('center_axis',(0.313150259135957,-0.452091025520515,-0.835194959184316));
#58235=DIRECTION('ref_axis',(-0.948683298050513,-0.108156265856636,-0.297156898213637));
#58236=DIRECTION('center_axis',(-0.313150259135957,0.452091025520515,0.835194959184316));
#58237=DIRECTION('ref_axis',(0.949703593340092,0.149070112809495,0.275392785424531));
#58238=DIRECTION('',(0.0570786439550534,0.886796551036219,-0.458621745531674));
#58239=DIRECTION('center_axis',(0.491310548314113,-0.424846618249728,-0.760341565401403));
#58240=DIRECTION('ref_axis',(-0.86824314212446,-0.169689510806249,-0.46621809925847));
#58241=DIRECTION('center_axis',(-0.491310548314113,0.424846618249728,0.760341565401403));
#58242=DIRECTION('ref_axis',(0.870984468928858,0.239650226161174,0.428898384218935));
#58243=DIRECTION('',(0.0552259184163649,0.886406742738185,-0.459601114406122));
#58244=DIRECTION('center_axis',(0.284551435696759,-0.455187678719167,-0.843702943923494));
#58245=DIRECTION('ref_axis',(-0.957826285221151,-0.0982787650057295,-0.270018687665128));
#58246=DIRECTION('center_axis',(-0.284551435696759,0.455187678719167,0.843702943923494));
#58247=DIRECTION('ref_axis',(0.958660774436356,0.135109635175349,0.250429443236754));
#58248=DIRECTION('',(0.0161503784824051,0.882236242379483,-0.470529890556387));
#58249=DIRECTION('center_axis',(-0.0617712249622997,-0.468811987424192,
-0.881135424446229));
#58250=DIRECTION('ref_axis',(-0.998052578482889,0.0213346303712045,0.0586164151972949));
#58251=DIRECTION('center_axis',(0.0617712249622997,0.468811987424192,0.881135424446229));
#58252=DIRECTION('ref_axis',(-0.998090334472114,0.0290144987282328,0.0545329542285435));
#58253=DIRECTION('',(-0.137998583506848,0.878353971058416,-0.457657833403968));
#58254=DIRECTION('center_axis',(-0.99026806874157,-0.130779935984066,0.0476000039374395));
#58255=DIRECTION('ref_axis',(0.,0.342020143325669,0.939692620785908));
#58256=DIRECTION('center_axis',(0.99026806874157,0.130779935984066,-0.0476000039374395));
#58257=DIRECTION('ref_axis',(-0.139173100960066,0.930547596796366,-0.338691626801825));
#58258=DIRECTION('',(-0.137844537491629,0.874518866989312,-0.464989929744128));
#58259=DIRECTION('center_axis',(0.,-0.469471562785892,-0.882947592858927));
#58260=DIRECTION('ref_axis',(-1.,0.,0.));
#58261=DIRECTION('',(-1.,0.,0.));
#58262=DIRECTION('center_axis',(0.,0.939692620785908,-0.342020143325669));
#58263=DIRECTION('ref_axis',(1.,0.,0.));
#58264=DIRECTION('center_axis',(1.,0.,0.));
#58265=DIRECTION('ref_axis',(0.,1.,0.));
#58266=DIRECTION('center_axis',(1.,0.,0.));
#58267=DIRECTION('ref_axis',(0.,0.,-1.));
#58268=DIRECTION('center_axis',(0.64930555798837,-0.253315153038432,-0.717100917309779));
#58269=DIRECTION('ref_axis',(0.760527640763576,0.216269505504613,0.612229702500115));
#58270=DIRECTION('',(1.,0.,0.));
#58271=DIRECTION('center_axis',(-0.99026806874157,0.120527440954873,-0.0695865504800327));
#58272=DIRECTION('ref_axis',(0.139173100960065,0.857597304086756,-0.495134034370783));
#58273=DIRECTION('center_axis',(-0.0617712249622996,-0.373642358743525,
-0.925513751123792));
#58274=DIRECTION('ref_axis',(-0.998090334472114,0.0231245062698635,0.0572795028183562));
#58275=DIRECTION('center_axis',(0.284551435696759,-0.353724951873058,-0.891015790469123));
#58276=DIRECTION('ref_axis',(0.958660774436356,0.104993283944912,0.264472928451193));
#58277=DIRECTION('center_axis',(0.491310548314114,-0.309369288819978,-0.814189528457782));
#58278=DIRECTION('ref_axis',(0.870984468928858,0.174511027858645,0.459273291233482));
#58279=DIRECTION('center_axis',(0.313150259135956,-0.34919794774906,-0.883174789320284));
#58280=DIRECTION('ref_axis',(0.949703593340092,0.115142691461001,0.291213401820783));
#58281=DIRECTION('',(1.,0.,0.));
#58282=DIRECTION('center_axis',(-0.313150259135957,-0.34919794774906,-0.883174789320284));
#58283=DIRECTION('ref_axis',(-0.949703593340092,0.115142691461001,0.291213401820784));
#58284=DIRECTION('center_axis',(-0.491310548314113,-0.309369288819978,-0.814189528457783));
#58285=DIRECTION('ref_axis',(-0.870984468928858,0.174511027858645,0.459273291233481));
#58286=DIRECTION('center_axis',(-0.284551435696759,-0.353724951873058,-0.891015790469123));
#58287=DIRECTION('ref_axis',(-0.958660774436356,0.104993283944912,0.264472928451192));
#58288=DIRECTION('center_axis',(0.0617712249622997,-0.373642358743525,-0.925513751123792));
#58289=DIRECTION('ref_axis',(0.998090334472114,0.0231245062698635,0.0572795028183562));
#58290=DIRECTION('center_axis',(0.99026806874157,0.120527440954873,-0.0695865504800329));
#58291=DIRECTION('ref_axis',(-0.139173100960066,0.857597304086755,-0.495134034370784));
#58292=DIRECTION('',(1.,0.,0.));
#58293=DIRECTION('center_axis',(0.,0.374606593415912,0.927183854566787));
#58294=DIRECTION('ref_axis',(1.,0.,0.));
#58295=DIRECTION('',(-0.137844537491629,0.918332843924613,-0.371030552991328));
#58296=DIRECTION('center_axis',(-0.99026806874157,-0.120527440954873,0.0695865504800329));
#58297=DIRECTION('ref_axis',(0.,0.5,0.866025403784438));
#58298=DIRECTION('',(-0.137998583506848,0.9151812896443,-0.378681393832731));
#58299=DIRECTION('center_axis',(-0.0617712249622997,0.373642358743525,0.925513751123792));
#58300=DIRECTION('ref_axis',(0.998052578482889,0.0311891430775903,0.0540211804549215));
#58301=DIRECTION('',(0.0161503784824051,0.927537333400043,-0.373381387356163));
#58302=DIRECTION('center_axis',(0.284551435696759,0.353724951873058,0.891015790469123));
#58303=DIRECTION('ref_axis',(0.957826285221151,-0.143673942783173,-0.248850568624199));
#58304=DIRECTION('',(0.0552259184163645,0.921846151116809,-0.383601057879401));
#58305=DIRECTION('center_axis',(0.491310548314113,0.309369288819978,0.814189528457783));
#58306=DIRECTION('ref_axis',(0.86824314212446,-0.248069469178416,-0.429668924423658));
#58307=DIRECTION('',(0.057078643955053,0.921346474976903,-0.384529194537799));
#58308=DIRECTION('center_axis',(0.313150259135957,0.34919794774906,0.883174789320284));
#58309=DIRECTION('ref_axis',(0.948683298050513,-0.15811388300842,-0.273861278752584));
#58310=DIRECTION('',(0.0225789275220278,0.926947481578288,-0.37451109252948));
#58311=DIRECTION('center_axis',(0.,0.374606593415913,0.927183854566787));
#58312=DIRECTION('ref_axis',(1.,0.,0.));
#58313=DIRECTION('',(-0.0225789275220274,0.926947481578288,-0.37451109252948));
#58314=DIRECTION('center_axis',(-0.313150259135956,0.34919794774906,0.883174789320284));
#58315=DIRECTION('ref_axis',(0.948683298050514,0.158113883008419,0.273861278752584));
#58316=DIRECTION('',(-0.0570786439550527,0.921346474976903,-0.384529194537799));
#58317=DIRECTION('center_axis',(-0.491310548314114,0.309369288819978,0.814189528457782));
#58318=DIRECTION('ref_axis',(0.86824314212446,0.248069469178417,0.429668924423659));
#58319=DIRECTION('',(-0.0552259184163635,0.921846151116809,-0.3836010578794));
#58320=DIRECTION('center_axis',(-0.284551435696759,0.353724951873058,0.891015790469123));
#58321=DIRECTION('ref_axis',(0.957826285221151,0.143673942783173,0.248850568624199));
#58322=DIRECTION('',(-0.0161503784824052,0.927537333400043,-0.373381387356163));
#58323=DIRECTION('center_axis',(0.0617712249622996,0.373642358743525,0.925513751123792));
#58324=DIRECTION('ref_axis',(0.998052578482889,-0.0311891430775903,-0.0540211804549214));
#58325=DIRECTION('',(0.137998583506848,0.9151812896443,-0.378681393832731));
#58326=DIRECTION('center_axis',(0.99026806874157,-0.120527440954873,0.0695865504800327));
#58327=DIRECTION('ref_axis',(0.,-0.5,-0.866025403784438));
#58328=DIRECTION('',(0.137844537491629,0.918332843924613,-0.371030552991328));
#58329=DIRECTION('center_axis',(0.,0.374606593415913,0.927183854566787));
#58330=DIRECTION('ref_axis',(1.,0.,0.));
#58331=DIRECTION('',(-0.051925424877728,0.925933051260727,-0.374101236076903));
#58332=DIRECTION('center_axis',(-0.64930555798837,0.253315153038432,0.717100917309779));
#58333=DIRECTION('ref_axis',(0.755033118392644,0.327843327723122,0.567841300538901));
#58334=DIRECTION('center_axis',(0.,-0.615661475325659,-0.788010753606722));
#58335=DIRECTION('ref_axis',(-1.,0.,0.));
#58336=DIRECTION('',(-1.,0.,0.));
#58337=DIRECTION('',(0.137844537491629,0.780488306432985,-0.609784295472662));
#58338=DIRECTION('center_axis',(0.99026806874157,-0.120527440954873,0.0695865504800328));
#58339=DIRECTION('ref_axis',(0.,-0.5,-0.866025403784438));
#58340=DIRECTION('center_axis',(-0.99026806874157,0.120527440954873,-0.0695865504800328));
#58341=DIRECTION('ref_axis',(0.139173100960065,0.857597304086756,-0.495134034370783));
#58342=DIRECTION('',(0.137998583506848,0.785538351821794,-0.603229548983803));
#58343=DIRECTION('center_axis',(0.0617712249622996,-0.614697240653271,-0.786340650163726));
#58344=DIRECTION('ref_axis',(-0.998052578482889,-0.0311891430775903,-0.0540211804549214));
#58345=DIRECTION('center_axis',(-0.0617712249622996,0.614697240653271,0.786340650163726));
#58346=DIRECTION('ref_axis',(0.998090334472114,0.0380432514219071,0.0486661612888523));
#58347=DIRECTION('',(-0.0161503784824054,0.787126433450736,-0.616580200004833));
#58348=DIRECTION('center_axis',(-0.284551435696759,-0.594779833782805,-0.751842689509057));
#58349=DIRECTION('ref_axis',(-0.957826285221151,0.143673942783173,0.248850568624199));
#58350=DIRECTION('center_axis',(0.284551435696759,0.594779833782805,0.751842689509057));
#58351=DIRECTION('ref_axis',(-0.958660774436356,0.176543632679542,0.223163315348643));
#58352=DIRECTION('',(-0.0552259184163638,0.793131336600549,-0.606541656308366));
#58353=DIRECTION('center_axis',(-0.491310548314114,-0.550424170729724,-0.675016427497717));
#58354=DIRECTION('ref_axis',(-0.86824314212446,0.248069469178417,0.429668924423659));
#58355=DIRECTION('center_axis',(0.491310548314114,0.550424170729724,0.675016427497717));
#58356=DIRECTION('ref_axis',(-0.870984468928858,0.310486823558562,0.380767628982861));
#58357=DIRECTION('',(-0.0570786439550532,0.793685288454953,-0.605644855748342));
#58358=DIRECTION('center_axis',(-0.313150259135956,-0.590252829658806,-0.744001688360219));
#58359=DIRECTION('ref_axis',(-0.948683298050514,0.158113883008419,0.273861278752584));
#58360=DIRECTION('center_axis',(0.313150259135956,0.590252829658806,0.744001688360219));
#58361=DIRECTION('ref_axis',(-0.949703593340092,0.194626858168784,0.245323196775732));
#58362=DIRECTION('',(-0.0225789275220273,0.787809860918737,-0.615504520756066));
#58363=DIRECTION('center_axis',(0.,-0.615661475325659,-0.788010753606722));
#58364=DIRECTION('ref_axis',(-1.,0.,0.));
#58365=DIRECTION('',(-1.,0.,0.));
#58366=DIRECTION('',(0.0225789275220281,0.787809860918737,-0.615504520756066));
#58367=DIRECTION('center_axis',(0.313150259135957,-0.590252829658806,-0.744001688360218));
#58368=DIRECTION('ref_axis',(-0.948683298050513,-0.15811388300842,-0.273861278752584));
#58369=DIRECTION('center_axis',(-0.313150259135957,0.590252829658806,0.744001688360218));
#58370=DIRECTION('ref_axis',(0.949703593340092,0.194626858168784,0.245323196775733));
#58371=DIRECTION('',(0.0570786439550533,0.793685288454953,-0.605644855748343));
#58372=DIRECTION('center_axis',(0.491310548314113,-0.550424170729725,-0.675016427497717));
#58373=DIRECTION('ref_axis',(-0.86824314212446,-0.248069469178416,-0.429668924423658));
#58374=DIRECTION('center_axis',(-0.491310548314113,0.550424170729725,0.675016427497717));
#58375=DIRECTION('ref_axis',(0.870984468928858,0.310486823558562,0.38076762898286));
#58376=DIRECTION('',(0.0552259184163649,0.793131336600549,-0.606541656308365));
#58377=DIRECTION('center_axis',(0.284551435696759,-0.594779833782805,-0.751842689509057));
#58378=DIRECTION('ref_axis',(-0.957826285221151,-0.143673942783173,-0.248850568624199));
#58379=DIRECTION('center_axis',(-0.284551435696759,0.594779833782805,0.751842689509057));
#58380=DIRECTION('ref_axis',(0.958660774436356,0.176543632679541,0.223163315348643));
#58381=DIRECTION('',(0.0161503784824051,0.787126433450736,-0.616580200004833));
#58382=DIRECTION('center_axis',(-0.0617712249622997,-0.614697240653271,
-0.786340650163726));
#58383=DIRECTION('ref_axis',(-0.998052578482889,0.0311891430775903,0.0540211804549215));
#58384=DIRECTION('center_axis',(0.0617712249622997,0.614697240653271,0.786340650163726));
#58385=DIRECTION('ref_axis',(-0.998090334472114,0.0380432514219072,0.0486661612888524));
#58386=DIRECTION('',(-0.137998583506848,0.785538351821794,-0.603229548983803));
#58387=DIRECTION('center_axis',(-0.99026806874157,-0.120527440954873,0.0695865504800329));
#58388=DIRECTION('ref_axis',(0.,0.5,0.866025403784438));
#58389=DIRECTION('center_axis',(0.99026806874157,0.120527440954873,-0.0695865504800329));
#58390=DIRECTION('ref_axis',(-0.139173100960066,0.857597304086755,-0.495134034370784));
#58391=DIRECTION('',(-0.137844537491629,0.780488306432985,-0.609784295472662));
#58392=DIRECTION('center_axis',(0.,-0.615661475325659,-0.788010753606722));
#58393=DIRECTION('ref_axis',(-1.,0.,0.));
#58394=DIRECTION('',(-1.,0.,0.));
#58395=DIRECTION('center_axis',(0.,0.866025403784438,-0.5));
#58396=DIRECTION('ref_axis',(1.,0.,0.));
#58397=DIRECTION('center_axis',(1.,0.,0.));
#58398=DIRECTION('ref_axis',(0.,1.,0.));
#58399=DIRECTION('center_axis',(1.,0.,0.));
#58400=DIRECTION('ref_axis',(0.,0.,-1.));
#58401=DIRECTION('center_axis',(0.64930555798837,-0.373989994161849,-0.662218828358294));
#58402=DIRECTION('ref_axis',(0.760527640763576,0.319296457913771,0.565373752130667));
#58403=DIRECTION('',(1.,0.,0.));
#58404=DIRECTION('center_axis',(-0.99026806874157,0.106612780622095,-0.0894587448987839));
#58405=DIRECTION('ref_axis',(0.139173100960065,0.758589351257639,-0.636532044855303));
#58406=DIRECTION('center_axis',(-0.0617712249622996,-0.528679668032723,
-0.846570802931135));
#58407=DIRECTION('ref_axis',(-0.998090334472114,0.0327196743412163,0.0523937700909925));
#58408=DIRECTION('center_axis',(0.284551435696759,-0.50307434332588,-0.816055565222214));
#58409=DIRECTION('ref_axis',(0.958660774436356,0.149323442110948,0.242223097976277));
#58410=DIRECTION('center_axis',(0.491310548314114,-0.446051802065978,-0.748098746816874));
#58411=DIRECTION('ref_axis',(0.870984468928858,0.25161178329511,0.42199237598773));
#58412=DIRECTION('center_axis',(0.313150259135956,-0.497254539006069,-0.809119792515883));
#58413=DIRECTION('ref_axis',(0.949703593340092,0.163962091791853,0.266794897350299));
#58414=DIRECTION('',(1.,0.,0.));
#58415=DIRECTION('center_axis',(-0.313150259135957,-0.497254539006068,-0.809119792515883));
#58416=DIRECTION('ref_axis',(-0.949703593340092,0.163962091791853,0.2667948973503));
#58417=DIRECTION('center_axis',(-0.491310548314113,-0.446051802065979,-0.748098746816875));
#58418=DIRECTION('ref_axis',(-0.870984468928858,0.25161178329511,0.421992375987729));
#58419=DIRECTION('center_axis',(-0.284551435696759,-0.503074343325881,-0.816055565222214));
#58420=DIRECTION('ref_axis',(-0.958660774436356,0.149323442110948,0.242223097976277));
#58421=DIRECTION('center_axis',(0.0617712249622997,-0.528679668032723,-0.846570802931135));
#58422=DIRECTION('ref_axis',(0.998090334472114,0.0327196743412163,0.0523937700909926));
#58423=DIRECTION('center_axis',(0.99026806874157,0.106612780622095,-0.0894587448987841));
#58424=DIRECTION('ref_axis',(-0.139173100960066,0.758589351257642,-0.636532044855299));
#58425=DIRECTION('',(1.,0.,0.));
#58426=DIRECTION('center_axis',(0.,0.529919264233205,0.848048096156426));
#58427=DIRECTION('ref_axis',(1.,0.,0.));
#58428=DIRECTION('',(-0.137844537491629,0.839952525157012,-0.524860590029465));
#58429=DIRECTION('center_axis',(-0.99026806874157,-0.106612780622095,0.0894587448987841));
#58430=DIRECTION('ref_axis',(0.,0.64278760968654,0.766044443118978));
#58431=DIRECTION('',(-0.137998583506848,0.835520295497991,-0.531847935749547));
#58432=DIRECTION('center_axis',(-0.0617712249622997,0.528679668032723,0.846570802931135));
#58433=DIRECTION('ref_axis',(0.998052578482889,0.0400959894540315,0.0477845394804615));
#58434=DIRECTION('',(0.0161503784824051,0.848608959651483,-0.528774052761765));
#58435=DIRECTION('center_axis',(0.284551435696759,0.503074343325881,0.816055565222214));
#58436=DIRECTION('ref_axis',(0.957826285221151,-0.184703660511672,-0.220121250980087));
#58437=DIRECTION('',(0.0552259184163645,0.841229612052432,-0.537850200094026));
#58438=DIRECTION('center_axis',(0.491310548314113,0.446051802065979,0.748098746816875));
#58439=DIRECTION('ref_axis',(0.86824314212446,-0.318911962258806,-0.3800644767432));
#58440=DIRECTION('',(0.057078643955053,0.840576357876501,-0.538677468419953));
#58441=DIRECTION('center_axis',(0.313150259135957,0.497254539006068,0.809119792515883));
#58442=DIRECTION('ref_axis',(0.948683298050513,-0.203267289834479,-0.242244522917128));
#58443=DIRECTION('',(0.0225789275220278,0.847831897759644,-0.529784168481124));
#58444=DIRECTION('center_axis',(0.,0.529919264233205,0.848048096156426));
#58445=DIRECTION('ref_axis',(1.,0.,0.));
#58446=DIRECTION('',(-0.0225789275220274,0.847831897759644,-0.529784168481124));
#58447=DIRECTION('center_axis',(-0.313150259135956,0.497254539006069,0.809119792515883));
#58448=DIRECTION('ref_axis',(0.948683298050514,0.203267289834478,0.242244522917128));
#58449=DIRECTION('',(-0.0570786439550527,0.840576357876501,-0.538677468419953));
#58450=DIRECTION('center_axis',(-0.491310548314114,0.446051802065978,0.748098746816874));
#58451=DIRECTION('ref_axis',(0.86824314212446,0.318911962258806,0.380064476743201));
#58452=DIRECTION('',(-0.0552259184163635,0.841229612052432,-0.537850200094025));
#58453=DIRECTION('center_axis',(-0.284551435696759,0.50307434332588,0.816055565222214));
#58454=DIRECTION('ref_axis',(0.957826285221151,0.184703660511673,0.220121250980087));
#58455=DIRECTION('',(-0.0161503784824052,0.848608959651484,-0.528774052761765));
#58456=DIRECTION('center_axis',(0.0617712249622996,0.528679668032723,0.846570802931135));
#58457=DIRECTION('ref_axis',(0.998052578482889,-0.0400959894540314,-0.0477845394804615));
#58458=DIRECTION('',(0.137998583506848,0.835520295497991,-0.531847935749547));
#58459=DIRECTION('center_axis',(0.99026806874157,-0.106612780622095,0.0894587448987839));
#58460=DIRECTION('ref_axis',(0.,-0.64278760968654,-0.766044443118978));
#58461=DIRECTION('',(0.137844537491629,0.839952525157012,-0.524860590029466));
#58462=DIRECTION('center_axis',(0.,0.529919264233205,0.848048096156426));
#58463=DIRECTION('ref_axis',(1.,0.,0.));
#58464=DIRECTION('',(-0.051925424877728,0.846904049744114,-0.52920438469299));
#58465=DIRECTION('center_axis',(-0.64930555798837,0.373989994161849,0.662218828358294));
#58466=DIRECTION('ref_axis',(0.755033118392644,0.421467257957652,0.502285118831862));
#58467=DIRECTION('center_axis',(0.,-0.743144825477394,-0.669130606358858));
#58468=DIRECTION('ref_axis',(-1.,0.,0.));
#58469=DIRECTION('',(-1.,0.,0.));
#58470=DIRECTION('',(0.137844537491629,0.662743003631831,-0.736050673949001));
#58471=DIRECTION('center_axis',(0.99026806874157,-0.106612780622095,0.0894587448987839));
#58472=DIRECTION('ref_axis',(0.,-0.64278760968654,-0.766044443118978));
#58473=DIRECTION('center_axis',(-0.99026806874157,0.106612780622095,-0.0894587448987839));
#58474=DIRECTION('ref_axis',(0.139173100960065,0.758589351257639,-0.636532044855303));
#58475=DIRECTION('',(0.137998583506848,0.668854547266653,-0.730472439966645));
#58476=DIRECTION('center_axis',(0.0617712249622996,-0.741905229276912,-0.667653313133567));
#58477=DIRECTION('ref_axis',(-0.998052578482889,-0.0400959894540314,-0.0477845394804615));
#58478=DIRECTION('center_axis',(-0.0617712249622996,0.741905229276912,0.667653313133567));
#58479=DIRECTION('ref_axis',(0.998090334472114,0.045916079171941,0.0413206716646654));
#58480=DIRECTION('',(-0.0161503784824054,0.668100186146782,-0.743896032080768));
#58481=DIRECTION('center_axis',(-0.284551435696759,-0.71629990457007,-0.637138075424646));
#58482=DIRECTION('ref_axis',(-0.957826285221151,0.184703660511673,0.220121250980087));
#58483=DIRECTION('center_axis',(0.284551435696759,0.71629990457007,0.637138075424646));
#58484=DIRECTION('ref_axis',(-0.958660774436356,0.212613441240154,0.18911648304975));
#58485=DIRECTION('',(-0.0552259184163638,0.675757036144127,-0.735052736908566));
#58486=DIRECTION('center_axis',(-0.491310548314114,-0.659277363310168,-0.569181257019306));
#58487=DIRECTION('ref_axis',(-0.86824314212446,0.318911962258806,0.380064476743201));
#58488=DIRECTION('center_axis',(0.491310548314114,0.659277363310168,0.569181257019306));
#58489=DIRECTION('ref_axis',(-0.870984468928858,0.371889435936037,0.32106744201786));
#58490=DIRECTION('',(-0.0570786439550532,0.676458300008118,-0.734265753494183));
#58491=DIRECTION('center_axis',(-0.313150259135956,-0.710480100250258,-0.630202302718315));
#58492=DIRECTION('ref_axis',(-0.948683298050514,0.203267289834478,0.242244522917128));
#58493=DIRECTION('center_axis',(0.313150259135956,0.710480100250258,0.630202302718315));
#58494=DIRECTION('ref_axis',(-0.949703593340092,0.234269964928557,0.207799586932431));
#58495=DIRECTION('',(-0.0225789275220273,0.668960020557194,-0.742955370751214));
#58496=DIRECTION('center_axis',(0.,-0.743144825477394,-0.669130606358858));
#58497=DIRECTION('ref_axis',(-1.,0.,0.));
#58498=DIRECTION('',(-1.,0.,0.));
#58499=DIRECTION('',(0.0225789275220281,0.668960020557194,-0.742955370751214));
#58500=DIRECTION('center_axis',(0.313150259135957,-0.710480100250258,-0.630202302718315));
#58501=DIRECTION('ref_axis',(-0.948683298050513,-0.203267289834479,-0.242244522917128));
#58502=DIRECTION('center_axis',(-0.313150259135957,0.710480100250258,0.630202302718315));
#58503=DIRECTION('ref_axis',(0.949703593340092,0.234269964928558,0.207799586932432));
#58504=DIRECTION('',(0.0570786439550534,0.676458300008118,-0.734265753494183));
#58505=DIRECTION('center_axis',(0.491310548314113,-0.659277363310168,-0.569181257019307));
#58506=DIRECTION('ref_axis',(-0.86824314212446,-0.318911962258806,-0.3800644767432));
#58507=DIRECTION('center_axis',(-0.491310548314113,0.659277363310168,0.569181257019307));
#58508=DIRECTION('ref_axis',(0.870984468928858,0.371889435936036,0.321067442017859));
#58509=DIRECTION('',(0.0552259184163649,0.675757036144127,-0.735052736908566));
#58510=DIRECTION('center_axis',(0.284551435696759,-0.71629990457007,-0.637138075424646));
#58511=DIRECTION('ref_axis',(-0.957826285221151,-0.184703660511672,-0.220121250980087));
#58512=DIRECTION('center_axis',(-0.284551435696759,0.71629990457007,0.637138075424646));
#58513=DIRECTION('ref_axis',(0.958660774436356,0.212613441240154,0.189116483049749));
#58514=DIRECTION('',(0.016150378482405,0.668100186146782,-0.743896032080768));
#58515=DIRECTION('center_axis',(-0.0617712249622997,-0.741905229276912,
-0.667653313133567));
#58516=DIRECTION('ref_axis',(-0.998052578482889,0.0400959894540315,0.0477845394804615));
#58517=DIRECTION('center_axis',(0.0617712249622997,0.741905229276912,0.667653313133567));
#58518=DIRECTION('ref_axis',(-0.998090334472114,0.045916079171941,0.0413206716646654));
#58519=DIRECTION('',(-0.137998583506848,0.668854547266653,-0.730472439966645));
#58520=DIRECTION('center_axis',(-0.99026806874157,-0.106612780622095,0.0894587448987841));
#58521=DIRECTION('ref_axis',(0.,0.64278760968654,0.766044443118978));
#58522=DIRECTION('center_axis',(0.99026806874157,0.106612780622095,-0.0894587448987841));
#58523=DIRECTION('ref_axis',(-0.139173100960066,0.758589351257642,-0.636532044855299));
#58524=DIRECTION('',(-0.137844537491629,0.662743003631831,-0.736050673949001));
#58525=DIRECTION('center_axis',(0.,-0.743144825477394,-0.669130606358858));
#58526=DIRECTION('ref_axis',(-1.,0.,0.));
#58527=DIRECTION('',(-1.,0.,0.));
#58528=DIRECTION('center_axis',(0.,0.766044443118978,-0.64278760968654));
#58529=DIRECTION('ref_axis',(1.,0.,0.));
#58530=DIRECTION('center_axis',(1.,0.,0.));
#58531=DIRECTION('ref_axis',(0.,1.,0.));
#58532=DIRECTION('center_axis',(1.,0.,0.));
#58533=DIRECTION('ref_axis',(0.,0.,-1.));
#58534=DIRECTION('center_axis',(0.64930555798837,-0.483301338560726,-0.587215555406038));
#58535=DIRECTION('ref_axis',(0.760527640763576,0.412621749021023,0.501339206395651));
#58536=DIRECTION('',(1.,0.,0.));
#58537=DIRECTION('center_axis',(-0.99026806874157,0.0894587448987838,-0.106612780622095));
#58538=DIRECTION('ref_axis',(0.139173100960065,0.636532044855299,-0.758589351257642));
#58539=DIRECTION('center_axis',(-0.0617712249622996,-0.667653313133568,
-0.741905229276912));
#58540=DIRECTION('ref_axis',(-0.998090334472114,0.0413206716646654,0.045916079171941));
#58541=DIRECTION('center_axis',(0.284551435696759,-0.637138075424647,-0.716299904570069));
#58542=DIRECTION('ref_axis',(0.958660774436356,0.18911648304975,0.212613441240154));
#58543=DIRECTION('center_axis',(0.491310548314114,-0.569181257019307,-0.659277363310167));
#58544=DIRECTION('ref_axis',(0.870984468928858,0.32106744201786,0.371889435936037));
#58545=DIRECTION('center_axis',(0.313150259135956,-0.630202302718316,-0.710480100250258));
#58546=DIRECTION('ref_axis',(0.949703593340092,0.207799586932431,0.234269964928557));
#58547=DIRECTION('',(1.,0.,0.));
#58548=DIRECTION('center_axis',(-0.313150259135957,-0.630202302718315,-0.710480100250257));
#58549=DIRECTION('ref_axis',(-0.949703593340092,0.207799586932432,0.234269964928558));
#58550=DIRECTION('center_axis',(-0.491310548314113,-0.569181257019307,-0.659277363310168));
#58551=DIRECTION('ref_axis',(-0.870984468928858,0.321067442017859,0.371889435936036));
#58552=DIRECTION('center_axis',(-0.284551435696759,-0.637138075424647,-0.71629990457007));
#58553=DIRECTION('ref_axis',(-0.958660774436356,0.18911648304975,0.212613441240154));
#58554=DIRECTION('center_axis',(0.0617712249622997,-0.667653313133568,-0.741905229276912));
#58555=DIRECTION('ref_axis',(0.998090334472114,0.0413206716646654,0.045916079171941));
#58556=DIRECTION('center_axis',(0.99026806874157,0.0894587448987841,-0.106612780622095));
#58557=DIRECTION('ref_axis',(-0.139173100960066,0.636532044855299,-0.758589351257642));
#58558=DIRECTION('',(1.,0.,0.));
#58559=DIRECTION('center_axis',(0.,0.669130606358858,0.743144825477394));
#58560=DIRECTION('ref_axis',(1.,0.,0.));
#58561=DIRECTION('',(-0.137844537491629,0.736050673949001,-0.662743003631831));
#58562=DIRECTION('center_axis',(-0.99026806874157,-0.0894587448987841,0.106612780622095));
#58563=DIRECTION('ref_axis',(0.,0.766044443118978,0.642787609686539));
#58564=DIRECTION('',(-0.137998583506848,0.730472439966645,-0.668854547266653));
#58565=DIRECTION('center_axis',(-0.0617712249622997,0.667653313133568,0.741905229276912));
#58566=DIRECTION('ref_axis',(0.998052578482889,0.0477845394804616,0.0400959894540315));
#58567=DIRECTION('',(0.0161503784824051,0.743896032080767,-0.668100186146782));
#58568=DIRECTION('center_axis',(0.284551435696759,0.637138075424647,0.71629990457007));
#58569=DIRECTION('ref_axis',(0.957826285221151,-0.220121250980087,-0.184703660511672));
#58570=DIRECTION('',(0.0552259184163645,0.735052736908566,-0.675757036144128));
#58571=DIRECTION('center_axis',(0.491310548314113,0.569181257019307,0.659277363310168));
#58572=DIRECTION('ref_axis',(0.86824314212446,-0.3800644767432,-0.318911962258805));
#58573=DIRECTION('',(0.057078643955053,0.734265753494182,-0.676458300008118));
#58574=DIRECTION('center_axis',(0.313150259135957,0.630202302718315,0.710480100250257));
#58575=DIRECTION('ref_axis',(0.948683298050513,-0.242244522917128,-0.203267289834479));
#58576=DIRECTION('',(0.0225789275220278,0.742955370751214,-0.668960020557194));
#58577=DIRECTION('center_axis',(0.,0.669130606358858,0.743144825477394));
#58578=DIRECTION('ref_axis',(1.,0.,0.));
#58579=DIRECTION('',(-0.0225789275220274,0.742955370751214,-0.668960020557194));
#58580=DIRECTION('center_axis',(-0.313150259135956,0.630202302718316,0.710480100250258));
#58581=DIRECTION('ref_axis',(0.948683298050514,0.242244522917128,0.203267289834478));
#58582=DIRECTION('',(-0.0570786439550527,0.734265753494182,-0.676458300008118));
#58583=DIRECTION('center_axis',(-0.491310548314114,0.569181257019307,0.659277363310167));
#58584=DIRECTION('ref_axis',(0.868243142124459,0.380064476743201,0.318911962258806));
#58585=DIRECTION('',(-0.0552259184163635,0.735052736908566,-0.675757036144127));
#58586=DIRECTION('center_axis',(-0.284551435696759,0.637138075424647,0.716299904570069));
#58587=DIRECTION('ref_axis',(0.957826285221151,0.220121250980087,0.184703660511673));
#58588=DIRECTION('',(-0.0161503784824052,0.743896032080767,-0.668100186146782));
#58589=DIRECTION('center_axis',(0.0617712249622996,0.667653313133568,0.741905229276912));
#58590=DIRECTION('ref_axis',(0.998052578482889,-0.0477845394804615,-0.0400959894540314));
#58591=DIRECTION('',(0.137998583506848,0.730472439966645,-0.668854547266653));
#58592=DIRECTION('center_axis',(0.99026806874157,-0.0894587448987838,0.106612780622095));
#58593=DIRECTION('ref_axis',(0.,-0.766044443118978,-0.642787609686539));
#58594=DIRECTION('',(0.137844537491629,0.736050673949,-0.662743003631831));
#58595=DIRECTION('center_axis',(0.,0.669130606358858,0.743144825477394));
#58596=DIRECTION('ref_axis',(1.,0.,0.));
#58597=DIRECTION('',(-0.0519254248777279,0.742142297230154,-0.66822792587052));
#58598=DIRECTION('center_axis',(-0.64930555798837,0.483301338560726,0.587215555406038));
#58599=DIRECTION('ref_axis',(0.755033118392644,0.502285118831863,0.421467257957652));
#58600=DIRECTION('center_axis',(0.,-0.848048096156426,-0.529919264233205));
#58601=DIRECTION('ref_axis',(-1.,0.,0.));
#58602=DIRECTION('',(-1.,0.,0.));
#58603=DIRECTION('',(0.137844537491629,0.524860590029465,-0.839952525157012));
#58604=DIRECTION('center_axis',(0.99026806874157,-0.0894587448987838,0.106612780622095));
#58605=DIRECTION('ref_axis',(0.,-0.766044443118978,-0.642787609686539));
#58606=DIRECTION('center_axis',(-0.99026806874157,0.0894587448987838,-0.106612780622095));
#58607=DIRECTION('ref_axis',(0.139173100960065,0.636532044855299,-0.758589351257642));
#58608=DIRECTION('',(0.137998583506848,0.531847935749546,-0.835520295497991));
#58609=DIRECTION('center_axis',(0.0617712249622996,-0.846570802931135,-0.528679668032723));
#58610=DIRECTION('ref_axis',(-0.998052578482889,-0.0477845394804615,-0.0400959894540314));
#58611=DIRECTION('center_axis',(-0.0617712249622996,0.846570802931135,0.528679668032723));
#58612=DIRECTION('ref_axis',(0.998090334472114,0.0523937700909925,0.0327196743412163));
#58613=DIRECTION('',(-0.0161503784824054,0.528774052761765,-0.848608959651484));
#58614=DIRECTION('center_axis',(-0.284551435696759,-0.816055565222214,-0.50307434332588));
#58615=DIRECTION('ref_axis',(-0.957826285221151,0.220121250980087,0.184703660511673));
#58616=DIRECTION('center_axis',(0.284551435696759,0.816055565222214,0.50307434332588));
#58617=DIRECTION('ref_axis',(-0.958660774436356,0.242223097976277,0.149323442110948));
#58618=DIRECTION('',(-0.0552259184163638,0.537850200094025,-0.841229612052433));
#58619=DIRECTION('center_axis',(-0.491310548314114,-0.748098746816874,-0.446051802065978));
#58620=DIRECTION('ref_axis',(-0.868243142124459,0.380064476743201,0.318911962258806));
#58621=DIRECTION('center_axis',(0.491310548314114,0.748098746816874,0.446051802065978));
#58622=DIRECTION('ref_axis',(-0.870984468928858,0.421992375987731,0.25161178329511));
#58623=DIRECTION('',(-0.0570786439550532,0.538677468419953,-0.840576357876501));
#58624=DIRECTION('center_axis',(-0.313150259135956,-0.809119792515883,-0.497254539006068));
#58625=DIRECTION('ref_axis',(-0.948683298050514,0.242244522917128,0.203267289834478));
#58626=DIRECTION('center_axis',(0.313150259135956,0.809119792515883,0.497254539006068));
#58627=DIRECTION('ref_axis',(-0.949703593340092,0.266794897350299,0.163962091791853));
#58628=DIRECTION('',(-0.0225789275220273,0.529784168481124,-0.847831897759644));
#58629=DIRECTION('center_axis',(0.,-0.848048096156426,-0.529919264233205));
#58630=DIRECTION('ref_axis',(-1.,0.,0.));
#58631=DIRECTION('',(-1.,0.,0.));
#58632=DIRECTION('',(0.0225789275220281,0.529784168481124,-0.847831897759644));
#58633=DIRECTION('center_axis',(0.313150259135957,-0.809119792515883,-0.497254539006068));
#58634=DIRECTION('ref_axis',(-0.948683298050513,-0.242244522917128,-0.203267289834479));
#58635=DIRECTION('center_axis',(-0.313150259135957,0.809119792515883,0.497254539006068));
#58636=DIRECTION('ref_axis',(0.949703593340092,0.2667948973503,0.163962091791853));
#58637=DIRECTION('',(0.0570786439550534,0.538677468419952,-0.840576357876501));
#58638=DIRECTION('center_axis',(0.491310548314113,-0.748098746816875,-0.446051802065978));
#58639=DIRECTION('ref_axis',(-0.86824314212446,-0.3800644767432,-0.318911962258805));
#58640=DIRECTION('center_axis',(-0.491310548314113,0.748098746816875,0.446051802065978));
#58641=DIRECTION('ref_axis',(0.870984468928858,0.421992375987729,0.25161178329511));
#58642=DIRECTION('',(0.0552259184163649,0.537850200094025,-0.841229612052432));
#58643=DIRECTION('center_axis',(0.284551435696759,-0.816055565222214,-0.50307434332588));
#58644=DIRECTION('ref_axis',(-0.957826285221151,-0.220121250980087,-0.184703660511672));
#58645=DIRECTION('center_axis',(-0.284551435696759,0.816055565222214,0.50307434332588));
#58646=DIRECTION('ref_axis',(0.958660774436356,0.242223097976277,0.149323442110947));
#58647=DIRECTION('',(0.0161503784824051,0.528774052761765,-0.848608959651484));
#58648=DIRECTION('center_axis',(-0.0617712249622997,-0.846570802931135,
-0.528679668032723));
#58649=DIRECTION('ref_axis',(-0.998052578482889,0.0477845394804616,0.0400959894540315));
#58650=DIRECTION('center_axis',(0.0617712249622997,0.846570802931135,0.528679668032723));
#58651=DIRECTION('ref_axis',(-0.998090334472114,0.0523937700909926,0.0327196743412163));
#58652=DIRECTION('',(-0.137998583506848,0.531847935749546,-0.835520295497991));
#58653=DIRECTION('center_axis',(-0.99026806874157,-0.0894587448987841,0.106612780622095));
#58654=DIRECTION('ref_axis',(0.,0.766044443118978,0.642787609686539));
#58655=DIRECTION('center_axis',(0.99026806874157,0.0894587448987841,-0.106612780622095));
#58656=DIRECTION('ref_axis',(-0.139173100960066,0.636532044855299,-0.758589351257642));
#58657=DIRECTION('',(-0.137844537491629,0.524860590029465,-0.839952525157012));
#58658=DIRECTION('center_axis',(0.,-0.848048096156426,-0.529919264233205));
#58659=DIRECTION('ref_axis',(-1.,0.,0.));
#58660=DIRECTION('',(-1.,0.,0.));
#58661=DIRECTION('center_axis',(0.,0.642787609686539,-0.766044443118978));
#58662=DIRECTION('ref_axis',(1.,0.,0.));
#58663=DIRECTION('center_axis',(1.,0.,0.));
#58664=DIRECTION('ref_axis',(0.,1.,0.));
#58665=DIRECTION('center_axis',(1.,0.,0.));
#58666=DIRECTION('ref_axis',(0.,0.,-1.));
#58667=DIRECTION('center_axis',(0.649305557988371,-0.577927816349714,-0.494370034948177));
#58668=DIRECTION('ref_axis',(0.760527640763576,0.49340973708095,0.422071722564183));
#58669=DIRECTION('',(1.,0.,0.));
#58670=DIRECTION('center_axis',(-0.99026806874157,0.0695865504800327,-0.120527440954873));
#58671=DIRECTION('ref_axis',(0.139173100960065,0.495134034370783,-0.857597304086756));
#58672=DIRECTION('center_axis',(-0.0617712249622996,-0.786340650163727,
-0.614697240653271));
#58673=DIRECTION('ref_axis',(-0.998090334472114,0.0486661612888524,0.0380432514219071));
#58674=DIRECTION('center_axis',(0.284551435696759,-0.751842689509058,-0.594779833782804));
#58675=DIRECTION('ref_axis',(0.958660774436356,0.223163315348643,0.176543632679541));
#58676=DIRECTION('center_axis',(0.491310548314114,-0.675016427497717,-0.550424170729724));
#58677=DIRECTION('ref_axis',(0.870984468928858,0.380767628982861,0.310486823558562));
#58678=DIRECTION('center_axis',(0.313150259135956,-0.744001688360219,-0.590252829658806));
#58679=DIRECTION('ref_axis',(0.949703593340092,0.245323196775732,0.194626858168784));
#58680=DIRECTION('',(1.,0.,0.));
#58681=DIRECTION('center_axis',(-0.313150259135957,-0.744001688360219,-0.590252829658806));
#58682=DIRECTION('ref_axis',(-0.949703593340092,0.245323196775733,0.194626858168784));
#58683=DIRECTION('center_axis',(-0.491310548314113,-0.675016427497717,-0.550424170729724));
#58684=DIRECTION('ref_axis',(-0.870984468928858,0.38076762898286,0.310486823558561));
#58685=DIRECTION('center_axis',(-0.284551435696759,-0.751842689509058,-0.594779833782804));
#58686=DIRECTION('ref_axis',(-0.958660774436356,0.223163315348643,0.176543632679541));
#58687=DIRECTION('center_axis',(0.0617712249622997,-0.786340650163727,-0.61469724065327));
#58688=DIRECTION('ref_axis',(0.998090334472114,0.0486661612888524,0.0380432514219071));
#58689=DIRECTION('center_axis',(0.99026806874157,0.0695865504800329,-0.120527440954873));
#58690=DIRECTION('ref_axis',(-0.139173100960066,0.495134034370784,-0.857597304086755));
#58691=DIRECTION('',(1.,0.,0.));
#58692=DIRECTION('center_axis',(0.,0.788010753606722,0.615661475325659));
#58693=DIRECTION('ref_axis',(1.,0.,0.));
#58694=DIRECTION('',(-0.137844537491629,0.609784295472662,-0.780488306432985));
#58695=DIRECTION('center_axis',(-0.99026806874157,-0.0695865504800329,0.120527440954873));
#58696=DIRECTION('ref_axis',(0.,0.866025403784439,0.5));
#58697=DIRECTION('',(-0.137998583506848,0.603229548983803,-0.785538351821795));
#58698=DIRECTION('center_axis',(-0.0617712249622997,0.786340650163727,0.61469724065327));
#58699=DIRECTION('ref_axis',(0.998052578482889,0.0540211804549215,0.0311891430775903));
#58700=DIRECTION('',(0.0161503784824051,0.616580200004832,-0.787126433450736));
#58701=DIRECTION('center_axis',(0.284551435696759,0.751842689509058,0.594779833782804));
#58702=DIRECTION('ref_axis',(0.957826285221151,-0.248850568624199,-0.143673942783173));
#58703=DIRECTION('',(0.0552259184163645,0.606541656308365,-0.79313133660055));
#58704=DIRECTION('center_axis',(0.491310548314113,0.675016427497717,0.550424170729724));
#58705=DIRECTION('ref_axis',(0.86824314212446,-0.429668924423658,-0.248069469178416));
#58706=DIRECTION('',(0.057078643955053,0.605644855748342,-0.793685288454953));
#58707=DIRECTION('center_axis',(0.313150259135957,0.744001688360219,0.590252829658806));
#58708=DIRECTION('ref_axis',(0.948683298050513,-0.273861278752585,-0.15811388300842));
#58709=DIRECTION('',(0.0225789275220278,0.615504520756066,-0.787809860918738));
#58710=DIRECTION('center_axis',(0.,0.788010753606722,0.615661475325658));
#58711=DIRECTION('ref_axis',(1.,0.,0.));
#58712=DIRECTION('',(-0.0225789275220274,0.615504520756066,-0.787809860918738));
#58713=DIRECTION('center_axis',(-0.313150259135956,0.744001688360219,0.590252829658806));
#58714=DIRECTION('ref_axis',(0.948683298050514,0.273861278752584,0.158113883008419));
#58715=DIRECTION('',(-0.0570786439550527,0.605644855748342,-0.793685288454953));
#58716=DIRECTION('center_axis',(-0.491310548314114,0.675016427497717,0.550424170729724));
#58717=DIRECTION('ref_axis',(0.868243142124459,0.429668924423659,0.248069469178417));
#58718=DIRECTION('',(-0.0552259184163635,0.606541656308365,-0.793131336600549));
#58719=DIRECTION('center_axis',(-0.284551435696759,0.751842689509058,0.594779833782804));
#58720=DIRECTION('ref_axis',(0.957826285221151,0.248850568624199,0.143673942783173));
#58721=DIRECTION('',(-0.0161503784824052,0.616580200004832,-0.787126433450736));
#58722=DIRECTION('center_axis',(0.0617712249622996,0.786340650163727,0.614697240653271));
#58723=DIRECTION('ref_axis',(0.998052578482889,-0.0540211804549215,-0.0311891430775903));
#58724=DIRECTION('',(0.137998583506848,0.603229548983803,-0.785538351821795));
#58725=DIRECTION('center_axis',(0.99026806874157,-0.0695865504800327,0.120527440954873));
#58726=DIRECTION('ref_axis',(0.,-0.866025403784439,-0.5));
#58727=DIRECTION('',(0.137844537491629,0.609784295472662,-0.780488306432985));
#58728=DIRECTION('center_axis',(0.,0.788010753606722,0.615661475325658));
#58729=DIRECTION('ref_axis',(1.,0.,0.));
#58730=DIRECTION('',(-0.051925424877728,0.614830926556978,-0.786947699660121));
#58731=DIRECTION('center_axis',(-0.649305557988371,0.577927816349714,0.494370034948177));
#58732=DIRECTION('ref_axis',(0.755033118392644,0.567841300538901,0.327843327723122));
#58733=DIRECTION('center_axis',(0.,-0.927183854566787,-0.374606593415912));
#58734=DIRECTION('ref_axis',(-1.,0.,0.));
#58735=DIRECTION('',(-1.,0.,0.));
#58736=DIRECTION('',(0.137844537491629,0.371030552991328,-0.918332843924613));
#58737=DIRECTION('center_axis',(0.99026806874157,-0.0695865504800327,0.120527440954873));
#58738=DIRECTION('ref_axis',(0.,-0.866025403784439,-0.5));
#58739=DIRECTION('center_axis',(-0.99026806874157,0.0695865504800327,-0.120527440954873));
#58740=DIRECTION('ref_axis',(0.139173100960065,0.495134034370783,-0.857597304086756));
#58741=DIRECTION('',(0.137998583506848,0.378681393832731,-0.9151812896443));
#58742=DIRECTION('center_axis',(0.0617712249622996,-0.925513751123792,-0.373642358743524));
#58743=DIRECTION('ref_axis',(-0.998052578482889,-0.0540211804549215,-0.0311891430775903));
#58744=DIRECTION('center_axis',(-0.0617712249622996,0.925513751123792,0.373642358743524));
#58745=DIRECTION('ref_axis',(0.998090334472114,0.0572795028183562,0.0231245062698634));
#58746=DIRECTION('',(-0.0161503784824054,0.373381387356163,-0.927537333400043));
#58747=DIRECTION('center_axis',(-0.284551435696759,-0.891015790469123,-0.353724951873058));
#58748=DIRECTION('ref_axis',(-0.957826285221151,0.248850568624199,0.143673942783173));
#58749=DIRECTION('center_axis',(0.284551435696759,0.891015790469123,0.353724951873058));
#58750=DIRECTION('ref_axis',(-0.958660774436356,0.264472928451193,0.104993283944912));
#58751=DIRECTION('',(-0.0552259184163638,0.3836010578794,-0.921846151116809));
#58752=DIRECTION('center_axis',(-0.491310548314114,-0.814189528457782,-0.309369288819978));
#58753=DIRECTION('ref_axis',(-0.868243142124459,0.429668924423659,0.248069469178417));
#58754=DIRECTION('center_axis',(0.491310548314114,0.814189528457782,0.309369288819978));
#58755=DIRECTION('ref_axis',(-0.870984468928858,0.459273291233482,0.174511027858645));
#58756=DIRECTION('',(-0.0570786439550532,0.384529194537798,-0.921346474976903));
#58757=DIRECTION('center_axis',(-0.313150259135956,-0.883174789320284,-0.34919794774906));
#58758=DIRECTION('ref_axis',(-0.948683298050514,0.273861278752584,0.158113883008419));
#58759=DIRECTION('center_axis',(0.313150259135956,0.883174789320284,0.34919794774906));
#58760=DIRECTION('ref_axis',(-0.949703593340092,0.291213401820783,0.115142691461001));
#58761=DIRECTION('',(-0.0225789275220273,0.374511092529479,-0.926947481578288));
#58762=DIRECTION('center_axis',(0.,-0.927183854566787,-0.374606593415912));
#58763=DIRECTION('ref_axis',(-1.,0.,0.));
#58764=DIRECTION('',(-1.,0.,0.));
#58765=DIRECTION('',(0.0225789275220281,0.374511092529479,-0.926947481578288));
#58766=DIRECTION('center_axis',(0.313150259135957,-0.883174789320284,-0.349197947749059));
#58767=DIRECTION('ref_axis',(-0.948683298050513,-0.273861278752585,-0.15811388300842));
#58768=DIRECTION('center_axis',(-0.313150259135957,0.883174789320284,0.349197947749059));
#58769=DIRECTION('ref_axis',(0.949703593340092,0.291213401820785,0.115142691461001));
#58770=DIRECTION('',(0.0570786439550534,0.384529194537798,-0.921346474976903));
#58771=DIRECTION('center_axis',(0.491310548314113,-0.814189528457783,-0.309369288819978));
#58772=DIRECTION('ref_axis',(-0.86824314212446,-0.429668924423658,-0.248069469178416));
#58773=DIRECTION('center_axis',(-0.491310548314113,0.814189528457783,0.309369288819978));
#58774=DIRECTION('ref_axis',(0.870984468928858,0.459273291233481,0.174511027858644));
#58775=DIRECTION('',(0.0552259184163649,0.3836010578794,-0.921846151116809));
#58776=DIRECTION('center_axis',(0.284551435696759,-0.891015790469123,-0.353724951873058));
#58777=DIRECTION('ref_axis',(-0.957826285221151,-0.248850568624199,-0.143673942783173));
#58778=DIRECTION('center_axis',(-0.284551435696759,0.891015790469123,0.353724951873058));
#58779=DIRECTION('ref_axis',(0.958660774436356,0.264472928451193,0.104993283944912));
#58780=DIRECTION('',(0.0161503784824051,0.373381387356163,-0.927537333400043));
#58781=DIRECTION('center_axis',(-0.0617712249622997,-0.925513751123792,
-0.373642358743524));
#58782=DIRECTION('ref_axis',(-0.998052578482889,0.0540211804549215,0.0311891430775903));
#58783=DIRECTION('center_axis',(0.0617712249622997,0.925513751123792,0.373642358743524));
#58784=DIRECTION('ref_axis',(-0.998090334472114,0.0572795028183562,0.0231245062698635));
#58785=DIRECTION('',(-0.137998583506848,0.378681393832731,-0.9151812896443));
#58786=DIRECTION('center_axis',(-0.99026806874157,-0.0695865504800329,0.120527440954873));
#58787=DIRECTION('ref_axis',(0.,0.866025403784439,0.5));
#58788=DIRECTION('center_axis',(0.99026806874157,0.0695865504800329,-0.120527440954873));
#58789=DIRECTION('ref_axis',(-0.139173100960066,0.495134034370784,-0.857597304086755));
#58790=DIRECTION('',(-0.137844537491629,0.371030552991328,-0.918332843924613));
#58791=DIRECTION('center_axis',(0.,-0.927183854566787,-0.374606593415912));
#58792=DIRECTION('ref_axis',(-1.,0.,0.));
#58793=DIRECTION('',(-1.,0.,0.));
#58794=DIRECTION('center_axis',(0.,0.5,-0.866025403784439));
#58795=DIRECTION('ref_axis',(1.,0.,0.));
#58796=DIRECTION('center_axis',(1.,0.,0.));
#58797=DIRECTION('ref_axis',(0.,1.,0.));
#58798=DIRECTION('center_axis',(1.,0.,0.));
#58799=DIRECTION('ref_axis',(0.,0.,-1.));
#58800=DIRECTION('center_axis',(0.64930555798837,-0.654994249884502,-0.386503331141725));
#58801=DIRECTION('ref_axis',(0.760527640763576,0.559205719957048,0.329979803021198));
#58802=DIRECTION('',(1.,0.,0.));
#58803=DIRECTION('center_axis',(-0.99026806874157,0.0476000039374393,-0.130779935984066));
#58804=DIRECTION('ref_axis',(0.139173100960065,0.338691626801823,-0.930547596796367));
#58805=DIRECTION('center_axis',(-0.0617712249622996,-0.88113542444623,-0.468811987424191));
#58806=DIRECTION('ref_axis',(-0.998090334472114,0.0545329542285434,0.0290144987282327));
#58807=DIRECTION('center_axis',(0.284551435696759,-0.843702943923494,-0.455187678719166));
#58808=DIRECTION('ref_axis',(0.958660774436356,0.250429443236755,0.135109635175349));
#58809=DIRECTION('center_axis',(0.491310548314114,-0.760341565401403,-0.424846618249727));
#58810=DIRECTION('ref_axis',(0.870984468928858,0.428898384218936,0.239650226161174));
#58811=DIRECTION('center_axis',(0.313150259135956,-0.835194959184317,-0.452091025520514));
#58812=DIRECTION('ref_axis',(0.949703593340092,0.27539278542453,0.149070112809494));
#58813=DIRECTION('',(1.,0.,0.));
#58814=DIRECTION('center_axis',(-0.313150259135957,-0.835194959184317,-0.452091025520514));
#58815=DIRECTION('ref_axis',(-0.949703593340092,0.275392785424531,0.149070112809494));
#58816=DIRECTION('center_axis',(-0.491310548314113,-0.760341565401403,-0.424846618249727));
#58817=DIRECTION('ref_axis',(-0.870984468928858,0.428898384218935,0.239650226161173));
#58818=DIRECTION('center_axis',(-0.284551435696759,-0.843702943923494,-0.455187678719166));
#58819=DIRECTION('ref_axis',(-0.958660774436356,0.250429443236754,0.135109635175349));
#58820=DIRECTION('center_axis',(0.0617712249622997,-0.88113542444623,-0.468811987424191));
#58821=DIRECTION('ref_axis',(0.998090334472114,0.0545329542285435,0.0290144987282327));
#58822=DIRECTION('center_axis',(0.99026806874157,0.0476000039374394,-0.130779935984066));
#58823=DIRECTION('ref_axis',(-0.139173100960066,0.338691626801824,-0.930547596796366));
#58824=DIRECTION('',(1.,0.,0.));
#58825=DIRECTION('center_axis',(0.,0.882947592858927,0.469471562785891));
#58826=DIRECTION('ref_axis',(1.,0.,0.));
#58827=DIRECTION('',(-0.137844537491629,0.464989929744127,-0.874518866989312));
#58828=DIRECTION('center_axis',(-0.99026806874157,-0.0476000039374394,0.130779935984066));
#58829=DIRECTION('ref_axis',(0.,0.939692620785909,0.342020143325668));
#58830=DIRECTION('',(-0.137998583506848,0.457657833403967,-0.878353971058417));
#58831=DIRECTION('center_axis',(-0.0617712249622997,0.88113542444623,0.468811987424191));
#58832=DIRECTION('ref_axis',(0.998052578482889,0.058616415197295,0.0213346303712044));
#58833=DIRECTION('',(0.0161503784824051,0.470529890556386,-0.882236242379484));
#58834=DIRECTION('center_axis',(0.284551435696759,0.843702943923494,0.455187678719166));
#58835=DIRECTION('ref_axis',(0.957826285221151,-0.270018687665128,-0.0982787650057291));
#58836=DIRECTION('',(0.0552259184163645,0.459601114406121,-0.886406742738186));
#58837=DIRECTION('center_axis',(0.491310548314113,0.760341565401403,0.424846618249727));
#58838=DIRECTION('ref_axis',(0.86824314212446,-0.46621809925847,-0.169689510806249));
#58839=DIRECTION('',(0.057078643955053,0.458621745531673,-0.886796551036219));
#58840=DIRECTION('center_axis',(0.313150259135957,0.835194959184317,0.452091025520514));
#58841=DIRECTION('ref_axis',(0.948683298050513,-0.297156898213637,-0.108156265856635));
#58842=DIRECTION('',(0.0225789275220278,0.46935187735806,-0.88272249730729));
#58843=DIRECTION('center_axis',(0.,0.882947592858927,0.46947156278589));
#58844=DIRECTION('ref_axis',(1.,0.,0.));
#58845=DIRECTION('',(-0.0225789275220274,0.46935187735806,-0.88272249730729));
#58846=DIRECTION('center_axis',(-0.313150259135956,0.835194959184317,0.452091025520514));
#58847=DIRECTION('ref_axis',(0.948683298050514,0.297156898213636,0.108156265856635));
#58848=DIRECTION('',(-0.0570786439550527,0.458621745531673,-0.886796551036219));
#58849=DIRECTION('center_axis',(-0.491310548314114,0.760341565401403,0.424846618249727));
#58850=DIRECTION('ref_axis',(0.868243142124459,0.466218099258471,0.169689510806249));
#58851=DIRECTION('',(-0.0552259184163635,0.459601114406122,-0.886406742738186));
#58852=DIRECTION('center_axis',(-0.284551435696759,0.843702943923494,0.455187678719166));
#58853=DIRECTION('ref_axis',(0.957826285221151,0.270018687665129,0.0982787650057294));
#58854=DIRECTION('',(-0.0161503784824052,0.470529890556386,-0.882236242379483));
#58855=DIRECTION('center_axis',(0.0617712249622996,0.88113542444623,0.468811987424191));
#58856=DIRECTION('ref_axis',(0.998052578482889,-0.0586164151972949,-0.0213346303712044));
#58857=DIRECTION('',(0.137998583506848,0.457657833403967,-0.878353971058417));
#58858=DIRECTION('center_axis',(0.99026806874157,-0.0476000039374393,0.130779935984066));
#58859=DIRECTION('ref_axis',(0.,-0.939692620785909,-0.342020143325668));
#58860=DIRECTION('',(0.137844537491629,0.464989929744127,-0.874518866989312));
#58861=DIRECTION('center_axis',(0.,0.882947592858927,0.46947156278589));
#58862=DIRECTION('ref_axis',(1.,0.,0.));
#58863=DIRECTION('',(-0.0519254248777279,0.468838229299828,-0.881756465810299));
#58864=DIRECTION('center_axis',(-0.64930555798837,0.654994249884502,0.386503331141725));
#58865=DIRECTION('ref_axis',(0.755033118392644,0.616143911670627,0.224258043872452));
#58866=DIRECTION('center_axis',(0.,-0.978147600733806,-0.207911690817759));
#58867=DIRECTION('ref_axis',(-1.,0.,0.));
#58868=DIRECTION('',(-1.,0.,0.));
#58869=DIRECTION('',(0.137844537491629,0.205926940351067,-0.968810083928407));
#58870=DIRECTION('center_axis',(0.99026806874157,-0.0476000039374393,0.130779935984066));
#58871=DIRECTION('ref_axis',(0.,-0.939692620785909,-0.342020143325668));
#58872=DIRECTION('center_axis',(-0.99026806874157,0.0476000039374393,-0.130779935984066));
#58873=DIRECTION('ref_axis',(0.139173100960065,0.338691626801823,-0.930547596796367));
#58874=DIRECTION('',(0.137998583506848,0.214008809386338,-0.967034963408845));
#58875=DIRECTION('center_axis',(0.0617712249622996,-0.976335432321108,-0.207252115456059));
#58876=DIRECTION('ref_axis',(-0.998052578482889,-0.0586164151972949,-0.0213346303712044));
#58877=DIRECTION('center_axis',(-0.0617712249622996,0.976335432321108,0.207252115456059));
#58878=DIRECTION('ref_axis',(0.998090334472114,0.0604248268374111,0.0128267117770655));
#58879=DIRECTION('',(-0.0161503784824054,0.206643717435841,-0.97828295462978));
#58880=DIRECTION('center_axis',(-0.284551435696759,-0.938902951798373,-0.193627806751034));
#58881=DIRECTION('ref_axis',(-0.957826285221151,0.270018687665129,0.0982787650057294));
#58882=DIRECTION('center_axis',(0.284551435696759,0.938902951798373,0.193627806751034));
#58883=DIRECTION('ref_axis',(-0.958660774436356,0.278686882824879,0.0574729579753753));
#58884=DIRECTION('',(-0.0552259184163638,0.21769639163261,-0.974452861356162));
#58885=DIRECTION('center_axis',(-0.491310548314114,-0.855541573276281,-0.163286746281595));
#58886=DIRECTION('ref_axis',(-0.868243142124459,0.466218099258471,0.169689510806249));
#58887=DIRECTION('center_axis',(0.491310548314114,0.855541573276281,0.163286746281595));
#58888=DIRECTION('ref_axis',(-0.870984468928858,0.482599419928604,0.0921078431475349));
#58889=DIRECTION('',(-0.0570786439550532,0.218697195660774,-0.974121945658943));
#58890=DIRECTION('center_axis',(-0.313150259135956,-0.930394967059196,-0.190531153552383));
#58891=DIRECTION('ref_axis',(-0.948683298050514,0.297156898213636,0.108156265856635));
#58892=DIRECTION('center_axis',(0.313150259135956,0.930394967059196,0.190531153552383));
#58893=DIRECTION('ref_axis',(-0.949703593340092,0.306783534438035,0.0628247387151194));
#58894=DIRECTION('',(-0.0225789275220273,0.207858686543083,-0.977898235227234));
#58895=DIRECTION('center_axis',(0.,-0.978147600733806,-0.207911690817759));
#58896=DIRECTION('ref_axis',(-1.,0.,0.));
#58897=DIRECTION('',(-1.,0.,0.));
#58898=DIRECTION('',(0.0225789275220281,0.207858686543083,-0.977898235227234));
#58899=DIRECTION('center_axis',(0.313150259135957,-0.930394967059196,-0.190531153552383));
#58900=DIRECTION('ref_axis',(-0.948683298050513,-0.297156898213637,-0.108156265856635));
#58901=DIRECTION('center_axis',(-0.313150259135957,0.930394967059196,0.190531153552383));
#58902=DIRECTION('ref_axis',(0.949703593340092,0.306783534438037,0.0628247387151195));
#58903=DIRECTION('',(0.0570786439550534,0.218697195660774,-0.974121945658944));
#58904=DIRECTION('center_axis',(0.491310548314113,-0.855541573276282,-0.163286746281595));
#58905=DIRECTION('ref_axis',(-0.86824314212446,-0.46621809925847,-0.169689510806249));
#58906=DIRECTION('center_axis',(-0.491310548314113,0.855541573276282,0.163286746281595));
#58907=DIRECTION('ref_axis',(0.870984468928858,0.482599419928603,0.0921078431475346));
#58908=DIRECTION('',(0.0552259184163649,0.21769639163261,-0.974452861356161));
#58909=DIRECTION('center_axis',(0.284551435696759,-0.938902951798373,-0.193627806751034));
#58910=DIRECTION('ref_axis',(-0.957826285221151,-0.270018687665128,-0.0982787650057291));
#58911=DIRECTION('center_axis',(-0.284551435696759,0.938902951798373,0.193627806751034));
#58912=DIRECTION('ref_axis',(0.958660774436356,0.278686882824878,0.0574729579753753));
#58913=DIRECTION('',(0.0161503784824051,0.206643717435841,-0.97828295462978));
#58914=DIRECTION('center_axis',(-0.0617712249622997,-0.976335432321108,
-0.207252115456059));
#58915=DIRECTION('ref_axis',(-0.998052578482889,0.058616415197295,0.0213346303712044));
#58916=DIRECTION('center_axis',(0.0617712249622997,0.976335432321108,0.207252115456059));
#58917=DIRECTION('ref_axis',(-0.998090334472114,0.0604248268374112,0.0128267117770655));
#58918=DIRECTION('',(-0.137998583506848,0.214008809386338,-0.967034963408845));
#58919=DIRECTION('center_axis',(-0.99026806874157,-0.0476000039374394,0.130779935984066));
#58920=DIRECTION('ref_axis',(0.,0.939692620785909,0.342020143325668));
#58921=DIRECTION('center_axis',(0.99026806874157,0.0476000039374394,-0.130779935984066));
#58922=DIRECTION('ref_axis',(-0.139173100960066,0.338691626801824,-0.930547596796366));
#58923=DIRECTION('',(-0.137844537491629,0.205926940351067,-0.968810083928407));
#58924=DIRECTION('center_axis',(0.,-0.978147600733806,-0.207911690817759));
#58925=DIRECTION('ref_axis',(-1.,0.,0.));
#58926=DIRECTION('',(-1.,0.,0.));
#58927=DIRECTION('center_axis',(0.,0.342020143325668,-0.939692620785909));
#58928=DIRECTION('ref_axis',(1.,0.,0.));
#58929=DIRECTION('center_axis',(1.,0.,0.));
#58930=DIRECTION('ref_axis',(0.,1.,0.));
#58931=DIRECTION('center_axis',(1.,0.,0.));
#58932=DIRECTION('ref_axis',(0.,0.,-1.));
#58933=DIRECTION('center_axis',(0.649305557988371,-0.712159014579632,-0.266892919198654));
#58934=DIRECTION('ref_axis',(0.760527640763576,0.608010520003998,0.227861614141252));
#58935=DIRECTION('',(1.,0.,0.));
#58936=DIRECTION('center_axis',(-0.99026806874157,0.024167155361971,-0.137058748836223));
#58937=DIRECTION('ref_axis',(0.139173100960065,0.171958245538723,-0.975223671657125));
#58938=DIRECTION('center_axis',(-0.0617712249622996,-0.949157344732972,
-0.30868211918754));
#58939=DIRECTION('ref_axis',(-0.998090334472114,0.0587427909490065,0.0191041551727457));
#58940=DIRECTION('center_axis',(0.284551435696759,-0.909927711321105,-0.301764876373726));
#58941=DIRECTION('ref_axis',(0.958660774436356,0.27008639921553,0.0895703997751285));
#58942=DIRECTION('center_axis',(0.491310548314114,-0.822564109591763,-0.286360316256974));
#58943=DIRECTION('ref_axis',(0.870984468928858,0.463997279083573,0.161531977910744));
#58944=DIRECTION('center_axis',(0.313150259135956,-0.901011253802641,-0.30019266434088));
#58945=DIRECTION('ref_axis',(0.949703593340092,0.297094703643677,0.0989839475056044));
#58946=DIRECTION('',(1.,0.,0.));
#58947=DIRECTION('center_axis',(-0.313150259135957,-0.901011253802641,-0.30019266434088));
#58948=DIRECTION('ref_axis',(-0.949703593340092,0.297094703643678,0.0989839475056048));
#58949=DIRECTION('center_axis',(-0.491310548314113,-0.822564109591764,-0.286360316256974));
#58950=DIRECTION('ref_axis',(-0.870984468928858,0.463997279083571,0.161531977910743));
#58951=DIRECTION('center_axis',(-0.284551435696759,-0.909927711321105,-0.301764876373726));
#58952=DIRECTION('ref_axis',(-0.958660774436356,0.270086399215529,0.0895703997751283));
#58953=DIRECTION('center_axis',(0.0617712249622997,-0.949157344732972,-0.30868211918754));
#58954=DIRECTION('ref_axis',(0.998090334472114,0.0587427909490066,0.0191041551727457));
#58955=DIRECTION('center_axis',(0.99026806874157,0.0241671553619711,-0.137058748836224));
#58956=DIRECTION('ref_axis',(-0.139173100960066,0.171958245538724,-0.975223671657125));
#58957=DIRECTION('',(1.,0.,0.));
#58958=DIRECTION('center_axis',(0.,0.951056516295154,0.309016994374947));
#58959=DIRECTION('ref_axis',(1.,0.,0.));
#58960=DIRECTION('',(-0.137844537491629,0.306067080296576,-0.941977614300068));
#58961=DIRECTION('center_axis',(-0.99026806874157,-0.0241671553619711,0.137058748836224));
#58962=DIRECTION('ref_axis',(0.,0.984807753012208,0.17364817766693));
#58963=DIRECTION('',(-0.137998583506848,0.298180416142191,-0.944481249352984));
#58964=DIRECTION('center_axis',(-0.0617712249622997,0.949157344732972,0.30868211918754));
#58965=DIRECTION('ref_axis',(0.998052578482889,0.0614306198252359,0.0108318757168334));
#58966=DIRECTION('',(0.0161503784824051,0.310182768482997,-0.950539749516609));
#58967=DIRECTION('center_axis',(0.284551435696759,0.909927711321105,0.301764876373726));
#58968=DIRECTION('ref_axis',(0.957826285221151,-0.282982425517402,-0.0498974366850414));
#58969=DIRECTION('',(0.0552259184163645,0.298695825212034,-0.952749128541176));
#58970=DIRECTION('center_axis',(0.491310548314113,0.822564109591764,0.286360316256974));
#58971=DIRECTION('ref_axis',(0.86824314212446,-0.488601473065054,-0.0861536225152692));
#58972=DIRECTION('',(0.057078643955053,0.297663645650825,-0.952962949154956));
#58973=DIRECTION('center_axis',(0.313150259135957,0.901011253802641,0.30019266434088));
#58974=DIRECTION('ref_axis',(0.948683298050513,-0.311423555691114,-0.0549123752965085));
#58975=DIRECTION('',(0.0225789275220278,0.30893821467004,-0.950814057294297));
#58976=DIRECTION('center_axis',(0.,0.951056516295154,0.309016994374947));
#58977=DIRECTION('ref_axis',(1.,0.,0.));
#58978=DIRECTION('',(-0.0225789275220274,0.30893821467004,-0.950814057294297));
#58979=DIRECTION('center_axis',(-0.313150259135956,0.901011253802641,0.30019266434088));
#58980=DIRECTION('ref_axis',(0.948683298050514,0.311423555691113,0.0549123752965084));
#58981=DIRECTION('',(-0.0570786439550527,0.297663645650825,-0.952962949154956));
#58982=DIRECTION('center_axis',(-0.491310548314114,0.822564109591763,0.286360316256974));
#58983=DIRECTION('ref_axis',(0.86824314212446,0.488601473065055,0.0861536225152694));
#58984=DIRECTION('',(-0.0552259184163635,0.298695825212034,-0.952749128541176));
#58985=DIRECTION('center_axis',(-0.284551435696759,0.909927711321105,0.301764876373726));
#58986=DIRECTION('ref_axis',(0.957826285221151,0.282982425517402,0.0498974366850415));
#58987=DIRECTION('',(-0.0161503784824052,0.310182768482997,-0.950539749516609));
#58988=DIRECTION('center_axis',(0.0617712249622996,0.949157344732972,0.30868211918754));
#58989=DIRECTION('ref_axis',(0.998052578482889,-0.0614306198252359,-0.0108318757168334));
#58990=DIRECTION('',(0.137998583506848,0.298180416142191,-0.944481249352984));
#58991=DIRECTION('center_axis',(0.99026806874157,-0.024167155361971,0.137058748836223));
#58992=DIRECTION('ref_axis',(0.,-0.984807753012208,-0.17364817766693));
#58993=DIRECTION('',(0.137844537491629,0.306067080296576,-0.941977614300068));
#58994=DIRECTION('center_axis',(0.,0.951056516295154,0.309016994374947));
#58995=DIRECTION('ref_axis',(1.,0.,0.));
#58996=DIRECTION('',(-0.051925424877728,0.308600119688995,-0.949773507937132));
#58997=DIRECTION('center_axis',(-0.649305557988371,0.712159014579632,0.266892919198654));
#58998=DIRECTION('ref_axis',(0.755033118392644,0.645725301830105,0.113858792838764));
#58999=DIRECTION('center_axis',(0.,-0.999390827019096,-0.0348994967025006));
#59000=DIRECTION('ref_axis',(-1.,0.,0.));
#59001=DIRECTION('',(-1.,0.,0.));
#59002=DIRECTION('',(0.137844537491629,0.0345663418323,-0.989850519773593));
#59003=DIRECTION('center_axis',(0.99026806874157,-0.024167155361971,0.137058748836223));
#59004=DIRECTION('ref_axis',(0.,-0.984807753012208,-0.17364817766693));
#59005=DIRECTION('center_axis',(-0.99026806874157,0.024167155361971,-0.137058748836223));
#59006=DIRECTION('ref_axis',(0.139173100960065,0.171958245538723,-0.975223671657125));
#59007=DIRECTION('',(0.137998583506848,0.0428336755604254,-0.989505769153514));
#59008=DIRECTION('center_axis',(0.0617712249622996,-0.997491655456914,-0.0345646215150937));
#59009=DIRECTION('ref_axis',(-0.998052578482889,-0.0614306198252359,-0.0108318757168334));
#59010=DIRECTION('center_axis',(-0.0617712249622996,0.997491655456914,0.0345646215150937));
#59011=DIRECTION('ref_axis',(0.998090334472114,0.061734173069449,0.00213918413755088));
#59012=DIRECTION('',(-0.0161503784824054,0.0336272827279992,-0.999303943318151));
#59013=DIRECTION('center_axis',(-0.284551435696759,-0.958262022045047,-0.0276473787012791));
#59014=DIRECTION('ref_axis',(-0.957826285221151,0.282982425517402,0.0498974366850415));
#59015=DIRECTION('center_axis',(0.284551435696759,0.958262022045047,0.0276473787012791));
#59016=DIRECTION('ref_axis',(-0.958660774436356,0.284433077286297,0.00820634526047697));
#59017=DIRECTION('',(-0.0552259184163638,0.0451771306857526,-0.997451314500147));
#59018=DIRECTION('center_axis',(-0.491310548314114,-0.870898420315705,-0.0122428185845276));
#59019=DIRECTION('ref_axis',(-0.86824314212446,0.488601473065055,0.0861536225152694));
#59020=DIRECTION('center_axis',(0.491310548314114,0.870898420315705,0.0122428185845276));
#59021=DIRECTION('ref_axis',(-0.870984468928858,0.491262009456284,0.0069060082312051));
#59022=DIRECTION('',(-0.0570786439550532,0.0462201931597179,-0.997299213951626));
#59023=DIRECTION('center_axis',(-0.313150259135956,-0.949345564526583,-0.0260751666684333));
#59024=DIRECTION('ref_axis',(-0.948683298050514,0.311423555691113,0.0549123752965084));
#59025=DIRECTION('center_axis',(0.313150259135956,0.949345564526583,0.0260751666684333));
#59026=DIRECTION('ref_axis',(-0.949703593340092,0.313032204601347,0.00859788807423104));
#59027=DIRECTION('',(-0.0225789275220273,0.0348905995476461,-0.999136045839184));
#59028=DIRECTION('center_axis',(0.,-0.999390827019096,-0.0348994967025006));
#59029=DIRECTION('ref_axis',(-1.,0.,0.));
#59030=DIRECTION('',(-1.,0.,0.));
#59031=DIRECTION('',(0.0225789275220281,0.0348905995476461,-0.999136045839184));
#59032=DIRECTION('center_axis',(0.313150259135957,-0.949345564526583,-0.0260751666684331));
#59033=DIRECTION('ref_axis',(-0.948683298050513,-0.311423555691114,-0.0549123752965085));
#59034=DIRECTION('center_axis',(-0.313150259135957,0.949345564526583,0.0260751666684331));
#59035=DIRECTION('ref_axis',(0.949703593340092,0.313032204601348,0.00859788807423098));
#59036=DIRECTION('',(0.0570786439550534,0.0462201931597177,-0.997299213951626));
#59037=DIRECTION('center_axis',(0.491310548314113,-0.870898420315706,-0.0122428185845275));
#59038=DIRECTION('ref_axis',(-0.86824314212446,-0.488601473065054,-0.0861536225152692));
#59039=DIRECTION('center_axis',(-0.491310548314113,0.870898420315706,0.0122428185845275));
#59040=DIRECTION('ref_axis',(0.870984468928858,0.491262009456283,0.00690600823120502));
#59041=DIRECTION('',(0.0552259184163649,0.045177130685753,-0.997451314500147));
#59042=DIRECTION('center_axis',(0.284551435696759,-0.958262022045047,-0.0276473787012793));
#59043=DIRECTION('ref_axis',(-0.957826285221151,-0.282982425517402,-0.0498974366850414));
#59044=DIRECTION('center_axis',(-0.284551435696759,0.958262022045047,0.0276473787012793));
#59045=DIRECTION('ref_axis',(0.958660774436356,0.284433077286297,0.008206345260477));
#59046=DIRECTION('',(0.0161503784824051,0.0336272827279992,-0.999303943318151));
#59047=DIRECTION('center_axis',(-0.0617712249622997,-0.997491655456914,
-0.0345646215150937));
#59048=DIRECTION('ref_axis',(-0.998052578482889,0.0614306198252359,0.0108318757168334));
#59049=DIRECTION('center_axis',(0.0617712249622997,0.997491655456914,0.0345646215150937));
#59050=DIRECTION('ref_axis',(-0.998090334472114,0.061734173069449,0.00213918413755088));
#59051=DIRECTION('',(-0.137998583506848,0.0428336755604254,-0.989505769153514));
#59052=DIRECTION('center_axis',(-0.99026806874157,-0.0241671553619711,0.137058748836224));
#59053=DIRECTION('ref_axis',(0.,0.984807753012208,0.17364817766693));
#59054=DIRECTION('center_axis',(0.99026806874157,0.0241671553619711,-0.137058748836224));
#59055=DIRECTION('ref_axis',(-0.139173100960066,0.171958245538724,-0.975223671657125));
#59056=DIRECTION('',(-0.137844537491629,0.0345663418322999,-0.989850519773593));
#59057=DIRECTION('center_axis',(0.,-0.999390827019096,-0.0348994967025006));
#59058=DIRECTION('ref_axis',(-1.,0.,0.));
#59059=DIRECTION('',(-1.,0.,0.));
#59060=DIRECTION('center_axis',(0.,0.17364817766693,-0.984807753012208));
#59061=DIRECTION('ref_axis',(1.,0.,0.));
#59062=DIRECTION('center_axis',(1.,0.,0.));
#59063=DIRECTION('ref_axis',(0.,1.,0.));
#59064=DIRECTION('center_axis',(1.,0.,0.));
#59065=DIRECTION('ref_axis',(0.,0.,-1.));
#59066=DIRECTION('center_axis',(0.649305557988371,-0.747685187986609,-0.139173100960065));
#59067=DIRECTION('ref_axis',(0.760527640763576,0.638341228068795,0.118819965419165));
#59068=DIRECTION('',(1.,0.,0.));
#59069=DIRECTION('center_axis',(-0.99026806874157,-2.55656838927233E-17,
-0.139173100960065));
#59070=DIRECTION('ref_axis',(-0.139173100960065,0.,0.99026806874157));
#59071=DIRECTION('center_axis',(-0.0617712249622996,-0.988339599396795,
-0.139173100960065));
#59072=DIRECTION('ref_axis',(-0.998090334472114,0.0611677576917705,0.00861334152950384));
#59073=DIRECTION('center_axis',(0.284551435696759,-0.948504785655862,-0.139173100960065));
#59074=DIRECTION('ref_axis',(0.958660774436356,0.281536916624453,0.0413096131025498));
#59075=DIRECTION('center_axis',(0.491310548314114,-0.859793459549701,-0.139173100960065));
#59076=DIRECTION('ref_axis',(0.870984468928858,0.484997851417207,0.0785056622506208));
#59077=DIRECTION('center_axis',(0.313150259135956,-0.939450777407866,-0.139173100960065));
#59078=DIRECTION('ref_axis',(0.949703593340092,0.309769549629784,0.0458902050450514));
#59079=DIRECTION('',(1.,0.,0.));
#59080=DIRECTION('center_axis',(-0.313150259135957,-0.939450777407865,-0.139173100960065));
#59081=DIRECTION('ref_axis',(-0.949703593340092,0.309769549629785,0.0458902050450517));
#59082=DIRECTION('center_axis',(-0.491310548314113,-0.859793459549702,-0.139173100960065));
#59083=DIRECTION('ref_axis',(-0.870984468928858,0.484997851417206,0.0785056622506207));
#59084=DIRECTION('center_axis',(-0.284551435696759,-0.948504785655862,-0.139173100960065));
#59085=DIRECTION('ref_axis',(-0.958660774436356,0.281536916624453,0.0413096131025497));
#59086=DIRECTION('center_axis',(0.0617712249622997,-0.988339599396795,-0.139173100960065));
#59087=DIRECTION('ref_axis',(0.998090334472114,0.0611677576917706,0.00861334152950384));
#59088=DIRECTION('center_axis',(0.99026806874157,-2.55656838927234E-17,
-0.139173100960066));
#59089=DIRECTION('ref_axis',(0.139173100960066,0.,0.99026806874157));
#59090=DIRECTION('',(1.,0.,0.));
#59091=DIRECTION('center_axis',(0.,0.99026806874157,0.139173100960065));
#59092=DIRECTION('ref_axis',(1.,0.,0.));
#59093=DIRECTION('',(-0.137844537491629,0.137844537491629,-0.980814848463989));
#59094=DIRECTION('center_axis',(-0.99026806874157,2.55656838927234E-17,
0.139173100960066));
#59095=DIRECTION('ref_axis',(0.,1.,-1.83697019872103E-16));
#59096=DIRECTION('',(-0.137998583506848,0.129642937822505,-0.981910942816534));
#59097=DIRECTION('center_axis',(-0.0617712249622997,0.988339599396795,0.139173100960065));
#59098=DIRECTION('ref_axis',(0.998052578482889,0.0623782861551806,-1.14587052714359E-17));
#59099=DIRECTION('',(0.0161503784824051,0.140410899949307,-0.989961587360995));
#59100=DIRECTION('center_axis',(0.284551435696759,0.948504785655862,0.139173100960065));
#59101=DIRECTION('ref_axis',(0.957826285221151,-0.287347885566345,5.27849502450877E-17));
#59102=DIRECTION('',(0.0552259184163645,0.128714814516259,-0.990142714187765));
#59103=DIRECTION('center_axis',(0.491310548314113,0.859793459549702,0.139173100960065));
#59104=DIRECTION('ref_axis',(0.86824314212446,-0.496138938356832,9.11392444186591E-17));
#59105=DIRECTION('',(0.057078643955053,0.12766118652195,-0.99017405028614));
#59106=DIRECTION('center_axis',(0.313150259135957,0.939450777407865,0.139173100960065));
#59107=DIRECTION('ref_axis',(0.948683298050513,-0.31622776601684,5.80900982181061E-17));
#59108=DIRECTION('',(0.0225789275220278,0.13913762065955,-0.990015613285545));
#59109=DIRECTION('center_axis',(0.,0.99026806874157,0.139173100960065));
#59110=DIRECTION('ref_axis',(1.,0.,0.));
#59111=DIRECTION('',(-0.0225789275220274,0.13913762065955,-0.990015613285545));
#59112=DIRECTION('center_axis',(-0.313150259135956,0.939450777407866,0.139173100960065));
#59113=DIRECTION('ref_axis',(0.948683298050514,0.316227766016839,-5.80900982181059E-17));
#59114=DIRECTION('',(-0.0570786439550527,0.12766118652195,-0.99017405028614));
#59115=DIRECTION('center_axis',(-0.491310548314114,0.859793459549701,0.139173100960065));
#59116=DIRECTION('ref_axis',(0.868243142124459,0.496138938356833,-9.11392444186592E-17));
#59117=DIRECTION('',(-0.0552259184163635,0.128714814516259,-0.990142714187765));
#59118=DIRECTION('center_axis',(-0.284551435696759,0.948504785655862,0.139173100960065));
#59119=DIRECTION('ref_axis',(0.957826285221151,0.287347885566346,-5.27849502450878E-17));
#59120=DIRECTION('',(-0.0161503784824052,0.140410899949307,-0.989961587360995));
#59121=DIRECTION('center_axis',(0.0617712249622996,0.988339599396795,0.139173100960065));
#59122=DIRECTION('ref_axis',(0.998052578482889,-0.0623782861551805,1.14587052714359E-17));
#59123=DIRECTION('',(0.137998583506848,0.129642937822505,-0.981910942816534));
#59124=DIRECTION('center_axis',(0.99026806874157,2.55656838927233E-17,0.139173100960065));
#59125=DIRECTION('ref_axis',(0.,-1.,1.83697019872103E-16));
#59126=DIRECTION('',(0.137844537491629,0.137844537491628,-0.980814848463989));
#59127=DIRECTION('center_axis',(0.,0.99026806874157,0.139173100960065));
#59128=DIRECTION('ref_axis',(1.,0.,0.));
#59129=DIRECTION('',(-0.051925424877728,0.138985351600606,-0.98893216263388));
#59130=DIRECTION('center_axis',(-0.649305557988371,0.747685187986609,0.139173100960065));
#59131=DIRECTION('ref_axis',(0.755033118392644,0.655686655446243,-1.20447684575381E-16));
#59132=DIRECTION('center_axis',(0.,-0.99026806874157,0.139173100960066));
#59133=DIRECTION('ref_axis',(-1.,0.,0.));
#59134=DIRECTION('',(-1.,0.,0.));
#59135=DIRECTION('',(0.137844537491629,-0.137844537491629,-0.980814848463989));
#59136=DIRECTION('center_axis',(0.99026806874157,2.55656838927233E-17,0.139173100960065));
#59137=DIRECTION('ref_axis',(0.,-1.,1.83697019872103E-16));
#59138=DIRECTION('center_axis',(-0.99026806874157,-2.55656838927233E-17,
-0.139173100960065));
#59139=DIRECTION('ref_axis',(-0.139173100960065,0.,0.99026806874157));
#59140=DIRECTION('',(0.137998583506848,-0.129642937822505,-0.981910942816534));
#59141=DIRECTION('center_axis',(0.0617712249622996,-0.988339599396795,0.139173100960066));
#59142=DIRECTION('ref_axis',(-0.998052578482889,-0.0623782861551805,1.14587052714359E-17));
#59143=DIRECTION('center_axis',(-0.0617712249622996,0.988339599396795,-0.139173100960066));
#59144=DIRECTION('ref_axis',(0.998090334472114,0.0611677576917705,-0.00861334152950386));
#59145=DIRECTION('',(-0.0161503784824054,-0.140410899949307,-0.989961587360995));
#59146=DIRECTION('center_axis',(-0.284551435696759,-0.948504785655862,0.139173100960066));
#59147=DIRECTION('ref_axis',(-0.957826285221151,0.287347885566346,-5.27849502450878E-17));
#59148=DIRECTION('center_axis',(0.284551435696759,0.948504785655862,-0.139173100960066));
#59149=DIRECTION('ref_axis',(-0.958660774436356,0.281536916624453,-0.0413096131025499));
#59150=DIRECTION('',(-0.0552259184163638,-0.12871481451626,-0.990142714187765));
#59151=DIRECTION('center_axis',(-0.491310548314114,-0.859793459549701,0.139173100960066));
#59152=DIRECTION('ref_axis',(-0.868243142124459,0.496138938356833,-9.11392444186592E-17));
#59153=DIRECTION('center_axis',(0.491310548314114,0.859793459549701,-0.139173100960066));
#59154=DIRECTION('ref_axis',(-0.870984468928858,0.484997851417207,-0.078505662250621));
#59155=DIRECTION('',(-0.0570786439550532,-0.12766118652195,-0.99017405028614));
#59156=DIRECTION('center_axis',(-0.313150259135956,-0.939450777407866,0.139173100960066));
#59157=DIRECTION('ref_axis',(-0.948683298050514,0.316227766016839,-5.80900982181059E-17));
#59158=DIRECTION('center_axis',(0.313150259135956,0.939450777407866,-0.139173100960066));
#59159=DIRECTION('ref_axis',(-0.949703593340092,0.309769549629784,-0.0458902050450515));
#59160=DIRECTION('',(-0.0225789275220273,-0.139137620659551,-0.990015613285545));
#59161=DIRECTION('center_axis',(0.,-0.99026806874157,0.139173100960066));
#59162=DIRECTION('ref_axis',(-1.,0.,0.));
#59163=DIRECTION('',(-1.,0.,0.));
#59164=DIRECTION('',(0.0225789275220281,-0.139137620659551,-0.990015613285545));
#59165=DIRECTION('center_axis',(0.313150259135957,-0.939450777407865,0.139173100960066));
#59166=DIRECTION('ref_axis',(-0.948683298050513,-0.31622776601684,5.80900982181061E-17));
#59167=DIRECTION('center_axis',(-0.313150259135957,0.939450777407865,-0.139173100960066));
#59168=DIRECTION('ref_axis',(0.949703593340092,0.309769549629785,-0.0458902050450518));
#59169=DIRECTION('',(0.0570786439550534,-0.12766118652195,-0.99017405028614));
#59170=DIRECTION('center_axis',(0.491310548314113,-0.859793459549702,0.139173100960066));
#59171=DIRECTION('ref_axis',(-0.86824314212446,-0.496138938356832,9.11392444186591E-17));
#59172=DIRECTION('center_axis',(-0.491310548314113,0.859793459549702,-0.139173100960066));
#59173=DIRECTION('ref_axis',(0.870984468928858,0.484997851417206,-0.0785056622506209));
#59174=DIRECTION('',(0.0552259184163649,-0.128714814516259,-0.990142714187765));
#59175=DIRECTION('center_axis',(0.284551435696759,-0.948504785655862,0.139173100960066));
#59176=DIRECTION('ref_axis',(-0.957826285221151,-0.287347885566345,5.27849502450877E-17));
#59177=DIRECTION('center_axis',(-0.284551435696759,0.948504785655862,-0.139173100960066));
#59178=DIRECTION('ref_axis',(0.958660774436356,0.281536916624453,-0.0413096131025498));
#59179=DIRECTION('',(0.0161503784824051,-0.140410899949307,-0.989961587360995));
#59180=DIRECTION('center_axis',(-0.0617712249622997,-0.988339599396795,
0.139173100960066));
#59181=DIRECTION('ref_axis',(-0.998052578482889,0.0623782861551806,-1.14587052714359E-17));
#59182=DIRECTION('center_axis',(0.0617712249622997,0.988339599396795,-0.139173100960066));
#59183=DIRECTION('ref_axis',(-0.998090334472114,0.0611677576917706,-0.00861334152950387));
#59184=DIRECTION('',(-0.137998583506848,-0.129642937822505,-0.981910942816533));
#59185=DIRECTION('center_axis',(-0.99026806874157,2.55656838927234E-17,
0.139173100960066));
#59186=DIRECTION('ref_axis',(0.,1.,-1.83697019872103E-16));
#59187=DIRECTION('center_axis',(0.99026806874157,-2.55656838927234E-17,
-0.139173100960066));
#59188=DIRECTION('ref_axis',(0.139173100960066,0.,0.99026806874157));
#59189=DIRECTION('',(-0.137844537491629,-0.137844537491629,-0.980814848463989));
#59190=DIRECTION('center_axis',(0.,-0.99026806874157,0.139173100960066));
#59191=DIRECTION('ref_axis',(-1.,0.,0.));
#59192=DIRECTION('',(-1.,0.,0.));
#59193=DIRECTION('center_axis',(0.,-1.83697019872103E-16,-1.));
#59194=DIRECTION('ref_axis',(1.,0.,0.));
#59195=DIRECTION('center_axis',(1.,0.,0.));
#59196=DIRECTION('ref_axis',(0.,1.,0.));
#59197=DIRECTION('center_axis',(1.,0.,0.));
#59198=DIRECTION('ref_axis',(0.,0.,-1.));
#59199=DIRECTION('center_axis',(0.64930555798837,-0.760493325303574,-0.00722457847379238));
#59200=DIRECTION('ref_axis',(0.760527640763576,0.649276260934969,0.00616803217361931));
#59201=DIRECTION('',(1.,0.,0.));
#59202=DIRECTION('center_axis',(-0.99026806874157,-0.0241671553619711,-0.137058748836223));
#59203=DIRECTION('ref_axis',(-0.139173100960065,0.171958245538723,0.975223671657125));
#59204=DIRECTION('center_axis',(-0.0617712249622996,-0.997491655456914,
0.0345646215150941));
#59205=DIRECTION('ref_axis',(-0.998090334472114,0.061734173069449,-0.0021391841375509));
#59206=DIRECTION('center_axis',(0.284551435696759,-0.958262022045047,0.0276473787012795));
#59207=DIRECTION('ref_axis',(0.958660774436356,0.284433077286297,-0.00820634526047709));
#59208=DIRECTION('center_axis',(0.491310548314114,-0.870898420315705,0.012242818584528));
#59209=DIRECTION('ref_axis',(0.870984468928858,0.491262009456284,-0.00690600823120533));
#59210=DIRECTION('center_axis',(0.313150259135956,-0.949345564526583,0.0260751666684337));
#59211=DIRECTION('ref_axis',(0.949703593340092,0.313032204601347,-0.00859788807423114));
#59212=DIRECTION('',(1.,0.,0.));
#59213=DIRECTION('center_axis',(-0.313150259135957,-0.949345564526583,0.0260751666684335));
#59214=DIRECTION('ref_axis',(-0.949703593340092,0.313032204601348,-0.00859788807423111));
#59215=DIRECTION('center_axis',(-0.491310548314113,-0.870898420315706,0.012242818584528));
#59216=DIRECTION('ref_axis',(-0.870984468928858,0.491262009456283,-0.00690600823120528));
#59217=DIRECTION('center_axis',(-0.284551435696759,-0.958262022045047,0.0276473787012796));
#59218=DIRECTION('ref_axis',(-0.958660774436356,0.284433077286297,-0.00820634526047711));
#59219=DIRECTION('center_axis',(0.0617712249622997,-0.997491655456914,0.0345646215150942));
#59220=DIRECTION('ref_axis',(0.998090334472114,0.061734173069449,-0.00213918413755091));
#59221=DIRECTION('center_axis',(0.99026806874157,-0.0241671553619711,-0.137058748836224));
#59222=DIRECTION('ref_axis',(0.139173100960066,0.171958245538724,0.975223671657125));
#59223=DIRECTION('',(1.,0.,0.));
#59224=DIRECTION('center_axis',(0.,0.999390827019096,-0.0348994967025008));
#59225=DIRECTION('ref_axis',(1.,0.,0.));
#59226=DIRECTION('',(-0.137844537491629,-0.0345663418323001,-0.989850519773593));
#59227=DIRECTION('center_axis',(-0.99026806874157,0.0241671553619711,0.137058748836224));
#59228=DIRECTION('ref_axis',(0.,0.984807753012208,-0.17364817766693));
#59229=DIRECTION('',(-0.137998583506848,-0.0428336755604259,-0.989505769153514));
#59230=DIRECTION('center_axis',(-0.0617712249622997,0.997491655456914,-0.0345646215150942));
#59231=DIRECTION('ref_axis',(0.998052578482889,0.0614306198252359,-0.0108318757168334));
#59232=DIRECTION('',(0.0161503784824051,-0.0336272827279996,-0.999303943318151));
#59233=DIRECTION('center_axis',(0.284551435696759,0.958262022045047,-0.0276473787012796));
#59234=DIRECTION('ref_axis',(0.957826285221151,-0.282982425517402,0.0498974366850415));
#59235=DIRECTION('',(0.0552259184163645,-0.0451771306857534,-0.997451314500147));
#59236=DIRECTION('center_axis',(0.491310548314113,0.870898420315706,-0.012242818584528));
#59237=DIRECTION('ref_axis',(0.86824314212446,-0.488601473065054,0.0861536225152694));
#59238=DIRECTION('',(0.057078643955053,-0.0462201931597181,-0.997299213951626));
#59239=DIRECTION('center_axis',(0.313150259135957,0.949345564526583,-0.0260751666684335));
#59240=DIRECTION('ref_axis',(0.948683298050513,-0.311423555691114,0.0549123752965087));
#59241=DIRECTION('',(0.0225789275220278,-0.0348905995476464,-0.999136045839184));
#59242=DIRECTION('center_axis',(0.,0.999390827019096,-0.0348994967025009));
#59243=DIRECTION('ref_axis',(1.,0.,0.));
#59244=DIRECTION('',(-0.0225789275220274,-0.0348905995476464,-0.999136045839184));
#59245=DIRECTION('center_axis',(-0.313150259135956,0.949345564526583,-0.0260751666684337));
#59246=DIRECTION('ref_axis',(0.948683298050514,0.311423555691113,-0.0549123752965085));
#59247=DIRECTION('',(-0.0570786439550527,-0.046220193159718,-0.997299213951626));
#59248=DIRECTION('center_axis',(-0.491310548314114,0.870898420315705,-0.012242818584528));
#59249=DIRECTION('ref_axis',(0.868243142124459,0.488601473065055,-0.0861536225152696));
#59250=DIRECTION('',(-0.0552259184163635,-0.0451771306857529,-0.997451314500147));
#59251=DIRECTION('center_axis',(-0.284551435696759,0.958262022045047,-0.0276473787012795));
#59252=DIRECTION('ref_axis',(0.957826285221151,0.282982425517402,-0.0498974366850416));
#59253=DIRECTION('',(-0.0161503784824052,-0.0336272827279995,-0.999303943318151));
#59254=DIRECTION('center_axis',(0.0617712249622996,0.997491655456914,-0.0345646215150941));
#59255=DIRECTION('ref_axis',(0.998052578482889,-0.0614306198252359,0.0108318757168334));
#59256=DIRECTION('',(0.137998583506848,-0.0428336755604257,-0.989505769153514));
#59257=DIRECTION('center_axis',(0.99026806874157,0.0241671553619711,0.137058748836223));
#59258=DIRECTION('ref_axis',(0.,-0.984807753012208,0.17364817766693));
#59259=DIRECTION('',(0.137844537491629,-0.0345663418323003,-0.989850519773593));
#59260=DIRECTION('center_axis',(0.,0.999390827019096,-0.0348994967025009));
#59261=DIRECTION('ref_axis',(1.,0.,0.));
#59262=DIRECTION('',(-0.051925424877728,-0.0348524160661845,-0.998042613992818));
#59263=DIRECTION('center_axis',(-0.64930555798837,0.760493325303574,0.00722457847379238));
#59264=DIRECTION('ref_axis',(0.755033118392644,0.645725301830105,-0.113858792838765));
#59265=DIRECTION('center_axis',(0.,-0.951056516295154,0.309016994374947));
#59266=DIRECTION('ref_axis',(-1.,0.,0.));
#59267=DIRECTION('',(-1.,0.,0.));
#59268=DIRECTION('',(0.137844537491629,-0.306067080296576,-0.941977614300068));
#59269=DIRECTION('center_axis',(0.99026806874157,0.0241671553619711,0.137058748836223));
#59270=DIRECTION('ref_axis',(0.,-0.984807753012208,0.17364817766693));
#59271=DIRECTION('center_axis',(-0.99026806874157,-0.0241671553619711,-0.137058748836223));
#59272=DIRECTION('ref_axis',(-0.139173100960065,0.171958245538723,0.975223671657125));
#59273=DIRECTION('',(0.137998583506848,-0.298180416142191,-0.944481249352984));
#59274=DIRECTION('center_axis',(0.0617712249622996,-0.949157344732972,0.308682119187541));
#59275=DIRECTION('ref_axis',(-0.998052578482889,-0.0614306198252359,0.0108318757168334));
#59276=DIRECTION('center_axis',(-0.0617712249622996,0.949157344732972,-0.308682119187541));
#59277=DIRECTION('ref_axis',(0.998090334472114,0.0587427909490065,-0.0191041551727457));
#59278=DIRECTION('',(-0.0161503784824054,-0.310182768482997,-0.950539749516609));
#59279=DIRECTION('center_axis',(-0.284551435696759,-0.909927711321104,0.301764876373726));
#59280=DIRECTION('ref_axis',(-0.957826285221151,0.282982425517402,-0.0498974366850416));
#59281=DIRECTION('center_axis',(0.284551435696759,0.909927711321104,-0.301764876373726));
#59282=DIRECTION('ref_axis',(-0.958660774436356,0.27008639921553,-0.0895703997751286));
#59283=DIRECTION('',(-0.0552259184163638,-0.298695825212034,-0.952749128541176));
#59284=DIRECTION('center_axis',(-0.491310548314114,-0.822564109591763,0.286360316256975));
#59285=DIRECTION('ref_axis',(-0.868243142124459,0.488601473065055,-0.0861536225152696));
#59286=DIRECTION('center_axis',(0.491310548314114,0.822564109591763,-0.286360316256975));
#59287=DIRECTION('ref_axis',(-0.870984468928858,0.463997279083572,-0.161531977910744));
#59288=DIRECTION('',(-0.0570786439550532,-0.297663645650825,-0.952962949154956));
#59289=DIRECTION('center_axis',(-0.313150259135956,-0.901011253802641,0.30019266434088));
#59290=DIRECTION('ref_axis',(-0.948683298050514,0.311423555691113,-0.0549123752965085));
#59291=DIRECTION('center_axis',(0.313150259135956,0.901011253802641,-0.30019266434088));
#59292=DIRECTION('ref_axis',(-0.949703593340092,0.297094703643677,-0.0989839475056044));
#59293=DIRECTION('',(-0.0225789275220273,-0.30893821467004,-0.950814057294297));
#59294=DIRECTION('center_axis',(0.,-0.951056516295154,0.309016994374947));
#59295=DIRECTION('ref_axis',(-1.,0.,0.));
#59296=DIRECTION('',(-1.,0.,0.));
#59297=DIRECTION('',(0.0225789275220281,-0.30893821467004,-0.950814057294297));
#59298=DIRECTION('center_axis',(0.313150259135957,-0.901011253802641,0.30019266434088));
#59299=DIRECTION('ref_axis',(-0.948683298050513,-0.311423555691114,0.0549123752965087));
#59300=DIRECTION('center_axis',(-0.313150259135957,0.901011253802641,-0.30019266434088));
#59301=DIRECTION('ref_axis',(0.949703593340092,0.297094703643678,-0.0989839475056049));
#59302=DIRECTION('',(0.0570786439550533,-0.297663645650825,-0.952962949154956));
#59303=DIRECTION('center_axis',(0.491310548314113,-0.822564109591764,0.286360316256975));
#59304=DIRECTION('ref_axis',(-0.86824314212446,-0.488601473065054,0.0861536225152694));
#59305=DIRECTION('center_axis',(-0.491310548314113,0.822564109591764,-0.286360316256975));
#59306=DIRECTION('ref_axis',(0.870984468928858,0.463997279083571,-0.161531977910744));
#59307=DIRECTION('',(0.0552259184163649,-0.298695825212034,-0.952749128541176));
#59308=DIRECTION('center_axis',(0.284551435696759,-0.909927711321105,0.301764876373726));
#59309=DIRECTION('ref_axis',(-0.957826285221151,-0.282982425517402,0.0498974366850415));
#59310=DIRECTION('center_axis',(-0.284551435696759,0.909927711321105,-0.301764876373726));
#59311=DIRECTION('ref_axis',(0.958660774436356,0.270086399215529,-0.0895703997751284));
#59312=DIRECTION('',(0.0161503784824051,-0.310182768482997,-0.950539749516609));
#59313=DIRECTION('center_axis',(-0.0617712249622997,-0.949157344732972,
0.308682119187541));
#59314=DIRECTION('ref_axis',(-0.998052578482889,0.0614306198252359,-0.0108318757168334));
#59315=DIRECTION('center_axis',(0.0617712249622997,0.949157344732972,-0.308682119187541));
#59316=DIRECTION('ref_axis',(-0.998090334472114,0.0587427909490066,-0.0191041551727457));
#59317=DIRECTION('',(-0.137998583506848,-0.298180416142191,-0.944481249352984));
#59318=DIRECTION('center_axis',(-0.99026806874157,0.0241671553619711,0.137058748836224));
#59319=DIRECTION('ref_axis',(0.,0.984807753012208,-0.17364817766693));
#59320=DIRECTION('center_axis',(0.99026806874157,-0.0241671553619711,-0.137058748836224));
#59321=DIRECTION('ref_axis',(0.139173100960066,0.171958245538724,0.975223671657125));
#59322=DIRECTION('',(-0.137844537491629,-0.306067080296576,-0.941977614300068));
#59323=DIRECTION('center_axis',(0.,-0.951056516295154,0.309016994374948));
#59324=DIRECTION('ref_axis',(-1.,0.,0.));
#59325=DIRECTION('',(-1.,0.,0.));
#59326=DIRECTION('center_axis',(0.,-0.17364817766693,-0.984807753012208));
#59327=DIRECTION('ref_axis',(1.,0.,0.));
#59328=DIRECTION('center_axis',(1.,0.,0.));
#59329=DIRECTION('ref_axis',(0.,1.,0.));
#59330=DIRECTION('center_axis',(1.,0.,0.));
#59331=DIRECTION('ref_axis',(0.,0.,-1.));
#59332=DIRECTION('center_axis',(0.64930555798837,-0.75019425775938,0.124943459173594));
#59333=DIRECTION('ref_axis',(0.760527640763576,0.640483363162275,-0.106671313608347));
#59334=DIRECTION('',(1.,0.,0.));
#59335=DIRECTION('center_axis',(-0.99026806874157,-0.0476000039374394,-0.130779935984066));
#59336=DIRECTION('ref_axis',(-0.139173100960065,0.338691626801824,0.930547596796367));
#59337=DIRECTION('center_axis',(-0.0617712249622996,-0.976335432321108,
0.207252115456061));
#59338=DIRECTION('ref_axis',(-0.998090334472114,0.0604248268374111,-0.0128267117770656));
#59339=DIRECTION('center_axis',(0.284551435696759,-0.938902951798372,0.193627806751035));
#59340=DIRECTION('ref_axis',(0.958660774436356,0.278686882824878,-0.0574729579753757));
#59341=DIRECTION('center_axis',(0.491310548314114,-0.855541573276281,0.163286746281596));
#59342=DIRECTION('ref_axis',(0.870984468928858,0.482599419928604,-0.0921078431475355));
#59343=DIRECTION('center_axis',(0.313150259135956,-0.930394967059196,0.190531153552384));
#59344=DIRECTION('ref_axis',(0.949703593340092,0.306783534438035,-0.0628247387151197));
#59345=DIRECTION('',(1.,0.,0.));
#59346=DIRECTION('center_axis',(-0.313150259135957,-0.930394967059195,0.190531153552384));
#59347=DIRECTION('ref_axis',(-0.949703593340092,0.306783534438037,-0.0628247387151199));
#59348=DIRECTION('center_axis',(-0.491310548314113,-0.855541573276282,0.163286746281596));
#59349=DIRECTION('ref_axis',(-0.870984468928858,0.482599419928602,-0.0921078431475352));
#59350=DIRECTION('center_axis',(-0.284551435696759,-0.938902951798373,0.193627806751036));
#59351=DIRECTION('ref_axis',(-0.958660774436356,0.278686882824878,-0.0574729579753756));
#59352=DIRECTION('center_axis',(0.0617712249622997,-0.976335432321108,0.207252115456061));
#59353=DIRECTION('ref_axis',(0.998090334472114,0.0604248268374111,-0.0128267117770656));
#59354=DIRECTION('center_axis',(0.99026806874157,-0.0476000039374395,-0.130779935984066));
#59355=DIRECTION('ref_axis',(0.139173100960066,0.338691626801825,0.930547596796366));
#59356=DIRECTION('',(1.,0.,0.));
#59357=DIRECTION('center_axis',(0.,0.978147600733806,-0.20791169081776));
#59358=DIRECTION('ref_axis',(1.,0.,0.));
#59359=DIRECTION('',(-0.137844537491629,-0.205926940351068,-0.968810083928407));
#59360=DIRECTION('center_axis',(-0.99026806874157,0.0476000039374395,0.130779935984066));
#59361=DIRECTION('ref_axis',(0.,0.939692620785908,-0.342020143325669));
#59362=DIRECTION('',(-0.137998583506848,-0.21400880938634,-0.967034963408844));
#59363=DIRECTION('center_axis',(-0.0617712249622997,0.976335432321108,-0.207252115456061));
#59364=DIRECTION('ref_axis',(0.998052578482889,0.058616415197295,-0.0213346303712045));
#59365=DIRECTION('',(0.0161503784824051,-0.206643717435843,-0.978282954629779));
#59366=DIRECTION('center_axis',(0.284551435696759,0.938902951798373,-0.193627806751036));
#59367=DIRECTION('ref_axis',(0.957826285221151,-0.270018687665128,0.0982787650057295));
#59368=DIRECTION('',(0.0552259184163645,-0.217696391632611,-0.974452861356161));
#59369=DIRECTION('center_axis',(0.491310548314113,0.855541573276282,-0.163286746281596));
#59370=DIRECTION('ref_axis',(0.86824314212446,-0.46621809925847,0.169689510806249));
#59371=DIRECTION('',(0.057078643955053,-0.218697195660775,-0.974121945658943));
#59372=DIRECTION('center_axis',(0.313150259135957,0.930394967059195,-0.190531153552384));
#59373=DIRECTION('ref_axis',(0.948683298050513,-0.297156898213637,0.108156265856636));
#59374=DIRECTION('',(0.0225789275220278,-0.207858686543084,-0.977898235227234));
#59375=DIRECTION('center_axis',(0.,0.978147600733806,-0.20791169081776));
#59376=DIRECTION('ref_axis',(1.,0.,0.));
#59377=DIRECTION('',(-0.0225789275220274,-0.207858686543084,-0.977898235227234));
#59378=DIRECTION('center_axis',(-0.313150259135956,0.930394967059196,-0.190531153552384));
#59379=DIRECTION('ref_axis',(0.948683298050514,0.297156898213636,-0.108156265856635));
#59380=DIRECTION('',(-0.0570786439550527,-0.218697195660775,-0.974121945658943));
#59381=DIRECTION('center_axis',(-0.491310548314114,0.855541573276281,-0.163286746281596));
#59382=DIRECTION('ref_axis',(0.868243142124459,0.466218099258471,-0.16968951080625));
#59383=DIRECTION('',(-0.0552259184163635,-0.217696391632611,-0.974452861356161));
#59384=DIRECTION('center_axis',(-0.284551435696759,0.938902951798372,-0.193627806751035));
#59385=DIRECTION('ref_axis',(0.957826285221151,0.270018687665129,-0.0982787650057297));
#59386=DIRECTION('',(-0.0161503784824052,-0.206643717435842,-0.978282954629779));
#59387=DIRECTION('center_axis',(0.0617712249622996,0.976335432321108,-0.207252115456061));
#59388=DIRECTION('ref_axis',(0.998052578482889,-0.0586164151972949,0.0213346303712045));
#59389=DIRECTION('',(0.137998583506848,-0.214008809386339,-0.967034963408844));
#59390=DIRECTION('center_axis',(0.99026806874157,0.0476000039374394,0.130779935984066));
#59391=DIRECTION('ref_axis',(0.,-0.939692620785908,0.342020143325669));
#59392=DIRECTION('',(0.137844537491629,-0.205926940351068,-0.968810083928407));
#59393=DIRECTION('center_axis',(0.,0.978147600733805,-0.20791169081776));
#59394=DIRECTION('ref_axis',(1.,0.,0.));
#59395=DIRECTION('',(-0.0519254248777279,-0.207631210706979,-0.976828045559515));
#59396=DIRECTION('center_axis',(-0.64930555798837,0.75019425775938,-0.124943459173594));
#59397=DIRECTION('ref_axis',(0.755033118392644,0.616143911670627,-0.224258043872453));
#59398=DIRECTION('center_axis',(0.,-0.882947592858927,0.469471562785891));
#59399=DIRECTION('ref_axis',(-1.,0.,0.));
#59400=DIRECTION('',(-1.,0.,0.));
#59401=DIRECTION('',(0.137844537491629,-0.464989929744128,-0.874518866989312));
#59402=DIRECTION('center_axis',(0.99026806874157,0.0476000039374394,0.130779935984066));
#59403=DIRECTION('ref_axis',(0.,-0.939692620785908,0.342020143325669));
#59404=DIRECTION('center_axis',(-0.99026806874157,-0.0476000039374394,-0.130779935984066));
#59405=DIRECTION('ref_axis',(-0.139173100960065,0.338691626801824,0.930547596796367));
#59406=DIRECTION('',(0.137998583506848,-0.457657833403968,-0.878353971058416));
#59407=DIRECTION('center_axis',(0.0617712249622996,-0.881135424446229,0.468811987424192));
#59408=DIRECTION('ref_axis',(-0.998052578482889,-0.0586164151972949,0.0213346303712045));
#59409=DIRECTION('center_axis',(-0.0617712249622996,0.881135424446229,-0.468811987424192));
#59410=DIRECTION('ref_axis',(0.998090334472114,0.0545329542285434,-0.0290144987282327));
#59411=DIRECTION('',(-0.0161503784824054,-0.470529890556387,-0.882236242379483));
#59412=DIRECTION('center_axis',(-0.284551435696759,-0.843702943923494,0.455187678719167));
#59413=DIRECTION('ref_axis',(-0.957826285221151,0.270018687665129,-0.0982787650057297));
#59414=DIRECTION('center_axis',(0.284551435696759,0.843702943923494,-0.455187678719167));
#59415=DIRECTION('ref_axis',(-0.958660774436356,0.250429443236754,-0.13510963517535));
#59416=DIRECTION('',(-0.0552259184163638,-0.459601114406123,-0.886406742738185));
#59417=DIRECTION('center_axis',(-0.491310548314114,-0.760341565401402,0.424846618249728));
#59418=DIRECTION('ref_axis',(-0.868243142124459,0.466218099258471,-0.16968951080625));
#59419=DIRECTION('center_axis',(0.491310548314114,0.760341565401402,-0.424846618249728));
#59420=DIRECTION('ref_axis',(-0.870984468928858,0.428898384218936,-0.239650226161174));
#59421=DIRECTION('',(-0.0570786439550532,-0.458621745531674,-0.886796551036219));
#59422=DIRECTION('center_axis',(-0.313150259135956,-0.835194959184317,0.452091025520515));
#59423=DIRECTION('ref_axis',(-0.948683298050514,0.297156898213636,-0.108156265856635));
#59424=DIRECTION('center_axis',(0.313150259135956,0.835194959184317,-0.452091025520515));
#59425=DIRECTION('ref_axis',(-0.949703593340092,0.27539278542453,-0.149070112809494));
#59426=DIRECTION('',(-0.0225789275220273,-0.469351877358061,-0.88272249730729));
#59427=DIRECTION('center_axis',(0.,-0.882947592858927,0.469471562785891));
#59428=DIRECTION('ref_axis',(-1.,0.,0.));
#59429=DIRECTION('',(-1.,0.,0.));
#59430=DIRECTION('',(0.0225789275220281,-0.469351877358061,-0.88272249730729));
#59431=DIRECTION('center_axis',(0.313150259135957,-0.835194959184316,0.452091025520515));
#59432=DIRECTION('ref_axis',(-0.948683298050513,-0.297156898213637,0.108156265856636));
#59433=DIRECTION('center_axis',(-0.313150259135957,0.835194959184316,-0.452091025520515));
#59434=DIRECTION('ref_axis',(0.949703593340092,0.275392785424531,-0.149070112809495));
#59435=DIRECTION('',(0.0570786439550534,-0.458621745531674,-0.886796551036219));
#59436=DIRECTION('center_axis',(0.491310548314113,-0.760341565401403,0.424846618249728));
#59437=DIRECTION('ref_axis',(-0.86824314212446,-0.46621809925847,0.169689510806249));
#59438=DIRECTION('center_axis',(-0.491310548314113,0.760341565401403,-0.424846618249728));
#59439=DIRECTION('ref_axis',(0.870984468928858,0.428898384218935,-0.239650226161174));
#59440=DIRECTION('',(0.0552259184163649,-0.459601114406122,-0.886406742738185));
#59441=DIRECTION('center_axis',(0.284551435696759,-0.843702943923494,0.455187678719167));
#59442=DIRECTION('ref_axis',(-0.957826285221151,-0.270018687665128,0.0982787650057295));
#59443=DIRECTION('center_axis',(-0.284551435696759,0.843702943923494,-0.455187678719167));
#59444=DIRECTION('ref_axis',(0.958660774436356,0.250429443236754,-0.135109635175349));
#59445=DIRECTION('',(0.0161503784824051,-0.470529890556387,-0.882236242379483));
#59446=DIRECTION('center_axis',(-0.0617712249622997,-0.881135424446229,
0.468811987424192));
#59447=DIRECTION('ref_axis',(-0.998052578482889,0.058616415197295,-0.0213346303712045));
#59448=DIRECTION('center_axis',(0.0617712249622997,0.881135424446229,-0.468811987424192));
#59449=DIRECTION('ref_axis',(-0.998090334472114,0.0545329542285434,-0.0290144987282328));
#59450=DIRECTION('',(-0.137998583506848,-0.457657833403968,-0.878353971058416));
#59451=DIRECTION('center_axis',(-0.99026806874157,0.0476000039374395,0.130779935984066));
#59452=DIRECTION('ref_axis',(0.,0.939692620785908,-0.342020143325669));
#59453=DIRECTION('center_axis',(0.99026806874157,-0.0476000039374395,-0.130779935984066));
#59454=DIRECTION('ref_axis',(0.139173100960066,0.338691626801825,0.930547596796366));
#59455=DIRECTION('',(-0.137844537491629,-0.464989929744128,-0.874518866989312));
#59456=DIRECTION('center_axis',(0.,-0.882947592858927,0.469471562785891));
#59457=DIRECTION('ref_axis',(-1.,0.,0.));
#59458=DIRECTION('',(-1.,0.,0.));
#59459=DIRECTION('center_axis',(0.,-0.342020143325669,-0.939692620785908));
#59460=DIRECTION('ref_axis',(1.,0.,0.));
#59461=DIRECTION('center_axis',(1.,0.,0.));
#59462=DIRECTION('ref_axis',(0.,1.,0.));
#59463=DIRECTION('center_axis',(1.,0.,0.));
#59464=DIRECTION('ref_axis',(0.,0.,-1.));
#59465=DIRECTION('center_axis',(0.64930555798837,-0.717100917309779,0.253315153038432));
#59466=DIRECTION('ref_axis',(0.760527640763576,0.612229702500115,-0.216269505504613));
#59467=DIRECTION('',(1.,0.,0.));
#59468=DIRECTION('center_axis',(-0.99026806874157,-0.0695865504800327,-0.120527440954873));
#59469=DIRECTION('ref_axis',(-0.139173100960065,0.495134034370783,0.857597304086756));
#59470=DIRECTION('center_axis',(-0.0617712249622996,-0.925513751123792,
0.373642358743525));
#59471=DIRECTION('ref_axis',(-0.998090334472114,0.0572795028183562,-0.0231245062698635));
#59472=DIRECTION('center_axis',(0.284551435696759,-0.891015790469123,0.353724951873058));
#59473=DIRECTION('ref_axis',(0.958660774436356,0.264472928451193,-0.104993283944912));
#59474=DIRECTION('center_axis',(0.491310548314114,-0.814189528457782,0.309369288819978));
#59475=DIRECTION('ref_axis',(0.870984468928858,0.459273291233482,-0.174511027858645));
#59476=DIRECTION('center_axis',(0.313150259135956,-0.883174789320284,0.34919794774906));
#59477=DIRECTION('ref_axis',(0.949703593340092,0.291213401820783,-0.115142691461001));
#59478=DIRECTION('',(1.,0.,0.));
#59479=DIRECTION('center_axis',(-0.313150259135957,-0.883174789320284,0.34919794774906));
#59480=DIRECTION('ref_axis',(-0.949703593340092,0.291213401820784,-0.115142691461001));
#59481=DIRECTION('center_axis',(-0.491310548314113,-0.814189528457783,0.309369288819978));
#59482=DIRECTION('ref_axis',(-0.870984468928858,0.459273291233481,-0.174511027858645));
#59483=DIRECTION('center_axis',(-0.284551435696759,-0.891015790469123,0.353724951873058));
#59484=DIRECTION('ref_axis',(-0.958660774436356,0.264472928451193,-0.104993283944912));
#59485=DIRECTION('center_axis',(0.0617712249622997,-0.925513751123792,0.373642358743525));
#59486=DIRECTION('ref_axis',(0.998090334472114,0.0572795028183562,-0.0231245062698635));
#59487=DIRECTION('center_axis',(0.99026806874157,-0.0695865504800329,-0.120527440954873));
#59488=DIRECTION('ref_axis',(0.139173100960066,0.495134034370784,0.857597304086755));
#59489=DIRECTION('',(1.,0.,0.));
#59490=DIRECTION('center_axis',(0.,0.927183854566787,-0.374606593415912));
#59491=DIRECTION('ref_axis',(1.,0.,0.));
#59492=DIRECTION('',(-0.137844537491629,-0.371030552991328,-0.918332843924613));
#59493=DIRECTION('center_axis',(-0.99026806874157,0.0695865504800329,0.120527440954873));
#59494=DIRECTION('ref_axis',(0.,0.866025403784438,-0.5));
#59495=DIRECTION('',(-0.137998583506848,-0.378681393832731,-0.9151812896443));
#59496=DIRECTION('center_axis',(-0.0617712249622997,0.925513751123792,-0.373642358743525));
#59497=DIRECTION('ref_axis',(0.998052578482889,0.0540211804549215,-0.0311891430775903));
#59498=DIRECTION('',(0.0161503784824051,-0.373381387356163,-0.927537333400043));
#59499=DIRECTION('center_axis',(0.284551435696759,0.891015790469123,-0.353724951873058));
#59500=DIRECTION('ref_axis',(0.957826285221151,-0.248850568624199,0.143673942783173));
#59501=DIRECTION('',(0.0552259184163645,-0.383601057879401,-0.921846151116809));
#59502=DIRECTION('center_axis',(0.491310548314113,0.814189528457783,-0.309369288819978));
#59503=DIRECTION('ref_axis',(0.86824314212446,-0.429668924423658,0.248069469178416));
#59504=DIRECTION('',(0.057078643955053,-0.384529194537799,-0.921346474976903));
#59505=DIRECTION('center_axis',(0.313150259135957,0.883174789320284,-0.34919794774906));
#59506=DIRECTION('ref_axis',(0.948683298050513,-0.273861278752584,0.15811388300842));
#59507=DIRECTION('',(0.0225789275220278,-0.37451109252948,-0.926947481578288));
#59508=DIRECTION('center_axis',(0.,0.927183854566787,-0.374606593415913));
#59509=DIRECTION('ref_axis',(1.,0.,0.));
#59510=DIRECTION('',(-0.0225789275220274,-0.37451109252948,-0.926947481578288));
#59511=DIRECTION('center_axis',(-0.313150259135956,0.883174789320284,-0.34919794774906));
#59512=DIRECTION('ref_axis',(0.948683298050514,0.273861278752584,-0.158113883008419));
#59513=DIRECTION('',(-0.0570786439550527,-0.384529194537799,-0.921346474976903));
#59514=DIRECTION('center_axis',(-0.491310548314114,0.814189528457782,-0.309369288819978));
#59515=DIRECTION('ref_axis',(0.86824314212446,0.429668924423659,-0.248069469178417));
#59516=DIRECTION('',(-0.0552259184163635,-0.3836010578794,-0.921846151116809));
#59517=DIRECTION('center_axis',(-0.284551435696759,0.891015790469123,-0.353724951873058));
#59518=DIRECTION('ref_axis',(0.957826285221151,0.248850568624199,-0.143673942783173));
#59519=DIRECTION('',(-0.0161503784824052,-0.373381387356163,-0.927537333400043));
#59520=DIRECTION('center_axis',(0.0617712249622996,0.925513751123792,-0.373642358743525));
#59521=DIRECTION('ref_axis',(0.998052578482889,-0.0540211804549214,0.0311891430775903));
#59522=DIRECTION('',(0.137998583506848,-0.378681393832731,-0.9151812896443));
#59523=DIRECTION('center_axis',(0.99026806874157,0.0695865504800327,0.120527440954873));
#59524=DIRECTION('ref_axis',(0.,-0.866025403784438,0.5));
#59525=DIRECTION('',(0.137844537491629,-0.371030552991328,-0.918332843924613));
#59526=DIRECTION('center_axis',(0.,0.927183854566787,-0.374606593415913));
#59527=DIRECTION('ref_axis',(1.,0.,0.));
#59528=DIRECTION('',(-0.051925424877728,-0.374101236076903,-0.925933051260727));
#59529=DIRECTION('center_axis',(-0.64930555798837,0.717100917309779,-0.253315153038432));
#59530=DIRECTION('ref_axis',(0.755033118392644,0.567841300538901,-0.327843327723122));
#59531=DIRECTION('center_axis',(0.,-0.788010753606722,0.615661475325659));
#59532=DIRECTION('ref_axis',(-1.,0.,0.));
#59533=DIRECTION('',(-1.,0.,0.));
#59534=DIRECTION('',(0.137844537491629,-0.609784295472662,-0.780488306432985));
#59535=DIRECTION('center_axis',(0.99026806874157,0.0695865504800328,0.120527440954873));
#59536=DIRECTION('ref_axis',(0.,-0.866025403784438,0.5));
#59537=DIRECTION('center_axis',(-0.99026806874157,-0.0695865504800328,-0.120527440954873));
#59538=DIRECTION('ref_axis',(-0.139173100960065,0.495134034370783,0.857597304086756));
#59539=DIRECTION('',(0.137998583506848,-0.603229548983803,-0.785538351821794));
#59540=DIRECTION('center_axis',(0.0617712249622996,-0.786340650163726,0.614697240653271));
#59541=DIRECTION('ref_axis',(-0.998052578482889,-0.0540211804549214,0.0311891430775903));
#59542=DIRECTION('center_axis',(-0.0617712249622996,0.786340650163726,-0.614697240653271));
#59543=DIRECTION('ref_axis',(0.998090334472114,0.0486661612888523,-0.0380432514219071));
#59544=DIRECTION('',(-0.0161503784824054,-0.616580200004833,-0.787126433450736));
#59545=DIRECTION('center_axis',(-0.284551435696759,-0.751842689509057,0.594779833782805));
#59546=DIRECTION('ref_axis',(-0.957826285221151,0.248850568624199,-0.143673942783173));
#59547=DIRECTION('center_axis',(0.284551435696759,0.751842689509057,-0.594779833782805));
#59548=DIRECTION('ref_axis',(-0.958660774436356,0.223163315348643,-0.176543632679542));
#59549=DIRECTION('',(-0.0552259184163638,-0.606541656308366,-0.793131336600549));
#59550=DIRECTION('center_axis',(-0.491310548314114,-0.675016427497717,0.550424170729724));
#59551=DIRECTION('ref_axis',(-0.86824314212446,0.429668924423659,-0.248069469178417));
#59552=DIRECTION('center_axis',(0.491310548314114,0.675016427497717,-0.550424170729724));
#59553=DIRECTION('ref_axis',(-0.870984468928858,0.380767628982861,-0.310486823558562));
#59554=DIRECTION('',(-0.0570786439550532,-0.605644855748342,-0.793685288454953));
#59555=DIRECTION('center_axis',(-0.313150259135956,-0.744001688360219,0.590252829658806));
#59556=DIRECTION('ref_axis',(-0.948683298050514,0.273861278752584,-0.158113883008419));
#59557=DIRECTION('center_axis',(0.313150259135956,0.744001688360219,-0.590252829658806));
#59558=DIRECTION('ref_axis',(-0.949703593340092,0.245323196775732,-0.194626858168784));
#59559=DIRECTION('',(-0.0225789275220273,-0.615504520756066,-0.787809860918737));
#59560=DIRECTION('center_axis',(0.,-0.788010753606722,0.615661475325659));
#59561=DIRECTION('ref_axis',(-1.,0.,0.));
#59562=DIRECTION('',(-1.,0.,0.));
#59563=DIRECTION('',(0.0225789275220281,-0.615504520756066,-0.787809860918737));
#59564=DIRECTION('center_axis',(0.313150259135957,-0.744001688360218,0.590252829658806));
#59565=DIRECTION('ref_axis',(-0.948683298050513,-0.273861278752584,0.15811388300842));
#59566=DIRECTION('center_axis',(-0.313150259135957,0.744001688360218,-0.590252829658806));
#59567=DIRECTION('ref_axis',(0.949703593340092,0.245323196775733,-0.194626858168784));
#59568=DIRECTION('',(0.0570786439550533,-0.605644855748343,-0.793685288454953));
#59569=DIRECTION('center_axis',(0.491310548314113,-0.675016427497717,0.550424170729725));
#59570=DIRECTION('ref_axis',(-0.86824314212446,-0.429668924423658,0.248069469178416));
#59571=DIRECTION('center_axis',(-0.491310548314113,0.675016427497717,-0.550424170729725));
#59572=DIRECTION('ref_axis',(0.870984468928858,0.38076762898286,-0.310486823558562));
#59573=DIRECTION('',(0.0552259184163649,-0.606541656308365,-0.793131336600549));
#59574=DIRECTION('center_axis',(0.284551435696759,-0.751842689509057,0.594779833782805));
#59575=DIRECTION('ref_axis',(-0.957826285221151,-0.248850568624199,0.143673942783173));
#59576=DIRECTION('center_axis',(-0.284551435696759,0.751842689509057,-0.594779833782805));
#59577=DIRECTION('ref_axis',(0.958660774436356,0.223163315348643,-0.176543632679541));
#59578=DIRECTION('',(0.0161503784824051,-0.616580200004833,-0.787126433450736));
#59579=DIRECTION('center_axis',(-0.0617712249622997,-0.786340650163726,
0.614697240653271));
#59580=DIRECTION('ref_axis',(-0.998052578482889,0.0540211804549215,-0.0311891430775903));
#59581=DIRECTION('center_axis',(0.0617712249622997,0.786340650163726,-0.614697240653271));
#59582=DIRECTION('ref_axis',(-0.998090334472114,0.0486661612888524,-0.0380432514219072));
#59583=DIRECTION('',(-0.137998583506848,-0.603229548983803,-0.785538351821794));
#59584=DIRECTION('center_axis',(-0.99026806874157,0.0695865504800329,0.120527440954873));
#59585=DIRECTION('ref_axis',(0.,0.866025403784438,-0.5));
#59586=DIRECTION('center_axis',(0.99026806874157,-0.0695865504800329,-0.120527440954873));
#59587=DIRECTION('ref_axis',(0.139173100960066,0.495134034370784,0.857597304086755));
#59588=DIRECTION('',(-0.137844537491629,-0.609784295472662,-0.780488306432985));
#59589=DIRECTION('center_axis',(0.,-0.788010753606722,0.615661475325659));
#59590=DIRECTION('ref_axis',(-1.,0.,0.));
#59591=DIRECTION('',(-1.,0.,0.));
#59592=DIRECTION('center_axis',(0.,-0.5,-0.866025403784438));
#59593=DIRECTION('ref_axis',(1.,0.,0.));
#59594=DIRECTION('center_axis',(1.,0.,0.));
#59595=DIRECTION('ref_axis',(0.,1.,0.));
#59596=DIRECTION('center_axis',(1.,0.,0.));
#59597=DIRECTION('ref_axis',(0.,0.,-1.));
#59598=DIRECTION('center_axis',(0.649305557988371,-0.662218828358294,0.373989994161849));
#59599=DIRECTION('ref_axis',(0.760527640763576,0.565373752130667,-0.319296457913771));
#59600=DIRECTION('',(1.,0.,0.));
#59601=DIRECTION('center_axis',(-0.99026806874157,-0.0894587448987839,-0.106612780622095));
#59602=DIRECTION('ref_axis',(-0.139173100960065,0.636532044855303,0.758589351257639));
#59603=DIRECTION('center_axis',(-0.0617712249622996,-0.846570802931135,
0.528679668032723));
#59604=DIRECTION('ref_axis',(-0.998090334472114,0.0523937700909925,-0.0327196743412163));
#59605=DIRECTION('center_axis',(0.284551435696759,-0.816055565222214,0.50307434332588));
#59606=DIRECTION('ref_axis',(0.958660774436356,0.242223097976277,-0.149323442110948));
#59607=DIRECTION('center_axis',(0.491310548314114,-0.748098746816874,0.446051802065978));
#59608=DIRECTION('ref_axis',(0.870984468928858,0.42199237598773,-0.25161178329511));
#59609=DIRECTION('center_axis',(0.313150259135956,-0.809119792515883,0.497254539006069));
#59610=DIRECTION('ref_axis',(0.949703593340092,0.266794897350299,-0.163962091791853));
#59611=DIRECTION('',(1.,0.,0.));
#59612=DIRECTION('center_axis',(-0.313150259135957,-0.809119792515883,0.497254539006068));
#59613=DIRECTION('ref_axis',(-0.949703593340092,0.2667948973503,-0.163962091791853));
#59614=DIRECTION('center_axis',(-0.491310548314113,-0.748098746816875,0.446051802065979));
#59615=DIRECTION('ref_axis',(-0.870984468928858,0.421992375987729,-0.25161178329511));
#59616=DIRECTION('center_axis',(-0.284551435696759,-0.816055565222214,0.503074343325881));
#59617=DIRECTION('ref_axis',(-0.958660774436356,0.242223097976277,-0.149323442110948));
#59618=DIRECTION('center_axis',(0.0617712249622997,-0.846570802931135,0.528679668032723));
#59619=DIRECTION('ref_axis',(0.998090334472114,0.0523937700909926,-0.0327196743412163));
#59620=DIRECTION('center_axis',(0.99026806874157,-0.0894587448987841,-0.106612780622095));
#59621=DIRECTION('ref_axis',(0.139173100960066,0.636532044855299,0.758589351257642));
#59622=DIRECTION('',(1.,0.,0.));
#59623=DIRECTION('center_axis',(0.,0.848048096156426,-0.529919264233205));
#59624=DIRECTION('ref_axis',(1.,0.,0.));
#59625=DIRECTION('',(-0.137844537491629,-0.524860590029465,-0.839952525157012));
#59626=DIRECTION('center_axis',(-0.99026806874157,0.0894587448987841,0.106612780622095));
#59627=DIRECTION('ref_axis',(0.,0.766044443118978,-0.642787609686539));
#59628=DIRECTION('',(-0.137998583506848,-0.531847935749547,-0.835520295497991));
#59629=DIRECTION('center_axis',(-0.0617712249622997,0.846570802931135,-0.528679668032723));
#59630=DIRECTION('ref_axis',(0.998052578482889,0.0477845394804615,-0.0400959894540315));
#59631=DIRECTION('',(0.0161503784824051,-0.528774052761765,-0.848608959651484));
#59632=DIRECTION('center_axis',(0.284551435696759,0.816055565222214,-0.503074343325881));
#59633=DIRECTION('ref_axis',(0.957826285221151,-0.220121250980087,0.184703660511672));
#59634=DIRECTION('',(0.0552259184163645,-0.537850200094026,-0.841229612052432));
#59635=DIRECTION('center_axis',(0.491310548314113,0.748098746816875,-0.446051802065979));
#59636=DIRECTION('ref_axis',(0.86824314212446,-0.3800644767432,0.318911962258805));
#59637=DIRECTION('',(0.057078643955053,-0.538677468419953,-0.840576357876501));
#59638=DIRECTION('center_axis',(0.313150259135957,0.809119792515883,-0.497254539006068));
#59639=DIRECTION('ref_axis',(0.948683298050513,-0.242244522917128,0.203267289834479));
#59640=DIRECTION('',(0.0225789275220278,-0.529784168481124,-0.847831897759644));
#59641=DIRECTION('center_axis',(0.,0.848048096156426,-0.529919264233205));
#59642=DIRECTION('ref_axis',(1.,0.,0.));
#59643=DIRECTION('',(-0.0225789275220274,-0.529784168481124,-0.847831897759644));
#59644=DIRECTION('center_axis',(-0.313150259135956,0.809119792515883,-0.497254539006069));
#59645=DIRECTION('ref_axis',(0.948683298050514,0.242244522917128,-0.203267289834478));
#59646=DIRECTION('',(-0.0570786439550527,-0.538677468419953,-0.840576357876501));
#59647=DIRECTION('center_axis',(-0.491310548314114,0.748098746816874,-0.446051802065978));
#59648=DIRECTION('ref_axis',(0.86824314212446,0.380064476743201,-0.318911962258806));
#59649=DIRECTION('',(-0.0552259184163635,-0.537850200094025,-0.841229612052432));
#59650=DIRECTION('center_axis',(-0.284551435696759,0.816055565222214,-0.50307434332588));
#59651=DIRECTION('ref_axis',(0.957826285221151,0.220121250980087,-0.184703660511673));
#59652=DIRECTION('',(-0.0161503784824052,-0.528774052761765,-0.848608959651484));
#59653=DIRECTION('center_axis',(0.0617712249622996,0.846570802931135,-0.528679668032723));
#59654=DIRECTION('ref_axis',(0.998052578482889,-0.0477845394804615,0.0400959894540314));
#59655=DIRECTION('',(0.137998583506848,-0.531847935749547,-0.835520295497991));
#59656=DIRECTION('center_axis',(0.99026806874157,0.0894587448987839,0.106612780622095));
#59657=DIRECTION('ref_axis',(0.,-0.766044443118978,0.642787609686539));
#59658=DIRECTION('',(0.137844537491629,-0.524860590029465,-0.839952525157012));
#59659=DIRECTION('center_axis',(0.,0.848048096156426,-0.529919264233205));
#59660=DIRECTION('ref_axis',(1.,0.,0.));
#59661=DIRECTION('',(-0.051925424877728,-0.52920438469299,-0.846904049744114));
#59662=DIRECTION('center_axis',(-0.649305557988371,0.662218828358294,-0.373989994161849));
#59663=DIRECTION('ref_axis',(0.755033118392644,0.502285118831862,-0.421467257957652));
#59664=DIRECTION('center_axis',(0.,-0.669130606358858,0.743144825477394));
#59665=DIRECTION('ref_axis',(-1.,0.,0.));
#59666=DIRECTION('',(-1.,0.,0.));
#59667=DIRECTION('',(0.137844537491629,-0.736050673949001,-0.662743003631831));
#59668=DIRECTION('center_axis',(0.99026806874157,0.0894587448987839,0.106612780622095));
#59669=DIRECTION('ref_axis',(0.,-0.766044443118978,0.642787609686539));
#59670=DIRECTION('center_axis',(-0.99026806874157,-0.0894587448987839,-0.106612780622095));
#59671=DIRECTION('ref_axis',(-0.139173100960065,0.636532044855303,0.758589351257639));
#59672=DIRECTION('',(0.137998583506848,-0.730472439966645,-0.668854547266653));
#59673=DIRECTION('center_axis',(0.0617712249622996,-0.667653313133567,0.741905229276912));
#59674=DIRECTION('ref_axis',(-0.998052578482889,-0.0477845394804615,0.0400959894540314));
#59675=DIRECTION('center_axis',(-0.0617712249622996,0.667653313133567,-0.741905229276912));
#59676=DIRECTION('ref_axis',(0.998090334472114,0.0413206716646654,-0.045916079171941));
#59677=DIRECTION('',(-0.0161503784824054,-0.743896032080768,-0.668100186146782));
#59678=DIRECTION('center_axis',(-0.284551435696759,-0.637138075424646,0.71629990457007));
#59679=DIRECTION('ref_axis',(-0.957826285221151,0.220121250980087,-0.184703660511673));
#59680=DIRECTION('center_axis',(0.284551435696759,0.637138075424646,-0.71629990457007));
#59681=DIRECTION('ref_axis',(-0.958660774436356,0.18911648304975,-0.212613441240154));
#59682=DIRECTION('',(-0.0552259184163638,-0.735052736908566,-0.675757036144127));
#59683=DIRECTION('center_axis',(-0.491310548314114,-0.569181257019306,0.659277363310168));
#59684=DIRECTION('ref_axis',(-0.86824314212446,0.380064476743201,-0.318911962258806));
#59685=DIRECTION('center_axis',(0.491310548314114,0.569181257019306,-0.659277363310168));
#59686=DIRECTION('ref_axis',(-0.870984468928858,0.32106744201786,-0.371889435936037));
#59687=DIRECTION('',(-0.0570786439550532,-0.734265753494182,-0.676458300008118));
#59688=DIRECTION('center_axis',(-0.313150259135956,-0.630202302718315,0.710480100250258));
#59689=DIRECTION('ref_axis',(-0.948683298050514,0.242244522917128,-0.203267289834478));
#59690=DIRECTION('center_axis',(0.313150259135956,0.630202302718315,-0.710480100250258));
#59691=DIRECTION('ref_axis',(-0.949703593340092,0.207799586932431,-0.234269964928557));
#59692=DIRECTION('',(-0.0225789275220273,-0.742955370751214,-0.668960020557194));
#59693=DIRECTION('center_axis',(0.,-0.669130606358858,0.743144825477394));
#59694=DIRECTION('ref_axis',(-1.,0.,0.));
#59695=DIRECTION('',(-1.,0.,0.));
#59696=DIRECTION('',(0.0225789275220281,-0.742955370751214,-0.668960020557194));
#59697=DIRECTION('center_axis',(0.313150259135957,-0.630202302718315,0.710480100250258));
#59698=DIRECTION('ref_axis',(-0.948683298050513,-0.242244522917128,0.203267289834479));
#59699=DIRECTION('center_axis',(-0.313150259135957,0.630202302718315,-0.710480100250258));
#59700=DIRECTION('ref_axis',(0.949703593340092,0.207799586932432,-0.234269964928558));
#59701=DIRECTION('',(0.0570786439550534,-0.734265753494183,-0.676458300008118));
#59702=DIRECTION('center_axis',(0.491310548314113,-0.569181257019307,0.659277363310168));
#59703=DIRECTION('ref_axis',(-0.86824314212446,-0.3800644767432,0.318911962258805));
#59704=DIRECTION('center_axis',(-0.491310548314113,0.569181257019307,-0.659277363310168));
#59705=DIRECTION('ref_axis',(0.870984468928858,0.321067442017859,-0.371889435936036));
#59706=DIRECTION('',(0.0552259184163649,-0.735052736908566,-0.675757036144127));
#59707=DIRECTION('center_axis',(0.284551435696759,-0.637138075424647,0.71629990457007));
#59708=DIRECTION('ref_axis',(-0.957826285221151,-0.220121250980087,0.184703660511672));
#59709=DIRECTION('center_axis',(-0.284551435696759,0.637138075424647,-0.71629990457007));
#59710=DIRECTION('ref_axis',(0.958660774436356,0.189116483049749,-0.212613441240154));
#59711=DIRECTION('',(0.0161503784824051,-0.743896032080768,-0.668100186146782));
#59712=DIRECTION('center_axis',(-0.0617712249622997,-0.667653313133567,
0.741905229276912));
#59713=DIRECTION('ref_axis',(-0.998052578482889,0.0477845394804615,-0.0400959894540315));
#59714=DIRECTION('center_axis',(0.0617712249622997,0.667653313133567,-0.741905229276912));
#59715=DIRECTION('ref_axis',(-0.998090334472114,0.0413206716646654,-0.045916079171941));
#59716=DIRECTION('',(-0.137998583506848,-0.730472439966645,-0.668854547266653));
#59717=DIRECTION('center_axis',(-0.99026806874157,0.0894587448987841,0.106612780622095));
#59718=DIRECTION('ref_axis',(0.,0.766044443118978,-0.642787609686539));
#59719=DIRECTION('center_axis',(0.99026806874157,-0.0894587448987841,-0.106612780622095));
#59720=DIRECTION('ref_axis',(0.139173100960066,0.636532044855299,0.758589351257642));
#59721=DIRECTION('',(-0.137844537491629,-0.736050673949,-0.662743003631831));
#59722=DIRECTION('center_axis',(0.,-0.669130606358858,0.743144825477394));
#59723=DIRECTION('ref_axis',(-1.,0.,0.));
#59724=DIRECTION('',(-1.,0.,0.));
#59725=DIRECTION('center_axis',(0.,-0.642787609686539,-0.766044443118978));
#59726=DIRECTION('ref_axis',(1.,0.,0.));
#59727=DIRECTION('center_axis',(1.,0.,0.));
#59728=DIRECTION('ref_axis',(0.,1.,0.));
#59729=DIRECTION('center_axis',(1.,0.,0.));
#59730=DIRECTION('ref_axis',(0.,0.,-1.));
#59731=DIRECTION('center_axis',(0.64930555798837,-0.587215555406038,0.483301338560726));
#59732=DIRECTION('ref_axis',(0.760527640763576,0.501339206395651,-0.412621749021023));
#59733=DIRECTION('',(1.,0.,0.));
#59734=DIRECTION('center_axis',(-0.99026806874157,-0.106612780622095,-0.0894587448987838));
#59735=DIRECTION('ref_axis',(-0.139173100960065,0.758589351257642,0.636532044855299));
#59736=DIRECTION('center_axis',(-0.0617712249622996,-0.741905229276912,
0.667653313133568));
#59737=DIRECTION('ref_axis',(-0.998090334472114,0.045916079171941,-0.0413206716646654));
#59738=DIRECTION('center_axis',(0.284551435696759,-0.71629990457007,0.637138075424647));
#59739=DIRECTION('ref_axis',(0.958660774436356,0.212613441240154,-0.18911648304975));
#59740=DIRECTION('center_axis',(0.491310548314114,-0.659277363310167,0.569181257019307));
#59741=DIRECTION('ref_axis',(0.870984468928858,0.371889435936037,-0.32106744201786));
#59742=DIRECTION('center_axis',(0.313150259135956,-0.710480100250258,0.630202302718316));
#59743=DIRECTION('ref_axis',(0.949703593340092,0.234269964928557,-0.207799586932431));
#59744=DIRECTION('',(1.,0.,0.));
#59745=DIRECTION('center_axis',(-0.313150259135957,-0.710480100250258,0.630202302718315));
#59746=DIRECTION('ref_axis',(-0.949703593340092,0.234269964928558,-0.207799586932432));
#59747=DIRECTION('center_axis',(-0.491310548314113,-0.659277363310168,0.569181257019307));
#59748=DIRECTION('ref_axis',(-0.870984468928858,0.371889435936036,-0.321067442017859));
#59749=DIRECTION('center_axis',(-0.284551435696759,-0.71629990457007,0.637138075424647));
#59750=DIRECTION('ref_axis',(-0.958660774436356,0.212613441240154,-0.189116483049749));
#59751=DIRECTION('center_axis',(0.0617712249622997,-0.741905229276912,0.667653313133568));
#59752=DIRECTION('ref_axis',(0.998090334472114,0.045916079171941,-0.0413206716646654));
#59753=DIRECTION('center_axis',(0.99026806874157,-0.106612780622095,-0.0894587448987841));
#59754=DIRECTION('ref_axis',(0.139173100960066,0.758589351257642,0.636532044855299));
#59755=DIRECTION('',(1.,0.,0.));
#59756=DIRECTION('center_axis',(0.,0.743144825477394,-0.669130606358858));
#59757=DIRECTION('ref_axis',(1.,0.,0.));
#59758=DIRECTION('',(-0.137844537491629,-0.662743003631831,-0.736050673949001));
#59759=DIRECTION('center_axis',(-0.99026806874157,0.106612780622095,0.0894587448987841));
#59760=DIRECTION('ref_axis',(0.,0.642787609686539,-0.766044443118978));
#59761=DIRECTION('',(-0.137998583506848,-0.668854547266653,-0.730472439966645));
#59762=DIRECTION('center_axis',(-0.0617712249622997,0.741905229276912,-0.667653313133568));
#59763=DIRECTION('ref_axis',(0.998052578482889,0.0400959894540315,-0.0477845394804616));
#59764=DIRECTION('',(0.0161503784824051,-0.668100186146782,-0.743896032080767));
#59765=DIRECTION('center_axis',(0.284551435696759,0.71629990457007,-0.637138075424647));
#59766=DIRECTION('ref_axis',(0.957826285221151,-0.184703660511672,0.220121250980087));
#59767=DIRECTION('',(0.0552259184163645,-0.675757036144128,-0.735052736908566));
#59768=DIRECTION('center_axis',(0.491310548314113,0.659277363310168,-0.569181257019307));
#59769=DIRECTION('ref_axis',(0.86824314212446,-0.318911962258805,0.3800644767432));
#59770=DIRECTION('',(0.057078643955053,-0.676458300008118,-0.734265753494182));
#59771=DIRECTION('center_axis',(0.313150259135957,0.710480100250258,-0.630202302718315));
#59772=DIRECTION('ref_axis',(0.948683298050513,-0.203267289834479,0.242244522917128));
#59773=DIRECTION('',(0.0225789275220278,-0.668960020557194,-0.742955370751214));
#59774=DIRECTION('center_axis',(0.,0.743144825477394,-0.669130606358858));
#59775=DIRECTION('ref_axis',(1.,0.,0.));
#59776=DIRECTION('',(-0.0225789275220274,-0.668960020557194,-0.742955370751214));
#59777=DIRECTION('center_axis',(-0.313150259135956,0.710480100250258,-0.630202302718316));
#59778=DIRECTION('ref_axis',(0.948683298050514,0.203267289834478,-0.242244522917128));
#59779=DIRECTION('',(-0.0570786439550527,-0.676458300008118,-0.734265753494182));
#59780=DIRECTION('center_axis',(-0.491310548314114,0.659277363310167,-0.569181257019307));
#59781=DIRECTION('ref_axis',(0.868243142124459,0.318911962258806,-0.380064476743201));
#59782=DIRECTION('',(-0.0552259184163635,-0.675757036144127,-0.735052736908566));
#59783=DIRECTION('center_axis',(-0.284551435696759,0.71629990457007,-0.637138075424647));
#59784=DIRECTION('ref_axis',(0.957826285221151,0.184703660511673,-0.220121250980087));
#59785=DIRECTION('',(-0.0161503784824052,-0.668100186146782,-0.743896032080767));
#59786=DIRECTION('center_axis',(0.0617712249622996,0.741905229276912,-0.667653313133568));
#59787=DIRECTION('ref_axis',(0.998052578482889,-0.0400959894540314,0.0477845394804615));
#59788=DIRECTION('',(0.137998583506848,-0.668854547266653,-0.730472439966645));
#59789=DIRECTION('center_axis',(0.99026806874157,0.106612780622095,0.0894587448987838));
#59790=DIRECTION('ref_axis',(0.,-0.642787609686539,0.766044443118978));
#59791=DIRECTION('',(0.137844537491629,-0.662743003631831,-0.736050673949001));
#59792=DIRECTION('center_axis',(0.,0.743144825477394,-0.669130606358858));
#59793=DIRECTION('ref_axis',(1.,0.,0.));
#59794=DIRECTION('',(-0.0519254248777279,-0.66822792587052,-0.742142297230154));
#59795=DIRECTION('center_axis',(-0.64930555798837,0.587215555406038,-0.483301338560726));
#59796=DIRECTION('ref_axis',(0.755033118392644,0.421467257957652,-0.502285118831862));
#59797=DIRECTION('center_axis',(0.,-0.529919264233205,0.848048096156426));
#59798=DIRECTION('ref_axis',(-1.,0.,0.));
#59799=DIRECTION('',(-1.,0.,0.));
#59800=DIRECTION('',(0.137844537491629,-0.839952525157012,-0.524860590029465));
#59801=DIRECTION('center_axis',(0.99026806874157,0.106612780622095,0.0894587448987839));
#59802=DIRECTION('ref_axis',(0.,-0.642787609686539,0.766044443118978));
#59803=DIRECTION('center_axis',(-0.99026806874157,-0.106612780622095,-0.0894587448987839));
#59804=DIRECTION('ref_axis',(-0.139173100960065,0.758589351257639,0.636532044855303));
#59805=DIRECTION('',(0.137998583506848,-0.835520295497991,-0.531847935749546));
#59806=DIRECTION('center_axis',(0.0617712249622996,-0.528679668032723,0.846570802931135));
#59807=DIRECTION('ref_axis',(-0.998052578482889,-0.0400959894540314,0.0477845394804615));
#59808=DIRECTION('center_axis',(-0.0617712249622996,0.528679668032723,-0.846570802931135));
#59809=DIRECTION('ref_axis',(0.998090334472114,0.0327196743412163,-0.0523937700909925));
#59810=DIRECTION('',(-0.0161503784824054,-0.848608959651484,-0.528774052761765));
#59811=DIRECTION('center_axis',(-0.284551435696759,-0.50307434332588,0.816055565222214));
#59812=DIRECTION('ref_axis',(-0.957826285221151,0.184703660511673,-0.220121250980087));
#59813=DIRECTION('center_axis',(0.284551435696759,0.50307434332588,-0.816055565222214));
#59814=DIRECTION('ref_axis',(-0.958660774436356,0.149323442110948,-0.242223097976277));
#59815=DIRECTION('',(-0.0552259184163638,-0.841229612052433,-0.537850200094025));
#59816=DIRECTION('center_axis',(-0.491310548314114,-0.446051802065978,0.748098746816874));
#59817=DIRECTION('ref_axis',(-0.868243142124459,0.318911962258806,-0.380064476743201));
#59818=DIRECTION('center_axis',(0.491310548314114,0.446051802065978,-0.748098746816874));
#59819=DIRECTION('ref_axis',(-0.870984468928858,0.25161178329511,-0.421992375987731));
#59820=DIRECTION('',(-0.0570786439550532,-0.840576357876501,-0.538677468419953));
#59821=DIRECTION('center_axis',(-0.313150259135956,-0.497254539006068,0.809119792515883));
#59822=DIRECTION('ref_axis',(-0.948683298050514,0.203267289834478,-0.242244522917128));
#59823=DIRECTION('center_axis',(0.313150259135956,0.497254539006068,-0.809119792515883));
#59824=DIRECTION('ref_axis',(-0.949703593340092,0.163962091791853,-0.266794897350299));
#59825=DIRECTION('',(-0.0225789275220273,-0.847831897759644,-0.529784168481124));
#59826=DIRECTION('center_axis',(0.,-0.529919264233205,0.848048096156426));
#59827=DIRECTION('ref_axis',(-1.,0.,0.));
#59828=DIRECTION('',(-1.,0.,0.));
#59829=DIRECTION('',(0.0225789275220281,-0.847831897759644,-0.529784168481124));
#59830=DIRECTION('center_axis',(0.313150259135957,-0.497254539006068,0.809119792515883));
#59831=DIRECTION('ref_axis',(-0.948683298050513,-0.203267289834479,0.242244522917128));
#59832=DIRECTION('center_axis',(-0.313150259135957,0.497254539006068,-0.809119792515883));
#59833=DIRECTION('ref_axis',(0.949703593340092,0.163962091791853,-0.2667948973503));
#59834=DIRECTION('',(0.0570786439550534,-0.840576357876501,-0.538677468419953));
#59835=DIRECTION('center_axis',(0.491310548314113,-0.446051802065978,0.748098746816875));
#59836=DIRECTION('ref_axis',(-0.86824314212446,-0.318911962258805,0.3800644767432));
#59837=DIRECTION('center_axis',(-0.491310548314113,0.446051802065978,-0.748098746816875));
#59838=DIRECTION('ref_axis',(0.870984468928858,0.25161178329511,-0.421992375987729));
#59839=DIRECTION('',(0.0552259184163649,-0.841229612052432,-0.537850200094026));
#59840=DIRECTION('center_axis',(0.284551435696759,-0.50307434332588,0.816055565222214));
#59841=DIRECTION('ref_axis',(-0.957826285221151,-0.184703660511672,0.220121250980087));
#59842=DIRECTION('center_axis',(-0.284551435696759,0.50307434332588,-0.816055565222214));
#59843=DIRECTION('ref_axis',(0.958660774436356,0.149323442110947,-0.242223097976277));
#59844=DIRECTION('',(0.0161503784824051,-0.848608959651484,-0.528774052761765));
#59845=DIRECTION('center_axis',(-0.0617712249622997,-0.528679668032723,
0.846570802931135));
#59846=DIRECTION('ref_axis',(-0.998052578482889,0.0400959894540315,-0.0477845394804616));
#59847=DIRECTION('center_axis',(0.0617712249622997,0.528679668032723,-0.846570802931135));
#59848=DIRECTION('ref_axis',(-0.998090334472114,0.0327196743412163,-0.0523937700909926));
#59849=DIRECTION('',(-0.137998583506848,-0.835520295497991,-0.531847935749546));
#59850=DIRECTION('center_axis',(-0.99026806874157,0.106612780622095,0.0894587448987841));
#59851=DIRECTION('ref_axis',(0.,0.642787609686539,-0.766044443118978));
#59852=DIRECTION('center_axis',(0.99026806874157,-0.106612780622095,-0.0894587448987841));
#59853=DIRECTION('ref_axis',(0.139173100960066,0.758589351257642,0.636532044855299));
#59854=DIRECTION('',(-0.137844537491629,-0.839952525157012,-0.524860590029465));
#59855=DIRECTION('center_axis',(0.,-0.529919264233205,0.848048096156426));
#59856=DIRECTION('ref_axis',(-1.,0.,0.));
#59857=DIRECTION('',(-1.,0.,0.));
#59858=DIRECTION('center_axis',(0.,-0.766044443118978,-0.642787609686539));
#59859=DIRECTION('ref_axis',(1.,0.,0.));
#59860=DIRECTION('center_axis',(1.,0.,0.));
#59861=DIRECTION('ref_axis',(0.,1.,0.));
#59862=DIRECTION('center_axis',(1.,0.,0.));
#59863=DIRECTION('ref_axis',(0.,0.,-1.));
#59864=DIRECTION('center_axis',(0.649305557988371,-0.494370034948177,0.577927816349714));
#59865=DIRECTION('ref_axis',(0.760527640763576,0.422071722564183,-0.49340973708095));
#59866=DIRECTION('',(1.,0.,0.));
#59867=DIRECTION('center_axis',(-0.99026806874157,-0.120527440954873,-0.0695865504800326));
#59868=DIRECTION('ref_axis',(-0.139173100960065,0.857597304086756,0.495134034370783));
#59869=DIRECTION('center_axis',(-0.0617712249622996,-0.61469724065327,0.786340650163727));
#59870=DIRECTION('ref_axis',(-0.998090334472114,0.0380432514219071,-0.0486661612888524));
#59871=DIRECTION('center_axis',(0.284551435696759,-0.594779833782804,0.751842689509058));
#59872=DIRECTION('ref_axis',(0.958660774436356,0.176543632679541,-0.223163315348643));
#59873=DIRECTION('center_axis',(0.491310548314114,-0.550424170729724,0.675016427497717));
#59874=DIRECTION('ref_axis',(0.870984468928858,0.310486823558562,-0.380767628982861));
#59875=DIRECTION('center_axis',(0.313150259135956,-0.590252829658806,0.744001688360219));
#59876=DIRECTION('ref_axis',(0.949703593340092,0.194626858168784,-0.245323196775732));
#59877=DIRECTION('',(1.,0.,0.));
#59878=DIRECTION('center_axis',(-0.313150259135957,-0.590252829658806,0.744001688360219));
#59879=DIRECTION('ref_axis',(-0.949703593340092,0.194626858168784,-0.245323196775733));
#59880=DIRECTION('center_axis',(-0.491310548314113,-0.550424170729724,0.675016427497718));
#59881=DIRECTION('ref_axis',(-0.870984468928858,0.310486823558561,-0.38076762898286));
#59882=DIRECTION('center_axis',(-0.284551435696759,-0.594779833782804,0.751842689509058));
#59883=DIRECTION('ref_axis',(-0.958660774436356,0.176543632679541,-0.223163315348643));
#59884=DIRECTION('center_axis',(0.0617712249622997,-0.61469724065327,0.786340650163727));
#59885=DIRECTION('ref_axis',(0.998090334472114,0.0380432514219071,-0.0486661612888524));
#59886=DIRECTION('center_axis',(0.99026806874157,-0.120527440954873,-0.0695865504800328));
#59887=DIRECTION('ref_axis',(0.139173100960066,0.857597304086755,0.495134034370784));
#59888=DIRECTION('',(1.,0.,0.));
#59889=DIRECTION('center_axis',(0.,0.615661475325658,-0.788010753606722));
#59890=DIRECTION('ref_axis',(1.,0.,0.));
#59891=DIRECTION('',(-0.137844537491629,-0.780488306432985,-0.609784295472661));
#59892=DIRECTION('center_axis',(-0.99026806874157,0.120527440954873,0.0695865504800328));
#59893=DIRECTION('ref_axis',(0.,0.5,-0.866025403784439));
#59894=DIRECTION('',(-0.137998583506848,-0.785538351821795,-0.603229548983802));
#59895=DIRECTION('center_axis',(-0.0617712249622997,0.61469724065327,-0.786340650163727));
#59896=DIRECTION('ref_axis',(0.998052578482889,0.0311891430775903,-0.0540211804549215));
#59897=DIRECTION('',(0.0161503784824051,-0.787126433450736,-0.616580200004832));
#59898=DIRECTION('center_axis',(0.284551435696759,0.594779833782804,-0.751842689509058));
#59899=DIRECTION('ref_axis',(0.957826285221151,-0.143673942783173,0.248850568624199));
#59900=DIRECTION('',(0.0552259184163645,-0.79313133660055,-0.606541656308365));
#59901=DIRECTION('center_axis',(0.491310548314113,0.550424170729724,-0.675016427497718));
#59902=DIRECTION('ref_axis',(0.86824314212446,-0.248069469178416,0.429668924423658));
#59903=DIRECTION('',(0.057078643955053,-0.793685288454953,-0.605644855748342));
#59904=DIRECTION('center_axis',(0.313150259135957,0.590252829658806,-0.744001688360219));
#59905=DIRECTION('ref_axis',(0.948683298050513,-0.15811388300842,0.273861278752585));
#59906=DIRECTION('',(0.0225789275220278,-0.787809860918738,-0.615504520756066));
#59907=DIRECTION('center_axis',(0.,0.615661475325658,-0.788010753606722));
#59908=DIRECTION('ref_axis',(1.,0.,0.));
#59909=DIRECTION('',(-0.0225789275220274,-0.787809860918738,-0.615504520756066));
#59910=DIRECTION('center_axis',(-0.313150259135956,0.590252829658806,-0.744001688360219));
#59911=DIRECTION('ref_axis',(0.948683298050513,0.158113883008419,-0.273861278752584));
#59912=DIRECTION('',(-0.0570786439550527,-0.793685288454953,-0.605644855748342));
#59913=DIRECTION('center_axis',(-0.491310548314114,0.550424170729724,-0.675016427497717));
#59914=DIRECTION('ref_axis',(0.868243142124459,0.248069469178416,-0.429668924423659));
#59915=DIRECTION('',(-0.0552259184163635,-0.79313133660055,-0.606541656308365));
#59916=DIRECTION('center_axis',(-0.284551435696759,0.594779833782804,-0.751842689509058));
#59917=DIRECTION('ref_axis',(0.957826285221151,0.143673942783173,-0.248850568624199));
#59918=DIRECTION('',(-0.0161503784824052,-0.787126433450736,-0.616580200004832));
#59919=DIRECTION('center_axis',(0.0617712249622996,0.61469724065327,-0.786340650163727));
#59920=DIRECTION('ref_axis',(0.998052578482889,-0.0311891430775902,0.0540211804549215));
#59921=DIRECTION('',(0.137998583506848,-0.785538351821795,-0.603229548983802));
#59922=DIRECTION('center_axis',(0.99026806874157,0.120527440954873,0.0695865504800326));
#59923=DIRECTION('ref_axis',(0.,-0.5,0.866025403784439));
#59924=DIRECTION('',(0.137844537491629,-0.780488306432985,-0.609784295472661));
#59925=DIRECTION('center_axis',(0.,0.615661475325658,-0.788010753606722));
#59926=DIRECTION('ref_axis',(1.,0.,0.));
#59927=DIRECTION('',(-0.0519254248777279,-0.786947699660121,-0.614830926556977));
#59928=DIRECTION('center_axis',(-0.649305557988371,0.494370034948177,-0.577927816349714));
#59929=DIRECTION('ref_axis',(0.755033118392644,0.327843327723121,-0.567841300538901));
#59930=DIRECTION('center_axis',(0.,-0.374606593415912,0.927183854566788));
#59931=DIRECTION('ref_axis',(-1.,0.,0.));
#59932=DIRECTION('',(-1.,0.,0.));
#59933=DIRECTION('',(0.137844537491629,-0.918332843924614,-0.371030552991327));
#59934=DIRECTION('center_axis',(0.99026806874157,0.120527440954873,0.0695865504800327));
#59935=DIRECTION('ref_axis',(0.,-0.5,0.866025403784439));
#59936=DIRECTION('center_axis',(-0.99026806874157,-0.120527440954873,-0.0695865504800327));
#59937=DIRECTION('ref_axis',(-0.139173100960065,0.857597304086756,0.495134034370783));
#59938=DIRECTION('',(0.137998583506848,-0.9151812896443,-0.378681393832731));
#59939=DIRECTION('center_axis',(0.0617712249622996,-0.373642358743524,0.925513751123792));
#59940=DIRECTION('ref_axis',(-0.998052578482889,-0.0311891430775902,0.0540211804549215));
#59941=DIRECTION('center_axis',(-0.0617712249622996,0.373642358743524,-0.925513751123792));
#59942=DIRECTION('ref_axis',(0.998090334472114,0.0231245062698634,-0.0572795028183562));
#59943=DIRECTION('',(-0.0161503784824054,-0.927537333400043,-0.373381387356162));
#59944=DIRECTION('center_axis',(-0.284551435696759,-0.353724951873057,0.891015790469123));
#59945=DIRECTION('ref_axis',(-0.957826285221151,0.143673942783173,-0.248850568624199));
#59946=DIRECTION('center_axis',(0.284551435696759,0.353724951873057,-0.891015790469123));
#59947=DIRECTION('ref_axis',(-0.958660774436356,0.104993283944912,-0.264472928451193));
#59948=DIRECTION('',(-0.0552259184163638,-0.921846151116809,-0.383601057879399));
#59949=DIRECTION('center_axis',(-0.491310548314114,-0.309369288819977,0.814189528457782));
#59950=DIRECTION('ref_axis',(-0.868243142124459,0.248069469178416,-0.429668924423659));
#59951=DIRECTION('center_axis',(0.491310548314114,0.309369288819977,-0.814189528457782));
#59952=DIRECTION('ref_axis',(-0.870984468928858,0.174511027858645,-0.459273291233482));
#59953=DIRECTION('',(-0.0570786439550532,-0.921346474976903,-0.384529194537798));
#59954=DIRECTION('center_axis',(-0.313150259135956,-0.349197947749059,0.883174789320284));
#59955=DIRECTION('ref_axis',(-0.948683298050513,0.158113883008419,-0.273861278752584));
#59956=DIRECTION('center_axis',(0.313150259135956,0.349197947749059,-0.883174789320284));
#59957=DIRECTION('ref_axis',(-0.949703593340092,0.115142691461001,-0.291213401820784));
#59958=DIRECTION('',(-0.0225789275220273,-0.926947481578288,-0.374511092529479));
#59959=DIRECTION('center_axis',(0.,-0.374606593415912,0.927183854566788));
#59960=DIRECTION('ref_axis',(-1.,0.,0.));
#59961=DIRECTION('',(-1.,0.,0.));
#59962=DIRECTION('',(0.0225789275220281,-0.926947481578288,-0.374511092529479));
#59963=DIRECTION('center_axis',(0.313150259135957,-0.349197947749059,0.883174789320284));
#59964=DIRECTION('ref_axis',(-0.948683298050513,-0.15811388300842,0.273861278752585));
#59965=DIRECTION('center_axis',(-0.313150259135957,0.349197947749059,-0.883174789320284));
#59966=DIRECTION('ref_axis',(0.949703593340092,0.115142691461001,-0.291213401820785));
#59967=DIRECTION('',(0.0570786439550533,-0.921346474976903,-0.384529194537798));
#59968=DIRECTION('center_axis',(0.491310548314113,-0.309369288819977,0.814189528457783));
#59969=DIRECTION('ref_axis',(-0.86824314212446,-0.248069469178416,0.429668924423658));
#59970=DIRECTION('center_axis',(-0.491310548314113,0.309369288819977,-0.814189528457783));
#59971=DIRECTION('ref_axis',(0.870984468928858,0.174511027858644,-0.459273291233481));
#59972=DIRECTION('',(0.0552259184163649,-0.921846151116809,-0.3836010578794));
#59973=DIRECTION('center_axis',(0.284551435696759,-0.353724951873058,0.891015790469123));
#59974=DIRECTION('ref_axis',(-0.957826285221151,-0.143673942783173,0.248850568624199));
#59975=DIRECTION('center_axis',(-0.284551435696759,0.353724951873058,-0.891015790469123));
#59976=DIRECTION('ref_axis',(0.958660774436356,0.104993283944912,-0.264472928451193));
#59977=DIRECTION('',(0.016150378482405,-0.927537333400043,-0.373381387356162));
#59978=DIRECTION('center_axis',(-0.0617712249622997,-0.373642358743524,
0.925513751123792));
#59979=DIRECTION('ref_axis',(-0.998052578482889,0.0311891430775903,-0.0540211804549215));
#59980=DIRECTION('center_axis',(0.0617712249622997,0.373642358743524,-0.925513751123792));
#59981=DIRECTION('ref_axis',(-0.998090334472114,0.0231245062698634,-0.0572795028183563));
#59982=DIRECTION('',(-0.137998583506848,-0.9151812896443,-0.378681393832731));
#59983=DIRECTION('center_axis',(-0.99026806874157,0.120527440954873,0.0695865504800328));
#59984=DIRECTION('ref_axis',(0.,0.5,-0.866025403784439));
#59985=DIRECTION('center_axis',(0.99026806874157,-0.120527440954873,-0.0695865504800328));
#59986=DIRECTION('ref_axis',(0.139173100960066,0.857597304086755,0.495134034370784));
#59987=DIRECTION('',(-0.137844537491629,-0.918332843924614,-0.371030552991327));
#59988=DIRECTION('center_axis',(0.,-0.374606593415912,0.927183854566788));
#59989=DIRECTION('ref_axis',(-1.,0.,0.));
#59990=DIRECTION('',(-1.,0.,0.));
#59991=DIRECTION('center_axis',(0.,-0.866025403784439,-0.5));
#59992=DIRECTION('ref_axis',(1.,0.,0.));
#59993=DIRECTION('center_axis',(1.,0.,0.));
#59994=DIRECTION('ref_axis',(0.,1.,0.));
#59995=DIRECTION('center_axis',(1.,0.,0.));
#59996=DIRECTION('ref_axis',(0.,0.,-1.));
#59997=DIRECTION('center_axis',(0.649305557988371,-0.386503331141725,0.654994249884502));
#59998=DIRECTION('ref_axis',(0.760527640763576,0.329979803021199,-0.559205719957048));
#59999=DIRECTION('',(1.,0.,0.));
#60000=DIRECTION('center_axis',(-0.99026806874157,-0.130779935984066,-0.0476000039374393));
#60001=DIRECTION('ref_axis',(-0.139173100960065,0.930547596796367,0.338691626801823));
#60002=DIRECTION('center_axis',(-0.0617712249622996,-0.468811987424191,
0.881135424446229));
#60003=DIRECTION('ref_axis',(-0.998090334472114,0.0290144987282327,-0.0545329542285434));
#60004=DIRECTION('center_axis',(0.284551435696759,-0.455187678719166,0.843702943923494));
#60005=DIRECTION('ref_axis',(0.958660774436356,0.135109635175349,-0.250429443236754));
#60006=DIRECTION('center_axis',(0.491310548314114,-0.424846618249727,0.760341565401402));
#60007=DIRECTION('ref_axis',(0.870984468928858,0.239650226161174,-0.428898384218936));
#60008=DIRECTION('center_axis',(0.313150259135956,-0.452091025520515,0.835194959184317));
#60009=DIRECTION('ref_axis',(0.949703593340092,0.149070112809494,-0.27539278542453));
#60010=DIRECTION('',(1.,0.,0.));
#60011=DIRECTION('center_axis',(-0.313150259135957,-0.452091025520515,0.835194959184317));
#60012=DIRECTION('ref_axis',(-0.949703593340092,0.149070112809494,-0.275392785424531));
#60013=DIRECTION('center_axis',(-0.491310548314113,-0.424846618249727,0.760341565401403));
#60014=DIRECTION('ref_axis',(-0.870984468928858,0.239650226161173,-0.428898384218935));
#60015=DIRECTION('center_axis',(-0.284551435696759,-0.455187678719166,0.843702943923494));
#60016=DIRECTION('ref_axis',(-0.958660774436356,0.135109635175349,-0.250429443236754));
#60017=DIRECTION('center_axis',(0.0617712249622997,-0.468811987424191,0.881135424446229));
#60018=DIRECTION('ref_axis',(0.998090334472114,0.0290144987282327,-0.0545329542285435));
#60019=DIRECTION('center_axis',(0.99026806874157,-0.130779935984066,-0.0476000039374394));
#60020=DIRECTION('ref_axis',(0.139173100960066,0.930547596796366,0.338691626801825));
#60021=DIRECTION('',(1.,0.,0.));
#60022=DIRECTION('center_axis',(0.,0.469471562785891,-0.882947592858927));
#60023=DIRECTION('ref_axis',(1.,0.,0.));
#60024=DIRECTION('',(-0.137844537491629,-0.874518866989312,-0.464989929744128));
#60025=DIRECTION('center_axis',(-0.99026806874157,0.130779935984066,0.0476000039374394));
#60026=DIRECTION('ref_axis',(0.,0.342020143325669,-0.939692620785909));
#60027=DIRECTION('',(-0.137998583506848,-0.878353971058417,-0.457657833403968));
#60028=DIRECTION('center_axis',(-0.0617712249622997,0.468811987424191,-0.881135424446229));
#60029=DIRECTION('ref_axis',(0.998052578482889,0.0213346303712044,-0.058616415197295));
#60030=DIRECTION('',(0.0161503784824051,-0.882236242379483,-0.470529890556386));
#60031=DIRECTION('center_axis',(0.284551435696759,0.455187678719166,-0.843702943923494));
#60032=DIRECTION('ref_axis',(0.957826285221151,-0.0982787650057293,0.270018687665128));
#60033=DIRECTION('',(0.0552259184163645,-0.886406742738186,-0.459601114406122));
#60034=DIRECTION('center_axis',(0.491310548314113,0.424846618249727,-0.760341565401403));
#60035=DIRECTION('ref_axis',(0.86824314212446,-0.169689510806249,0.46621809925847));
#60036=DIRECTION('',(0.057078643955053,-0.886796551036219,-0.458621745531673));
#60037=DIRECTION('center_axis',(0.313150259135957,0.452091025520515,-0.835194959184317));
#60038=DIRECTION('ref_axis',(0.948683298050513,-0.108156265856636,0.297156898213637));
#60039=DIRECTION('',(0.0225789275220278,-0.88272249730729,-0.469351877358061));
#60040=DIRECTION('center_axis',(0.,0.469471562785891,-0.882947592858927));
#60041=DIRECTION('ref_axis',(1.,0.,0.));
#60042=DIRECTION('',(-0.0225789275220274,-0.88272249730729,-0.46935187735806));
#60043=DIRECTION('center_axis',(-0.313150259135956,0.452091025520515,-0.835194959184317));
#60044=DIRECTION('ref_axis',(0.948683298050514,0.108156265856635,-0.297156898213636));
#60045=DIRECTION('',(-0.0570786439550527,-0.886796551036219,-0.458621745531673));
#60046=DIRECTION('center_axis',(-0.491310548314114,0.424846618249727,-0.760341565401402));
#60047=DIRECTION('ref_axis',(0.868243142124459,0.169689510806249,-0.466218099258471));
#60048=DIRECTION('',(-0.0552259184163635,-0.886406742738186,-0.459601114406122));
#60049=DIRECTION('center_axis',(-0.284551435696759,0.455187678719166,-0.843702943923494));
#60050=DIRECTION('ref_axis',(0.957826285221151,0.0982787650057295,-0.270018687665129));
#60051=DIRECTION('',(-0.0161503784824052,-0.882236242379483,-0.470529890556386));
#60052=DIRECTION('center_axis',(0.0617712249622996,0.468811987424191,-0.881135424446229));
#60053=DIRECTION('ref_axis',(0.998052578482889,-0.0213346303712044,0.0586164151972949));
#60054=DIRECTION('',(0.137998583506848,-0.878353971058417,-0.457657833403968));
#60055=DIRECTION('center_axis',(0.99026806874157,0.130779935984066,0.0476000039374393));
#60056=DIRECTION('ref_axis',(0.,-0.342020143325669,0.939692620785909));
#60057=DIRECTION('',(0.137844537491629,-0.874518866989312,-0.464989929744127));
#60058=DIRECTION('center_axis',(0.,0.469471562785891,-0.882947592858927));
#60059=DIRECTION('ref_axis',(1.,0.,0.));
#60060=DIRECTION('',(-0.0519254248777279,-0.881756465810299,-0.468838229299828));
#60061=DIRECTION('center_axis',(-0.649305557988371,0.386503331141725,-0.654994249884502));
#60062=DIRECTION('ref_axis',(0.755033118392644,0.224258043872452,-0.616143911670627));
#60063=DIRECTION('center_axis',(0.,-0.207911690817759,0.978147600733806));
#60064=DIRECTION('ref_axis',(-1.,0.,0.));
#60065=DIRECTION('',(-1.,0.,0.));
#60066=DIRECTION('',(0.137844537491629,-0.968810083928407,-0.205926940351068));
#60067=DIRECTION('center_axis',(0.99026806874157,0.130779935984066,0.0476000039374393));
#60068=DIRECTION('ref_axis',(0.,-0.342020143325669,0.939692620785909));
#60069=DIRECTION('center_axis',(-0.99026806874157,-0.130779935984066,-0.0476000039374393));
#60070=DIRECTION('ref_axis',(-0.139173100960065,0.930547596796367,0.338691626801823));
#60071=DIRECTION('',(0.137998583506848,-0.967034963408845,-0.214008809386339));
#60072=DIRECTION('center_axis',(0.0617712249622996,-0.20725211545606,0.976335432321108));
#60073=DIRECTION('ref_axis',(-0.998052578482889,-0.0213346303712044,0.0586164151972949));
#60074=DIRECTION('center_axis',(-0.0617712249622996,0.20725211545606,-0.976335432321108));
#60075=DIRECTION('ref_axis',(0.998090334472114,0.0128267117770656,-0.0604248268374111));
#60076=DIRECTION('',(-0.0161503784824054,-0.978282954629779,-0.206643717435842));
#60077=DIRECTION('center_axis',(-0.284551435696759,-0.193627806751035,0.938902951798373));
#60078=DIRECTION('ref_axis',(-0.957826285221151,0.0982787650057295,-0.270018687665129));
#60079=DIRECTION('center_axis',(0.284551435696759,0.193627806751035,-0.938902951798373));
#60080=DIRECTION('ref_axis',(-0.958660774436356,0.0574729579753754,-0.278686882824879));
#60081=DIRECTION('',(-0.0552259184163638,-0.974452861356161,-0.21769639163261));
#60082=DIRECTION('center_axis',(-0.491310548314114,-0.163286746281596,0.855541573276281));
#60083=DIRECTION('ref_axis',(-0.868243142124459,0.169689510806249,-0.466218099258471));
#60084=DIRECTION('center_axis',(0.491310548314114,0.163286746281596,-0.855541573276281));
#60085=DIRECTION('ref_axis',(-0.870984468928858,0.0921078431475352,-0.482599419928604));
#60086=DIRECTION('',(-0.0570786439550532,-0.974121945658943,-0.218697195660774));
#60087=DIRECTION('center_axis',(-0.313150259135956,-0.190531153552383,0.930394967059196));
#60088=DIRECTION('ref_axis',(-0.948683298050514,0.108156265856635,-0.297156898213636));
#60089=DIRECTION('center_axis',(0.313150259135956,0.190531153552383,-0.930394967059196));
#60090=DIRECTION('ref_axis',(-0.949703593340092,0.0628247387151195,-0.306783534438035));
#60091=DIRECTION('',(-0.0225789275220273,-0.977898235227234,-0.207858686543083));
#60092=DIRECTION('center_axis',(0.,-0.207911690817759,0.978147600733806));
#60093=DIRECTION('ref_axis',(-1.,0.,0.));
#60094=DIRECTION('',(-1.,0.,0.));
#60095=DIRECTION('',(0.0225789275220281,-0.977898235227234,-0.207858686543083));
#60096=DIRECTION('center_axis',(0.313150259135957,-0.190531153552383,0.930394967059195));
#60097=DIRECTION('ref_axis',(-0.948683298050513,-0.108156265856636,0.297156898213637));
#60098=DIRECTION('center_axis',(-0.313150259135957,0.190531153552383,-0.930394967059195));
#60099=DIRECTION('ref_axis',(0.949703593340092,0.0628247387151197,-0.306783534438037));
#60100=DIRECTION('',(0.0570786439550534,-0.974121945658943,-0.218697195660774));
#60101=DIRECTION('center_axis',(0.491310548314113,-0.163286746281596,0.855541573276282));
#60102=DIRECTION('ref_axis',(-0.86824314212446,-0.169689510806249,0.46621809925847));
#60103=DIRECTION('center_axis',(-0.491310548314113,0.163286746281596,-0.855541573276282));
#60104=DIRECTION('ref_axis',(0.870984468928858,0.0921078431475348,-0.482599419928602));
#60105=DIRECTION('',(0.0552259184163649,-0.974452861356161,-0.21769639163261));
#60106=DIRECTION('center_axis',(0.284551435696759,-0.193627806751035,0.938902951798373));
#60107=DIRECTION('ref_axis',(-0.957826285221151,-0.0982787650057293,0.270018687665128));
#60108=DIRECTION('center_axis',(-0.284551435696759,0.193627806751035,-0.938902951798373));
#60109=DIRECTION('ref_axis',(0.958660774436356,0.0574729579753754,-0.278686882824878));
#60110=DIRECTION('',(0.0161503784824051,-0.978282954629779,-0.206643717435842));
#60111=DIRECTION('center_axis',(-0.0617712249622997,-0.20725211545606,0.976335432321108));
#60112=DIRECTION('ref_axis',(-0.998052578482889,0.0213346303712044,-0.058616415197295));
#60113=DIRECTION('center_axis',(0.0617712249622997,0.20725211545606,-0.976335432321108));
#60114=DIRECTION('ref_axis',(-0.998090334472114,0.0128267117770656,-0.0604248268374111));
#60115=DIRECTION('',(-0.137998583506848,-0.967034963408845,-0.214008809386339));
#60116=DIRECTION('center_axis',(-0.99026806874157,0.130779935984066,0.0476000039374394));
#60117=DIRECTION('ref_axis',(0.,0.342020143325669,-0.939692620785909));
#60118=DIRECTION('center_axis',(0.99026806874157,-0.130779935984066,-0.0476000039374394));
#60119=DIRECTION('ref_axis',(0.139173100960066,0.930547596796366,0.338691626801825));
#60120=DIRECTION('',(-0.137844537491629,-0.968810083928407,-0.205926940351068));
#60121=DIRECTION('center_axis',(0.,-0.207911690817759,0.978147600733806));
#60122=DIRECTION('ref_axis',(-1.,0.,0.));
#60123=DIRECTION('',(-1.,0.,0.));
#60124=DIRECTION('center_axis',(0.,-0.939692620785908,-0.342020143325669));
#60125=DIRECTION('ref_axis',(1.,0.,0.));
#60126=DIRECTION('center_axis',(1.,0.,0.));
#60127=DIRECTION('ref_axis',(0.,1.,0.));
#60128=DIRECTION('center_axis',(1.,0.,0.));
#60129=DIRECTION('ref_axis',(0.,0.,-1.));
#60130=DIRECTION('center_axis',(0.649305557988371,-0.266892919198654,0.712159014579632));
#60131=DIRECTION('ref_axis',(0.760527640763576,0.227861614141252,-0.608010520003998));
#60132=DIRECTION('',(1.,0.,0.));
#60133=DIRECTION('center_axis',(-0.99026806874157,-0.137058748836223,-0.024167155361971));
#60134=DIRECTION('ref_axis',(-0.139173100960065,0.975223671657125,0.171958245538723));
#60135=DIRECTION('center_axis',(-0.0617712249622996,-0.30868211918754,0.949157344732972));
#60136=DIRECTION('ref_axis',(-0.998090334472114,0.0191041551727457,-0.0587427909490065));
#60137=DIRECTION('center_axis',(0.284551435696759,-0.301764876373726,0.909927711321105));
#60138=DIRECTION('ref_axis',(0.958660774436356,0.0895703997751285,-0.27008639921553));
#60139=DIRECTION('center_axis',(0.491310548314114,-0.286360316256974,0.822564109591763));
#60140=DIRECTION('ref_axis',(0.870984468928858,0.161531977910744,-0.463997279083573));
#60141=DIRECTION('center_axis',(0.313150259135956,-0.30019266434088,0.901011253802641));
#60142=DIRECTION('ref_axis',(0.949703593340092,0.0989839475056044,-0.297094703643677));
#60143=DIRECTION('',(1.,0.,0.));
#60144=DIRECTION('center_axis',(-0.313150259135957,-0.30019266434088,0.901011253802641));
#60145=DIRECTION('ref_axis',(-0.949703593340092,0.0989839475056048,-0.297094703643678));
#60146=DIRECTION('center_axis',(-0.491310548314113,-0.286360316256974,0.822564109591764));
#60147=DIRECTION('ref_axis',(-0.870984468928858,0.161531977910743,-0.463997279083571));
#60148=DIRECTION('center_axis',(-0.284551435696759,-0.301764876373726,0.909927711321105));
#60149=DIRECTION('ref_axis',(-0.958660774436356,0.0895703997751283,-0.270086399215529));
#60150=DIRECTION('center_axis',(0.0617712249622997,-0.30868211918754,0.949157344732972));
#60151=DIRECTION('ref_axis',(0.998090334472114,0.0191041551727457,-0.0587427909490066));
#60152=DIRECTION('center_axis',(0.99026806874157,-0.137058748836224,-0.0241671553619711));
#60153=DIRECTION('ref_axis',(0.139173100960066,0.975223671657125,0.171958245538724));
#60154=DIRECTION('',(1.,0.,0.));
#60155=DIRECTION('center_axis',(0.,0.309016994374947,-0.951056516295154));
#60156=DIRECTION('ref_axis',(1.,0.,0.));
#60157=DIRECTION('',(-0.137844537491629,-0.941977614300068,-0.306067080296576));
#60158=DIRECTION('center_axis',(-0.99026806874157,0.137058748836224,0.0241671553619711));
#60159=DIRECTION('ref_axis',(0.,0.17364817766693,-0.984807753012208));
#60160=DIRECTION('',(-0.137998583506848,-0.944481249352984,-0.298180416142191));
#60161=DIRECTION('center_axis',(-0.0617712249622997,0.30868211918754,-0.949157344732972));
#60162=DIRECTION('ref_axis',(0.998052578482889,0.0108318757168334,-0.0614306198252359));
#60163=DIRECTION('',(0.0161503784824051,-0.950539749516609,-0.310182768482997));
#60164=DIRECTION('center_axis',(0.284551435696759,0.301764876373726,-0.909927711321105));
#60165=DIRECTION('ref_axis',(0.957826285221151,-0.0498974366850414,0.282982425517402));
#60166=DIRECTION('',(0.0552259184163645,-0.952749128541176,-0.298695825212034));
#60167=DIRECTION('center_axis',(0.491310548314113,0.286360316256974,-0.822564109591764));
#60168=DIRECTION('ref_axis',(0.86824314212446,-0.0861536225152693,0.488601473065054));
#60169=DIRECTION('',(0.057078643955053,-0.952962949154956,-0.297663645650825));
#60170=DIRECTION('center_axis',(0.313150259135957,0.30019266434088,-0.901011253802641));
#60171=DIRECTION('ref_axis',(0.948683298050513,-0.0549123752965086,0.311423555691114));
#60172=DIRECTION('',(0.0225789275220278,-0.950814057294297,-0.30893821467004));
#60173=DIRECTION('center_axis',(0.,0.309016994374947,-0.951056516295154));
#60174=DIRECTION('ref_axis',(1.,0.,0.));
#60175=DIRECTION('',(-0.0225789275220274,-0.950814057294297,-0.30893821467004));
#60176=DIRECTION('center_axis',(-0.313150259135956,0.30019266434088,-0.901011253802641));
#60177=DIRECTION('ref_axis',(0.948683298050514,0.0549123752965084,-0.311423555691113));
#60178=DIRECTION('',(-0.0570786439550527,-0.952962949154956,-0.297663645650825));
#60179=DIRECTION('center_axis',(-0.491310548314114,0.286360316256974,-0.822564109591763));
#60180=DIRECTION('ref_axis',(0.868243142124459,0.0861536225152694,-0.488601473065055));
#60181=DIRECTION('',(-0.0552259184163635,-0.952749128541176,-0.298695825212034));
#60182=DIRECTION('center_axis',(-0.284551435696759,0.301764876373726,-0.909927711321105));
#60183=DIRECTION('ref_axis',(0.957826285221151,0.0498974366850415,-0.282982425517402));
#60184=DIRECTION('',(-0.0161503784824052,-0.950539749516609,-0.310182768482997));
#60185=DIRECTION('center_axis',(0.0617712249622996,0.30868211918754,-0.949157344732972));
#60186=DIRECTION('ref_axis',(0.998052578482889,-0.0108318757168334,0.0614306198252359));
#60187=DIRECTION('',(0.137998583506848,-0.944481249352984,-0.298180416142191));
#60188=DIRECTION('center_axis',(0.99026806874157,0.137058748836223,0.024167155361971));
#60189=DIRECTION('ref_axis',(0.,-0.17364817766693,0.984807753012208));
#60190=DIRECTION('',(0.137844537491629,-0.941977614300068,-0.306067080296576));
#60191=DIRECTION('center_axis',(0.,0.309016994374947,-0.951056516295154));
#60192=DIRECTION('ref_axis',(1.,0.,0.));
#60193=DIRECTION('',(-0.051925424877728,-0.949773507937132,-0.308600119688995));
#60194=DIRECTION('center_axis',(-0.649305557988371,0.266892919198654,-0.712159014579632));
#60195=DIRECTION('ref_axis',(0.755033118392644,0.113858792838764,-0.645725301830105));
#60196=DIRECTION('center_axis',(0.,-0.0348994967025007,0.999390827019096));
#60197=DIRECTION('ref_axis',(-1.,0.,0.));
#60198=DIRECTION('',(-1.,0.,0.));
#60199=DIRECTION('',(0.137844537491629,-0.989850519773593,-0.0345663418323));
#60200=DIRECTION('center_axis',(0.99026806874157,0.137058748836223,0.024167155361971));
#60201=DIRECTION('ref_axis',(0.,-0.17364817766693,0.984807753012208));
#60202=DIRECTION('center_axis',(-0.99026806874157,-0.137058748836223,-0.024167155361971));
#60203=DIRECTION('ref_axis',(-0.139173100960065,0.975223671657125,0.171958245538723));
#60204=DIRECTION('',(0.137998583506848,-0.989505769153514,-0.0428336755604255));
#60205=DIRECTION('center_axis',(0.0617712249622996,-0.0345646215150938,
0.997491655456914));
#60206=DIRECTION('ref_axis',(-0.998052578482889,-0.0108318757168334,0.0614306198252359));
#60207=DIRECTION('center_axis',(-0.0617712249622996,0.0345646215150938,
-0.997491655456914));
#60208=DIRECTION('ref_axis',(0.998090334472114,0.00213918413755088,-0.061734173069449));
#60209=DIRECTION('',(-0.0161503784824054,-0.999303943318151,-0.0336272827279993));
#60210=DIRECTION('center_axis',(-0.284551435696759,-0.0276473787012792,
0.958262022045047));
#60211=DIRECTION('ref_axis',(-0.957826285221151,0.0498974366850415,-0.282982425517402));
#60212=DIRECTION('center_axis',(0.284551435696759,0.0276473787012792,-0.958262022045047));
#60213=DIRECTION('ref_axis',(-0.958660774436356,0.00820634526047697,-0.284433077286297));
#60214=DIRECTION('',(-0.0552259184163638,-0.997451314500147,-0.0451771306857527));
#60215=DIRECTION('center_axis',(-0.491310548314114,-0.0122428185845277,
0.870898420315705));
#60216=DIRECTION('ref_axis',(-0.868243142124459,0.0861536225152694,-0.488601473065055));
#60217=DIRECTION('center_axis',(0.491310548314114,0.0122428185845277,-0.870898420315705));
#60218=DIRECTION('ref_axis',(-0.870984468928858,0.00690600823120518,-0.491262009456284));
#60219=DIRECTION('',(-0.0570786439550532,-0.997299213951626,-0.0462201931597179));
#60220=DIRECTION('center_axis',(-0.313150259135956,-0.0260751666684334,
0.949345564526583));
#60221=DIRECTION('ref_axis',(-0.948683298050514,0.0549123752965084,-0.311423555691113));
#60222=DIRECTION('center_axis',(0.313150259135956,0.0260751666684334,-0.949345564526583));
#60223=DIRECTION('ref_axis',(-0.949703593340092,0.00859788807423102,-0.313032204601347));
#60224=DIRECTION('',(-0.0225789275220273,-0.999136045839184,-0.0348905995476462));
#60225=DIRECTION('center_axis',(0.,-0.0348994967025007,0.999390827019096));
#60226=DIRECTION('ref_axis',(-1.,0.,0.));
#60227=DIRECTION('',(-1.,0.,0.));
#60228=DIRECTION('',(0.0225789275220281,-0.999136045839184,-0.0348905995476462));
#60229=DIRECTION('center_axis',(0.313150259135957,-0.0260751666684331,0.949345564526583));
#60230=DIRECTION('ref_axis',(-0.948683298050513,-0.0549123752965086,0.311423555691114));
#60231=DIRECTION('center_axis',(-0.313150259135957,0.0260751666684331,-0.949345564526583));
#60232=DIRECTION('ref_axis',(0.949703593340092,0.00859788807423098,-0.313032204601348));
#60233=DIRECTION('',(0.0570786439550534,-0.997299213951626,-0.0462201931597178));
#60234=DIRECTION('center_axis',(0.491310548314113,-0.0122428185845276,0.870898420315706));
#60235=DIRECTION('ref_axis',(-0.86824314212446,-0.0861536225152693,0.488601473065054));
#60236=DIRECTION('center_axis',(-0.491310548314113,0.0122428185845276,-0.870898420315706));
#60237=DIRECTION('ref_axis',(0.870984468928858,0.00690600823120505,-0.491262009456283));
#60238=DIRECTION('',(0.0552259184163649,-0.997451314500147,-0.0451771306857531));
#60239=DIRECTION('center_axis',(0.284551435696759,-0.0276473787012793,0.958262022045047));
#60240=DIRECTION('ref_axis',(-0.957826285221151,-0.0498974366850414,0.282982425517402));
#60241=DIRECTION('center_axis',(-0.284551435696759,0.0276473787012793,-0.958262022045047));
#60242=DIRECTION('ref_axis',(0.958660774436356,0.00820634526047701,-0.284433077286297));
#60243=DIRECTION('',(0.0161503784824051,-0.999303943318151,-0.0336272827279993));
#60244=DIRECTION('center_axis',(-0.0617712249622997,-0.0345646215150938,
0.997491655456914));
#60245=DIRECTION('ref_axis',(-0.998052578482889,0.0108318757168334,-0.0614306198252359));
#60246=DIRECTION('center_axis',(0.0617712249622997,0.0345646215150938,-0.997491655456914));
#60247=DIRECTION('ref_axis',(-0.998090334472114,0.00213918413755088,-0.061734173069449));
#60248=DIRECTION('',(-0.137998583506848,-0.989505769153514,-0.0428336755604255));
#60249=DIRECTION('center_axis',(-0.99026806874157,0.137058748836224,0.0241671553619711));
#60250=DIRECTION('ref_axis',(0.,0.17364817766693,-0.984807753012208));
#60251=DIRECTION('center_axis',(0.99026806874157,-0.137058748836224,-0.0241671553619711));
#60252=DIRECTION('ref_axis',(0.139173100960066,0.975223671657125,0.171958245538724));
#60253=DIRECTION('',(-0.137844537491629,-0.989850519773593,-0.0345663418323));
#60254=DIRECTION('center_axis',(0.,-0.0348994967025007,0.999390827019096));
#60255=DIRECTION('ref_axis',(-1.,0.,0.));
#60256=DIRECTION('',(-1.,0.,0.));
#60257=DIRECTION('center_axis',(0.,-0.984807753012208,-0.17364817766693));
#60258=DIRECTION('ref_axis',(1.,0.,0.));
#60259=DIRECTION('center_axis',(1.,0.,0.));
#60260=DIRECTION('ref_axis',(0.,1.,0.));
#60261=DIRECTION('center_axis',(1.,0.,0.));
#60262=DIRECTION('ref_axis',(0.,0.,-1.));
#60263=DIRECTION('center_axis',(0.649305557988371,-0.139173100960065,0.747685187986609));
#60264=DIRECTION('ref_axis',(0.760527640763576,0.118819965419165,-0.638341228068795));
#60265=DIRECTION('',(1.,0.,0.));
#60266=DIRECTION('center_axis',(-0.99026806874157,-0.139173100960065,1.70437892618156E-17));
#60267=DIRECTION('ref_axis',(-0.139173100960065,0.99026806874157,0.));
#60268=DIRECTION('center_axis',(-0.0617712249622996,-0.139173100960065,
0.988339599396795));
#60269=DIRECTION('ref_axis',(-0.998090334472114,0.00861334152950385,-0.0611677576917705));
#60270=DIRECTION('center_axis',(0.284551435696759,-0.139173100960065,0.948504785655862));
#60271=DIRECTION('ref_axis',(0.958660774436356,0.0413096131025498,-0.281536916624453));
#60272=DIRECTION('center_axis',(0.491310548314114,-0.139173100960065,0.859793459549701));
#60273=DIRECTION('ref_axis',(0.870984468928858,0.0785056622506208,-0.484997851417207));
#60274=DIRECTION('center_axis',(0.313150259135956,-0.139173100960065,0.939450777407866));
#60275=DIRECTION('ref_axis',(0.949703593340092,0.0458902050450515,-0.309769549629784));
#60276=DIRECTION('',(1.,0.,0.));
#60277=DIRECTION('center_axis',(-0.313150259135957,-0.139173100960065,0.939450777407865));
#60278=DIRECTION('ref_axis',(-0.949703593340092,0.0458902050450517,-0.309769549629785));
#60279=DIRECTION('center_axis',(-0.491310548314113,-0.139173100960065,0.859793459549702));
#60280=DIRECTION('ref_axis',(-0.870984468928858,0.0785056622506207,-0.484997851417206));
#60281=DIRECTION('center_axis',(-0.284551435696759,-0.139173100960065,0.948504785655862));
#60282=DIRECTION('ref_axis',(-0.958660774436356,0.0413096131025497,-0.281536916624453));
#60283=DIRECTION('center_axis',(0.0617712249622997,-0.139173100960065,0.988339599396795));
#60284=DIRECTION('ref_axis',(0.998090334472114,0.00861334152950384,-0.0611677576917706));
#60285=DIRECTION('center_axis',(0.99026806874157,-0.139173100960066,1.70437892618156E-17));
#60286=DIRECTION('ref_axis',(0.139173100960066,0.99026806874157,0.));
#60287=DIRECTION('',(1.,0.,0.));
#60288=DIRECTION('center_axis',(0.,0.139173100960066,-0.99026806874157));
#60289=DIRECTION('ref_axis',(1.,0.,0.));
#60290=DIRECTION('',(-0.137844537491629,-0.980814848463989,-0.137844537491629));
#60291=DIRECTION('center_axis',(-0.99026806874157,0.139173100960066,-1.70437892618156E-17));
#60292=DIRECTION('ref_axis',(0.,-1.22464679914735E-16,-1.));
#60293=DIRECTION('',(-0.137998583506848,-0.981910942816533,-0.129642937822505));
#60294=DIRECTION('center_axis',(-0.0617712249622997,0.139173100960065,-0.988339599396795));
#60295=DIRECTION('ref_axis',(0.998052578482889,-7.63913684762395E-18,-0.0623782861551806));
#60296=DIRECTION('',(0.0161503784824051,-0.989961587360995,-0.140410899949307));
#60297=DIRECTION('center_axis',(0.284551435696759,0.139173100960065,-0.948504785655862));
#60298=DIRECTION('ref_axis',(0.957826285221151,3.51899668300585E-17,0.287347885566345));
#60299=DIRECTION('',(0.0552259184163645,-0.990142714187765,-0.128714814516259));
#60300=DIRECTION('center_axis',(0.491310548314113,0.139173100960065,-0.859793459549702));
#60301=DIRECTION('ref_axis',(0.86824314212446,6.0759496279106E-17,0.496138938356832));
#60302=DIRECTION('',(0.057078643955053,-0.99017405028614,-0.12766118652195));
#60303=DIRECTION('center_axis',(0.313150259135957,0.139173100960065,-0.939450777407865));
#60304=DIRECTION('ref_axis',(0.948683298050513,3.87267321454041E-17,0.31622776601684));
#60305=DIRECTION('',(0.0225789275220278,-0.990015613285545,-0.13913762065955));
#60306=DIRECTION('center_axis',(0.,0.139173100960065,-0.99026806874157));
#60307=DIRECTION('ref_axis',(1.,0.,0.));
#60308=DIRECTION('',(-0.0225789275220274,-0.990015613285545,-0.13913762065955));
#60309=DIRECTION('center_axis',(-0.313150259135956,0.139173100960065,-0.939450777407866));
#60310=DIRECTION('ref_axis',(0.948683298050514,-3.8726732145404E-17,-0.316227766016839));
#60311=DIRECTION('',(-0.0570786439550527,-0.99017405028614,-0.12766118652195));
#60312=DIRECTION('center_axis',(-0.491310548314114,0.139173100960065,-0.859793459549701));
#60313=DIRECTION('ref_axis',(0.868243142124459,-6.07594962791062E-17,-0.496138938356833));
#60314=DIRECTION('',(-0.0552259184163635,-0.990142714187765,-0.128714814516259));
#60315=DIRECTION('center_axis',(-0.284551435696759,0.139173100960065,-0.948504785655862));
#60316=DIRECTION('ref_axis',(0.957826285221151,-3.51899668300585E-17,-0.287347885566346));
#60317=DIRECTION('',(-0.0161503784824052,-0.989961587360995,-0.140410899949307));
#60318=DIRECTION('center_axis',(0.0617712249622996,0.139173100960065,-0.988339599396795));
#60319=DIRECTION('ref_axis',(0.998052578482889,7.63913684762395E-18,0.0623782861551805));
#60320=DIRECTION('',(0.137998583506848,-0.981910942816534,-0.129642937822505));
#60321=DIRECTION('center_axis',(0.99026806874157,0.139173100960065,-1.70437892618156E-17));
#60322=DIRECTION('ref_axis',(0.,1.22464679914735E-16,1.));
#60323=DIRECTION('',(0.137844537491629,-0.980814848463989,-0.137844537491628));
#60324=DIRECTION('center_axis',(0.,0.139173100960065,-0.99026806874157));
#60325=DIRECTION('ref_axis',(1.,0.,0.));
#60326=DIRECTION('',(-0.051925424877728,-0.98893216263388,-0.138985351600607));
#60327=DIRECTION('center_axis',(-0.649305557988371,0.139173100960065,-0.747685187986609));
#60328=DIRECTION('ref_axis',(0.755033118392644,-8.02984563835875E-17,-0.655686655446243));
#60329=DIRECTION('center_axis',(0.,0.139173100960066,0.99026806874157));
#60330=DIRECTION('ref_axis',(-1.,0.,0.));
#60331=DIRECTION('',(-1.,0.,0.));
#60332=DIRECTION('',(0.137844537491629,-0.980814848463989,0.137844537491629));
#60333=DIRECTION('center_axis',(0.99026806874157,0.139173100960065,-1.70437892618156E-17));
#60334=DIRECTION('ref_axis',(0.,1.22464679914735E-16,1.));
#60335=DIRECTION('center_axis',(-0.99026806874157,-0.139173100960065,1.70437892618156E-17));
#60336=DIRECTION('ref_axis',(-0.139173100960065,0.99026806874157,0.));
#60337=DIRECTION('',(0.137998583506848,-0.981910942816534,0.129642937822505));
#60338=DIRECTION('center_axis',(0.0617712249622996,0.139173100960066,0.988339599396795));
#60339=DIRECTION('ref_axis',(-0.998052578482889,7.63913684762395E-18,0.0623782861551805));
#60340=DIRECTION('center_axis',(-0.0617712249622996,-0.139173100960066,
-0.988339599396795));
#60341=DIRECTION('ref_axis',(-0.998090334472114,0.00861334152950386,0.0611677576917705));
#60342=DIRECTION('',(-0.0161503784824054,-0.989961587360995,0.140410899949307));
#60343=DIRECTION('center_axis',(-0.284551435696759,0.139173100960066,0.948504785655862));
#60344=DIRECTION('ref_axis',(-0.957826285221151,-3.51899668300585E-17,-0.287347885566346));
#60345=DIRECTION('center_axis',(0.284551435696759,-0.139173100960066,-0.948504785655862));
#60346=DIRECTION('ref_axis',(0.958660774436356,0.0413096131025499,0.281536916624453));
#60347=DIRECTION('',(-0.0552259184163638,-0.990142714187765,0.12871481451626));
#60348=DIRECTION('center_axis',(-0.491310548314114,0.139173100960066,0.859793459549701));
#60349=DIRECTION('ref_axis',(-0.868243142124459,-6.07594962791062E-17,-0.496138938356833));
#60350=DIRECTION('center_axis',(0.491310548314114,-0.139173100960066,-0.859793459549701));
#60351=DIRECTION('ref_axis',(0.870984468928858,0.078505662250621,0.484997851417207));
#60352=DIRECTION('',(-0.0570786439550532,-0.99017405028614,0.12766118652195));
#60353=DIRECTION('center_axis',(-0.313150259135956,0.139173100960065,0.939450777407866));
#60354=DIRECTION('ref_axis',(-0.948683298050514,-3.8726732145404E-17,-0.316227766016839));
#60355=DIRECTION('center_axis',(0.313150259135956,-0.139173100960065,-0.939450777407866));
#60356=DIRECTION('ref_axis',(0.949703593340092,0.0458902050450515,0.309769549629784));
#60357=DIRECTION('',(-0.0225789275220273,-0.990015613285545,0.139137620659551));
#60358=DIRECTION('center_axis',(0.,0.139173100960066,0.99026806874157));
#60359=DIRECTION('ref_axis',(-1.,0.,0.));
#60360=DIRECTION('',(-1.,0.,0.));
#60361=DIRECTION('',(0.0225789275220281,-0.990015613285545,0.139137620659551));
#60362=DIRECTION('center_axis',(0.313150259135957,0.139173100960066,0.939450777407865));
#60363=DIRECTION('ref_axis',(-0.948683298050513,3.87267321454041E-17,0.31622776601684));
#60364=DIRECTION('center_axis',(-0.313150259135957,-0.139173100960066,-0.939450777407865));
#60365=DIRECTION('ref_axis',(-0.949703593340092,0.0458902050450518,0.309769549629785));
#60366=DIRECTION('',(0.0570786439550534,-0.99017405028614,0.12766118652195));
#60367=DIRECTION('center_axis',(0.491310548314113,0.139173100960066,0.859793459549702));
#60368=DIRECTION('ref_axis',(-0.86824314212446,6.0759496279106E-17,0.496138938356832));
#60369=DIRECTION('center_axis',(-0.491310548314113,-0.139173100960066,-0.859793459549702));
#60370=DIRECTION('ref_axis',(-0.870984468928858,0.0785056622506208,0.484997851417206));
#60371=DIRECTION('',(0.0552259184163649,-0.990142714187765,0.128714814516259));
#60372=DIRECTION('center_axis',(0.284551435696759,0.139173100960066,0.948504785655862));
#60373=DIRECTION('ref_axis',(-0.957826285221151,3.51899668300585E-17,0.287347885566345));
#60374=DIRECTION('center_axis',(-0.284551435696759,-0.139173100960066,-0.948504785655862));
#60375=DIRECTION('ref_axis',(-0.958660774436356,0.0413096131025497,0.281536916624453));
#60376=DIRECTION('',(0.0161503784824051,-0.989961587360995,0.140410899949307));
#60377=DIRECTION('center_axis',(-0.0617712249622997,0.139173100960066,0.988339599396795));
#60378=DIRECTION('ref_axis',(-0.998052578482889,-7.63913684762395E-18,-0.0623782861551806));
#60379=DIRECTION('center_axis',(0.0617712249622997,-0.139173100960066,-0.988339599396795));
#60380=DIRECTION('ref_axis',(0.998090334472114,0.00861334152950386,0.0611677576917706));
#60381=DIRECTION('',(-0.137998583506848,-0.981910942816533,0.129642937822505));
#60382=DIRECTION('center_axis',(-0.99026806874157,0.139173100960066,-1.70437892618156E-17));
#60383=DIRECTION('ref_axis',(0.,-1.22464679914735E-16,-1.));
#60384=DIRECTION('center_axis',(0.99026806874157,-0.139173100960066,1.70437892618156E-17));
#60385=DIRECTION('ref_axis',(0.139173100960066,0.99026806874157,0.));
#60386=DIRECTION('',(-0.137844537491629,-0.980814848463989,0.137844537491629));
#60387=DIRECTION('center_axis',(0.,0.139173100960066,0.99026806874157));
#60388=DIRECTION('ref_axis',(-1.,0.,0.));
#60389=DIRECTION('',(-1.,0.,0.));
#60390=DIRECTION('center_axis',(0.,-1.,1.22464679914735E-16));
#60391=DIRECTION('ref_axis',(1.,0.,0.));
#60392=DIRECTION('center_axis',(1.,0.,0.));
#60393=DIRECTION('ref_axis',(0.,1.,0.));
#60394=DIRECTION('center_axis',(1.,0.,0.));
#60395=DIRECTION('ref_axis',(0.,0.,-1.));
#60396=DIRECTION('center_axis',(0.649305557988371,-0.0072245784737921,0.760493325303574));
#60397=DIRECTION('ref_axis',(0.760527640763576,0.00616803217361909,-0.649276260934969));
#60398=DIRECTION('',(1.,0.,0.));
#60399=DIRECTION('center_axis',(-0.99026806874157,-0.137058748836223,0.0241671553619711));
#60400=DIRECTION('ref_axis',(-0.139173100960065,0.975223671657125,-0.171958245538723));
#60401=DIRECTION('center_axis',(-0.0617712249622996,0.0345646215150944,
0.997491655456914));
#60402=DIRECTION('ref_axis',(0.998090334472114,0.00213918413755092,0.061734173069449));
#60403=DIRECTION('center_axis',(0.284551435696759,0.0276473787012799,0.958262022045047));
#60404=DIRECTION('ref_axis',(-0.958660774436356,0.00820634526047722,0.284433077286297));
#60405=DIRECTION('center_axis',(0.491310548314114,0.0122428185845284,0.870898420315705));
#60406=DIRECTION('ref_axis',(-0.870984468928858,0.00690600823120551,0.491262009456284));
#60407=DIRECTION('center_axis',(0.313150259135956,0.026075166668434,0.949345564526583));
#60408=DIRECTION('ref_axis',(-0.949703593340092,0.00859788807423123,0.313032204601347));
#60409=DIRECTION('',(1.,0.,0.));
#60410=DIRECTION('center_axis',(-0.313150259135957,0.0260751666684338,0.949345564526583));
#60411=DIRECTION('ref_axis',(0.949703593340092,0.00859788807423126,0.313032204601348));
#60412=DIRECTION('center_axis',(-0.491310548314113,0.0122428185845283,0.870898420315706));
#60413=DIRECTION('ref_axis',(0.870984468928858,0.00690600823120549,0.491262009456283));
#60414=DIRECTION('center_axis',(-0.284551435696759,0.02764737870128,0.958262022045047));
#60415=DIRECTION('ref_axis',(0.958660774436356,0.0082063452604772,0.284433077286297));
#60416=DIRECTION('center_axis',(0.0617712249622997,0.0345646215150945,0.997491655456914));
#60417=DIRECTION('ref_axis',(-0.998090334472114,0.00213918413755093,0.061734173069449));
#60418=DIRECTION('center_axis',(0.99026806874157,-0.137058748836224,0.0241671553619712));
#60419=DIRECTION('ref_axis',(0.139173100960066,0.975223671657125,-0.171958245538724));
#60420=DIRECTION('',(1.,0.,0.));
#60421=DIRECTION('center_axis',(0.,-0.0348994967025011,-0.999390827019096));
#60422=DIRECTION('ref_axis',(1.,0.,0.));
#60423=DIRECTION('',(-0.137844537491629,-0.989850519773593,0.0345663418323005));
#60424=DIRECTION('center_axis',(-0.99026806874157,0.137058748836224,-0.0241671553619712));
#60425=DIRECTION('ref_axis',(0.,-0.173648177666931,-0.984807753012208));
#60426=DIRECTION('',(-0.137998583506848,-0.989505769153514,0.0428336755604262));
#60427=DIRECTION('center_axis',(-0.0617712249622997,-0.0345646215150945,
-0.997491655456914));
#60428=DIRECTION('ref_axis',(0.998052578482889,-0.0108318757168334,-0.0614306198252359));
#60429=DIRECTION('',(0.0161503784824051,-0.999303943318151,0.033627282728));
#60430=DIRECTION('center_axis',(0.284551435696759,-0.02764737870128,-0.958262022045047));
#60431=DIRECTION('ref_axis',(0.957826285221151,0.0498974366850416,0.282982425517402));
#60432=DIRECTION('',(0.0552259184163645,-0.997451314500147,0.0451771306857537));
#60433=DIRECTION('center_axis',(0.491310548314113,-0.0122428185845283,-0.870898420315706));
#60434=DIRECTION('ref_axis',(0.86824314212446,0.0861536225152695,0.488601473065054));
#60435=DIRECTION('',(0.057078643955053,-0.997299213951626,0.0462201931597184));
#60436=DIRECTION('center_axis',(0.313150259135957,-0.0260751666684338,-0.949345564526583));
#60437=DIRECTION('ref_axis',(0.948683298050513,0.0549123752965088,0.311423555691114));
#60438=DIRECTION('',(0.0225789275220278,-0.999136045839184,0.0348905995476467));
#60439=DIRECTION('center_axis',(0.,-0.0348994967025013,-0.999390827019096));
#60440=DIRECTION('ref_axis',(1.,0.,0.));
#60441=DIRECTION('',(-0.0225789275220274,-0.999136045839184,0.0348905995476468));
#60442=DIRECTION('center_axis',(-0.313150259135956,-0.026075166668434,-0.949345564526583));
#60443=DIRECTION('ref_axis',(0.948683298050514,-0.0549123752965086,-0.311423555691113));
#60444=DIRECTION('',(-0.0570786439550527,-0.997299213951626,0.0462201931597183));
#60445=DIRECTION('center_axis',(-0.491310548314114,-0.0122428185845284,
-0.870898420315705));
#60446=DIRECTION('ref_axis',(0.868243142124459,-0.0861536225152698,-0.488601473065055));
#60447=DIRECTION('',(-0.0552259184163635,-0.997451314500147,0.0451771306857533));
#60448=DIRECTION('center_axis',(-0.284551435696759,-0.0276473787012799,
-0.958262022045047));
#60449=DIRECTION('ref_axis',(0.957826285221151,-0.0498974366850417,-0.282982425517402));
#60450=DIRECTION('',(-0.0161503784824052,-0.999303943318151,0.0336272827279999));
#60451=DIRECTION('center_axis',(0.0617712249622996,-0.0345646215150944,
-0.997491655456914));
#60452=DIRECTION('ref_axis',(0.998052578482889,0.0108318757168334,0.0614306198252359));
#60453=DIRECTION('',(0.137998583506848,-0.989505769153514,0.0428336755604261));
#60454=DIRECTION('center_axis',(0.99026806874157,0.137058748836223,-0.0241671553619711));
#60455=DIRECTION('ref_axis',(0.,0.173648177666931,0.984807753012208));
#60456=DIRECTION('',(0.137844537491629,-0.989850519773593,0.0345663418323007));
#60457=DIRECTION('center_axis',(0.,-0.0348994967025013,-0.999390827019096));
#60458=DIRECTION('ref_axis',(1.,0.,0.));
#60459=DIRECTION('',(-0.051925424877728,-0.998042613992818,0.0348524160661849));
#60460=DIRECTION('center_axis',(-0.649305557988371,0.0072245784737921,-0.760493325303574));
#60461=DIRECTION('ref_axis',(0.755033118392644,-0.113858792838765,-0.645725301830104));
#60462=DIRECTION('center_axis',(0.,0.309016994374948,0.951056516295154));
#60463=DIRECTION('ref_axis',(-1.,0.,0.));
#60464=DIRECTION('',(-1.,0.,0.));
#60465=DIRECTION('',(0.137844537491629,-0.941977614300068,0.306067080296576));
#60466=DIRECTION('center_axis',(0.99026806874157,0.137058748836223,-0.0241671553619711));
#60467=DIRECTION('ref_axis',(0.,0.173648177666931,0.984807753012208));
#60468=DIRECTION('center_axis',(-0.99026806874157,-0.137058748836223,0.0241671553619711));
#60469=DIRECTION('ref_axis',(-0.139173100960065,0.975223671657125,-0.171958245538723));
#60470=DIRECTION('',(0.137998583506848,-0.944481249352984,0.298180416142191));
#60471=DIRECTION('center_axis',(0.0617712249622996,0.308682119187541,0.949157344732972));
#60472=DIRECTION('ref_axis',(-0.998052578482889,0.0108318757168334,0.0614306198252359));
#60473=DIRECTION('center_axis',(-0.0617712249622996,-0.308682119187541,
-0.949157344732972));
#60474=DIRECTION('ref_axis',(-0.998090334472114,0.0191041551727458,0.0587427909490065));
#60475=DIRECTION('',(-0.0161503784824054,-0.950539749516609,0.310182768482998));
#60476=DIRECTION('center_axis',(-0.284551435696759,0.301764876373726,0.909927711321104));
#60477=DIRECTION('ref_axis',(-0.957826285221151,-0.0498974366850417,-0.282982425517402));
#60478=DIRECTION('center_axis',(0.284551435696759,-0.301764876373726,-0.909927711321104));
#60479=DIRECTION('ref_axis',(0.958660774436356,0.0895703997751287,0.27008639921553));
#60480=DIRECTION('',(-0.0552259184163638,-0.952749128541176,0.298695825212035));
#60481=DIRECTION('center_axis',(-0.491310548314114,0.286360316256975,0.822564109591763));
#60482=DIRECTION('ref_axis',(-0.868243142124459,-0.0861536225152698,-0.488601473065055));
#60483=DIRECTION('center_axis',(0.491310548314114,-0.286360316256975,-0.822564109591763));
#60484=DIRECTION('ref_axis',(0.870984468928858,0.161531977910744,0.463997279083572));
#60485=DIRECTION('',(-0.0570786439550532,-0.952962949154956,0.297663645650826));
#60486=DIRECTION('center_axis',(-0.313150259135956,0.30019266434088,0.901011253802641));
#60487=DIRECTION('ref_axis',(-0.948683298050514,-0.0549123752965086,-0.311423555691113));
#60488=DIRECTION('center_axis',(0.313150259135956,-0.30019266434088,-0.901011253802641));
#60489=DIRECTION('ref_axis',(0.949703593340092,0.0989839475056046,0.297094703643677));
#60490=DIRECTION('',(-0.0225789275220273,-0.950814057294297,0.308938214670041));
#60491=DIRECTION('center_axis',(0.,0.309016994374948,0.951056516295154));
#60492=DIRECTION('ref_axis',(-1.,0.,0.));
#60493=DIRECTION('',(-1.,0.,0.));
#60494=DIRECTION('',(0.0225789275220281,-0.950814057294297,0.308938214670041));
#60495=DIRECTION('center_axis',(0.313150259135957,0.30019266434088,0.901011253802641));
#60496=DIRECTION('ref_axis',(-0.948683298050513,0.0549123752965088,0.311423555691114));
#60497=DIRECTION('center_axis',(-0.313150259135957,-0.30019266434088,-0.901011253802641));
#60498=DIRECTION('ref_axis',(-0.949703593340092,0.098983947505605,0.297094703643678));
#60499=DIRECTION('',(0.0570786439550534,-0.952962949154956,0.297663645650826));
#60500=DIRECTION('center_axis',(0.491310548314113,0.286360316256975,0.822564109591764));
#60501=DIRECTION('ref_axis',(-0.86824314212446,0.0861536225152695,0.488601473065054));
#60502=DIRECTION('center_axis',(-0.491310548314113,-0.286360316256975,-0.822564109591764));
#60503=DIRECTION('ref_axis',(-0.870984468928858,0.161531977910744,0.463997279083571));
#60504=DIRECTION('',(0.0552259184163649,-0.952749128541176,0.298695825212034));
#60505=DIRECTION('center_axis',(0.284551435696759,0.301764876373726,0.909927711321105));
#60506=DIRECTION('ref_axis',(-0.957826285221151,0.0498974366850416,0.282982425517402));
#60507=DIRECTION('center_axis',(-0.284551435696759,-0.301764876373726,-0.909927711321105));
#60508=DIRECTION('ref_axis',(-0.958660774436356,0.0895703997751285,0.270086399215529));
#60509=DIRECTION('',(0.016150378482405,-0.950539749516609,0.310182768482998));
#60510=DIRECTION('center_axis',(-0.0617712249622997,0.308682119187541,0.949157344732972));
#60511=DIRECTION('ref_axis',(-0.998052578482889,-0.0108318757168334,-0.0614306198252359));
#60512=DIRECTION('center_axis',(0.0617712249622997,-0.308682119187541,-0.949157344732972));
#60513=DIRECTION('ref_axis',(0.998090334472114,0.0191041551727458,0.0587427909490066));
#60514=DIRECTION('',(-0.137998583506848,-0.944481249352984,0.298180416142191));
#60515=DIRECTION('center_axis',(-0.99026806874157,0.137058748836224,-0.0241671553619712));
#60516=DIRECTION('ref_axis',(0.,-0.173648177666931,-0.984807753012208));
#60517=DIRECTION('center_axis',(0.99026806874157,-0.137058748836224,0.0241671553619712));
#60518=DIRECTION('ref_axis',(0.139173100960066,0.975223671657125,-0.171958245538724));
#60519=DIRECTION('',(-0.137844537491629,-0.941977614300068,0.306067080296576));
#60520=DIRECTION('center_axis',(0.,0.309016994374948,0.951056516295154));
#60521=DIRECTION('ref_axis',(-1.,0.,0.));
#60522=DIRECTION('',(-1.,0.,0.));
#60523=DIRECTION('center_axis',(0.,-0.984807753012208,0.173648177666931));
#60524=DIRECTION('ref_axis',(1.,0.,0.));
#60525=DIRECTION('center_axis',(1.,0.,0.));
#60526=DIRECTION('ref_axis',(0.,1.,0.));
#60527=DIRECTION('center_axis',(1.,0.,0.));
#60528=DIRECTION('ref_axis',(0.,0.,-1.));
#60529=DIRECTION('center_axis',(0.64930555798837,0.124943459173594,0.75019425775938));
#60530=DIRECTION('ref_axis',(-0.760527640763576,0.106671313608347,0.640483363162275));
#60531=DIRECTION('',(1.,0.,0.));
#60532=DIRECTION('center_axis',(-0.99026806874157,-0.130779935984066,0.0476000039374394));
#60533=DIRECTION('ref_axis',(-0.139173100960065,0.930547596796367,-0.338691626801824));
#60534=DIRECTION('center_axis',(-0.0617712249622996,0.20725211545606,0.976335432321108));
#60535=DIRECTION('ref_axis',(0.998090334472114,0.0128267117770656,0.0604248268374111));
#60536=DIRECTION('center_axis',(0.284551435696759,0.193627806751035,0.938902951798373));
#60537=DIRECTION('ref_axis',(-0.958660774436356,0.0574729579753755,0.278686882824878));
#60538=DIRECTION('center_axis',(0.491310548314114,0.163286746281596,0.855541573276281));
#60539=DIRECTION('ref_axis',(-0.870984468928858,0.0921078431475353,0.482599419928604));
#60540=DIRECTION('center_axis',(0.313150259135956,0.190531153552384,0.930394967059196));
#60541=DIRECTION('ref_axis',(-0.949703593340092,0.0628247387151196,0.306783534438036));
#60542=DIRECTION('',(1.,0.,0.));
#60543=DIRECTION('center_axis',(-0.313150259135957,0.190531153552383,0.930394967059195));
#60544=DIRECTION('ref_axis',(0.949703593340092,0.0628247387151198,0.306783534438036));
#60545=DIRECTION('center_axis',(-0.491310548314113,0.163286746281596,0.855541573276282));
#60546=DIRECTION('ref_axis',(0.870984468928858,0.092107843147535,0.482599419928602));
#60547=DIRECTION('center_axis',(-0.284551435696759,0.193627806751035,0.938902951798373));
#60548=DIRECTION('ref_axis',(0.958660774436356,0.0574729579753754,0.278686882824878));
#60549=DIRECTION('center_axis',(0.0617712249622997,0.20725211545606,0.976335432321108));
#60550=DIRECTION('ref_axis',(-0.998090334472114,0.0128267117770656,0.0604248268374112));
#60551=DIRECTION('center_axis',(0.99026806874157,-0.130779935984066,0.0476000039374395));
#60552=DIRECTION('ref_axis',(0.139173100960066,0.930547596796366,-0.338691626801825));
#60553=DIRECTION('',(1.,0.,0.));
#60554=DIRECTION('center_axis',(0.,-0.207911690817759,-0.978147600733806));
#60555=DIRECTION('ref_axis',(1.,0.,0.));
#60556=DIRECTION('',(-0.137844537491629,-0.968810083928407,0.205926940351068));
#60557=DIRECTION('center_axis',(-0.99026806874157,0.130779935984066,-0.0476000039374395));
#60558=DIRECTION('ref_axis',(0.,-0.342020143325669,-0.939692620785908));
#60559=DIRECTION('',(-0.137998583506848,-0.967034963408845,0.214008809386339));
#60560=DIRECTION('center_axis',(-0.0617712249622997,-0.20725211545606,-0.976335432321108));
#60561=DIRECTION('ref_axis',(0.998052578482889,-0.0213346303712044,-0.058616415197295));
#60562=DIRECTION('',(0.0161503784824051,-0.978282954629779,0.206643717435842));
#60563=DIRECTION('center_axis',(0.284551435696759,-0.193627806751035,-0.938902951798373));
#60564=DIRECTION('ref_axis',(0.957826285221151,0.0982787650057294,0.270018687665128));
#60565=DIRECTION('',(0.0552259184163645,-0.974452861356161,0.217696391632611));
#60566=DIRECTION('center_axis',(0.491310548314113,-0.163286746281596,-0.855541573276282));
#60567=DIRECTION('ref_axis',(0.86824314212446,0.169689510806249,0.46621809925847));
#60568=DIRECTION('',(0.057078643955053,-0.974121945658943,0.218697195660774));
#60569=DIRECTION('center_axis',(0.313150259135957,-0.190531153552383,-0.930394967059195));
#60570=DIRECTION('ref_axis',(0.948683298050513,0.108156265856636,0.297156898213637));
#60571=DIRECTION('',(0.0225789275220278,-0.977898235227234,0.207858686543084));
#60572=DIRECTION('center_axis',(0.,-0.20791169081776,-0.978147600733806));
#60573=DIRECTION('ref_axis',(1.,0.,0.));
#60574=DIRECTION('',(-0.0225789275220274,-0.977898235227234,0.207858686543084));
#60575=DIRECTION('center_axis',(-0.313150259135956,-0.190531153552384,-0.930394967059196));
#60576=DIRECTION('ref_axis',(0.948683298050514,-0.108156265856635,-0.297156898213636));
#60577=DIRECTION('',(-0.0570786439550527,-0.974121945658943,0.218697195660774));
#60578=DIRECTION('center_axis',(-0.491310548314114,-0.163286746281596,-0.855541573276281));
#60579=DIRECTION('ref_axis',(0.868243142124459,-0.169689510806249,-0.466218099258471));
#60580=DIRECTION('',(-0.0552259184163635,-0.974452861356161,0.21769639163261));
#60581=DIRECTION('center_axis',(-0.284551435696759,-0.193627806751035,-0.938902951798373));
#60582=DIRECTION('ref_axis',(0.957826285221151,-0.0982787650057296,-0.270018687665129));
#60583=DIRECTION('',(-0.0161503784824052,-0.978282954629779,0.206643717435842));
#60584=DIRECTION('center_axis',(0.0617712249622996,-0.20725211545606,-0.976335432321108));
#60585=DIRECTION('ref_axis',(0.998052578482889,0.0213346303712044,0.0586164151972949));
#60586=DIRECTION('',(0.137998583506848,-0.967034963408845,0.214008809386339));
#60587=DIRECTION('center_axis',(0.99026806874157,0.130779935984066,-0.0476000039374394));
#60588=DIRECTION('ref_axis',(0.,0.342020143325669,0.939692620785908));
#60589=DIRECTION('',(0.137844537491629,-0.968810083928407,0.205926940351068));
#60590=DIRECTION('center_axis',(0.,-0.20791169081776,-0.978147600733806));
#60591=DIRECTION('ref_axis',(1.,0.,0.));
#60592=DIRECTION('',(-0.0519254248777279,-0.976828045559515,0.207631210706978));
#60593=DIRECTION('center_axis',(-0.64930555798837,-0.124943459173594,-0.75019425775938));
#60594=DIRECTION('ref_axis',(0.755033118392644,-0.224258043872452,-0.616143911670627));
#60595=DIRECTION('center_axis',(0.,0.469471562785891,0.882947592858927));
#60596=DIRECTION('ref_axis',(-1.,0.,0.));
#60597=DIRECTION('',(-1.,0.,0.));
#60598=DIRECTION('',(0.137844537491629,-0.874518866989312,0.464989929744128));
#60599=DIRECTION('center_axis',(0.99026806874157,0.130779935984066,-0.0476000039374394));
#60600=DIRECTION('ref_axis',(0.,0.342020143325669,0.939692620785908));
#60601=DIRECTION('center_axis',(-0.99026806874157,-0.130779935984066,0.0476000039374394));
#60602=DIRECTION('ref_axis',(-0.139173100960065,0.930547596796367,-0.338691626801824));
#60603=DIRECTION('',(0.137998583506848,-0.878353971058417,0.457657833403968));
#60604=DIRECTION('center_axis',(0.0617712249622996,0.468811987424192,0.881135424446229));
#60605=DIRECTION('ref_axis',(-0.998052578482889,0.0213346303712044,0.0586164151972949));
#60606=DIRECTION('center_axis',(-0.0617712249622996,-0.468811987424192,
-0.881135424446229));
#60607=DIRECTION('ref_axis',(-0.998090334472114,0.0290144987282327,0.0545329542285434));
#60608=DIRECTION('',(-0.0161503784824054,-0.882236242379483,0.470529890556386));
#60609=DIRECTION('center_axis',(-0.284551435696759,0.455187678719167,0.843702943923494));
#60610=DIRECTION('ref_axis',(-0.957826285221151,-0.0982787650057296,-0.270018687665129));
#60611=DIRECTION('center_axis',(0.284551435696759,-0.455187678719167,-0.843702943923494));
#60612=DIRECTION('ref_axis',(0.958660774436356,0.135109635175349,0.250429443236754));
#60613=DIRECTION('',(-0.0552259184163638,-0.886406742738186,0.459601114406122));
#60614=DIRECTION('center_axis',(-0.491310548314114,0.424846618249727,0.760341565401402));
#60615=DIRECTION('ref_axis',(-0.868243142124459,-0.169689510806249,-0.466218099258471));
#60616=DIRECTION('center_axis',(0.491310548314114,-0.424846618249727,-0.760341565401402));
#60617=DIRECTION('ref_axis',(0.870984468928858,0.239650226161174,0.428898384218936));
#60618=DIRECTION('',(-0.0570786439550532,-0.886796551036219,0.458621745531673));
#60619=DIRECTION('center_axis',(-0.313150259135956,0.452091025520515,0.835194959184317));
#60620=DIRECTION('ref_axis',(-0.948683298050514,-0.108156265856635,-0.297156898213636));
#60621=DIRECTION('center_axis',(0.313150259135956,-0.452091025520515,-0.835194959184317));
#60622=DIRECTION('ref_axis',(0.949703593340092,0.149070112809494,0.27539278542453));
#60623=DIRECTION('',(-0.0225789275220273,-0.88272249730729,0.469351877358061));
#60624=DIRECTION('center_axis',(0.,0.469471562785891,0.882947592858927));
#60625=DIRECTION('ref_axis',(-1.,0.,0.));
#60626=DIRECTION('',(-1.,0.,0.));
#60627=DIRECTION('',(0.0225789275220281,-0.88272249730729,0.469351877358061));
#60628=DIRECTION('center_axis',(0.313150259135957,0.452091025520515,0.835194959184317));
#60629=DIRECTION('ref_axis',(-0.948683298050513,0.108156265856636,0.297156898213637));
#60630=DIRECTION('center_axis',(-0.313150259135957,-0.452091025520515,-0.835194959184317));
#60631=DIRECTION('ref_axis',(-0.949703593340092,0.149070112809494,0.275392785424531));
#60632=DIRECTION('',(0.0570786439550533,-0.886796551036219,0.458621745531673));
#60633=DIRECTION('center_axis',(0.491310548314113,0.424846618249728,0.760341565401403));
#60634=DIRECTION('ref_axis',(-0.86824314212446,0.169689510806249,0.46621809925847));
#60635=DIRECTION('center_axis',(-0.491310548314113,-0.424846618249728,-0.760341565401403));
#60636=DIRECTION('ref_axis',(-0.870984468928858,0.239650226161173,0.428898384218935));
#60637=DIRECTION('',(0.0552259184163649,-0.886406742738186,0.459601114406122));
#60638=DIRECTION('center_axis',(0.284551435696759,0.455187678719167,0.843702943923494));
#60639=DIRECTION('ref_axis',(-0.957826285221151,0.0982787650057294,0.270018687665128));
#60640=DIRECTION('center_axis',(-0.284551435696759,-0.455187678719167,-0.843702943923494));
#60641=DIRECTION('ref_axis',(-0.958660774436356,0.135109635175349,0.250429443236754));
#60642=DIRECTION('',(0.0161503784824051,-0.882236242379483,0.470529890556386));
#60643=DIRECTION('center_axis',(-0.0617712249622997,0.468811987424192,0.881135424446229));
#60644=DIRECTION('ref_axis',(-0.998052578482889,-0.0213346303712044,-0.058616415197295));
#60645=DIRECTION('center_axis',(0.0617712249622997,-0.468811987424192,-0.881135424446229));
#60646=DIRECTION('ref_axis',(0.998090334472114,0.0290144987282327,0.0545329542285434));
#60647=DIRECTION('',(-0.137998583506848,-0.878353971058417,0.457657833403968));
#60648=DIRECTION('center_axis',(-0.99026806874157,0.130779935984066,-0.0476000039374395));
#60649=DIRECTION('ref_axis',(0.,-0.342020143325669,-0.939692620785908));
#60650=DIRECTION('center_axis',(0.99026806874157,-0.130779935984066,0.0476000039374395));
#60651=DIRECTION('ref_axis',(0.139173100960066,0.930547596796366,-0.338691626801825));
#60652=DIRECTION('',(-0.137844537491629,-0.874518866989312,0.464989929744128));
#60653=DIRECTION('center_axis',(0.,0.469471562785891,0.882947592858927));
#60654=DIRECTION('ref_axis',(-1.,0.,0.));
#60655=DIRECTION('',(-1.,0.,0.));
#60656=DIRECTION('center_axis',(0.,-0.939692620785908,0.342020143325669));
#60657=DIRECTION('ref_axis',(1.,0.,0.));
#60658=DIRECTION('center_axis',(1.,0.,0.));
#60659=DIRECTION('ref_axis',(0.,1.,0.));
#60660=DIRECTION('center_axis',(1.,0.,0.));
#60661=DIRECTION('ref_axis',(0.,0.,-1.));
#60662=DIRECTION('center_axis',(0.64930555798837,0.253315153038431,0.717100917309779));
#60663=DIRECTION('ref_axis',(-0.760527640763576,0.216269505504612,0.612229702500115));
#60664=DIRECTION('',(1.,0.,0.));
#60665=DIRECTION('center_axis',(-0.99026806874157,-0.120527440954873,0.0695865504800327));
#60666=DIRECTION('ref_axis',(-0.139173100960065,0.857597304086756,-0.495134034370783));
#60667=DIRECTION('center_axis',(-0.0617712249622996,0.373642358743524,0.925513751123792));
#60668=DIRECTION('ref_axis',(0.998090334472114,0.0231245062698634,0.0572795028183562));
#60669=DIRECTION('center_axis',(0.284551435696759,0.353724951873058,0.891015790469123));
#60670=DIRECTION('ref_axis',(-0.958660774436356,0.104993283944912,0.264472928451193));
#60671=DIRECTION('center_axis',(0.491310548314114,0.309369288819977,0.814189528457782));
#60672=DIRECTION('ref_axis',(-0.870984468928858,0.174511027858645,0.459273291233482));
#60673=DIRECTION('center_axis',(0.313150259135956,0.34919794774906,0.883174789320284));
#60674=DIRECTION('ref_axis',(-0.949703593340092,0.115142691461001,0.291213401820784));
#60675=DIRECTION('',(1.,0.,0.));
#60676=DIRECTION('center_axis',(-0.313150259135957,0.349197947749059,0.883174789320284));
#60677=DIRECTION('ref_axis',(0.949703593340092,0.115142691461001,0.291213401820785));
#60678=DIRECTION('center_axis',(-0.491310548314113,0.309369288819978,0.814189528457783));
#60679=DIRECTION('ref_axis',(0.870984468928858,0.174511027858644,0.459273291233481));
#60680=DIRECTION('center_axis',(-0.284551435696759,0.353724951873058,0.891015790469123));
#60681=DIRECTION('ref_axis',(0.958660774436356,0.104993283944912,0.264472928451193));
#60682=DIRECTION('center_axis',(0.0617712249622997,0.373642358743524,0.925513751123792));
#60683=DIRECTION('ref_axis',(-0.998090334472114,0.0231245062698634,0.0572795028183563));
#60684=DIRECTION('center_axis',(0.99026806874157,-0.120527440954873,0.0695865504800329));
#60685=DIRECTION('ref_axis',(0.139173100960066,0.857597304086755,-0.495134034370784));
#60686=DIRECTION('',(1.,0.,0.));
#60687=DIRECTION('center_axis',(0.,-0.374606593415912,-0.927183854566788));
#60688=DIRECTION('ref_axis',(1.,0.,0.));
#60689=DIRECTION('',(-0.137844537491629,-0.918332843924614,0.371030552991327));
#60690=DIRECTION('center_axis',(-0.99026806874157,0.120527440954873,-0.0695865504800329));
#60691=DIRECTION('ref_axis',(0.,-0.5,-0.866025403784439));
#60692=DIRECTION('',(-0.137998583506848,-0.9151812896443,0.378681393832731));
#60693=DIRECTION('center_axis',(-0.0617712249622997,-0.373642358743524,
-0.925513751123792));
#60694=DIRECTION('ref_axis',(0.998052578482889,-0.0311891430775903,-0.0540211804549215));
#60695=DIRECTION('',(0.0161503784824051,-0.927537333400043,0.373381387356163));
#60696=DIRECTION('center_axis',(0.284551435696759,-0.353724951873058,-0.891015790469123));
#60697=DIRECTION('ref_axis',(0.957826285221151,0.143673942783173,0.248850568624199));
#60698=DIRECTION('',(0.0552259184163645,-0.921846151116809,0.3836010578794));
#60699=DIRECTION('center_axis',(0.491310548314113,-0.309369288819978,-0.814189528457783));
#60700=DIRECTION('ref_axis',(0.86824314212446,0.248069469178416,0.429668924423658));
#60701=DIRECTION('',(0.057078643955053,-0.921346474976903,0.384529194537798));
#60702=DIRECTION('center_axis',(0.313150259135957,-0.349197947749059,-0.883174789320284));
#60703=DIRECTION('ref_axis',(0.948683298050513,0.15811388300842,0.273861278752585));
#60704=DIRECTION('',(0.0225789275220278,-0.926947481578288,0.374511092529479));
#60705=DIRECTION('center_axis',(0.,-0.374606593415912,-0.927183854566788));
#60706=DIRECTION('ref_axis',(1.,0.,0.));
#60707=DIRECTION('',(-0.0225789275220274,-0.926947481578288,0.374511092529479));
#60708=DIRECTION('center_axis',(-0.313150259135956,-0.34919794774906,-0.883174789320284));
#60709=DIRECTION('ref_axis',(0.948683298050514,-0.158113883008419,-0.273861278752584));
#60710=DIRECTION('',(-0.0570786439550527,-0.921346474976903,0.384529194537798));
#60711=DIRECTION('center_axis',(-0.491310548314114,-0.309369288819977,-0.814189528457782));
#60712=DIRECTION('ref_axis',(0.868243142124459,-0.248069469178417,-0.429668924423659));
#60713=DIRECTION('',(-0.0552259184163635,-0.921846151116809,0.3836010578794));
#60714=DIRECTION('center_axis',(-0.284551435696759,-0.353724951873058,-0.891015790469123));
#60715=DIRECTION('ref_axis',(0.957826285221151,-0.143673942783173,-0.248850568624199));
#60716=DIRECTION('',(-0.0161503784824052,-0.927537333400043,0.373381387356162));
#60717=DIRECTION('center_axis',(0.0617712249622996,-0.373642358743524,-0.925513751123792));
#60718=DIRECTION('ref_axis',(0.998052578482889,0.0311891430775903,0.0540211804549215));
#60719=DIRECTION('',(0.137998583506848,-0.9151812896443,0.378681393832731));
#60720=DIRECTION('center_axis',(0.99026806874157,0.120527440954873,-0.0695865504800327));
#60721=DIRECTION('ref_axis',(0.,0.5,0.866025403784439));
#60722=DIRECTION('',(0.137844537491629,-0.918332843924614,0.371030552991328));
#60723=DIRECTION('center_axis',(0.,-0.374606593415912,-0.927183854566787));
#60724=DIRECTION('ref_axis',(1.,0.,0.));
#60725=DIRECTION('',(-0.051925424877728,-0.925933051260728,0.374101236076902));
#60726=DIRECTION('center_axis',(-0.64930555798837,-0.253315153038431,-0.717100917309779));
#60727=DIRECTION('ref_axis',(0.755033118392644,-0.327843327723121,-0.567841300538901));
#60728=DIRECTION('center_axis',(0.,0.615661475325658,0.788010753606722));
#60729=DIRECTION('ref_axis',(-1.,0.,0.));
#60730=DIRECTION('',(-1.,0.,0.));
#60731=DIRECTION('',(0.137844537491629,-0.780488306432985,0.609784295472661));
#60732=DIRECTION('center_axis',(0.99026806874157,0.120527440954873,-0.0695865504800327));
#60733=DIRECTION('ref_axis',(0.,0.5,0.866025403784439));
#60734=DIRECTION('center_axis',(-0.99026806874157,-0.120527440954873,0.0695865504800327));
#60735=DIRECTION('ref_axis',(-0.139173100960065,0.857597304086756,-0.495134034370783));
#60736=DIRECTION('',(0.137998583506848,-0.785538351821795,0.603229548983803));
#60737=DIRECTION('center_axis',(0.0617712249622996,0.61469724065327,0.786340650163727));
#60738=DIRECTION('ref_axis',(-0.998052578482889,0.0311891430775903,0.0540211804549215));
#60739=DIRECTION('center_axis',(-0.0617712249622996,-0.61469724065327,-0.786340650163727));
#60740=DIRECTION('ref_axis',(-0.998090334472114,0.0380432514219071,0.0486661612888524));
#60741=DIRECTION('',(-0.0161503784824054,-0.787126433450736,0.616580200004832));
#60742=DIRECTION('center_axis',(-0.284551435696759,0.594779833782804,0.751842689509058));
#60743=DIRECTION('ref_axis',(-0.957826285221151,-0.143673942783173,-0.248850568624199));
#60744=DIRECTION('center_axis',(0.284551435696759,-0.594779833782804,-0.751842689509058));
#60745=DIRECTION('ref_axis',(0.958660774436356,0.176543632679541,0.223163315348643));
#60746=DIRECTION('',(-0.0552259184163638,-0.793131336600549,0.606541656308365));
#60747=DIRECTION('center_axis',(-0.491310548314114,0.550424170729724,0.675016427497717));
#60748=DIRECTION('ref_axis',(-0.868243142124459,-0.248069469178417,-0.429668924423659));
#60749=DIRECTION('center_axis',(0.491310548314114,-0.550424170729724,-0.675016427497717));
#60750=DIRECTION('ref_axis',(0.870984468928858,0.310486823558562,0.380767628982861));
#60751=DIRECTION('',(-0.0570786439550532,-0.793685288454953,0.605644855748342));
#60752=DIRECTION('center_axis',(-0.313150259135956,0.590252829658806,0.744001688360219));
#60753=DIRECTION('ref_axis',(-0.948683298050514,-0.158113883008419,-0.273861278752584));
#60754=DIRECTION('center_axis',(0.313150259135956,-0.590252829658806,-0.744001688360219));
#60755=DIRECTION('ref_axis',(0.949703593340092,0.194626858168784,0.245323196775732));
#60756=DIRECTION('',(-0.0225789275220273,-0.787809860918738,0.615504520756066));
#60757=DIRECTION('center_axis',(0.,0.615661475325658,0.788010753606722));
#60758=DIRECTION('ref_axis',(-1.,0.,0.));
#60759=DIRECTION('',(-1.,0.,0.));
#60760=DIRECTION('',(0.0225789275220281,-0.787809860918738,0.615504520756066));
#60761=DIRECTION('center_axis',(0.313150259135957,0.590252829658806,0.744001688360219));
#60762=DIRECTION('ref_axis',(-0.948683298050513,0.15811388300842,0.273861278752585));
#60763=DIRECTION('center_axis',(-0.313150259135957,-0.590252829658806,-0.744001688360219));
#60764=DIRECTION('ref_axis',(-0.949703593340092,0.194626858168784,0.245323196775733));
#60765=DIRECTION('',(0.0570786439550533,-0.793685288454953,0.605644855748342));
#60766=DIRECTION('center_axis',(0.491310548314113,0.550424170729724,0.675016427497717));
#60767=DIRECTION('ref_axis',(-0.86824314212446,0.248069469178416,0.429668924423658));
#60768=DIRECTION('center_axis',(-0.491310548314113,-0.550424170729724,-0.675016427497717));
#60769=DIRECTION('ref_axis',(-0.870984468928858,0.310486823558561,0.38076762898286));
#60770=DIRECTION('',(0.0552259184163649,-0.79313133660055,0.606541656308365));
#60771=DIRECTION('center_axis',(0.284551435696759,0.594779833782804,0.751842689509058));
#60772=DIRECTION('ref_axis',(-0.957826285221151,0.143673942783173,0.248850568624199));
#60773=DIRECTION('center_axis',(-0.284551435696759,-0.594779833782804,-0.751842689509058));
#60774=DIRECTION('ref_axis',(-0.958660774436356,0.176543632679541,0.223163315348643));
#60775=DIRECTION('',(0.016150378482405,-0.787126433450736,0.616580200004832));
#60776=DIRECTION('center_axis',(-0.0617712249622997,0.61469724065327,0.786340650163727));
#60777=DIRECTION('ref_axis',(-0.998052578482889,-0.0311891430775903,-0.0540211804549215));
#60778=DIRECTION('center_axis',(0.0617712249622997,-0.61469724065327,-0.786340650163727));
#60779=DIRECTION('ref_axis',(0.998090334472114,0.0380432514219071,0.0486661612888524));
#60780=DIRECTION('',(-0.137998583506848,-0.785538351821795,0.603229548983803));
#60781=DIRECTION('center_axis',(-0.99026806874157,0.120527440954873,-0.0695865504800329));
#60782=DIRECTION('ref_axis',(0.,-0.5,-0.866025403784439));
#60783=DIRECTION('center_axis',(0.99026806874157,-0.120527440954873,0.0695865504800329));
#60784=DIRECTION('ref_axis',(0.139173100960066,0.857597304086755,-0.495134034370784));
#60785=DIRECTION('',(-0.137844537491629,-0.780488306432985,0.609784295472661));
#60786=DIRECTION('center_axis',(0.,0.615661475325658,0.788010753606722));
#60787=DIRECTION('ref_axis',(-1.,0.,0.));
#60788=DIRECTION('',(-1.,0.,0.));
#60789=DIRECTION('center_axis',(0.,-0.866025403784439,0.5));
#60790=DIRECTION('ref_axis',(1.,0.,0.));
#60791=DIRECTION('center_axis',(1.,0.,0.));
#60792=DIRECTION('ref_axis',(0.,1.,0.));
#60793=DIRECTION('center_axis',(1.,0.,0.));
#60794=DIRECTION('ref_axis',(0.,0.,-1.));
#60795=DIRECTION('center_axis',(0.64930555798837,0.373989994161848,0.662218828358294));
#60796=DIRECTION('ref_axis',(-0.760527640763576,0.319296457913771,0.565373752130667));
#60797=DIRECTION('',(1.,0.,0.));
#60798=DIRECTION('center_axis',(-0.99026806874157,-0.106612780622095,0.0894587448987839));
#60799=DIRECTION('ref_axis',(-0.139173100960065,0.758589351257639,-0.636532044855303));
#60800=DIRECTION('center_axis',(-0.0617712249622996,0.528679668032723,0.846570802931135));
#60801=DIRECTION('ref_axis',(0.998090334472114,0.0327196743412163,0.0523937700909925));
#60802=DIRECTION('center_axis',(0.284551435696759,0.50307434332588,0.816055565222214));
#60803=DIRECTION('ref_axis',(-0.958660774436356,0.149323442110948,0.242223097976277));
#60804=DIRECTION('center_axis',(0.491310548314114,0.446051802065978,0.748098746816874));
#60805=DIRECTION('ref_axis',(-0.870984468928858,0.25161178329511,0.42199237598773));
#60806=DIRECTION('center_axis',(0.313150259135956,0.497254539006069,0.809119792515883));
#60807=DIRECTION('ref_axis',(-0.949703593340092,0.163962091791853,0.266794897350299));
#60808=DIRECTION('',(1.,0.,0.));
#60809=DIRECTION('center_axis',(-0.313150259135957,0.497254539006068,0.809119792515883));
#60810=DIRECTION('ref_axis',(0.949703593340092,0.163962091791853,0.2667948973503));
#60811=DIRECTION('center_axis',(-0.491310548314113,0.446051802065979,0.748098746816875));
#60812=DIRECTION('ref_axis',(0.870984468928858,0.25161178329511,0.421992375987729));
#60813=DIRECTION('center_axis',(-0.284551435696759,0.503074343325881,0.816055565222214));
#60814=DIRECTION('ref_axis',(0.958660774436356,0.149323442110948,0.242223097976277));
#60815=DIRECTION('center_axis',(0.0617712249622997,0.528679668032723,0.846570802931135));
#60816=DIRECTION('ref_axis',(-0.998090334472114,0.0327196743412163,0.0523937700909926));
#60817=DIRECTION('center_axis',(0.99026806874157,-0.106612780622095,0.0894587448987841));
#60818=DIRECTION('ref_axis',(0.139173100960066,0.758589351257642,-0.636532044855299));
#60819=DIRECTION('',(1.,0.,0.));
#60820=DIRECTION('center_axis',(0.,-0.529919264233205,-0.848048096156426));
#60821=DIRECTION('ref_axis',(1.,0.,0.));
#60822=DIRECTION('',(-0.137844537491629,-0.839952525157012,0.524860590029465));
#60823=DIRECTION('center_axis',(-0.99026806874157,0.106612780622095,-0.0894587448987841));
#60824=DIRECTION('ref_axis',(0.,-0.642787609686539,-0.766044443118978));
#60825=DIRECTION('',(-0.137998583506848,-0.835520295497991,0.531847935749547));
#60826=DIRECTION('center_axis',(-0.0617712249622997,-0.528679668032723,
-0.846570802931135));
#60827=DIRECTION('ref_axis',(0.998052578482889,-0.0400959894540315,-0.0477845394804615));
#60828=DIRECTION('',(0.0161503784824051,-0.848608959651484,0.528774052761765));
#60829=DIRECTION('center_axis',(0.284551435696759,-0.503074343325881,-0.816055565222214));
#60830=DIRECTION('ref_axis',(0.957826285221151,0.184703660511672,0.220121250980087));
#60831=DIRECTION('',(0.0552259184163645,-0.841229612052432,0.537850200094026));
#60832=DIRECTION('center_axis',(0.491310548314113,-0.446051802065979,-0.748098746816875));
#60833=DIRECTION('ref_axis',(0.86824314212446,0.318911962258805,0.3800644767432));
#60834=DIRECTION('',(0.057078643955053,-0.840576357876501,0.538677468419953));
#60835=DIRECTION('center_axis',(0.313150259135957,-0.497254539006068,-0.809119792515883));
#60836=DIRECTION('ref_axis',(0.948683298050513,0.203267289834479,0.242244522917128));
#60837=DIRECTION('',(0.0225789275220278,-0.847831897759644,0.529784168481124));
#60838=DIRECTION('center_axis',(0.,-0.529919264233205,-0.848048096156426));
#60839=DIRECTION('ref_axis',(1.,0.,0.));
#60840=DIRECTION('',(-0.0225789275220274,-0.847831897759644,0.529784168481124));
#60841=DIRECTION('center_axis',(-0.313150259135956,-0.497254539006069,-0.809119792515883));
#60842=DIRECTION('ref_axis',(0.948683298050514,-0.203267289834478,-0.242244522917128));
#60843=DIRECTION('',(-0.0570786439550527,-0.840576357876501,0.538677468419953));
#60844=DIRECTION('center_axis',(-0.491310548314114,-0.446051802065978,-0.748098746816874));
#60845=DIRECTION('ref_axis',(0.868243142124459,-0.318911962258806,-0.380064476743201));
#60846=DIRECTION('',(-0.0552259184163635,-0.841229612052433,0.537850200094025));
#60847=DIRECTION('center_axis',(-0.284551435696759,-0.50307434332588,-0.816055565222214));
#60848=DIRECTION('ref_axis',(0.957826285221151,-0.184703660511673,-0.220121250980087));
#60849=DIRECTION('',(-0.0161503784824052,-0.848608959651484,0.528774052761765));
#60850=DIRECTION('center_axis',(0.0617712249622996,-0.528679668032723,-0.846570802931135));
#60851=DIRECTION('ref_axis',(0.998052578482889,0.0400959894540314,0.0477845394804615));
#60852=DIRECTION('',(0.137998583506848,-0.835520295497991,0.531847935749547));
#60853=DIRECTION('center_axis',(0.99026806874157,0.106612780622095,-0.0894587448987839));
#60854=DIRECTION('ref_axis',(0.,0.642787609686539,0.766044443118978));
#60855=DIRECTION('',(0.137844537491629,-0.839952525157012,0.524860590029465));
#60856=DIRECTION('center_axis',(0.,-0.529919264233205,-0.848048096156426));
#60857=DIRECTION('ref_axis',(1.,0.,0.));
#60858=DIRECTION('',(-0.051925424877728,-0.846904049744114,0.52920438469299));
#60859=DIRECTION('center_axis',(-0.64930555798837,-0.373989994161848,-0.662218828358294));
#60860=DIRECTION('ref_axis',(0.755033118392644,-0.421467257957652,-0.502285118831862));
#60861=DIRECTION('center_axis',(0.,0.743144825477394,0.669130606358858));
#60862=DIRECTION('ref_axis',(-1.,0.,0.));
#60863=DIRECTION('',(-1.,0.,0.));
#60864=DIRECTION('',(0.137844537491629,-0.662743003631831,0.736050673949001));
#60865=DIRECTION('center_axis',(0.99026806874157,0.106612780622095,-0.0894587448987839));
#60866=DIRECTION('ref_axis',(0.,0.642787609686539,0.766044443118978));
#60867=DIRECTION('center_axis',(-0.99026806874157,-0.106612780622095,0.0894587448987839));
#60868=DIRECTION('ref_axis',(-0.139173100960065,0.758589351257639,-0.636532044855303));
#60869=DIRECTION('',(0.137998583506848,-0.668854547266653,0.730472439966645));
#60870=DIRECTION('center_axis',(0.0617712249622996,0.741905229276912,0.667653313133567));
#60871=DIRECTION('ref_axis',(-0.998052578482889,0.0400959894540314,0.0477845394804615));
#60872=DIRECTION('center_axis',(-0.0617712249622996,-0.741905229276912,
-0.667653313133567));
#60873=DIRECTION('ref_axis',(-0.998090334472114,0.045916079171941,0.0413206716646654));
#60874=DIRECTION('',(-0.0161503784824054,-0.668100186146782,0.743896032080768));
#60875=DIRECTION('center_axis',(-0.284551435696759,0.71629990457007,0.637138075424646));
#60876=DIRECTION('ref_axis',(-0.957826285221151,-0.184703660511673,-0.220121250980087));
#60877=DIRECTION('center_axis',(0.284551435696759,-0.71629990457007,-0.637138075424646));
#60878=DIRECTION('ref_axis',(0.958660774436356,0.212613441240154,0.18911648304975));
#60879=DIRECTION('',(-0.0552259184163638,-0.675757036144127,0.735052736908566));
#60880=DIRECTION('center_axis',(-0.491310548314114,0.659277363310168,0.569181257019306));
#60881=DIRECTION('ref_axis',(-0.868243142124459,-0.318911962258806,-0.380064476743201));
#60882=DIRECTION('center_axis',(0.491310548314114,-0.659277363310168,-0.569181257019306));
#60883=DIRECTION('ref_axis',(0.870984468928858,0.371889435936037,0.32106744201786));
#60884=DIRECTION('',(-0.0570786439550532,-0.676458300008118,0.734265753494182));
#60885=DIRECTION('center_axis',(-0.313150259135956,0.710480100250258,0.630202302718315));
#60886=DIRECTION('ref_axis',(-0.948683298050514,-0.203267289834478,-0.242244522917128));
#60887=DIRECTION('center_axis',(0.313150259135956,-0.710480100250258,-0.630202302718315));
#60888=DIRECTION('ref_axis',(0.949703593340092,0.234269964928557,0.207799586932431));
#60889=DIRECTION('',(-0.0225789275220273,-0.668960020557194,0.742955370751214));
#60890=DIRECTION('center_axis',(0.,0.743144825477394,0.669130606358858));
#60891=DIRECTION('ref_axis',(-1.,0.,0.));
#60892=DIRECTION('',(-1.,0.,0.));
#60893=DIRECTION('',(0.0225789275220281,-0.668960020557194,0.742955370751214));
#60894=DIRECTION('center_axis',(0.313150259135957,0.710480100250258,0.630202302718315));
#60895=DIRECTION('ref_axis',(-0.948683298050513,0.203267289834479,0.242244522917128));
#60896=DIRECTION('center_axis',(-0.313150259135957,-0.710480100250258,-0.630202302718315));
#60897=DIRECTION('ref_axis',(-0.949703593340092,0.234269964928558,0.207799586932432));
#60898=DIRECTION('',(0.0570786439550534,-0.676458300008118,0.734265753494183));
#60899=DIRECTION('center_axis',(0.491310548314113,0.659277363310168,0.569181257019307));
#60900=DIRECTION('ref_axis',(-0.86824314212446,0.318911962258805,0.3800644767432));
#60901=DIRECTION('center_axis',(-0.491310548314113,-0.659277363310168,-0.569181257019307));
#60902=DIRECTION('ref_axis',(-0.870984468928858,0.371889435936036,0.321067442017859));
#60903=DIRECTION('',(0.0552259184163649,-0.675757036144127,0.735052736908566));
#60904=DIRECTION('center_axis',(0.284551435696759,0.71629990457007,0.637138075424647));
#60905=DIRECTION('ref_axis',(-0.957826285221151,0.184703660511672,0.220121250980087));
#60906=DIRECTION('center_axis',(-0.284551435696759,-0.71629990457007,-0.637138075424647));
#60907=DIRECTION('ref_axis',(-0.958660774436356,0.212613441240154,0.189116483049749));
#60908=DIRECTION('',(0.0161503784824051,-0.668100186146782,0.743896032080768));
#60909=DIRECTION('center_axis',(-0.0617712249622997,0.741905229276912,0.667653313133567));
#60910=DIRECTION('ref_axis',(-0.998052578482889,-0.0400959894540315,-0.0477845394804615));
#60911=DIRECTION('center_axis',(0.0617712249622997,-0.741905229276912,-0.667653313133567));
#60912=DIRECTION('ref_axis',(0.998090334472114,0.045916079171941,0.0413206716646654));
#60913=DIRECTION('',(-0.137998583506848,-0.668854547266653,0.730472439966645));
#60914=DIRECTION('center_axis',(-0.99026806874157,0.106612780622095,-0.0894587448987841));
#60915=DIRECTION('ref_axis',(0.,-0.642787609686539,-0.766044443118978));
#60916=DIRECTION('center_axis',(0.99026806874157,-0.106612780622095,0.0894587448987841));
#60917=DIRECTION('ref_axis',(0.139173100960066,0.758589351257642,-0.636532044855299));
#60918=DIRECTION('',(-0.137844537491629,-0.662743003631831,0.736050673949));
#60919=DIRECTION('center_axis',(0.,0.743144825477394,0.669130606358858));
#60920=DIRECTION('ref_axis',(-1.,0.,0.));
#60921=DIRECTION('',(-1.,0.,0.));
#60922=DIRECTION('center_axis',(0.,-0.766044443118978,0.642787609686539));
#60923=DIRECTION('ref_axis',(1.,0.,0.));
#60924=DIRECTION('center_axis',(1.,0.,0.));
#60925=DIRECTION('ref_axis',(0.,1.,0.));
#60926=DIRECTION('center_axis',(1.,0.,0.));
#60927=DIRECTION('ref_axis',(0.,0.,-1.));
#60928=DIRECTION('center_axis',(0.64930555798837,0.483301338560726,0.587215555406038));
#60929=DIRECTION('ref_axis',(-0.760527640763576,0.412621749021023,0.501339206395651));
#60930=DIRECTION('',(1.,0.,0.));
#60931=DIRECTION('center_axis',(-0.99026806874157,-0.0894587448987838,0.106612780622095));
#60932=DIRECTION('ref_axis',(-0.139173100960065,0.636532044855299,-0.758589351257642));
#60933=DIRECTION('center_axis',(-0.0617712249622996,0.667653313133567,0.741905229276912));
#60934=DIRECTION('ref_axis',(0.998090334472114,0.0413206716646654,0.045916079171941));
#60935=DIRECTION('center_axis',(0.284551435696759,0.637138075424646,0.71629990457007));
#60936=DIRECTION('ref_axis',(-0.958660774436356,0.18911648304975,0.212613441240154));
#60937=DIRECTION('center_axis',(0.491310548314114,0.569181257019307,0.659277363310167));
#60938=DIRECTION('ref_axis',(-0.870984468928858,0.32106744201786,0.371889435936037));
#60939=DIRECTION('center_axis',(0.313150259135956,0.630202302718315,0.710480100250258));
#60940=DIRECTION('ref_axis',(-0.949703593340092,0.207799586932431,0.234269964928557));
#60941=DIRECTION('',(1.,0.,0.));
#60942=DIRECTION('center_axis',(-0.313150259135957,0.630202302718315,0.710480100250258));
#60943=DIRECTION('ref_axis',(0.949703593340092,0.207799586932432,0.234269964928558));
#60944=DIRECTION('center_axis',(-0.491310548314113,0.569181257019307,0.659277363310168));
#60945=DIRECTION('ref_axis',(0.870984468928858,0.321067442017859,0.371889435936036));
#60946=DIRECTION('center_axis',(-0.284551435696759,0.637138075424647,0.71629990457007));
#60947=DIRECTION('ref_axis',(0.958660774436356,0.18911648304975,0.212613441240154));
#60948=DIRECTION('center_axis',(0.0617712249622997,0.667653313133568,0.741905229276912));
#60949=DIRECTION('ref_axis',(-0.998090334472114,0.0413206716646654,0.045916079171941));
#60950=DIRECTION('center_axis',(0.99026806874157,-0.0894587448987841,0.106612780622095));
#60951=DIRECTION('ref_axis',(0.139173100960066,0.636532044855299,-0.758589351257642));
#60952=DIRECTION('',(1.,0.,0.));
#60953=DIRECTION('center_axis',(0.,-0.669130606358858,-0.743144825477394));
#60954=DIRECTION('ref_axis',(1.,0.,0.));
#60955=DIRECTION('',(-0.137844537491629,-0.736050673949001,0.662743003631831));
#60956=DIRECTION('center_axis',(-0.99026806874157,0.0894587448987841,-0.106612780622095));
#60957=DIRECTION('ref_axis',(0.,-0.766044443118978,-0.642787609686539));
#60958=DIRECTION('',(-0.137998583506848,-0.730472439966645,0.668854547266653));
#60959=DIRECTION('center_axis',(-0.0617712249622997,-0.667653313133568,
-0.741905229276912));
#60960=DIRECTION('ref_axis',(0.998052578482889,-0.0477845394804615,-0.0400959894540315));
#60961=DIRECTION('',(0.0161503784824051,-0.743896032080767,0.668100186146782));
#60962=DIRECTION('center_axis',(0.284551435696759,-0.637138075424647,-0.71629990457007));
#60963=DIRECTION('ref_axis',(0.957826285221151,0.220121250980087,0.184703660511672));
#60964=DIRECTION('',(0.0552259184163645,-0.735052736908566,0.675757036144127));
#60965=DIRECTION('center_axis',(0.491310548314113,-0.569181257019307,-0.659277363310168));
#60966=DIRECTION('ref_axis',(0.86824314212446,0.3800644767432,0.318911962258805));
#60967=DIRECTION('',(0.057078643955053,-0.734265753494182,0.676458300008118));
#60968=DIRECTION('center_axis',(0.313150259135957,-0.630202302718315,-0.710480100250258));
#60969=DIRECTION('ref_axis',(0.948683298050513,0.242244522917128,0.203267289834479));
#60970=DIRECTION('',(0.0225789275220278,-0.742955370751214,0.668960020557194));
#60971=DIRECTION('center_axis',(0.,-0.669130606358858,-0.743144825477394));
#60972=DIRECTION('ref_axis',(1.,0.,0.));
#60973=DIRECTION('',(-0.0225789275220274,-0.742955370751214,0.668960020557194));
#60974=DIRECTION('center_axis',(-0.313150259135956,-0.630202302718315,-0.710480100250258));
#60975=DIRECTION('ref_axis',(0.948683298050513,-0.242244522917128,-0.203267289834478));
#60976=DIRECTION('',(-0.0570786439550527,-0.734265753494182,0.676458300008118));
#60977=DIRECTION('center_axis',(-0.491310548314114,-0.569181257019307,-0.659277363310167));
#60978=DIRECTION('ref_axis',(0.868243142124459,-0.380064476743201,-0.318911962258806));
#60979=DIRECTION('',(-0.0552259184163635,-0.735052736908566,0.675757036144127));
#60980=DIRECTION('center_axis',(-0.284551435696759,-0.637138075424646,-0.71629990457007));
#60981=DIRECTION('ref_axis',(0.957826285221151,-0.220121250980087,-0.184703660511673));
#60982=DIRECTION('',(-0.0161503784824052,-0.743896032080767,0.668100186146782));
#60983=DIRECTION('center_axis',(0.0617712249622996,-0.667653313133567,-0.741905229276912));
#60984=DIRECTION('ref_axis',(0.998052578482889,0.0477845394804615,0.0400959894540314));
#60985=DIRECTION('',(0.137998583506848,-0.730472439966645,0.668854547266653));
#60986=DIRECTION('center_axis',(0.99026806874157,0.0894587448987838,-0.106612780622095));
#60987=DIRECTION('ref_axis',(0.,0.766044443118978,0.642787609686539));
#60988=DIRECTION('',(0.137844537491629,-0.736050673949001,0.662743003631831));
#60989=DIRECTION('center_axis',(0.,-0.669130606358858,-0.743144825477394));
#60990=DIRECTION('ref_axis',(1.,0.,0.));
#60991=DIRECTION('',(-0.0519254248777279,-0.742142297230154,0.66822792587052));
#60992=DIRECTION('center_axis',(-0.64930555798837,-0.483301338560726,-0.587215555406038));
#60993=DIRECTION('ref_axis',(0.755033118392644,-0.502285118831862,-0.421467257957652));
#60994=DIRECTION('center_axis',(0.,0.848048096156426,0.529919264233205));
#60995=DIRECTION('ref_axis',(-1.,0.,0.));
#60996=DIRECTION('',(-1.,0.,0.));
#60997=DIRECTION('',(0.137844537491629,-0.524860590029465,0.839952525157012));
#60998=DIRECTION('center_axis',(0.99026806874157,0.0894587448987839,-0.106612780622095));
#60999=DIRECTION('ref_axis',(0.,0.766044443118978,0.642787609686539));
#61000=DIRECTION('center_axis',(-0.99026806874157,-0.0894587448987839,0.106612780622095));
#61001=DIRECTION('ref_axis',(-0.139173100960065,0.636532044855303,-0.758589351257639));
#61002=DIRECTION('',(0.137998583506848,-0.531847935749546,0.835520295497991));
#61003=DIRECTION('center_axis',(0.0617712249622996,0.846570802931135,0.528679668032723));
#61004=DIRECTION('ref_axis',(-0.998052578482889,0.0477845394804615,0.0400959894540314));
#61005=DIRECTION('center_axis',(-0.0617712249622996,-0.846570802931135,
-0.528679668032723));
#61006=DIRECTION('ref_axis',(-0.998090334472114,0.0523937700909925,0.0327196743412163));
#61007=DIRECTION('',(-0.0161503784824054,-0.528774052761765,0.848608959651484));
#61008=DIRECTION('center_axis',(-0.284551435696759,0.816055565222214,0.50307434332588));
#61009=DIRECTION('ref_axis',(-0.957826285221151,-0.220121250980087,-0.184703660511673));
#61010=DIRECTION('center_axis',(0.284551435696759,-0.816055565222214,-0.50307434332588));
#61011=DIRECTION('ref_axis',(0.958660774436356,0.242223097976277,0.149323442110948));
#61012=DIRECTION('',(-0.0552259184163639,-0.537850200094025,0.841229612052433));
#61013=DIRECTION('center_axis',(-0.491310548314114,0.748098746816874,0.446051802065978));
#61014=DIRECTION('ref_axis',(-0.868243142124459,-0.380064476743201,-0.318911962258806));
#61015=DIRECTION('center_axis',(0.491310548314114,-0.748098746816874,-0.446051802065978));
#61016=DIRECTION('ref_axis',(0.870984468928858,0.421992375987731,0.25161178329511));
#61017=DIRECTION('',(-0.0570786439550532,-0.538677468419953,0.840576357876501));
#61018=DIRECTION('center_axis',(-0.313150259135956,0.809119792515883,0.497254539006069));
#61019=DIRECTION('ref_axis',(-0.948683298050513,-0.242244522917128,-0.203267289834478));
#61020=DIRECTION('center_axis',(0.313150259135956,-0.809119792515883,-0.497254539006069));
#61021=DIRECTION('ref_axis',(0.949703593340092,0.266794897350299,0.163962091791853));
#61022=DIRECTION('',(-0.0225789275220273,-0.529784168481124,0.847831897759644));
#61023=DIRECTION('center_axis',(0.,0.848048096156426,0.529919264233205));
#61024=DIRECTION('ref_axis',(-1.,0.,0.));
#61025=DIRECTION('',(-1.,0.,0.));
#61026=DIRECTION('',(0.0225789275220281,-0.529784168481124,0.847831897759644));
#61027=DIRECTION('center_axis',(0.313150259135957,0.809119792515883,0.497254539006068));
#61028=DIRECTION('ref_axis',(-0.948683298050513,0.242244522917128,0.203267289834479));
#61029=DIRECTION('center_axis',(-0.313150259135957,-0.809119792515883,-0.497254539006068));
#61030=DIRECTION('ref_axis',(-0.949703593340092,0.2667948973503,0.163962091791853));
#61031=DIRECTION('',(0.0570786439550534,-0.538677468419953,0.840576357876501));
#61032=DIRECTION('center_axis',(0.491310548314113,0.748098746816875,0.446051802065978));
#61033=DIRECTION('ref_axis',(-0.86824314212446,0.3800644767432,0.318911962258805));
#61034=DIRECTION('center_axis',(-0.491310548314113,-0.748098746816875,-0.446051802065978));
#61035=DIRECTION('ref_axis',(-0.870984468928858,0.421992375987729,0.25161178329511));
#61036=DIRECTION('',(0.0552259184163649,-0.537850200094026,0.841229612052432));
#61037=DIRECTION('center_axis',(0.284551435696759,0.816055565222214,0.50307434332588));
#61038=DIRECTION('ref_axis',(-0.957826285221151,0.220121250980087,0.184703660511672));
#61039=DIRECTION('center_axis',(-0.284551435696759,-0.816055565222214,-0.50307434332588));
#61040=DIRECTION('ref_axis',(-0.958660774436356,0.242223097976277,0.149323442110947));
#61041=DIRECTION('',(0.0161503784824051,-0.528774052761765,0.848608959651484));
#61042=DIRECTION('center_axis',(-0.0617712249622997,0.846570802931135,0.528679668032723));
#61043=DIRECTION('ref_axis',(-0.998052578482889,-0.0477845394804615,-0.0400959894540315));
#61044=DIRECTION('center_axis',(0.0617712249622997,-0.846570802931135,-0.528679668032723));
#61045=DIRECTION('ref_axis',(0.998090334472114,0.0523937700909926,0.0327196743412163));
#61046=DIRECTION('',(-0.137998583506848,-0.531847935749546,0.835520295497991));
#61047=DIRECTION('center_axis',(-0.99026806874157,0.0894587448987841,-0.106612780622095));
#61048=DIRECTION('ref_axis',(0.,-0.766044443118978,-0.642787609686539));
#61049=DIRECTION('center_axis',(0.99026806874157,-0.0894587448987841,0.106612780622095));
#61050=DIRECTION('ref_axis',(0.139173100960066,0.636532044855299,-0.758589351257642));
#61051=DIRECTION('',(-0.137844537491629,-0.524860590029465,0.839952525157012));
#61052=DIRECTION('center_axis',(0.,0.848048096156426,0.529919264233205));
#61053=DIRECTION('ref_axis',(-1.,0.,0.));
#61054=DIRECTION('',(-1.,0.,0.));
#61055=DIRECTION('center_axis',(0.,-0.642787609686539,0.766044443118978));
#61056=DIRECTION('ref_axis',(1.,0.,0.));
#61057=DIRECTION('center_axis',(1.,0.,0.));
#61058=DIRECTION('ref_axis',(0.,1.,0.));
#61059=DIRECTION('center_axis',(1.,0.,0.));
#61060=DIRECTION('ref_axis',(0.,0.,-1.));
#61061=DIRECTION('center_axis',(0.64930555798837,0.577927816349714,0.494370034948177));
#61062=DIRECTION('ref_axis',(-0.760527640763576,0.49340973708095,0.422071722564183));
#61063=DIRECTION('',(1.,0.,0.));
#61064=DIRECTION('center_axis',(-0.99026806874157,-0.0695865504800327,0.120527440954873));
#61065=DIRECTION('ref_axis',(-0.139173100960065,0.495134034370783,-0.857597304086756));
#61066=DIRECTION('center_axis',(-0.0617712249622996,0.786340650163727,0.61469724065327));
#61067=DIRECTION('ref_axis',(0.998090334472114,0.0486661612888524,0.0380432514219071));
#61068=DIRECTION('center_axis',(0.284551435696759,0.751842689509058,0.594779833782804));
#61069=DIRECTION('ref_axis',(-0.958660774436356,0.223163315348643,0.176543632679541));
#61070=DIRECTION('center_axis',(0.491310548314114,0.675016427497717,0.550424170729724));
#61071=DIRECTION('ref_axis',(-0.870984468928858,0.380767628982861,0.310486823558562));
#61072=DIRECTION('center_axis',(0.313150259135956,0.744001688360219,0.590252829658806));
#61073=DIRECTION('ref_axis',(-0.949703593340092,0.245323196775732,0.194626858168784));
#61074=DIRECTION('',(1.,0.,0.));
#61075=DIRECTION('center_axis',(-0.313150259135957,0.744001688360219,0.590252829658806));
#61076=DIRECTION('ref_axis',(0.949703593340092,0.245323196775733,0.194626858168784));
#61077=DIRECTION('center_axis',(-0.491310548314113,0.675016427497717,0.550424170729724));
#61078=DIRECTION('ref_axis',(0.870984468928858,0.38076762898286,0.310486823558561));
#61079=DIRECTION('center_axis',(-0.284551435696759,0.751842689509058,0.594779833782804));
#61080=DIRECTION('ref_axis',(0.958660774436356,0.223163315348643,0.176543632679541));
#61081=DIRECTION('center_axis',(0.0617712249622997,0.786340650163727,0.61469724065327));
#61082=DIRECTION('ref_axis',(-0.998090334472114,0.0486661612888524,0.0380432514219071));
#61083=DIRECTION('center_axis',(0.99026806874157,-0.0695865504800328,0.120527440954873));
#61084=DIRECTION('ref_axis',(0.139173100960066,0.495134034370784,-0.857597304086755));
#61085=DIRECTION('',(1.,0.,0.));
#61086=DIRECTION('center_axis',(0.,-0.788010753606722,-0.615661475325658));
#61087=DIRECTION('ref_axis',(1.,0.,0.));
#61088=DIRECTION('',(-0.137844537491629,-0.609784295472661,0.780488306432985));
#61089=DIRECTION('center_axis',(-0.99026806874157,0.0695865504800328,-0.120527440954873));
#61090=DIRECTION('ref_axis',(0.,-0.866025403784439,-0.5));
#61091=DIRECTION('',(-0.137998583506848,-0.603229548983802,0.785538351821795));
#61092=DIRECTION('center_axis',(-0.0617712249622997,-0.786340650163727,
-0.61469724065327));
#61093=DIRECTION('ref_axis',(0.998052578482889,-0.0540211804549215,-0.0311891430775903));
#61094=DIRECTION('',(0.0161503784824051,-0.616580200004832,0.787126433450736));
#61095=DIRECTION('center_axis',(0.284551435696759,-0.751842689509058,-0.594779833782804));
#61096=DIRECTION('ref_axis',(0.957826285221151,0.248850568624199,0.143673942783173));
#61097=DIRECTION('',(0.0552259184163645,-0.606541656308365,0.79313133660055));
#61098=DIRECTION('center_axis',(0.491310548314113,-0.675016427497717,-0.550424170729724));
#61099=DIRECTION('ref_axis',(0.86824314212446,0.429668924423658,0.248069469178416));
#61100=DIRECTION('',(0.057078643955053,-0.605644855748342,0.793685288454953));
#61101=DIRECTION('center_axis',(0.313150259135957,-0.744001688360219,-0.590252829658806));
#61102=DIRECTION('ref_axis',(0.948683298050513,0.273861278752585,0.15811388300842));
#61103=DIRECTION('',(0.0225789275220278,-0.615504520756066,0.787809860918738));
#61104=DIRECTION('center_axis',(0.,-0.788010753606722,-0.615661475325658));
#61105=DIRECTION('ref_axis',(1.,0.,0.));
#61106=DIRECTION('',(-0.0225789275220274,-0.615504520756066,0.787809860918738));
#61107=DIRECTION('center_axis',(-0.313150259135956,-0.744001688360219,-0.590252829658806));
#61108=DIRECTION('ref_axis',(0.948683298050513,-0.273861278752584,-0.158113883008419));
#61109=DIRECTION('',(-0.0570786439550527,-0.605644855748342,0.793685288454953));
#61110=DIRECTION('center_axis',(-0.491310548314114,-0.675016427497717,-0.550424170729724));
#61111=DIRECTION('ref_axis',(0.868243142124459,-0.429668924423659,-0.248069469178417));
#61112=DIRECTION('',(-0.0552259184163635,-0.606541656308365,0.79313133660055));
#61113=DIRECTION('center_axis',(-0.284551435696759,-0.751842689509058,-0.594779833782804));
#61114=DIRECTION('ref_axis',(0.957826285221151,-0.248850568624199,-0.143673942783173));
#61115=DIRECTION('',(-0.0161503784824052,-0.616580200004832,0.787126433450736));
#61116=DIRECTION('center_axis',(0.0617712249622996,-0.786340650163727,-0.61469724065327));
#61117=DIRECTION('ref_axis',(0.998052578482889,0.0540211804549215,0.0311891430775902));
#61118=DIRECTION('',(0.137998583506848,-0.603229548983803,0.785538351821795));
#61119=DIRECTION('center_axis',(0.99026806874157,0.0695865504800327,-0.120527440954873));
#61120=DIRECTION('ref_axis',(0.,0.866025403784439,0.5));
#61121=DIRECTION('',(0.137844537491629,-0.609784295472661,0.780488306432985));
#61122=DIRECTION('center_axis',(0.,-0.788010753606722,-0.615661475325658));
#61123=DIRECTION('ref_axis',(1.,0.,0.));
#61124=DIRECTION('',(-0.0519254248777279,-0.614830926556977,0.786947699660121));
#61125=DIRECTION('center_axis',(-0.64930555798837,-0.577927816349714,-0.494370034948177));
#61126=DIRECTION('ref_axis',(0.755033118392644,-0.567841300538901,-0.327843327723121));
#61127=DIRECTION('center_axis',(0.,0.927183854566788,0.374606593415912));
#61128=DIRECTION('ref_axis',(-1.,0.,0.));
#61129=DIRECTION('',(-1.,0.,0.));
#61130=DIRECTION('',(0.137844537491629,-0.371030552991328,0.918332843924614));
#61131=DIRECTION('center_axis',(0.99026806874157,0.0695865504800327,-0.120527440954873));
#61132=DIRECTION('ref_axis',(0.,0.866025403784439,0.5));
#61133=DIRECTION('center_axis',(-0.99026806874157,-0.0695865504800327,0.120527440954873));
#61134=DIRECTION('ref_axis',(-0.139173100960065,0.495134034370783,-0.857597304086756));
#61135=DIRECTION('',(0.137998583506848,-0.378681393832731,0.9151812896443));
#61136=DIRECTION('center_axis',(0.0617712249622996,0.925513751123792,0.373642358743524));
#61137=DIRECTION('ref_axis',(-0.998052578482889,0.0540211804549215,0.0311891430775902));
#61138=DIRECTION('center_axis',(-0.0617712249622996,-0.925513751123792,
-0.373642358743524));
#61139=DIRECTION('ref_axis',(-0.998090334472114,0.0572795028183562,0.0231245062698634));
#61140=DIRECTION('',(-0.0161503784824054,-0.373381387356162,0.927537333400043));
#61141=DIRECTION('center_axis',(-0.284551435696759,0.891015790469123,0.353724951873058));
#61142=DIRECTION('ref_axis',(-0.957826285221151,-0.248850568624199,-0.143673942783173));
#61143=DIRECTION('center_axis',(0.284551435696759,-0.891015790469123,-0.353724951873058));
#61144=DIRECTION('ref_axis',(0.958660774436356,0.264472928451193,0.104993283944912));
#61145=DIRECTION('',(-0.0552259184163638,-0.3836010578794,0.921846151116809));
#61146=DIRECTION('center_axis',(-0.491310548314114,0.814189528457782,0.309369288819977));
#61147=DIRECTION('ref_axis',(-0.868243142124459,-0.429668924423659,-0.248069469178417));
#61148=DIRECTION('center_axis',(0.491310548314114,-0.814189528457782,-0.309369288819977));
#61149=DIRECTION('ref_axis',(0.870984468928858,0.459273291233482,0.174511027858645));
#61150=DIRECTION('',(-0.0570786439550532,-0.384529194537798,0.921346474976903));
#61151=DIRECTION('center_axis',(-0.313150259135956,0.883174789320284,0.34919794774906));
#61152=DIRECTION('ref_axis',(-0.948683298050513,-0.273861278752584,-0.158113883008419));
#61153=DIRECTION('center_axis',(0.313150259135956,-0.883174789320284,-0.34919794774906));
#61154=DIRECTION('ref_axis',(0.949703593340092,0.291213401820784,0.115142691461001));
#61155=DIRECTION('',(-0.0225789275220273,-0.374511092529479,0.926947481578288));
#61156=DIRECTION('center_axis',(0.,0.927183854566788,0.374606593415912));
#61157=DIRECTION('ref_axis',(-1.,0.,0.));
#61158=DIRECTION('',(-1.,0.,0.));
#61159=DIRECTION('',(0.0225789275220281,-0.374511092529479,0.926947481578288));
#61160=DIRECTION('center_axis',(0.313150259135957,0.883174789320284,0.349197947749059));
#61161=DIRECTION('ref_axis',(-0.948683298050513,0.273861278752585,0.15811388300842));
#61162=DIRECTION('center_axis',(-0.313150259135957,-0.883174789320284,-0.349197947749059));
#61163=DIRECTION('ref_axis',(-0.949703593340092,0.291213401820785,0.115142691461001));
#61164=DIRECTION('',(0.0570786439550533,-0.384529194537798,0.921346474976903));
#61165=DIRECTION('center_axis',(0.491310548314113,0.814189528457783,0.309369288819977));
#61166=DIRECTION('ref_axis',(-0.86824314212446,0.429668924423658,0.248069469178416));
#61167=DIRECTION('center_axis',(-0.491310548314113,-0.814189528457783,-0.309369288819977));
#61168=DIRECTION('ref_axis',(-0.870984468928858,0.459273291233481,0.174511027858644));
#61169=DIRECTION('',(0.0552259184163649,-0.3836010578794,0.921846151116809));
#61170=DIRECTION('center_axis',(0.284551435696759,0.891015790469123,0.353724951873058));
#61171=DIRECTION('ref_axis',(-0.957826285221151,0.248850568624199,0.143673942783173));
#61172=DIRECTION('center_axis',(-0.284551435696759,-0.891015790469123,-0.353724951873058));
#61173=DIRECTION('ref_axis',(-0.958660774436356,0.264472928451193,0.104993283944912));
#61174=DIRECTION('',(0.016150378482405,-0.373381387356162,0.927537333400043));
#61175=DIRECTION('center_axis',(-0.0617712249622997,0.925513751123792,0.373642358743524));
#61176=DIRECTION('ref_axis',(-0.998052578482889,-0.0540211804549215,-0.0311891430775903));
#61177=DIRECTION('center_axis',(0.0617712249622997,-0.925513751123792,-0.373642358743524));
#61178=DIRECTION('ref_axis',(0.998090334472114,0.0572795028183563,0.0231245062698634));
#61179=DIRECTION('',(-0.137998583506848,-0.378681393832731,0.9151812896443));
#61180=DIRECTION('center_axis',(-0.99026806874157,0.0695865504800328,-0.120527440954873));
#61181=DIRECTION('ref_axis',(0.,-0.866025403784439,-0.5));
#61182=DIRECTION('center_axis',(0.99026806874157,-0.0695865504800328,0.120527440954873));
#61183=DIRECTION('ref_axis',(0.139173100960066,0.495134034370784,-0.857597304086755));
#61184=DIRECTION('',(-0.137844537491629,-0.371030552991328,0.918332843924614));
#61185=DIRECTION('center_axis',(0.,0.927183854566788,0.374606593415912));
#61186=DIRECTION('ref_axis',(-1.,0.,0.));
#61187=DIRECTION('',(-1.,0.,0.));
#61188=DIRECTION('center_axis',(0.,-0.5,0.866025403784439));
#61189=DIRECTION('ref_axis',(1.,0.,0.));
#61190=DIRECTION('center_axis',(1.,0.,0.));
#61191=DIRECTION('ref_axis',(0.,1.,0.));
#61192=DIRECTION('center_axis',(1.,0.,0.));
#61193=DIRECTION('ref_axis',(0.,0.,-1.));
#61194=DIRECTION('center_axis',(0.649305557988371,0.654994249884502,0.386503331141725));
#61195=DIRECTION('ref_axis',(-0.760527640763576,0.559205719957048,0.329979803021199));
#61196=DIRECTION('',(1.,0.,0.));
#61197=DIRECTION('center_axis',(-0.99026806874157,-0.0476000039374393,0.130779935984066));
#61198=DIRECTION('ref_axis',(-0.139173100960065,0.338691626801824,-0.930547596796367));
#61199=DIRECTION('center_axis',(-0.0617712249622996,0.881135424446229,0.468811987424192));
#61200=DIRECTION('ref_axis',(0.998090334472114,0.0545329542285434,0.0290144987282327));
#61201=DIRECTION('center_axis',(0.284551435696759,0.843702943923494,0.455187678719166));
#61202=DIRECTION('ref_axis',(-0.958660774436356,0.250429443236754,0.135109635175349));
#61203=DIRECTION('center_axis',(0.491310548314114,0.760341565401402,0.424846618249727));
#61204=DIRECTION('ref_axis',(-0.870984468928858,0.428898384218936,0.239650226161174));
#61205=DIRECTION('center_axis',(0.313150259135956,0.835194959184317,0.452091025520515));
#61206=DIRECTION('ref_axis',(-0.949703593340092,0.27539278542453,0.149070112809494));
#61207=DIRECTION('',(1.,0.,0.));
#61208=DIRECTION('center_axis',(-0.313150259135957,0.835194959184317,0.452091025520515));
#61209=DIRECTION('ref_axis',(0.949703593340092,0.275392785424531,0.149070112809494));
#61210=DIRECTION('center_axis',(-0.491310548314113,0.760341565401403,0.424846618249727));
#61211=DIRECTION('ref_axis',(0.870984468928858,0.428898384218935,0.239650226161173));
#61212=DIRECTION('center_axis',(-0.284551435696759,0.843702943923494,0.455187678719166));
#61213=DIRECTION('ref_axis',(0.958660774436356,0.250429443236754,0.135109635175349));
#61214=DIRECTION('center_axis',(0.0617712249622997,0.881135424446229,0.468811987424191));
#61215=DIRECTION('ref_axis',(-0.998090334472114,0.0545329542285435,0.0290144987282327));
#61216=DIRECTION('center_axis',(0.99026806874157,-0.0476000039374394,0.130779935984066));
#61217=DIRECTION('ref_axis',(0.139173100960066,0.338691626801825,-0.930547596796366));
#61218=DIRECTION('',(1.,0.,0.));
#61219=DIRECTION('center_axis',(0.,-0.882947592858927,-0.469471562785891));
#61220=DIRECTION('ref_axis',(1.,0.,0.));
#61221=DIRECTION('',(-0.137844537491629,-0.464989929744128,0.874518866989312));
#61222=DIRECTION('center_axis',(-0.99026806874157,0.0476000039374394,-0.130779935984066));
#61223=DIRECTION('ref_axis',(0.,-0.939692620785908,-0.342020143325669));
#61224=DIRECTION('',(-0.137998583506848,-0.457657833403968,0.878353971058417));
#61225=DIRECTION('center_axis',(-0.0617712249622997,-0.881135424446229,
-0.468811987424191));
#61226=DIRECTION('ref_axis',(0.998052578482889,-0.058616415197295,-0.0213346303712044));
#61227=DIRECTION('',(0.0161503784824051,-0.470529890556386,0.882236242379483));
#61228=DIRECTION('center_axis',(0.284551435696759,-0.843702943923494,-0.455187678719166));
#61229=DIRECTION('ref_axis',(0.957826285221151,0.270018687665128,0.0982787650057293));
#61230=DIRECTION('',(0.0552259184163645,-0.459601114406122,0.886406742738186));
#61231=DIRECTION('center_axis',(0.491310548314113,-0.760341565401403,-0.424846618249727));
#61232=DIRECTION('ref_axis',(0.86824314212446,0.46621809925847,0.169689510806249));
#61233=DIRECTION('',(0.057078643955053,-0.458621745531673,0.886796551036219));
#61234=DIRECTION('center_axis',(0.313150259135957,-0.835194959184317,-0.452091025520515));
#61235=DIRECTION('ref_axis',(0.948683298050513,0.297156898213637,0.108156265856636));
#61236=DIRECTION('',(0.0225789275220278,-0.469351877358061,0.88272249730729));
#61237=DIRECTION('center_axis',(0.,-0.882947592858927,-0.469471562785891));
#61238=DIRECTION('ref_axis',(1.,0.,0.));
#61239=DIRECTION('',(-0.0225789275220274,-0.469351877358061,0.88272249730729));
#61240=DIRECTION('center_axis',(-0.313150259135956,-0.835194959184317,-0.452091025520515));
#61241=DIRECTION('ref_axis',(0.948683298050514,-0.297156898213636,-0.108156265856635));
#61242=DIRECTION('',(-0.0570786439550527,-0.458621745531673,0.886796551036219));
#61243=DIRECTION('center_axis',(-0.491310548314114,-0.760341565401402,-0.424846618249727));
#61244=DIRECTION('ref_axis',(0.868243142124459,-0.466218099258471,-0.169689510806249));
#61245=DIRECTION('',(-0.0552259184163635,-0.459601114406122,0.886406742738186));
#61246=DIRECTION('center_axis',(-0.284551435696759,-0.843702943923494,-0.455187678719166));
#61247=DIRECTION('ref_axis',(0.957826285221151,-0.270018687665129,-0.0982787650057295));
#61248=DIRECTION('',(-0.0161503784824052,-0.470529890556386,0.882236242379483));
#61249=DIRECTION('center_axis',(0.0617712249622996,-0.881135424446229,-0.468811987424192));
#61250=DIRECTION('ref_axis',(0.998052578482889,0.0586164151972949,0.0213346303712044));
#61251=DIRECTION('',(0.137998583506848,-0.457657833403968,0.878353971058417));
#61252=DIRECTION('center_axis',(0.99026806874157,0.0476000039374393,-0.130779935984066));
#61253=DIRECTION('ref_axis',(0.,0.939692620785908,0.342020143325669));
#61254=DIRECTION('',(0.137844537491629,-0.464989929744127,0.874518866989312));
#61255=DIRECTION('center_axis',(0.,-0.882947592858927,-0.469471562785891));
#61256=DIRECTION('ref_axis',(1.,0.,0.));
#61257=DIRECTION('',(-0.0519254248777279,-0.468838229299828,0.881756465810299));
#61258=DIRECTION('center_axis',(-0.649305557988371,-0.654994249884502,-0.386503331141725));
#61259=DIRECTION('ref_axis',(0.755033118392644,-0.616143911670627,-0.224258043872452));
#61260=DIRECTION('center_axis',(0.,0.978147600733806,0.207911690817759));
#61261=DIRECTION('ref_axis',(-1.,0.,0.));
#61262=DIRECTION('',(-1.,0.,0.));
#61263=DIRECTION('',(0.137844537491629,-0.205926940351068,0.968810083928407));
#61264=DIRECTION('center_axis',(0.99026806874157,0.0476000039374393,-0.130779935984066));
#61265=DIRECTION('ref_axis',(0.,0.939692620785908,0.342020143325669));
#61266=DIRECTION('center_axis',(-0.99026806874157,-0.0476000039374393,0.130779935984066));
#61267=DIRECTION('ref_axis',(-0.139173100960065,0.338691626801824,-0.930547596796367));
#61268=DIRECTION('',(0.137998583506848,-0.214008809386339,0.967034963408845));
#61269=DIRECTION('center_axis',(0.0617712249622996,0.976335432321108,0.20725211545606));
#61270=DIRECTION('ref_axis',(-0.998052578482889,0.0586164151972949,0.0213346303712044));
#61271=DIRECTION('center_axis',(-0.0617712249622996,-0.976335432321108,
-0.20725211545606));
#61272=DIRECTION('ref_axis',(-0.998090334472114,0.0604248268374111,0.0128267117770656));
#61273=DIRECTION('',(-0.0161503784824054,-0.206643717435842,0.978282954629779));
#61274=DIRECTION('center_axis',(-0.284551435696759,0.938902951798373,0.193627806751035));
#61275=DIRECTION('ref_axis',(-0.957826285221151,-0.270018687665129,-0.0982787650057295));
#61276=DIRECTION('center_axis',(0.284551435696759,-0.938902951798373,-0.193627806751035));
#61277=DIRECTION('ref_axis',(0.958660774436356,0.278686882824878,0.0574729579753755));
#61278=DIRECTION('',(-0.0552259184163638,-0.21769639163261,0.974452861356161));
#61279=DIRECTION('center_axis',(-0.491310548314114,0.855541573276281,0.163286746281596));
#61280=DIRECTION('ref_axis',(-0.868243142124459,-0.466218099258471,-0.169689510806249));
#61281=DIRECTION('center_axis',(0.491310548314114,-0.855541573276281,-0.163286746281596));
#61282=DIRECTION('ref_axis',(0.870984468928858,0.482599419928604,0.0921078431475351));
#61283=DIRECTION('',(-0.0570786439550532,-0.218697195660774,0.974121945658943));
#61284=DIRECTION('center_axis',(-0.313150259135956,0.930394967059196,0.190531153552383));
#61285=DIRECTION('ref_axis',(-0.948683298050514,-0.297156898213636,-0.108156265856635));
#61286=DIRECTION('center_axis',(0.313150259135956,-0.930394967059196,-0.190531153552383));
#61287=DIRECTION('ref_axis',(0.949703593340092,0.306783534438035,0.0628247387151196));
#61288=DIRECTION('',(-0.0225789275220273,-0.207858686543083,0.977898235227234));
#61289=DIRECTION('center_axis',(0.,0.978147600733806,0.207911690817759));
#61290=DIRECTION('ref_axis',(-1.,0.,0.));
#61291=DIRECTION('',(-1.,0.,0.));
#61292=DIRECTION('',(0.0225789275220281,-0.207858686543083,0.977898235227234));
#61293=DIRECTION('center_axis',(0.313150259135957,0.930394967059195,0.190531153552383));
#61294=DIRECTION('ref_axis',(-0.948683298050513,0.297156898213637,0.108156265856636));
#61295=DIRECTION('center_axis',(-0.313150259135957,-0.930394967059195,-0.190531153552383));
#61296=DIRECTION('ref_axis',(-0.949703593340092,0.306783534438037,0.0628247387151197));
#61297=DIRECTION('',(0.0570786439550534,-0.218697195660774,0.974121945658943));
#61298=DIRECTION('center_axis',(0.491310548314113,0.855541573276282,0.163286746281596));
#61299=DIRECTION('ref_axis',(-0.86824314212446,0.46621809925847,0.169689510806249));
#61300=DIRECTION('center_axis',(-0.491310548314113,-0.855541573276282,-0.163286746281596));
#61301=DIRECTION('ref_axis',(-0.870984468928858,0.482599419928602,0.0921078431475348));
#61302=DIRECTION('',(0.0552259184163649,-0.21769639163261,0.974452861356161));
#61303=DIRECTION('center_axis',(0.284551435696759,0.938902951798373,0.193627806751035));
#61304=DIRECTION('ref_axis',(-0.957826285221151,0.270018687665128,0.0982787650057293));
#61305=DIRECTION('center_axis',(-0.284551435696759,-0.938902951798373,-0.193627806751035));
#61306=DIRECTION('ref_axis',(-0.958660774436356,0.278686882824878,0.0574729579753754));
#61307=DIRECTION('',(0.0161503784824051,-0.206643717435842,0.978282954629779));
#61308=DIRECTION('center_axis',(-0.0617712249622997,0.976335432321108,0.20725211545606));
#61309=DIRECTION('ref_axis',(-0.998052578482889,-0.058616415197295,-0.0213346303712044));
#61310=DIRECTION('center_axis',(0.0617712249622997,-0.976335432321108,-0.20725211545606));
#61311=DIRECTION('ref_axis',(0.998090334472114,0.0604248268374111,0.0128267117770656));
#61312=DIRECTION('',(-0.137998583506848,-0.214008809386339,0.967034963408845));
#61313=DIRECTION('center_axis',(-0.99026806874157,0.0476000039374394,-0.130779935984066));
#61314=DIRECTION('ref_axis',(0.,-0.939692620785908,-0.342020143325669));
#61315=DIRECTION('center_axis',(0.99026806874157,-0.0476000039374394,0.130779935984066));
#61316=DIRECTION('ref_axis',(0.139173100960066,0.338691626801825,-0.930547596796366));
#61317=DIRECTION('',(-0.137844537491629,-0.205926940351068,0.968810083928407));
#61318=DIRECTION('center_axis',(0.,0.978147600733806,0.207911690817759));
#61319=DIRECTION('ref_axis',(-1.,0.,0.));
#61320=DIRECTION('',(-1.,0.,0.));
#61321=DIRECTION('center_axis',(0.,-0.342020143325669,0.939692620785908));
#61322=DIRECTION('ref_axis',(1.,0.,0.));
#61323=DIRECTION('center_axis',(1.,0.,0.));
#61324=DIRECTION('ref_axis',(0.,1.,0.));
#61325=DIRECTION('center_axis',(1.,0.,0.));
#61326=DIRECTION('ref_axis',(0.,0.,-1.));
#61327=DIRECTION('center_axis',(0.64930555798837,0.712159014579631,0.266892919198654));
#61328=DIRECTION('ref_axis',(-0.760527640763576,0.608010520003998,0.227861614141253));
#61329=DIRECTION('',(1.,0.,0.));
#61330=DIRECTION('center_axis',(-0.99026806874157,-0.0241671553619711,0.137058748836223));
#61331=DIRECTION('ref_axis',(-0.139173100960065,0.171958245538723,-0.975223671657125));
#61332=DIRECTION('center_axis',(-0.0617712249622996,0.949157344732972,0.308682119187541));
#61333=DIRECTION('ref_axis',(0.998090334472114,0.0587427909490065,0.0191041551727457));
#61334=DIRECTION('center_axis',(0.284551435696759,0.909927711321104,0.301764876373726));
#61335=DIRECTION('ref_axis',(-0.958660774436356,0.27008639921553,0.0895703997751286));
#61336=DIRECTION('center_axis',(0.491310548314114,0.822564109591763,0.286360316256974));
#61337=DIRECTION('ref_axis',(-0.870984468928858,0.463997279083573,0.161531977910744));
#61338=DIRECTION('center_axis',(0.313150259135956,0.901011253802641,0.30019266434088));
#61339=DIRECTION('ref_axis',(-0.949703593340092,0.297094703643677,0.0989839475056044));
#61340=DIRECTION('',(1.,0.,0.));
#61341=DIRECTION('center_axis',(-0.313150259135957,0.901011253802641,0.30019266434088));
#61342=DIRECTION('ref_axis',(0.949703593340092,0.297094703643678,0.0989839475056048));
#61343=DIRECTION('center_axis',(-0.491310548314113,0.822564109591764,0.286360316256975));
#61344=DIRECTION('ref_axis',(0.870984468928858,0.463997279083571,0.161531977910744));
#61345=DIRECTION('center_axis',(-0.284551435696759,0.909927711321105,0.301764876373726));
#61346=DIRECTION('ref_axis',(0.958660774436356,0.270086399215529,0.0895703997751284));
#61347=DIRECTION('center_axis',(0.0617712249622997,0.949157344732972,0.308682119187541));
#61348=DIRECTION('ref_axis',(-0.998090334472114,0.0587427909490066,0.0191041551727457));
#61349=DIRECTION('center_axis',(0.99026806874157,-0.0241671553619711,0.137058748836224));
#61350=DIRECTION('ref_axis',(0.139173100960066,0.171958245538724,-0.975223671657125));
#61351=DIRECTION('',(1.,0.,0.));
#61352=DIRECTION('center_axis',(0.,-0.951056516295154,-0.309016994374948));
#61353=DIRECTION('ref_axis',(1.,0.,0.));
#61354=DIRECTION('',(-0.137844537491629,-0.306067080296576,0.941977614300068));
#61355=DIRECTION('center_axis',(-0.99026806874157,0.0241671553619711,-0.137058748836224));
#61356=DIRECTION('ref_axis',(0.,-0.984807753012208,-0.17364817766693));
#61357=DIRECTION('',(-0.137998583506848,-0.298180416142191,0.944481249352984));
#61358=DIRECTION('center_axis',(-0.0617712249622997,-0.949157344732972,
-0.308682119187541));
#61359=DIRECTION('ref_axis',(0.998052578482889,-0.0614306198252359,-0.0108318757168334));
#61360=DIRECTION('',(0.0161503784824051,-0.310182768482997,0.950539749516609));
#61361=DIRECTION('center_axis',(0.284551435696759,-0.909927711321105,-0.301764876373726));
#61362=DIRECTION('ref_axis',(0.957826285221151,0.282982425517402,0.0498974366850415));
#61363=DIRECTION('',(0.0552259184163645,-0.298695825212034,0.952749128541176));
#61364=DIRECTION('center_axis',(0.491310548314113,-0.822564109591764,-0.286360316256975));
#61365=DIRECTION('ref_axis',(0.86824314212446,0.488601473065054,0.0861536225152694));
#61366=DIRECTION('',(0.057078643955053,-0.297663645650825,0.952962949154956));
#61367=DIRECTION('center_axis',(0.313150259135957,-0.901011253802641,-0.30019266434088));
#61368=DIRECTION('ref_axis',(0.948683298050513,0.311423555691114,0.0549123752965087));
#61369=DIRECTION('',(0.0225789275220278,-0.30893821467004,0.950814057294297));
#61370=DIRECTION('center_axis',(0.,-0.951056516295154,-0.309016994374947));
#61371=DIRECTION('ref_axis',(1.,0.,0.));
#61372=DIRECTION('',(-0.0225789275220274,-0.30893821467004,0.950814057294297));
#61373=DIRECTION('center_axis',(-0.313150259135956,-0.901011253802641,-0.30019266434088));
#61374=DIRECTION('ref_axis',(0.948683298050514,-0.311423555691113,-0.0549123752965085));
#61375=DIRECTION('',(-0.0570786439550527,-0.297663645650826,0.952962949154956));
#61376=DIRECTION('center_axis',(-0.491310548314114,-0.822564109591763,-0.286360316256974));
#61377=DIRECTION('ref_axis',(0.868243142124459,-0.488601473065055,-0.0861536225152696));
#61378=DIRECTION('',(-0.0552259184163635,-0.298695825212034,0.952749128541176));
#61379=DIRECTION('center_axis',(-0.284551435696759,-0.909927711321104,-0.301764876373726));
#61380=DIRECTION('ref_axis',(0.957826285221151,-0.282982425517402,-0.0498974366850416));
#61381=DIRECTION('',(-0.0161503784824052,-0.310182768482997,0.950539749516609));
#61382=DIRECTION('center_axis',(0.0617712249622996,-0.949157344732972,-0.308682119187541));
#61383=DIRECTION('ref_axis',(0.998052578482889,0.0614306198252359,0.0108318757168334));
#61384=DIRECTION('',(0.137998583506848,-0.298180416142191,0.944481249352984));
#61385=DIRECTION('center_axis',(0.99026806874157,0.0241671553619711,-0.137058748836223));
#61386=DIRECTION('ref_axis',(0.,0.984807753012208,0.17364817766693));
#61387=DIRECTION('',(0.137844537491629,-0.306067080296576,0.941977614300068));
#61388=DIRECTION('center_axis',(0.,-0.951056516295154,-0.309016994374947));
#61389=DIRECTION('ref_axis',(1.,0.,0.));
#61390=DIRECTION('',(-0.0519254248777279,-0.308600119688995,0.949773507937132));
#61391=DIRECTION('center_axis',(-0.64930555798837,-0.712159014579631,-0.266892919198654));
#61392=DIRECTION('ref_axis',(0.755033118392644,-0.645725301830105,-0.113858792838765));
#61393=DIRECTION('center_axis',(0.,0.999390827019096,0.034899496702501));
#61394=DIRECTION('ref_axis',(-1.,0.,0.));
#61395=DIRECTION('',(-1.,0.,0.));
#61396=DIRECTION('',(0.137844537491629,-0.0345663418323003,0.989850519773593));
#61397=DIRECTION('center_axis',(0.99026806874157,0.0241671553619711,-0.137058748836223));
#61398=DIRECTION('ref_axis',(0.,0.984807753012208,0.17364817766693));
#61399=DIRECTION('center_axis',(-0.99026806874157,-0.0241671553619711,0.137058748836223));
#61400=DIRECTION('ref_axis',(-0.139173100960065,0.171958245538723,-0.975223671657125));
#61401=DIRECTION('',(0.137998583506848,-0.0428336755604258,0.989505769153514));
#61402=DIRECTION('center_axis',(0.0617712249622996,0.997491655456914,0.0345646215150941));
#61403=DIRECTION('ref_axis',(-0.998052578482889,0.0614306198252359,0.0108318757168334));
#61404=DIRECTION('center_axis',(-0.0617712249622996,-0.997491655456914,
-0.0345646215150941));
#61405=DIRECTION('ref_axis',(-0.998090334472114,0.061734173069449,0.0021391841375509));
#61406=DIRECTION('',(-0.0161503784824054,-0.0336272827279996,0.999303943318151));
#61407=DIRECTION('center_axis',(-0.284551435696759,0.958262022045047,0.0276473787012795));
#61408=DIRECTION('ref_axis',(-0.957826285221151,-0.282982425517402,-0.0498974366850416));
#61409=DIRECTION('center_axis',(0.284551435696759,-0.958262022045047,-0.0276473787012795));
#61410=DIRECTION('ref_axis',(0.958660774436356,0.284433077286297,0.00820634526047707));
#61411=DIRECTION('',(-0.0552259184163638,-0.045177130685753,0.997451314500147));
#61412=DIRECTION('center_axis',(-0.491310548314114,0.870898420315705,0.0122428185845279));
#61413=DIRECTION('ref_axis',(-0.868243142124459,-0.488601473065055,-0.0861536225152696));
#61414=DIRECTION('center_axis',(0.491310548314114,-0.870898420315705,-0.0122428185845279));
#61415=DIRECTION('ref_axis',(0.870984468928858,0.491262009456284,0.00690600823120527));
#61416=DIRECTION('',(-0.0570786439550532,-0.0462201931597182,0.997299213951626));
#61417=DIRECTION('center_axis',(-0.313150259135956,0.949345564526583,0.0260751666684337));
#61418=DIRECTION('ref_axis',(-0.948683298050514,-0.311423555691113,-0.0549123752965085));
#61419=DIRECTION('center_axis',(0.313150259135956,-0.949345564526583,-0.0260751666684337));
#61420=DIRECTION('ref_axis',(0.949703593340092,0.313032204601347,0.00859788807423115));
#61421=DIRECTION('',(-0.0225789275220273,-0.0348905995476465,0.999136045839184));
#61422=DIRECTION('center_axis',(0.,0.999390827019096,0.034899496702501));
#61423=DIRECTION('ref_axis',(-1.,0.,0.));
#61424=DIRECTION('',(-1.,0.,0.));
#61425=DIRECTION('',(0.0225789275220281,-0.0348905995476465,0.999136045839184));
#61426=DIRECTION('center_axis',(0.313150259135957,0.949345564526583,0.0260751666684334));
#61427=DIRECTION('ref_axis',(-0.948683298050513,0.311423555691114,0.0549123752965087));
#61428=DIRECTION('center_axis',(-0.313150259135957,-0.949345564526583,-0.0260751666684334));
#61429=DIRECTION('ref_axis',(-0.949703593340092,0.313032204601348,0.0085978880742311));
#61430=DIRECTION('',(0.0570786439550533,-0.0462201931597181,0.997299213951626));
#61431=DIRECTION('center_axis',(0.491310548314113,0.870898420315706,0.0122428185845278));
#61432=DIRECTION('ref_axis',(-0.86824314212446,0.488601473065054,0.0861536225152694));
#61433=DIRECTION('center_axis',(-0.491310548314113,-0.870898420315706,-0.0122428185845278));
#61434=DIRECTION('ref_axis',(-0.870984468928858,0.491262009456283,0.0069060082312052));
#61435=DIRECTION('',(0.0552259184163649,-0.0451771306857534,0.997451314500147));
#61436=DIRECTION('center_axis',(0.284551435696759,0.958262022045047,0.0276473787012796));
#61437=DIRECTION('ref_axis',(-0.957826285221151,0.282982425517402,0.0498974366850415));
#61438=DIRECTION('center_axis',(-0.284551435696759,-0.958262022045047,-0.0276473787012796));
#61439=DIRECTION('ref_axis',(-0.958660774436356,0.284433077286297,0.00820634526047709));
#61440=DIRECTION('',(0.016150378482405,-0.0336272827279996,0.999303943318151));
#61441=DIRECTION('center_axis',(-0.0617712249622997,0.997491655456914,0.0345646215150941));
#61442=DIRECTION('ref_axis',(-0.998052578482889,-0.0614306198252359,-0.0108318757168334));
#61443=DIRECTION('center_axis',(0.0617712249622997,-0.997491655456914,-0.0345646215150941));
#61444=DIRECTION('ref_axis',(0.998090334472114,0.061734173069449,0.0021391841375509));
#61445=DIRECTION('',(-0.137998583506848,-0.0428336755604258,0.989505769153514));
#61446=DIRECTION('center_axis',(-0.99026806874157,0.0241671553619711,-0.137058748836224));
#61447=DIRECTION('ref_axis',(0.,-0.984807753012208,-0.17364817766693));
#61448=DIRECTION('center_axis',(0.99026806874157,-0.0241671553619711,0.137058748836224));
#61449=DIRECTION('ref_axis',(0.139173100960066,0.171958245538724,-0.975223671657125));
#61450=DIRECTION('',(-0.137844537491629,-0.0345663418323003,0.989850519773593));
#61451=DIRECTION('center_axis',(0.,0.999390827019096,0.0348994967025009));
#61452=DIRECTION('ref_axis',(-1.,0.,0.));
#61453=DIRECTION('',(-1.,0.,0.));
#61454=DIRECTION('center_axis',(0.,-0.17364817766693,0.984807753012208));
#61455=DIRECTION('ref_axis',(1.,0.,0.));
#61456=DIRECTION('center_axis',(1.,0.,0.));
#61457=DIRECTION('ref_axis',(0.,1.,0.));
#61458=DIRECTION('center_axis',(1.,0.,0.));
#61459=DIRECTION('ref_axis',(0.,0.,-1.));
#61460=DIRECTION('center_axis',(0.649305557988371,0.747685187986609,0.139173100960065));
#61461=DIRECTION('ref_axis',(-0.760527640763576,0.638341228068795,0.118819965419165));
#61462=DIRECTION('',(1.,0.,0.));
#61463=DIRECTION('center_axis',(-0.99026806874157,8.52189463090778E-18,
0.139173100960065));
#61464=DIRECTION('ref_axis',(0.139173100960065,0.,0.99026806874157));
#61465=DIRECTION('center_axis',(-0.0617712249622996,0.988339599396795,0.139173100960065));
#61466=DIRECTION('ref_axis',(0.998090334472114,0.0611677576917705,0.00861334152950385));
#61467=DIRECTION('center_axis',(0.284551435696759,0.948504785655862,0.139173100960065));
#61468=DIRECTION('ref_axis',(-0.958660774436356,0.281536916624453,0.0413096131025498));
#61469=DIRECTION('center_axis',(0.491310548314114,0.859793459549701,0.139173100960065));
#61470=DIRECTION('ref_axis',(-0.870984468928858,0.484997851417207,0.0785056622506209));
#61471=DIRECTION('center_axis',(0.313150259135956,0.939450777407866,0.139173100960065));
#61472=DIRECTION('ref_axis',(-0.949703593340092,0.309769549629784,0.0458902050450515));
#61473=DIRECTION('',(1.,0.,0.));
#61474=DIRECTION('center_axis',(-0.313150259135957,0.939450777407865,0.139173100960065));
#61475=DIRECTION('ref_axis',(0.949703593340092,0.309769549629785,0.0458902050450517));
#61476=DIRECTION('center_axis',(-0.491310548314113,0.859793459549702,0.139173100960066));
#61477=DIRECTION('ref_axis',(0.870984468928858,0.484997851417206,0.0785056622506207));
#61478=DIRECTION('center_axis',(-0.284551435696759,0.948504785655862,0.139173100960065));
#61479=DIRECTION('ref_axis',(0.958660774436356,0.281536916624453,0.0413096131025497));
#61480=DIRECTION('center_axis',(0.0617712249622997,0.988339599396795,0.139173100960065));
#61481=DIRECTION('ref_axis',(-0.998090334472114,0.0611677576917706,0.00861334152950385));
#61482=DIRECTION('center_axis',(0.99026806874157,8.5218946309078E-18,0.139173100960066));
#61483=DIRECTION('ref_axis',(-0.139173100960066,0.,0.99026806874157));
#61484=DIRECTION('',(1.,0.,0.));
#61485=DIRECTION('center_axis',(0.,-0.99026806874157,-0.139173100960066));
#61486=DIRECTION('ref_axis',(1.,0.,0.));
#61487=DIRECTION('',(-0.137844537491629,-0.137844537491629,0.980814848463989));
#61488=DIRECTION('center_axis',(-0.99026806874157,-8.5218946309078E-18,
-0.139173100960066));
#61489=DIRECTION('ref_axis',(0.,-1.,6.12323399573677E-17));
#61490=DIRECTION('',(-0.137998583506848,-0.129642937822505,0.981910942816534));
#61491=DIRECTION('center_axis',(-0.0617712249622997,-0.988339599396795,
-0.139173100960065));
#61492=DIRECTION('ref_axis',(0.998052578482889,-0.0623782861551806,3.81956842381198E-18));
#61493=DIRECTION('',(0.0161503784824051,-0.140410899949307,0.989961587360995));
#61494=DIRECTION('center_axis',(0.284551435696759,-0.948504785655862,-0.139173100960065));
#61495=DIRECTION('ref_axis',(0.957826285221151,0.287347885566345,-1.75949834150292E-17));
#61496=DIRECTION('',(0.0552259184163645,-0.128714814516259,0.990142714187765));
#61497=DIRECTION('center_axis',(0.491310548314113,-0.859793459549702,-0.139173100960066));
#61498=DIRECTION('ref_axis',(0.86824314212446,0.496138938356832,-3.0379748139553E-17));
#61499=DIRECTION('',(0.057078643955053,-0.12766118652195,0.99017405028614));
#61500=DIRECTION('center_axis',(0.313150259135957,-0.939450777407865,-0.139173100960065));
#61501=DIRECTION('ref_axis',(0.948683298050513,0.31622776601684,-1.9363366072702E-17));
#61502=DIRECTION('',(0.0225789275220278,-0.13913762065955,0.990015613285545));
#61503=DIRECTION('center_axis',(0.,-0.99026806874157,-0.139173100960065));
#61504=DIRECTION('ref_axis',(1.,0.,0.));
#61505=DIRECTION('',(-0.0225789275220274,-0.13913762065955,0.990015613285545));
#61506=DIRECTION('center_axis',(-0.313150259135956,-0.939450777407866,-0.139173100960065));
#61507=DIRECTION('ref_axis',(0.948683298050514,-0.316227766016839,1.9363366072702E-17));
#61508=DIRECTION('',(-0.0570786439550527,-0.12766118652195,0.99017405028614));
#61509=DIRECTION('center_axis',(-0.491310548314114,-0.859793459549701,-0.139173100960065));
#61510=DIRECTION('ref_axis',(0.868243142124459,-0.496138938356833,3.03797481395531E-17));
#61511=DIRECTION('',(-0.0552259184163635,-0.128714814516259,0.990142714187765));
#61512=DIRECTION('center_axis',(-0.284551435696759,-0.948504785655862,-0.139173100960065));
#61513=DIRECTION('ref_axis',(0.957826285221151,-0.287347885566346,1.75949834150293E-17));
#61514=DIRECTION('',(-0.0161503784824052,-0.140410899949307,0.989961587360995));
#61515=DIRECTION('center_axis',(0.0617712249622996,-0.988339599396795,-0.139173100960065));
#61516=DIRECTION('ref_axis',(0.998052578482889,0.0623782861551805,-3.81956842381197E-18));
#61517=DIRECTION('',(0.137998583506848,-0.129642937822505,0.981910942816534));
#61518=DIRECTION('center_axis',(0.99026806874157,-8.52189463090778E-18,
-0.139173100960065));
#61519=DIRECTION('ref_axis',(0.,1.,-6.12323399573677E-17));
#61520=DIRECTION('',(0.137844537491629,-0.137844537491629,0.980814848463989));
#61521=DIRECTION('center_axis',(0.,-0.99026806874157,-0.139173100960065));
#61522=DIRECTION('ref_axis',(1.,0.,0.));
#61523=DIRECTION('',(-0.051925424877728,-0.138985351600607,0.98893216263388));
#61524=DIRECTION('center_axis',(-0.649305557988371,-0.747685187986609,-0.139173100960065));
#61525=DIRECTION('ref_axis',(0.755033118392644,-0.655686655446243,4.01492281917938E-17));
#61526=DIRECTION('center_axis',(0.,0.99026806874157,-0.139173100960065));
#61527=DIRECTION('ref_axis',(-1.,0.,0.));
#61528=DIRECTION('',(-1.,0.,0.));
#61529=DIRECTION('',(0.137844537491629,0.137844537491629,0.980814848463989));
#61530=DIRECTION('center_axis',(0.99026806874157,-8.52189463090778E-18,
-0.139173100960065));
#61531=DIRECTION('ref_axis',(0.,1.,-6.12323399573677E-17));
#61532=DIRECTION('center_axis',(-0.99026806874157,8.52189463090778E-18,
0.139173100960065));
#61533=DIRECTION('ref_axis',(0.139173100960065,0.,0.99026806874157));
#61534=DIRECTION('',(0.137998583506848,0.129642937822505,0.981910942816534));
#61535=DIRECTION('center_axis',(0.0617712249622996,0.988339599396795,-0.139173100960065));
#61536=DIRECTION('ref_axis',(-0.998052578482889,0.0623782861551805,-3.81956842381197E-18));
#61537=DIRECTION('center_axis',(-0.0617712249622996,-0.988339599396795,
0.139173100960065));
#61538=DIRECTION('ref_axis',(-0.998090334472114,0.0611677576917705,-0.00861334152950385));
#61539=DIRECTION('',(-0.0161503784824054,0.140410899949307,0.989961587360995));
#61540=DIRECTION('center_axis',(-0.284551435696759,0.948504785655862,-0.139173100960066));
#61541=DIRECTION('ref_axis',(-0.957826285221151,-0.287347885566346,1.75949834150293E-17));
#61542=DIRECTION('center_axis',(0.284551435696759,-0.948504785655862,0.139173100960066));
#61543=DIRECTION('ref_axis',(0.958660774436356,0.281536916624453,-0.0413096131025498));
#61544=DIRECTION('',(-0.0552259184163638,0.12871481451626,0.990142714187765));
#61545=DIRECTION('center_axis',(-0.491310548314114,0.859793459549701,-0.139173100960066));
#61546=DIRECTION('ref_axis',(-0.868243142124459,-0.496138938356833,3.03797481395531E-17));
#61547=DIRECTION('center_axis',(0.491310548314114,-0.859793459549701,0.139173100960066));
#61548=DIRECTION('ref_axis',(0.870984468928858,0.484997851417207,-0.0785056622506209));
#61549=DIRECTION('',(-0.0570786439550532,0.12766118652195,0.99017405028614));
#61550=DIRECTION('center_axis',(-0.313150259135956,0.939450777407866,-0.139173100960065));
#61551=DIRECTION('ref_axis',(-0.948683298050514,-0.316227766016839,1.9363366072702E-17));
#61552=DIRECTION('center_axis',(0.313150259135956,-0.939450777407866,0.139173100960065));
#61553=DIRECTION('ref_axis',(0.949703593340092,0.309769549629784,-0.0458902050450515));
#61554=DIRECTION('',(-0.0225789275220273,0.139137620659551,0.990015613285545));
#61555=DIRECTION('center_axis',(0.,0.99026806874157,-0.139173100960065));
#61556=DIRECTION('ref_axis',(-1.,0.,0.));
#61557=DIRECTION('',(-1.,0.,0.));
#61558=DIRECTION('',(0.0225789275220281,0.139137620659551,0.990015613285545));
#61559=DIRECTION('center_axis',(0.313150259135957,0.939450777407865,-0.139173100960066));
#61560=DIRECTION('ref_axis',(-0.948683298050513,0.31622776601684,-1.9363366072702E-17));
#61561=DIRECTION('center_axis',(-0.313150259135957,-0.939450777407865,0.139173100960066));
#61562=DIRECTION('ref_axis',(-0.949703593340092,0.309769549629785,-0.0458902050450517));
#61563=DIRECTION('',(0.0570786439550534,0.12766118652195,0.99017405028614));
#61564=DIRECTION('center_axis',(0.491310548314113,0.859793459549702,-0.139173100960066));
#61565=DIRECTION('ref_axis',(-0.86824314212446,0.496138938356832,-3.0379748139553E-17));
#61566=DIRECTION('center_axis',(-0.491310548314113,-0.859793459549702,0.139173100960066));
#61567=DIRECTION('ref_axis',(-0.870984468928858,0.484997851417206,-0.0785056622506208));
#61568=DIRECTION('',(0.0552259184163649,0.128714814516259,0.990142714187765));
#61569=DIRECTION('center_axis',(0.284551435696759,0.948504785655862,-0.139173100960065));
#61570=DIRECTION('ref_axis',(-0.957826285221151,0.287347885566345,-1.75949834150292E-17));
#61571=DIRECTION('center_axis',(-0.284551435696759,-0.948504785655862,0.139173100960065));
#61572=DIRECTION('ref_axis',(-0.958660774436356,0.281536916624453,-0.0413096131025497));
#61573=DIRECTION('',(0.0161503784824051,0.140410899949307,0.989961587360995));
#61574=DIRECTION('center_axis',(-0.0617712249622997,0.988339599396795,-0.139173100960066));
#61575=DIRECTION('ref_axis',(-0.998052578482889,-0.0623782861551806,3.81956842381198E-18));
#61576=DIRECTION('center_axis',(0.0617712249622997,-0.988339599396795,0.139173100960066));
#61577=DIRECTION('ref_axis',(0.998090334472114,0.0611677576917706,-0.00861334152950386));
#61578=DIRECTION('',(-0.137998583506848,0.129642937822505,0.981910942816533));
#61579=DIRECTION('center_axis',(-0.99026806874157,-8.5218946309078E-18,
-0.139173100960066));
#61580=DIRECTION('ref_axis',(0.,-1.,6.12323399573677E-17));
#61581=DIRECTION('center_axis',(0.99026806874157,8.5218946309078E-18,0.139173100960066));
#61582=DIRECTION('ref_axis',(-0.139173100960066,0.,0.99026806874157));
#61583=DIRECTION('',(-0.137844537491629,0.137844537491629,0.980814848463989));
#61584=DIRECTION('center_axis',(0.,0.99026806874157,-0.139173100960066));
#61585=DIRECTION('ref_axis',(-1.,0.,0.));
#61586=DIRECTION('',(-1.,0.,0.));
#61587=DIRECTION('center_axis',(0.,6.12323399573677E-17,1.));
#61588=DIRECTION('ref_axis',(1.,0.,0.));
#61589=DIRECTION('center_axis',(1.,0.,0.));
#61590=DIRECTION('ref_axis',(0.,1.,0.));
#61591=DIRECTION('center_axis',(1.,0.,0.));
#61592=DIRECTION('ref_axis',(0.,0.,-1.));
#61593=DIRECTION('center_axis',(0.64930555798837,0.760493325303574,0.00722457847379229));
#61594=DIRECTION('ref_axis',(-0.760527640763576,0.649276260934969,0.00616803217361924));
#61595=DIRECTION('',(1.,0.,0.));
#61596=DIRECTION('center_axis',(-0.99026806874157,0.0241671553619711,0.137058748836223));
#61597=DIRECTION('ref_axis',(0.139173100960065,0.171958245538723,0.975223671657125));
#61598=DIRECTION('center_axis',(-0.0617712249622996,0.997491655456914,-0.0345646215150942));
#61599=DIRECTION('ref_axis',(0.998090334472114,0.061734173069449,-0.0021391841375509));
#61600=DIRECTION('center_axis',(0.284551435696759,0.958262022045047,-0.0276473787012796));
#61601=DIRECTION('ref_axis',(-0.958660774436356,0.284433077286297,-0.00820634526047711));
#61602=DIRECTION('center_axis',(0.491310548314114,0.870898420315705,-0.0122428185845281));
#61603=DIRECTION('ref_axis',(-0.870984468928858,0.491262009456284,-0.00690600823120538));
#61604=DIRECTION('center_axis',(0.313150259135956,0.949345564526583,-0.0260751666684337));
#61605=DIRECTION('ref_axis',(-0.949703593340092,0.313032204601347,-0.00859788807423117));
#61606=DIRECTION('',(1.,0.,0.));
#61607=DIRECTION('center_axis',(-0.313150259135957,0.949345564526583,-0.0260751666684336));
#61608=DIRECTION('ref_axis',(0.949703593340092,0.313032204601348,-0.00859788807423114));
#61609=DIRECTION('center_axis',(-0.491310548314113,0.870898420315706,-0.0122428185845281));
#61610=DIRECTION('ref_axis',(0.870984468928858,0.491262009456283,-0.00690600823120532));
#61611=DIRECTION('center_axis',(-0.284551435696759,0.958262022045047,-0.0276473787012797));
#61612=DIRECTION('ref_axis',(0.958660774436356,0.284433077286297,-0.00820634526047713));
#61613=DIRECTION('center_axis',(0.0617712249622997,0.997491655456914,-0.0345646215150942));
#61614=DIRECTION('ref_axis',(-0.998090334472114,0.061734173069449,-0.00213918413755091));
#61615=DIRECTION('center_axis',(0.99026806874157,0.0241671553619711,0.137058748836224));
#61616=DIRECTION('ref_axis',(-0.139173100960066,0.171958245538724,0.975223671657125));
#61617=DIRECTION('',(1.,0.,0.));
#61618=DIRECTION('center_axis',(0.,-0.999390827019096,0.0348994967025009));
#61619=DIRECTION('ref_axis',(1.,0.,0.));
#61620=DIRECTION('',(-0.137844537491629,0.0345663418323002,0.989850519773593));
#61621=DIRECTION('center_axis',(-0.99026806874157,-0.0241671553619711,-0.137058748836224));
#61622=DIRECTION('ref_axis',(0.,-0.984807753012208,0.17364817766693));
#61623=DIRECTION('',(-0.137998583506848,0.0428336755604259,0.989505769153514));
#61624=DIRECTION('center_axis',(-0.0617712249622997,-0.997491655456914,
0.0345646215150942));
#61625=DIRECTION('ref_axis',(0.998052578482889,-0.0614306198252359,0.0108318757168334));
#61626=DIRECTION('',(0.0161503784824051,0.0336272827279997,0.999303943318151));
#61627=DIRECTION('center_axis',(0.284551435696759,-0.958262022045047,0.0276473787012797));
#61628=DIRECTION('ref_axis',(0.957826285221151,0.282982425517402,-0.0498974366850415));
#61629=DIRECTION('',(0.0552259184163645,0.0451771306857535,0.997451314500147));
#61630=DIRECTION('center_axis',(0.491310548314113,-0.870898420315706,0.0122428185845281));
#61631=DIRECTION('ref_axis',(0.86824314212446,0.488601473065054,-0.0861536225152694));
#61632=DIRECTION('',(0.057078643955053,0.0462201931597181,0.997299213951626));
#61633=DIRECTION('center_axis',(0.313150259135957,-0.949345564526583,0.0260751666684336));
#61634=DIRECTION('ref_axis',(0.948683298050513,0.311423555691114,-0.0549123752965087));
#61635=DIRECTION('',(0.0225789275220278,0.0348905995476465,0.999136045839184));
#61636=DIRECTION('center_axis',(0.,-0.999390827019096,0.034899496702501));
#61637=DIRECTION('ref_axis',(1.,0.,0.));
#61638=DIRECTION('',(-0.0225789275220274,0.0348905995476465,0.999136045839184));
#61639=DIRECTION('center_axis',(-0.313150259135956,-0.949345564526583,0.0260751666684337));
#61640=DIRECTION('ref_axis',(0.948683298050514,-0.311423555691113,0.0549123752965085));
#61641=DIRECTION('',(-0.0570786439550527,0.0462201931597181,0.997299213951626));
#61642=DIRECTION('center_axis',(-0.491310548314114,-0.870898420315705,0.0122428185845281));
#61643=DIRECTION('ref_axis',(0.868243142124459,-0.488601473065055,0.0861536225152696));
#61644=DIRECTION('',(-0.0552259184163635,0.045177130685753,0.997451314500147));
#61645=DIRECTION('center_axis',(-0.284551435696759,-0.958262022045047,0.0276473787012796));
#61646=DIRECTION('ref_axis',(0.957826285221151,-0.282982425517402,0.0498974366850416));
#61647=DIRECTION('',(-0.0161503784824052,0.0336272827279996,0.999303943318151));
#61648=DIRECTION('center_axis',(0.0617712249622996,-0.997491655456914,0.0345646215150942));
#61649=DIRECTION('ref_axis',(0.998052578482889,0.0614306198252359,-0.0108318757168334));
#61650=DIRECTION('',(0.137998583506848,0.0428336755604258,0.989505769153514));
#61651=DIRECTION('center_axis',(0.99026806874157,-0.0241671553619711,-0.137058748836223));
#61652=DIRECTION('ref_axis',(0.,0.984807753012208,-0.17364817766693));
#61653=DIRECTION('',(0.137844537491629,0.0345663418323004,0.989850519773593));
#61654=DIRECTION('center_axis',(0.,-0.999390827019096,0.034899496702501));
#61655=DIRECTION('ref_axis',(1.,0.,0.));
#61656=DIRECTION('',(-0.051925424877728,0.0348524160661846,0.998042613992818));
#61657=DIRECTION('center_axis',(-0.64930555798837,-0.760493325303574,-0.00722457847379229));
#61658=DIRECTION('ref_axis',(0.755033118392644,-0.645725301830105,0.113858792838765));
#61659=DIRECTION('center_axis',(0.,0.951056516295154,-0.309016994374948));
#61660=DIRECTION('ref_axis',(-1.,0.,0.));
#61661=DIRECTION('',(-1.,0.,0.));
#61662=DIRECTION('',(0.137844537491629,0.306067080296576,0.941977614300068));
#61663=DIRECTION('center_axis',(0.99026806874157,-0.0241671553619711,-0.137058748836223));
#61664=DIRECTION('ref_axis',(0.,0.984807753012208,-0.17364817766693));
#61665=DIRECTION('center_axis',(-0.99026806874157,0.0241671553619711,0.137058748836223));
#61666=DIRECTION('ref_axis',(0.139173100960065,0.171958245538723,0.975223671657125));
#61667=DIRECTION('',(0.137998583506848,0.298180416142191,0.944481249352984));
#61668=DIRECTION('center_axis',(0.0617712249622996,0.949157344732972,-0.308682119187541));
#61669=DIRECTION('ref_axis',(-0.998052578482889,0.0614306198252359,-0.0108318757168334));
#61670=DIRECTION('center_axis',(-0.0617712249622996,-0.949157344732972,
0.308682119187541));
#61671=DIRECTION('ref_axis',(-0.998090334472114,0.0587427909490065,-0.0191041551727457));
#61672=DIRECTION('',(-0.0161503784824054,0.310182768482997,0.950539749516609));
#61673=DIRECTION('center_axis',(-0.284551435696759,0.909927711321104,-0.301764876373726));
#61674=DIRECTION('ref_axis',(-0.957826285221151,-0.282982425517402,0.0498974366850416));
#61675=DIRECTION('center_axis',(0.284551435696759,-0.909927711321104,0.301764876373726));
#61676=DIRECTION('ref_axis',(0.958660774436356,0.27008639921553,-0.0895703997751286));
#61677=DIRECTION('',(-0.0552259184163638,0.298695825212034,0.952749128541176));
#61678=DIRECTION('center_axis',(-0.491310548314114,0.822564109591763,-0.286360316256975));
#61679=DIRECTION('ref_axis',(-0.868243142124459,-0.488601473065055,0.0861536225152696));
#61680=DIRECTION('center_axis',(0.491310548314114,-0.822564109591763,0.286360316256975));
#61681=DIRECTION('ref_axis',(0.870984468928858,0.463997279083572,-0.161531977910744));
#61682=DIRECTION('',(-0.0570786439550532,0.297663645650825,0.952962949154956));
#61683=DIRECTION('center_axis',(-0.313150259135956,0.901011253802641,-0.30019266434088));
#61684=DIRECTION('ref_axis',(-0.948683298050514,-0.311423555691113,0.0549123752965085));
#61685=DIRECTION('center_axis',(0.313150259135956,-0.901011253802641,0.30019266434088));
#61686=DIRECTION('ref_axis',(0.949703593340092,0.297094703643677,-0.0989839475056044));
#61687=DIRECTION('',(-0.0225789275220273,0.30893821467004,0.950814057294297));
#61688=DIRECTION('center_axis',(0.,0.951056516295154,-0.309016994374948));
#61689=DIRECTION('ref_axis',(-1.,0.,0.));
#61690=DIRECTION('',(-1.,0.,0.));
#61691=DIRECTION('',(0.0225789275220281,0.30893821467004,0.950814057294297));
#61692=DIRECTION('center_axis',(0.313150259135957,0.901011253802641,-0.30019266434088));
#61693=DIRECTION('ref_axis',(-0.948683298050513,0.311423555691114,-0.0549123752965087));
#61694=DIRECTION('center_axis',(-0.313150259135957,-0.901011253802641,0.30019266434088));
#61695=DIRECTION('ref_axis',(-0.949703593340092,0.297094703643678,-0.0989839475056049));
#61696=DIRECTION('',(0.0570786439550533,0.297663645650825,0.952962949154956));
#61697=DIRECTION('center_axis',(0.491310548314113,0.822564109591764,-0.286360316256975));
#61698=DIRECTION('ref_axis',(-0.86824314212446,0.488601473065054,-0.0861536225152694));
#61699=DIRECTION('center_axis',(-0.491310548314113,-0.822564109591764,0.286360316256975));
#61700=DIRECTION('ref_axis',(-0.870984468928858,0.463997279083571,-0.161531977910744));
#61701=DIRECTION('',(0.0552259184163649,0.298695825212034,0.952749128541176));
#61702=DIRECTION('center_axis',(0.284551435696759,0.909927711321105,-0.301764876373726));
#61703=DIRECTION('ref_axis',(-0.957826285221151,0.282982425517402,-0.0498974366850415));
#61704=DIRECTION('center_axis',(-0.284551435696759,-0.909927711321105,0.301764876373726));
#61705=DIRECTION('ref_axis',(-0.958660774436356,0.270086399215529,-0.0895703997751284));
#61706=DIRECTION('',(0.0161503784824051,0.310182768482997,0.950539749516609));
#61707=DIRECTION('center_axis',(-0.0617712249622997,0.949157344732972,-0.308682119187541));
#61708=DIRECTION('ref_axis',(-0.998052578482889,-0.0614306198252359,0.0108318757168334));
#61709=DIRECTION('center_axis',(0.0617712249622997,-0.949157344732972,0.308682119187541));
#61710=DIRECTION('ref_axis',(0.998090334472114,0.0587427909490065,-0.0191041551727457));
#61711=DIRECTION('',(-0.137998583506848,0.298180416142191,0.944481249352984));
#61712=DIRECTION('center_axis',(-0.99026806874157,-0.0241671553619711,-0.137058748836224));
#61713=DIRECTION('ref_axis',(0.,-0.984807753012208,0.17364817766693));
#61714=DIRECTION('center_axis',(0.99026806874157,0.0241671553619711,0.137058748836224));
#61715=DIRECTION('ref_axis',(-0.139173100960066,0.171958245538724,0.975223671657125));
#61716=DIRECTION('',(-0.137844537491629,0.306067080296576,0.941977614300068));
#61717=DIRECTION('center_axis',(0.,0.951056516295154,-0.309016994374948));
#61718=DIRECTION('ref_axis',(-1.,0.,0.));
#61719=DIRECTION('',(-1.,0.,0.));
#61720=DIRECTION('center_axis',(0.,0.17364817766693,0.984807753012208));
#61721=DIRECTION('ref_axis',(1.,0.,0.));
#61722=DIRECTION('center_axis',(1.,0.,0.));
#61723=DIRECTION('ref_axis',(0.,1.,0.));
#61724=DIRECTION('center_axis',(1.,0.,0.));
#61725=DIRECTION('ref_axis',(0.,0.,-1.));
#61726=DIRECTION('center_axis',(0.64930555798837,0.75019425775938,-0.124943459173594));
#61727=DIRECTION('ref_axis',(-0.760527640763576,0.640483363162275,-0.106671313608347));
#61728=DIRECTION('',(1.,0.,0.));
#61729=DIRECTION('center_axis',(-0.99026806874157,0.0476000039374394,0.130779935984066));
#61730=DIRECTION('ref_axis',(0.139173100960065,0.338691626801824,0.930547596796367));
#61731=DIRECTION('center_axis',(-0.0617712249622996,0.976335432321108,-0.20725211545606));
#61732=DIRECTION('ref_axis',(0.998090334472114,0.0604248268374111,-0.0128267117770656));
#61733=DIRECTION('center_axis',(0.284551435696759,0.938902951798373,-0.193627806751035));
#61734=DIRECTION('ref_axis',(-0.958660774436356,0.278686882824878,-0.0574729579753755));
#61735=DIRECTION('center_axis',(0.491310548314114,0.855541573276281,-0.163286746281596));
#61736=DIRECTION('ref_axis',(-0.870984468928858,0.482599419928604,-0.0921078431475353));
#61737=DIRECTION('center_axis',(0.313150259135956,0.930394967059196,-0.190531153552384));
#61738=DIRECTION('ref_axis',(-0.949703593340092,0.306783534438036,-0.0628247387151196));
#61739=DIRECTION('',(1.,0.,0.));
#61740=DIRECTION('center_axis',(-0.313150259135957,0.930394967059195,-0.190531153552383));
#61741=DIRECTION('ref_axis',(0.949703593340092,0.306783534438036,-0.0628247387151197));
#61742=DIRECTION('center_axis',(-0.491310548314113,0.855541573276282,-0.163286746281596));
#61743=DIRECTION('ref_axis',(0.870984468928858,0.482599419928602,-0.092107843147535));
#61744=DIRECTION('center_axis',(-0.284551435696759,0.938902951798373,-0.193627806751035));
#61745=DIRECTION('ref_axis',(0.958660774436356,0.278686882824878,-0.0574729579753754));
#61746=DIRECTION('center_axis',(0.0617712249622997,0.976335432321108,-0.20725211545606));
#61747=DIRECTION('ref_axis',(-0.998090334472114,0.0604248268374112,-0.0128267117770656));
#61748=DIRECTION('center_axis',(0.99026806874157,0.0476000039374395,0.130779935984066));
#61749=DIRECTION('ref_axis',(-0.139173100960066,0.338691626801825,0.930547596796366));
#61750=DIRECTION('',(1.,0.,0.));
#61751=DIRECTION('center_axis',(0.,-0.978147600733806,0.207911690817759));
#61752=DIRECTION('ref_axis',(1.,0.,0.));
#61753=DIRECTION('',(-0.137844537491629,0.205926940351068,0.968810083928407));
#61754=DIRECTION('center_axis',(-0.99026806874157,-0.0476000039374395,-0.130779935984066));
#61755=DIRECTION('ref_axis',(0.,-0.939692620785908,0.342020143325669));
#61756=DIRECTION('',(-0.137998583506848,0.214008809386339,0.967034963408844));
#61757=DIRECTION('center_axis',(-0.0617712249622997,-0.976335432321108,
0.20725211545606));
#61758=DIRECTION('ref_axis',(0.998052578482889,-0.058616415197295,0.0213346303712044));
#61759=DIRECTION('',(0.0161503784824051,0.206643717435842,0.978282954629779));
#61760=DIRECTION('center_axis',(0.284551435696759,-0.938902951798373,0.193627806751035));
#61761=DIRECTION('ref_axis',(0.957826285221151,0.270018687665128,-0.0982787650057293));
#61762=DIRECTION('',(0.0552259184163645,0.217696391632611,0.974452861356161));
#61763=DIRECTION('center_axis',(0.491310548314113,-0.855541573276282,0.163286746281596));
#61764=DIRECTION('ref_axis',(0.86824314212446,0.46621809925847,-0.169689510806249));
#61765=DIRECTION('',(0.057078643955053,0.218697195660774,0.974121945658943));
#61766=DIRECTION('center_axis',(0.313150259135957,-0.930394967059195,0.190531153552383));
#61767=DIRECTION('ref_axis',(0.948683298050513,0.297156898213637,-0.108156265856636));
#61768=DIRECTION('',(0.0225789275220278,0.207858686543084,0.977898235227234));
#61769=DIRECTION('center_axis',(0.,-0.978147600733806,0.207911690817759));
#61770=DIRECTION('ref_axis',(1.,0.,0.));
#61771=DIRECTION('',(-0.0225789275220274,0.207858686543084,0.977898235227234));
#61772=DIRECTION('center_axis',(-0.313150259135956,-0.930394967059196,0.190531153552384));
#61773=DIRECTION('ref_axis',(0.948683298050514,-0.297156898213636,0.108156265856635));
#61774=DIRECTION('',(-0.0570786439550527,0.218697195660774,0.974121945658943));
#61775=DIRECTION('center_axis',(-0.491310548314114,-0.855541573276281,0.163286746281596));
#61776=DIRECTION('ref_axis',(0.868243142124459,-0.466218099258471,0.169689510806249));
#61777=DIRECTION('',(-0.0552259184163635,0.21769639163261,0.974452861356161));
#61778=DIRECTION('center_axis',(-0.284551435696759,-0.938902951798373,0.193627806751035));
#61779=DIRECTION('ref_axis',(0.957826285221151,-0.270018687665129,0.0982787650057295));
#61780=DIRECTION('',(-0.0161503784824052,0.206643717435842,0.978282954629779));
#61781=DIRECTION('center_axis',(0.0617712249622996,-0.976335432321108,0.20725211545606));
#61782=DIRECTION('ref_axis',(0.998052578482889,0.0586164151972949,-0.0213346303712044));
#61783=DIRECTION('',(0.137998583506848,0.214008809386339,0.967034963408845));
#61784=DIRECTION('center_axis',(0.99026806874157,-0.0476000039374394,-0.130779935984066));
#61785=DIRECTION('ref_axis',(0.,0.939692620785908,-0.342020143325669));
#61786=DIRECTION('',(0.137844537491629,0.205926940351068,0.968810083928407));
#61787=DIRECTION('center_axis',(0.,-0.978147600733806,0.207911690817759));
#61788=DIRECTION('ref_axis',(1.,0.,0.));
#61789=DIRECTION('',(-0.0519254248777279,0.207631210706978,0.976828045559515));
#61790=DIRECTION('center_axis',(-0.64930555798837,-0.75019425775938,0.124943459173594));
#61791=DIRECTION('ref_axis',(0.755033118392644,-0.616143911670627,0.224258043872453));
#61792=DIRECTION('center_axis',(0.,0.882947592858927,-0.469471562785891));
#61793=DIRECTION('ref_axis',(-1.,0.,0.));
#61794=DIRECTION('',(-1.,0.,0.));
#61795=DIRECTION('',(0.137844537491629,0.464989929744128,0.874518866989312));
#61796=DIRECTION('center_axis',(0.99026806874157,-0.0476000039374394,-0.130779935984066));
#61797=DIRECTION('ref_axis',(0.,0.939692620785908,-0.342020143325669));
#61798=DIRECTION('center_axis',(-0.99026806874157,0.0476000039374394,0.130779935984066));
#61799=DIRECTION('ref_axis',(0.139173100960065,0.338691626801824,0.930547596796367));
#61800=DIRECTION('',(0.137998583506848,0.457657833403968,0.878353971058417));
#61801=DIRECTION('center_axis',(0.0617712249622996,0.881135424446229,-0.468811987424192));
#61802=DIRECTION('ref_axis',(-0.998052578482889,0.0586164151972949,-0.0213346303712044));
#61803=DIRECTION('center_axis',(-0.0617712249622996,-0.881135424446229,
0.468811987424192));
#61804=DIRECTION('ref_axis',(-0.998090334472114,0.0545329542285434,-0.0290144987282327));
#61805=DIRECTION('',(-0.0161503784824054,0.470529890556386,0.882236242379483));
#61806=DIRECTION('center_axis',(-0.284551435696759,0.843702943923494,-0.455187678719166));
#61807=DIRECTION('ref_axis',(-0.957826285221151,-0.270018687665129,0.0982787650057295));
#61808=DIRECTION('center_axis',(0.284551435696759,-0.843702943923494,0.455187678719166));
#61809=DIRECTION('ref_axis',(0.958660774436356,0.250429443236754,-0.135109635175349));
#61810=DIRECTION('',(-0.0552259184163638,0.459601114406122,0.886406742738186));
#61811=DIRECTION('center_axis',(-0.491310548314114,0.760341565401402,-0.424846618249727));
#61812=DIRECTION('ref_axis',(-0.868243142124459,-0.466218099258471,0.169689510806249));
#61813=DIRECTION('center_axis',(0.491310548314114,-0.760341565401402,0.424846618249727));
#61814=DIRECTION('ref_axis',(0.870984468928858,0.428898384218936,-0.239650226161174));
#61815=DIRECTION('',(-0.0570786439550532,0.458621745531673,0.886796551036219));
#61816=DIRECTION('center_axis',(-0.313150259135956,0.835194959184317,-0.452091025520515));
#61817=DIRECTION('ref_axis',(-0.948683298050514,-0.297156898213636,0.108156265856635));
#61818=DIRECTION('center_axis',(0.313150259135956,-0.835194959184317,0.452091025520515));
#61819=DIRECTION('ref_axis',(0.949703593340092,0.27539278542453,-0.149070112809494));
#61820=DIRECTION('',(-0.0225789275220273,0.469351877358061,0.88272249730729));
#61821=DIRECTION('center_axis',(0.,0.882947592858927,-0.469471562785891));
#61822=DIRECTION('ref_axis',(-1.,0.,0.));
#61823=DIRECTION('',(-1.,0.,0.));
#61824=DIRECTION('',(0.0225789275220281,0.469351877358061,0.88272249730729));
#61825=DIRECTION('center_axis',(0.313150259135957,0.835194959184317,-0.452091025520515));
#61826=DIRECTION('ref_axis',(-0.948683298050513,0.297156898213637,-0.108156265856636));
#61827=DIRECTION('center_axis',(-0.313150259135957,-0.835194959184317,0.452091025520515));
#61828=DIRECTION('ref_axis',(-0.949703593340092,0.275392785424531,-0.149070112809494));
#61829=DIRECTION('',(0.0570786439550534,0.458621745531673,0.886796551036219));
#61830=DIRECTION('center_axis',(0.491310548314113,0.760341565401403,-0.424846618249728));
#61831=DIRECTION('ref_axis',(-0.86824314212446,0.46621809925847,-0.169689510806249));
#61832=DIRECTION('center_axis',(-0.491310548314113,-0.760341565401403,0.424846618249728));
#61833=DIRECTION('ref_axis',(-0.870984468928858,0.428898384218935,-0.239650226161173));
#61834=DIRECTION('',(0.0552259184163649,0.459601114406122,0.886406742738186));
#61835=DIRECTION('center_axis',(0.284551435696759,0.843702943923494,-0.455187678719166));
#61836=DIRECTION('ref_axis',(-0.957826285221151,0.270018687665128,-0.0982787650057293));
#61837=DIRECTION('center_axis',(-0.284551435696759,-0.843702943923494,0.455187678719166));
#61838=DIRECTION('ref_axis',(-0.958660774436356,0.250429443236754,-0.135109635175349));
#61839=DIRECTION('',(0.0161503784824051,0.470529890556386,0.882236242379483));
#61840=DIRECTION('center_axis',(-0.0617712249622997,0.881135424446229,-0.468811987424192));
#61841=DIRECTION('ref_axis',(-0.998052578482889,-0.058616415197295,0.0213346303712044));
#61842=DIRECTION('center_axis',(0.0617712249622997,-0.881135424446229,0.468811987424192));
#61843=DIRECTION('ref_axis',(0.998090334472114,0.0545329542285434,-0.0290144987282327));
#61844=DIRECTION('',(-0.137998583506848,0.457657833403968,0.878353971058417));
#61845=DIRECTION('center_axis',(-0.99026806874157,-0.0476000039374395,-0.130779935984066));
#61846=DIRECTION('ref_axis',(0.,-0.939692620785908,0.342020143325669));
#61847=DIRECTION('center_axis',(0.99026806874157,0.0476000039374395,0.130779935984066));
#61848=DIRECTION('ref_axis',(-0.139173100960066,0.338691626801825,0.930547596796366));
#61849=DIRECTION('',(-0.137844537491629,0.464989929744128,0.874518866989312));
#61850=DIRECTION('center_axis',(0.,0.882947592858927,-0.469471562785891));
#61851=DIRECTION('ref_axis',(-1.,0.,0.));
#61852=DIRECTION('',(-1.,0.,0.));
#61853=DIRECTION('center_axis',(0.,0.342020143325669,0.939692620785908));
#61854=DIRECTION('ref_axis',(1.,0.,0.));
#61855=DIRECTION('center_axis',(1.,0.,0.));
#61856=DIRECTION('ref_axis',(0.,1.,0.));
#61857=DIRECTION('center_axis',(1.,0.,0.));
#61858=DIRECTION('ref_axis',(0.,0.,-1.));
#61859=DIRECTION('center_axis',(0.649305557988371,0.717100917309779,-0.253315153038431));
#61860=DIRECTION('ref_axis',(-0.760527640763576,0.612229702500115,-0.216269505504612));
#61861=DIRECTION('',(1.,0.,0.));
#61862=DIRECTION('center_axis',(-0.99026806874157,0.0695865504800327,0.120527440954873));
#61863=DIRECTION('ref_axis',(0.139173100960065,0.495134034370783,0.857597304086756));
#61864=DIRECTION('center_axis',(-0.0617712249622996,0.925513751123792,-0.373642358743524));
#61865=DIRECTION('ref_axis',(0.998090334472114,0.0572795028183562,-0.0231245062698634));
#61866=DIRECTION('center_axis',(0.284551435696759,0.891015790469123,-0.353724951873058));
#61867=DIRECTION('ref_axis',(-0.958660774436356,0.264472928451193,-0.104993283944912));
#61868=DIRECTION('center_axis',(0.491310548314114,0.814189528457782,-0.309369288819978));
#61869=DIRECTION('ref_axis',(-0.870984468928858,0.459273291233482,-0.174511027858645));
#61870=DIRECTION('center_axis',(0.313150259135956,0.883174789320284,-0.34919794774906));
#61871=DIRECTION('ref_axis',(-0.949703593340092,0.291213401820784,-0.115142691461001));
#61872=DIRECTION('',(1.,0.,0.));
#61873=DIRECTION('center_axis',(-0.313150259135957,0.883174789320284,-0.34919794774906));
#61874=DIRECTION('ref_axis',(0.949703593340092,0.291213401820784,-0.115142691461001));
#61875=DIRECTION('center_axis',(-0.491310548314113,0.814189528457783,-0.309369288819978));
#61876=DIRECTION('ref_axis',(0.870984468928858,0.459273291233481,-0.174511027858644));
#61877=DIRECTION('center_axis',(-0.284551435696759,0.891015790469123,-0.353724951873058));
#61878=DIRECTION('ref_axis',(0.958660774436356,0.264472928451193,-0.104993283944912));
#61879=DIRECTION('center_axis',(0.0617712249622997,0.925513751123792,-0.373642358743524));
#61880=DIRECTION('ref_axis',(-0.998090334472114,0.0572795028183562,-0.0231245062698635));
#61881=DIRECTION('center_axis',(0.99026806874157,0.0695865504800329,0.120527440954873));
#61882=DIRECTION('ref_axis',(-0.139173100960066,0.495134034370784,0.857597304086755));
#61883=DIRECTION('',(1.,0.,0.));
#61884=DIRECTION('center_axis',(0.,-0.927183854566788,0.374606593415912));
#61885=DIRECTION('ref_axis',(1.,0.,0.));
#61886=DIRECTION('',(-0.137844537491629,0.371030552991328,0.918332843924613));
#61887=DIRECTION('center_axis',(-0.99026806874157,-0.0695865504800329,-0.120527440954873));
#61888=DIRECTION('ref_axis',(0.,-0.866025403784439,0.5));
#61889=DIRECTION('',(-0.137998583506848,0.378681393832731,0.9151812896443));
#61890=DIRECTION('center_axis',(-0.0617712249622997,-0.925513751123792,
0.373642358743524));
#61891=DIRECTION('ref_axis',(0.998052578482889,-0.0540211804549215,0.0311891430775903));
#61892=DIRECTION('',(0.0161503784824051,0.373381387356163,0.927537333400043));
#61893=DIRECTION('center_axis',(0.284551435696759,-0.891015790469123,0.353724951873058));
#61894=DIRECTION('ref_axis',(0.957826285221151,0.248850568624199,-0.143673942783173));
#61895=DIRECTION('',(0.0552259184163645,0.3836010578794,0.921846151116809));
#61896=DIRECTION('center_axis',(0.491310548314113,-0.814189528457783,0.309369288819978));
#61897=DIRECTION('ref_axis',(0.86824314212446,0.429668924423658,-0.248069469178416));
#61898=DIRECTION('',(0.057078643955053,0.384529194537798,0.921346474976903));
#61899=DIRECTION('center_axis',(0.313150259135957,-0.883174789320284,0.34919794774906));
#61900=DIRECTION('ref_axis',(0.948683298050513,0.273861278752585,-0.15811388300842));
#61901=DIRECTION('',(0.0225789275220278,0.374511092529479,0.926947481578288));
#61902=DIRECTION('center_axis',(0.,-0.927183854566787,0.374606593415912));
#61903=DIRECTION('ref_axis',(1.,0.,0.));
#61904=DIRECTION('',(-0.0225789275220274,0.374511092529479,0.926947481578288));
#61905=DIRECTION('center_axis',(-0.313150259135956,-0.883174789320284,0.34919794774906));
#61906=DIRECTION('ref_axis',(0.948683298050514,-0.273861278752584,0.158113883008419));
#61907=DIRECTION('',(-0.0570786439550527,0.384529194537798,0.921346474976903));
#61908=DIRECTION('center_axis',(-0.491310548314114,-0.814189528457782,0.309369288819978));
#61909=DIRECTION('ref_axis',(0.868243142124459,-0.429668924423659,0.248069469178417));
#61910=DIRECTION('',(-0.0552259184163635,0.3836010578794,0.921846151116809));
#61911=DIRECTION('center_axis',(-0.284551435696759,-0.891015790469123,0.353724951873058));
#61912=DIRECTION('ref_axis',(0.957826285221151,-0.248850568624199,0.143673942783173));
#61913=DIRECTION('',(-0.0161503784824052,0.373381387356163,0.927537333400043));
#61914=DIRECTION('center_axis',(0.0617712249622996,-0.925513751123792,0.373642358743524));
#61915=DIRECTION('ref_axis',(0.998052578482889,0.0540211804549215,-0.0311891430775903));
#61916=DIRECTION('',(0.137998583506848,0.378681393832731,0.9151812896443));
#61917=DIRECTION('center_axis',(0.99026806874157,-0.0695865504800327,-0.120527440954873));
#61918=DIRECTION('ref_axis',(0.,0.866025403784439,-0.5));
#61919=DIRECTION('',(0.137844537491629,0.371030552991328,0.918332843924613));
#61920=DIRECTION('center_axis',(0.,-0.927183854566787,0.374606593415912));
#61921=DIRECTION('ref_axis',(1.,0.,0.));
#61922=DIRECTION('',(-0.0519254248777279,0.374101236076903,0.925933051260727));
#61923=DIRECTION('center_axis',(-0.649305557988371,-0.717100917309779,0.253315153038431));
#61924=DIRECTION('ref_axis',(0.755033118392644,-0.567841300538901,0.327843327723122));
#61925=DIRECTION('center_axis',(0.,0.788010753606722,-0.615661475325658));
#61926=DIRECTION('ref_axis',(-1.,0.,0.));
#61927=DIRECTION('',(-1.,0.,0.));
#61928=DIRECTION('',(0.137844537491629,0.609784295472662,0.780488306432985));
#61929=DIRECTION('center_axis',(0.99026806874157,-0.0695865504800327,-0.120527440954873));
#61930=DIRECTION('ref_axis',(0.,0.866025403784439,-0.5));
#61931=DIRECTION('center_axis',(-0.99026806874157,0.0695865504800327,0.120527440954873));
#61932=DIRECTION('ref_axis',(0.139173100960065,0.495134034370783,0.857597304086756));
#61933=DIRECTION('',(0.137998583506848,0.603229548983803,0.785538351821795));
#61934=DIRECTION('center_axis',(0.0617712249622996,0.786340650163727,-0.61469724065327));
#61935=DIRECTION('ref_axis',(-0.998052578482889,0.0540211804549215,-0.0311891430775903));
#61936=DIRECTION('center_axis',(-0.0617712249622996,-0.786340650163727,
0.61469724065327));
#61937=DIRECTION('ref_axis',(-0.998090334472114,0.0486661612888524,-0.0380432514219071));
#61938=DIRECTION('',(-0.0161503784824054,0.616580200004832,0.787126433450736));
#61939=DIRECTION('center_axis',(-0.284551435696759,0.751842689509057,-0.594779833782804));
#61940=DIRECTION('ref_axis',(-0.957826285221151,-0.248850568624199,0.143673942783173));
#61941=DIRECTION('center_axis',(0.284551435696759,-0.751842689509057,0.594779833782804));
#61942=DIRECTION('ref_axis',(0.958660774436356,0.223163315348643,-0.176543632679541));
#61943=DIRECTION('',(-0.0552259184163638,0.606541656308365,0.793131336600549));
#61944=DIRECTION('center_axis',(-0.491310548314114,0.675016427497717,-0.550424170729724));
#61945=DIRECTION('ref_axis',(-0.868243142124459,-0.429668924423659,0.248069469178417));
#61946=DIRECTION('center_axis',(0.491310548314114,-0.675016427497717,0.550424170729724));
#61947=DIRECTION('ref_axis',(0.870984468928858,0.380767628982861,-0.310486823558562));
#61948=DIRECTION('',(-0.0570786439550532,0.605644855748342,0.793685288454953));
#61949=DIRECTION('center_axis',(-0.313150259135956,0.744001688360219,-0.590252829658806));
#61950=DIRECTION('ref_axis',(-0.948683298050514,-0.273861278752584,0.158113883008419));
#61951=DIRECTION('center_axis',(0.313150259135956,-0.744001688360219,0.590252829658806));
#61952=DIRECTION('ref_axis',(0.949703593340092,0.245323196775732,-0.194626858168784));
#61953=DIRECTION('',(-0.0225789275220273,0.615504520756066,0.787809860918738));
#61954=DIRECTION('center_axis',(0.,0.788010753606722,-0.615661475325658));
#61955=DIRECTION('ref_axis',(-1.,0.,0.));
#61956=DIRECTION('',(-1.,0.,0.));
#61957=DIRECTION('',(0.0225789275220281,0.615504520756066,0.787809860918738));
#61958=DIRECTION('center_axis',(0.313150259135957,0.744001688360218,-0.590252829658806));
#61959=DIRECTION('ref_axis',(-0.948683298050513,0.273861278752585,-0.15811388300842));
#61960=DIRECTION('center_axis',(-0.313150259135957,-0.744001688360218,0.590252829658806));
#61961=DIRECTION('ref_axis',(-0.949703593340092,0.245323196775733,-0.194626858168784));
#61962=DIRECTION('',(0.0570786439550533,0.605644855748342,0.793685288454953));
#61963=DIRECTION('center_axis',(0.491310548314113,0.675016427497717,-0.550424170729724));
#61964=DIRECTION('ref_axis',(-0.86824314212446,0.429668924423658,-0.248069469178416));
#61965=DIRECTION('center_axis',(-0.491310548314113,-0.675016427497717,0.550424170729724));
#61966=DIRECTION('ref_axis',(-0.870984468928858,0.38076762898286,-0.310486823558561));
#61967=DIRECTION('',(0.0552259184163649,0.606541656308365,0.79313133660055));
#61968=DIRECTION('center_axis',(0.284551435696759,0.751842689509058,-0.594779833782804));
#61969=DIRECTION('ref_axis',(-0.957826285221151,0.248850568624199,-0.143673942783173));
#61970=DIRECTION('center_axis',(-0.284551435696759,-0.751842689509058,0.594779833782804));
#61971=DIRECTION('ref_axis',(-0.958660774436356,0.223163315348643,-0.176543632679541));
#61972=DIRECTION('',(0.0161503784824051,0.616580200004832,0.787126433450736));
#61973=DIRECTION('center_axis',(-0.0617712249622997,0.786340650163727,-0.614697240653271));
#61974=DIRECTION('ref_axis',(-0.998052578482889,-0.0540211804549215,0.0311891430775903));
#61975=DIRECTION('center_axis',(0.0617712249622997,-0.786340650163727,0.614697240653271));
#61976=DIRECTION('ref_axis',(0.998090334472114,0.0486661612888524,-0.0380432514219071));
#61977=DIRECTION('',(-0.137998583506848,0.603229548983803,0.785538351821795));
#61978=DIRECTION('center_axis',(-0.99026806874157,-0.0695865504800329,-0.120527440954873));
#61979=DIRECTION('ref_axis',(0.,-0.866025403784439,0.5));
#61980=DIRECTION('center_axis',(0.99026806874157,0.0695865504800329,0.120527440954873));
#61981=DIRECTION('ref_axis',(-0.139173100960066,0.495134034370784,0.857597304086755));
#61982=DIRECTION('',(-0.137844537491629,0.609784295472662,0.780488306432985));
#61983=DIRECTION('center_axis',(0.,0.788010753606722,-0.615661475325658));
#61984=DIRECTION('ref_axis',(-1.,0.,0.));
#61985=DIRECTION('',(-1.,0.,0.));
#61986=DIRECTION('center_axis',(0.,0.5,0.866025403784439));
#61987=DIRECTION('ref_axis',(1.,0.,0.));
#61988=DIRECTION('center_axis',(1.,0.,0.));
#61989=DIRECTION('ref_axis',(0.,1.,0.));
#61990=DIRECTION('center_axis',(1.,0.,0.));
#61991=DIRECTION('ref_axis',(0.,0.,-1.));
#61992=DIRECTION('center_axis',(0.64930555798837,0.662218828358294,-0.373989994161848));
#61993=DIRECTION('ref_axis',(-0.760527640763576,0.565373752130667,-0.31929645791377));
#61994=DIRECTION('',(1.,0.,0.));
#61995=DIRECTION('center_axis',(-0.99026806874157,0.0894587448987838,0.106612780622095));
#61996=DIRECTION('ref_axis',(0.139173100960065,0.636532044855299,0.758589351257642));
#61997=DIRECTION('center_axis',(-0.0617712249622996,0.846570802931135,-0.528679668032723));
#61998=DIRECTION('ref_axis',(0.998090334472114,0.0523937700909925,-0.0327196743412163));
#61999=DIRECTION('center_axis',(0.284551435696759,0.816055565222214,-0.50307434332588));
#62000=DIRECTION('ref_axis',(-0.958660774436356,0.242223097976277,-0.149323442110948));
#62001=DIRECTION('center_axis',(0.491310548314114,0.748098746816874,-0.446051802065978));
#62002=DIRECTION('ref_axis',(-0.870984468928858,0.42199237598773,-0.25161178329511));
#62003=DIRECTION('center_axis',(0.313150259135956,0.809119792515883,-0.497254539006068));
#62004=DIRECTION('ref_axis',(-0.949703593340092,0.266794897350299,-0.163962091791853));
#62005=DIRECTION('',(1.,0.,0.));
#62006=DIRECTION('center_axis',(-0.313150259135957,0.809119792515883,-0.497254539006068));
#62007=DIRECTION('ref_axis',(0.949703593340092,0.2667948973503,-0.163962091791853));
#62008=DIRECTION('center_axis',(-0.491310548314113,0.748098746816875,-0.446051802065978));
#62009=DIRECTION('ref_axis',(0.870984468928858,0.421992375987729,-0.25161178329511));
#62010=DIRECTION('center_axis',(-0.284551435696759,0.816055565222214,-0.503074343325881));
#62011=DIRECTION('ref_axis',(0.958660774436356,0.242223097976277,-0.149323442110948));
#62012=DIRECTION('center_axis',(0.0617712249622997,0.846570802931135,-0.528679668032723));
#62013=DIRECTION('ref_axis',(-0.998090334472114,0.0523937700909926,-0.0327196743412163));
#62014=DIRECTION('center_axis',(0.99026806874157,0.0894587448987841,0.106612780622095));
#62015=DIRECTION('ref_axis',(-0.139173100960066,0.636532044855299,0.758589351257642));
#62016=DIRECTION('',(1.,0.,0.));
#62017=DIRECTION('center_axis',(0.,-0.848048096156426,0.529919264233205));
#62018=DIRECTION('ref_axis',(1.,0.,0.));
#62019=DIRECTION('',(-0.137844537491629,0.524860590029465,0.839952525157012));
#62020=DIRECTION('center_axis',(-0.99026806874157,-0.0894587448987841,-0.106612780622095));
#62021=DIRECTION('ref_axis',(0.,-0.766044443118978,0.642787609686539));
#62022=DIRECTION('',(-0.137998583506848,0.531847935749546,0.835520295497991));
#62023=DIRECTION('center_axis',(-0.0617712249622997,-0.846570802931135,
0.528679668032723));
#62024=DIRECTION('ref_axis',(0.998052578482889,-0.0477845394804615,0.0400959894540315));
#62025=DIRECTION('',(0.0161503784824051,0.528774052761765,0.848608959651484));
#62026=DIRECTION('center_axis',(0.284551435696759,-0.816055565222214,0.503074343325881));
#62027=DIRECTION('ref_axis',(0.957826285221151,0.220121250980087,-0.184703660511672));
#62028=DIRECTION('',(0.0552259184163645,0.537850200094026,0.841229612052432));
#62029=DIRECTION('center_axis',(0.491310548314113,-0.748098746816875,0.446051802065978));
#62030=DIRECTION('ref_axis',(0.86824314212446,0.3800644767432,-0.318911962258805));
#62031=DIRECTION('',(0.057078643955053,0.538677468419953,0.840576357876501));
#62032=DIRECTION('center_axis',(0.313150259135957,-0.809119792515883,0.497254539006068));
#62033=DIRECTION('ref_axis',(0.948683298050513,0.242244522917128,-0.203267289834479));
#62034=DIRECTION('',(0.0225789275220278,0.529784168481124,0.847831897759644));
#62035=DIRECTION('center_axis',(0.,-0.848048096156426,0.529919264233205));
#62036=DIRECTION('ref_axis',(1.,0.,0.));
#62037=DIRECTION('',(-0.0225789275220274,0.529784168481124,0.847831897759644));
#62038=DIRECTION('center_axis',(-0.313150259135956,-0.809119792515883,0.497254539006068));
#62039=DIRECTION('ref_axis',(0.948683298050513,-0.242244522917128,0.203267289834478));
#62040=DIRECTION('',(-0.0570786439550527,0.538677468419953,0.840576357876501));
#62041=DIRECTION('center_axis',(-0.491310548314114,-0.748098746816874,0.446051802065978));
#62042=DIRECTION('ref_axis',(0.868243142124459,-0.380064476743201,0.318911962258806));
#62043=DIRECTION('',(-0.0552259184163635,0.537850200094025,0.841229612052433));
#62044=DIRECTION('center_axis',(-0.284551435696759,-0.816055565222214,0.50307434332588));
#62045=DIRECTION('ref_axis',(0.957826285221151,-0.220121250980087,0.184703660511673));
#62046=DIRECTION('',(-0.0161503784824052,0.528774052761765,0.848608959651484));
#62047=DIRECTION('center_axis',(0.0617712249622996,-0.846570802931135,0.528679668032723));
#62048=DIRECTION('ref_axis',(0.998052578482889,0.0477845394804615,-0.0400959894540314));
#62049=DIRECTION('',(0.137998583506848,0.531847935749546,0.835520295497991));
#62050=DIRECTION('center_axis',(0.99026806874157,-0.0894587448987838,-0.106612780622095));
#62051=DIRECTION('ref_axis',(0.,0.766044443118978,-0.642787609686539));
#62052=DIRECTION('',(0.137844537491629,0.524860590029465,0.839952525157012));
#62053=DIRECTION('center_axis',(0.,-0.848048096156426,0.529919264233205));
#62054=DIRECTION('ref_axis',(1.,0.,0.));
#62055=DIRECTION('',(-0.051925424877728,0.52920438469299,0.846904049744115));
#62056=DIRECTION('center_axis',(-0.64930555798837,-0.662218828358294,0.373989994161848));
#62057=DIRECTION('ref_axis',(0.755033118392644,-0.502285118831862,0.421467257957652));
#62058=DIRECTION('center_axis',(0.,0.669130606358858,-0.743144825477394));
#62059=DIRECTION('ref_axis',(-1.,0.,0.));
#62060=DIRECTION('',(-1.,0.,0.));
#62061=DIRECTION('',(0.137844537491629,0.736050673949001,0.662743003631831));
#62062=DIRECTION('center_axis',(0.99026806874157,-0.0894587448987839,-0.106612780622095));
#62063=DIRECTION('ref_axis',(0.,0.766044443118978,-0.642787609686539));
#62064=DIRECTION('center_axis',(-0.99026806874157,0.0894587448987839,0.106612780622095));
#62065=DIRECTION('ref_axis',(0.139173100960065,0.636532044855303,0.758589351257639));
#62066=DIRECTION('',(0.137998583506848,0.730472439966645,0.668854547266653));
#62067=DIRECTION('center_axis',(0.0617712249622996,0.667653313133567,-0.741905229276912));
#62068=DIRECTION('ref_axis',(-0.998052578482889,0.0477845394804615,-0.0400959894540314));
#62069=DIRECTION('center_axis',(-0.0617712249622996,-0.667653313133567,
0.741905229276912));
#62070=DIRECTION('ref_axis',(-0.998090334472114,0.0413206716646654,-0.045916079171941));
#62071=DIRECTION('',(-0.0161503784824054,0.743896032080767,0.668100186146782));
#62072=DIRECTION('center_axis',(-0.284551435696759,0.637138075424646,-0.71629990457007));
#62073=DIRECTION('ref_axis',(-0.957826285221151,-0.220121250980087,0.184703660511673));
#62074=DIRECTION('center_axis',(0.284551435696759,-0.637138075424646,0.71629990457007));
#62075=DIRECTION('ref_axis',(0.958660774436356,0.18911648304975,-0.212613441240154));
#62076=DIRECTION('',(-0.0552259184163638,0.735052736908566,0.675757036144127));
#62077=DIRECTION('center_axis',(-0.491310548314114,0.569181257019307,-0.659277363310167));
#62078=DIRECTION('ref_axis',(-0.868243142124459,-0.380064476743201,0.318911962258806));
#62079=DIRECTION('center_axis',(0.491310548314114,-0.569181257019307,0.659277363310167));
#62080=DIRECTION('ref_axis',(0.870984468928858,0.32106744201786,-0.371889435936037));
#62081=DIRECTION('',(-0.0570786439550532,0.734265753494182,0.676458300008118));
#62082=DIRECTION('center_axis',(-0.313150259135956,0.630202302718316,-0.710480100250258));
#62083=DIRECTION('ref_axis',(-0.948683298050513,-0.242244522917128,0.203267289834478));
#62084=DIRECTION('center_axis',(0.313150259135956,-0.630202302718316,0.710480100250258));
#62085=DIRECTION('ref_axis',(0.949703593340092,0.207799586932431,-0.234269964928557));
#62086=DIRECTION('',(-0.0225789275220273,0.742955370751214,0.668960020557194));
#62087=DIRECTION('center_axis',(0.,0.669130606358858,-0.743144825477394));
#62088=DIRECTION('ref_axis',(-1.,0.,0.));
#62089=DIRECTION('',(-1.,0.,0.));
#62090=DIRECTION('',(0.0225789275220281,0.742955370751214,0.668960020557194));
#62091=DIRECTION('center_axis',(0.313150259135957,0.630202302718315,-0.710480100250258));
#62092=DIRECTION('ref_axis',(-0.948683298050513,0.242244522917128,-0.203267289834479));
#62093=DIRECTION('center_axis',(-0.313150259135957,-0.630202302718315,0.710480100250258));
#62094=DIRECTION('ref_axis',(-0.949703593340092,0.207799586932432,-0.234269964928558));
#62095=DIRECTION('',(0.0570786439550534,0.734265753494182,0.676458300008118));
#62096=DIRECTION('center_axis',(0.491310548314113,0.569181257019307,-0.659277363310168));
#62097=DIRECTION('ref_axis',(-0.86824314212446,0.3800644767432,-0.318911962258805));
#62098=DIRECTION('center_axis',(-0.491310548314113,-0.569181257019307,0.659277363310168));
#62099=DIRECTION('ref_axis',(-0.870984468928858,0.321067442017859,-0.371889435936036));
#62100=DIRECTION('',(0.0552259184163649,0.735052736908566,0.675757036144127));
#62101=DIRECTION('center_axis',(0.284551435696759,0.637138075424647,-0.71629990457007));
#62102=DIRECTION('ref_axis',(-0.957826285221151,0.220121250980087,-0.184703660511672));
#62103=DIRECTION('center_axis',(-0.284551435696759,-0.637138075424647,0.71629990457007));
#62104=DIRECTION('ref_axis',(-0.958660774436356,0.189116483049749,-0.212613441240154));
#62105=DIRECTION('',(0.016150378482405,0.743896032080767,0.668100186146782));
#62106=DIRECTION('center_axis',(-0.0617712249622997,0.667653313133567,-0.741905229276912));
#62107=DIRECTION('ref_axis',(-0.998052578482889,-0.0477845394804615,0.0400959894540315));
#62108=DIRECTION('center_axis',(0.0617712249622997,-0.667653313133567,0.741905229276912));
#62109=DIRECTION('ref_axis',(0.998090334472114,0.0413206716646654,-0.045916079171941));
#62110=DIRECTION('',(-0.137998583506848,0.730472439966645,0.668854547266653));
#62111=DIRECTION('center_axis',(-0.99026806874157,-0.0894587448987841,-0.106612780622095));
#62112=DIRECTION('ref_axis',(0.,-0.766044443118978,0.642787609686539));
#62113=DIRECTION('center_axis',(0.99026806874157,0.0894587448987841,0.106612780622095));
#62114=DIRECTION('ref_axis',(-0.139173100960066,0.636532044855299,0.758589351257642));
#62115=DIRECTION('',(-0.137844537491629,0.736050673949001,0.662743003631831));
#62116=DIRECTION('center_axis',(0.,0.669130606358858,-0.743144825477394));
#62117=DIRECTION('ref_axis',(-1.,0.,0.));
#62118=DIRECTION('',(-1.,0.,0.));
#62119=DIRECTION('center_axis',(0.,0.642787609686539,0.766044443118978));
#62120=DIRECTION('ref_axis',(1.,0.,0.));
#62121=DIRECTION('center_axis',(1.,0.,0.));
#62122=DIRECTION('ref_axis',(0.,1.,0.));
#62123=DIRECTION('center_axis',(1.,0.,0.));
#62124=DIRECTION('ref_axis',(0.,0.,-1.));
#62125=DIRECTION('center_axis',(0.64930555798837,0.587215555406038,-0.483301338560726));
#62126=DIRECTION('ref_axis',(-0.760527640763576,0.501339206395651,-0.412621749021023));
#62127=DIRECTION('',(1.,0.,0.));
#62128=DIRECTION('center_axis',(-0.99026806874157,0.106612780622095,0.0894587448987838));
#62129=DIRECTION('ref_axis',(0.139173100960065,0.758589351257642,0.636532044855299));
#62130=DIRECTION('center_axis',(-0.0617712249622996,0.741905229276912,-0.667653313133568));
#62131=DIRECTION('ref_axis',(0.998090334472114,0.045916079171941,-0.0413206716646654));
#62132=DIRECTION('center_axis',(0.284551435696759,0.71629990457007,-0.637138075424647));
#62133=DIRECTION('ref_axis',(-0.958660774436356,0.212613441240154,-0.18911648304975));
#62134=DIRECTION('center_axis',(0.491310548314114,0.659277363310167,-0.569181257019307));
#62135=DIRECTION('ref_axis',(-0.870984468928858,0.371889435936037,-0.32106744201786));
#62136=DIRECTION('center_axis',(0.313150259135956,0.710480100250258,-0.630202302718316));
#62137=DIRECTION('ref_axis',(-0.949703593340092,0.234269964928557,-0.207799586932431));
#62138=DIRECTION('',(1.,0.,0.));
#62139=DIRECTION('center_axis',(-0.313150259135957,0.710480100250258,-0.630202302718315));
#62140=DIRECTION('ref_axis',(0.949703593340092,0.234269964928558,-0.207799586932432));
#62141=DIRECTION('center_axis',(-0.491310548314113,0.659277363310168,-0.569181257019307));
#62142=DIRECTION('ref_axis',(0.870984468928858,0.371889435936036,-0.321067442017859));
#62143=DIRECTION('center_axis',(-0.284551435696759,0.71629990457007,-0.637138075424647));
#62144=DIRECTION('ref_axis',(0.958660774436356,0.212613441240154,-0.189116483049749));
#62145=DIRECTION('center_axis',(0.0617712249622997,0.741905229276912,-0.667653313133568));
#62146=DIRECTION('ref_axis',(-0.998090334472114,0.045916079171941,-0.0413206716646654));
#62147=DIRECTION('center_axis',(0.99026806874157,0.106612780622095,0.0894587448987841));
#62148=DIRECTION('ref_axis',(-0.139173100960066,0.758589351257642,0.636532044855299));
#62149=DIRECTION('',(1.,0.,0.));
#62150=DIRECTION('center_axis',(0.,-0.743144825477394,0.669130606358858));
#62151=DIRECTION('ref_axis',(1.,0.,0.));
#62152=DIRECTION('',(-0.137844537491629,0.662743003631831,0.736050673949001));
#62153=DIRECTION('center_axis',(-0.99026806874157,-0.106612780622095,-0.0894587448987841));
#62154=DIRECTION('ref_axis',(0.,-0.642787609686539,0.766044443118978));
#62155=DIRECTION('',(-0.137998583506848,0.668854547266653,0.730472439966645));
#62156=DIRECTION('center_axis',(-0.0617712249622997,-0.741905229276912,
0.667653313133568));
#62157=DIRECTION('ref_axis',(0.998052578482889,-0.0400959894540315,0.0477845394804616));
#62158=DIRECTION('',(0.0161503784824051,0.668100186146782,0.743896032080767));
#62159=DIRECTION('center_axis',(0.284551435696759,-0.71629990457007,0.637138075424647));
#62160=DIRECTION('ref_axis',(0.957826285221151,0.184703660511672,-0.220121250980087));
#62161=DIRECTION('',(0.0552259184163645,0.675757036144128,0.735052736908566));
#62162=DIRECTION('center_axis',(0.491310548314113,-0.659277363310168,0.569181257019307));
#62163=DIRECTION('ref_axis',(0.86824314212446,0.318911962258805,-0.3800644767432));
#62164=DIRECTION('',(0.057078643955053,0.676458300008118,0.734265753494182));
#62165=DIRECTION('center_axis',(0.313150259135957,-0.710480100250258,0.630202302718315));
#62166=DIRECTION('ref_axis',(0.948683298050513,0.203267289834479,-0.242244522917128));
#62167=DIRECTION('',(0.0225789275220278,0.668960020557194,0.742955370751214));
#62168=DIRECTION('center_axis',(0.,-0.743144825477394,0.669130606358858));
#62169=DIRECTION('ref_axis',(1.,0.,0.));
#62170=DIRECTION('',(-0.0225789275220274,0.668960020557194,0.742955370751214));
#62171=DIRECTION('center_axis',(-0.313150259135956,-0.710480100250258,0.630202302718316));
#62172=DIRECTION('ref_axis',(0.948683298050514,-0.203267289834478,0.242244522917128));
#62173=DIRECTION('',(-0.0570786439550527,0.676458300008118,0.734265753494182));
#62174=DIRECTION('center_axis',(-0.491310548314114,-0.659277363310167,0.569181257019307));
#62175=DIRECTION('ref_axis',(0.868243142124459,-0.318911962258806,0.380064476743201));
#62176=DIRECTION('',(-0.0552259184163635,0.675757036144127,0.735052736908566));
#62177=DIRECTION('center_axis',(-0.284551435696759,-0.71629990457007,0.637138075424647));
#62178=DIRECTION('ref_axis',(0.957826285221151,-0.184703660511673,0.220121250980087));
#62179=DIRECTION('',(-0.0161503784824052,0.668100186146782,0.743896032080767));
#62180=DIRECTION('center_axis',(0.0617712249622996,-0.741905229276912,0.667653313133568));
#62181=DIRECTION('ref_axis',(0.998052578482889,0.0400959894540314,-0.0477845394804615));
#62182=DIRECTION('',(0.137998583506848,0.668854547266653,0.730472439966645));
#62183=DIRECTION('center_axis',(0.99026806874157,-0.106612780622095,-0.0894587448987838));
#62184=DIRECTION('ref_axis',(0.,0.642787609686539,-0.766044443118978));
#62185=DIRECTION('',(0.137844537491629,0.662743003631831,0.736050673949001));
#62186=DIRECTION('center_axis',(0.,-0.743144825477394,0.669130606358858));
#62187=DIRECTION('ref_axis',(1.,0.,0.));
#62188=DIRECTION('',(-0.0519254248777279,0.66822792587052,0.742142297230154));
#62189=DIRECTION('center_axis',(-0.64930555798837,-0.587215555406038,0.483301338560726));
#62190=DIRECTION('ref_axis',(0.755033118392644,-0.421467257957652,0.502285118831862));
#62191=DIRECTION('center_axis',(0.,0.529919264233205,-0.848048096156426));
#62192=DIRECTION('ref_axis',(-1.,0.,0.));
#62193=DIRECTION('',(-1.,0.,0.));
#62194=DIRECTION('',(0.137844537491629,0.839952525157012,0.524860590029465));
#62195=DIRECTION('center_axis',(0.99026806874157,-0.106612780622095,-0.0894587448987839));
#62196=DIRECTION('ref_axis',(0.,0.642787609686539,-0.766044443118978));
#62197=DIRECTION('center_axis',(-0.99026806874157,0.106612780622095,0.0894587448987839));
#62198=DIRECTION('ref_axis',(0.139173100960065,0.758589351257639,0.636532044855303));
#62199=DIRECTION('',(0.137998583506848,0.835520295497991,0.531847935749546));
#62200=DIRECTION('center_axis',(0.0617712249622996,0.528679668032723,-0.846570802931135));
#62201=DIRECTION('ref_axis',(-0.998052578482889,0.0400959894540314,-0.0477845394804615));
#62202=DIRECTION('center_axis',(-0.0617712249622996,-0.528679668032723,
0.846570802931135));
#62203=DIRECTION('ref_axis',(-0.998090334472114,0.0327196743412163,-0.0523937700909925));
#62204=DIRECTION('',(-0.0161503784824054,0.848608959651484,0.528774052761765));
#62205=DIRECTION('center_axis',(-0.284551435696759,0.50307434332588,-0.816055565222214));
#62206=DIRECTION('ref_axis',(-0.957826285221151,-0.184703660511673,0.220121250980087));
#62207=DIRECTION('center_axis',(0.284551435696759,-0.50307434332588,0.816055565222214));
#62208=DIRECTION('ref_axis',(0.958660774436356,0.149323442110948,-0.242223097976277));
#62209=DIRECTION('',(-0.0552259184163638,0.841229612052433,0.537850200094025));
#62210=DIRECTION('center_axis',(-0.491310548314114,0.446051802065978,-0.748098746816874));
#62211=DIRECTION('ref_axis',(-0.868243142124459,-0.318911962258806,0.380064476743201));
#62212=DIRECTION('center_axis',(0.491310548314114,-0.446051802065978,0.748098746816874));
#62213=DIRECTION('ref_axis',(0.870984468928858,0.25161178329511,-0.421992375987731));
#62214=DIRECTION('',(-0.0570786439550532,0.840576357876501,0.538677468419953));
#62215=DIRECTION('center_axis',(-0.313150259135956,0.497254539006068,-0.809119792515883));
#62216=DIRECTION('ref_axis',(-0.948683298050514,-0.203267289834478,0.242244522917128));
#62217=DIRECTION('center_axis',(0.313150259135956,-0.497254539006068,0.809119792515883));
#62218=DIRECTION('ref_axis',(0.949703593340092,0.163962091791853,-0.266794897350299));
#62219=DIRECTION('',(-0.0225789275220273,0.847831897759644,0.529784168481124));
#62220=DIRECTION('center_axis',(0.,0.529919264233205,-0.848048096156426));
#62221=DIRECTION('ref_axis',(-1.,0.,0.));
#62222=DIRECTION('',(-1.,0.,0.));
#62223=DIRECTION('',(0.0225789275220281,0.847831897759644,0.529784168481124));
#62224=DIRECTION('center_axis',(0.313150259135957,0.497254539006068,-0.809119792515883));
#62225=DIRECTION('ref_axis',(-0.948683298050513,0.203267289834479,-0.242244522917128));
#62226=DIRECTION('center_axis',(-0.313150259135957,-0.497254539006068,0.809119792515883));
#62227=DIRECTION('ref_axis',(-0.949703593340092,0.163962091791853,-0.2667948973503));
#62228=DIRECTION('',(0.0570786439550534,0.840576357876501,0.538677468419953));
#62229=DIRECTION('center_axis',(0.491310548314113,0.446051802065978,-0.748098746816875));
#62230=DIRECTION('ref_axis',(-0.86824314212446,0.318911962258805,-0.3800644767432));
#62231=DIRECTION('center_axis',(-0.491310548314113,-0.446051802065978,0.748098746816875));
#62232=DIRECTION('ref_axis',(-0.870984468928858,0.25161178329511,-0.421992375987729));
#62233=DIRECTION('',(0.0552259184163649,0.841229612052432,0.537850200094026));
#62234=DIRECTION('center_axis',(0.284551435696759,0.50307434332588,-0.816055565222214));
#62235=DIRECTION('ref_axis',(-0.957826285221151,0.184703660511672,-0.220121250980087));
#62236=DIRECTION('center_axis',(-0.284551435696759,-0.50307434332588,0.816055565222214));
#62237=DIRECTION('ref_axis',(-0.958660774436356,0.149323442110947,-0.242223097976277));
#62238=DIRECTION('',(0.0161503784824051,0.848608959651484,0.528774052761765));
#62239=DIRECTION('center_axis',(-0.0617712249622997,0.528679668032723,-0.846570802931135));
#62240=DIRECTION('ref_axis',(-0.998052578482889,-0.0400959894540315,0.0477845394804616));
#62241=DIRECTION('center_axis',(0.0617712249622997,-0.528679668032723,0.846570802931135));
#62242=DIRECTION('ref_axis',(0.998090334472114,0.0327196743412163,-0.0523937700909926));
#62243=DIRECTION('',(-0.137998583506848,0.835520295497991,0.531847935749546));
#62244=DIRECTION('center_axis',(-0.99026806874157,-0.106612780622095,-0.0894587448987841));
#62245=DIRECTION('ref_axis',(0.,-0.642787609686539,0.766044443118978));
#62246=DIRECTION('center_axis',(0.99026806874157,0.106612780622095,0.0894587448987841));
#62247=DIRECTION('ref_axis',(-0.139173100960066,0.758589351257642,0.636532044855299));
#62248=DIRECTION('',(-0.137844537491629,0.839952525157012,0.524860590029465));
#62249=DIRECTION('center_axis',(0.,0.529919264233205,-0.848048096156426));
#62250=DIRECTION('ref_axis',(-1.,0.,0.));
#62251=DIRECTION('',(-1.,0.,0.));
#62252=DIRECTION('center_axis',(0.,0.766044443118978,0.642787609686539));
#62253=DIRECTION('ref_axis',(1.,0.,0.));
#62254=DIRECTION('center_axis',(1.,0.,0.));
#62255=DIRECTION('ref_axis',(0.,1.,0.));
#62256=DIRECTION('center_axis',(1.,0.,0.));
#62257=DIRECTION('ref_axis',(0.,0.,-1.));
#62258=DIRECTION('center_axis',(0.64930555798837,0.494370034948177,-0.577927816349714));
#62259=DIRECTION('ref_axis',(-0.760527640763576,0.422071722564183,-0.49340973708095));
#62260=DIRECTION('',(1.,0.,0.));
#62261=DIRECTION('center_axis',(-0.99026806874157,0.120527440954873,0.0695865504800327));
#62262=DIRECTION('ref_axis',(0.139173100960065,0.857597304086756,0.495134034370783));
#62263=DIRECTION('center_axis',(-0.0617712249622996,0.61469724065327,-0.786340650163727));
#62264=DIRECTION('ref_axis',(0.998090334472114,0.0380432514219071,-0.0486661612888524));
#62265=DIRECTION('center_axis',(0.284551435696759,0.594779833782804,-0.751842689509058));
#62266=DIRECTION('ref_axis',(-0.958660774436356,0.176543632679541,-0.223163315348643));
#62267=DIRECTION('center_axis',(0.491310548314114,0.550424170729724,-0.675016427497717));
#62268=DIRECTION('ref_axis',(-0.870984468928858,0.310486823558562,-0.380767628982861));
#62269=DIRECTION('center_axis',(0.313150259135956,0.590252829658806,-0.744001688360219));
#62270=DIRECTION('ref_axis',(-0.949703593340092,0.194626858168784,-0.245323196775732));
#62271=DIRECTION('',(1.,0.,0.));
#62272=DIRECTION('center_axis',(-0.313150259135957,0.590252829658806,-0.744001688360219));
#62273=DIRECTION('ref_axis',(0.949703593340092,0.194626858168784,-0.245323196775733));
#62274=DIRECTION('center_axis',(-0.491310548314113,0.550424170729724,-0.675016427497717));
#62275=DIRECTION('ref_axis',(0.870984468928858,0.310486823558561,-0.38076762898286));
#62276=DIRECTION('center_axis',(-0.284551435696759,0.594779833782804,-0.751842689509058));
#62277=DIRECTION('ref_axis',(0.958660774436356,0.176543632679541,-0.223163315348643));
#62278=DIRECTION('center_axis',(0.0617712249622997,0.61469724065327,-0.786340650163727));
#62279=DIRECTION('ref_axis',(-0.998090334472114,0.0380432514219071,-0.0486661612888524));
#62280=DIRECTION('center_axis',(0.99026806874157,0.120527440954873,0.0695865504800329));
#62281=DIRECTION('ref_axis',(-0.139173100960066,0.857597304086755,0.495134034370784));
#62282=DIRECTION('',(1.,0.,0.));
#62283=DIRECTION('center_axis',(0.,-0.615661475325658,0.788010753606722));
#62284=DIRECTION('ref_axis',(1.,0.,0.));
#62285=DIRECTION('',(-0.137844537491629,0.780488306432985,0.609784295472662));
#62286=DIRECTION('center_axis',(-0.99026806874157,-0.120527440954873,-0.0695865504800329));
#62287=DIRECTION('ref_axis',(0.,-0.5,0.866025403784439));
#62288=DIRECTION('',(-0.137998583506848,0.785538351821795,0.603229548983802));
#62289=DIRECTION('center_axis',(-0.0617712249622997,-0.61469724065327,0.786340650163727));
#62290=DIRECTION('ref_axis',(0.998052578482889,-0.0311891430775903,0.0540211804549215));
#62291=DIRECTION('',(0.0161503784824051,0.787126433450736,0.616580200004832));
#62292=DIRECTION('center_axis',(0.284551435696759,-0.594779833782804,0.751842689509058));
#62293=DIRECTION('ref_axis',(0.957826285221151,0.143673942783173,-0.248850568624199));
#62294=DIRECTION('',(0.0552259184163645,0.79313133660055,0.606541656308365));
#62295=DIRECTION('center_axis',(0.491310548314113,-0.550424170729724,0.675016427497717));
#62296=DIRECTION('ref_axis',(0.86824314212446,0.248069469178416,-0.429668924423658));
#62297=DIRECTION('',(0.057078643955053,0.793685288454953,0.605644855748342));
#62298=DIRECTION('center_axis',(0.313150259135957,-0.590252829658806,0.744001688360219));
#62299=DIRECTION('ref_axis',(0.948683298050513,0.15811388300842,-0.273861278752585));
#62300=DIRECTION('',(0.0225789275220278,0.787809860918738,0.615504520756066));
#62301=DIRECTION('center_axis',(0.,-0.615661475325658,0.788010753606722));
#62302=DIRECTION('ref_axis',(1.,0.,0.));
#62303=DIRECTION('',(-0.0225789275220274,0.787809860918738,0.615504520756066));
#62304=DIRECTION('center_axis',(-0.313150259135956,-0.590252829658806,0.744001688360219));
#62305=DIRECTION('ref_axis',(0.948683298050514,-0.158113883008419,0.273861278752584));
#62306=DIRECTION('',(-0.0570786439550527,0.793685288454953,0.605644855748342));
#62307=DIRECTION('center_axis',(-0.491310548314114,-0.550424170729724,0.675016427497717));
#62308=DIRECTION('ref_axis',(0.868243142124459,-0.248069469178417,0.429668924423659));
#62309=DIRECTION('',(-0.0552259184163635,0.793131336600549,0.606541656308365));
#62310=DIRECTION('center_axis',(-0.284551435696759,-0.594779833782804,0.751842689509058));
#62311=DIRECTION('ref_axis',(0.957826285221151,-0.143673942783173,0.248850568624199));
#62312=DIRECTION('',(-0.0161503784824052,0.787126433450736,0.616580200004832));
#62313=DIRECTION('center_axis',(0.0617712249622996,-0.61469724065327,0.786340650163727));
#62314=DIRECTION('ref_axis',(0.998052578482889,0.0311891430775903,-0.0540211804549215));
#62315=DIRECTION('',(0.137998583506848,0.785538351821795,0.603229548983803));
#62316=DIRECTION('center_axis',(0.99026806874157,-0.120527440954873,-0.0695865504800327));
#62317=DIRECTION('ref_axis',(0.,0.5,-0.866025403784439));
#62318=DIRECTION('',(0.137844537491629,0.780488306432985,0.609784295472661));
#62319=DIRECTION('center_axis',(0.,-0.615661475325658,0.788010753606722));
#62320=DIRECTION('ref_axis',(1.,0.,0.));
#62321=DIRECTION('',(-0.0519254248777279,0.786947699660121,0.614830926556978));
#62322=DIRECTION('center_axis',(-0.64930555798837,-0.494370034948177,0.577927816349714));
#62323=DIRECTION('ref_axis',(0.755033118392644,-0.327843327723121,0.567841300538901));
#62324=DIRECTION('center_axis',(0.,0.374606593415912,-0.927183854566788));
#62325=DIRECTION('ref_axis',(-1.,0.,0.));
#62326=DIRECTION('',(-1.,0.,0.));
#62327=DIRECTION('',(0.137844537491629,0.918332843924614,0.371030552991328));
#62328=DIRECTION('center_axis',(0.99026806874157,-0.120527440954873,-0.0695865504800327));
#62329=DIRECTION('ref_axis',(0.,0.5,-0.866025403784439));
#62330=DIRECTION('center_axis',(-0.99026806874157,0.120527440954873,0.0695865504800327));
#62331=DIRECTION('ref_axis',(0.139173100960065,0.857597304086756,0.495134034370783));
#62332=DIRECTION('',(0.137998583506848,0.9151812896443,0.378681393832731));
#62333=DIRECTION('center_axis',(0.0617712249622996,0.373642358743524,-0.925513751123792));
#62334=DIRECTION('ref_axis',(-0.998052578482889,0.0311891430775903,-0.0540211804549215));
#62335=DIRECTION('center_axis',(-0.0617712249622996,-0.373642358743524,
0.925513751123792));
#62336=DIRECTION('ref_axis',(-0.998090334472114,0.0231245062698634,-0.0572795028183562));
#62337=DIRECTION('',(-0.0161503784824054,0.927537333400043,0.373381387356162));
#62338=DIRECTION('center_axis',(-0.284551435696759,0.353724951873058,-0.891015790469123));
#62339=DIRECTION('ref_axis',(-0.957826285221151,-0.143673942783173,0.248850568624199));
#62340=DIRECTION('center_axis',(0.284551435696759,-0.353724951873058,0.891015790469123));
#62341=DIRECTION('ref_axis',(0.958660774436356,0.104993283944912,-0.264472928451193));
#62342=DIRECTION('',(-0.0552259184163638,0.921846151116809,0.3836010578794));
#62343=DIRECTION('center_axis',(-0.491310548314114,0.309369288819977,-0.814189528457782));
#62344=DIRECTION('ref_axis',(-0.868243142124459,-0.248069469178417,0.429668924423659));
#62345=DIRECTION('center_axis',(0.491310548314114,-0.309369288819977,0.814189528457782));
#62346=DIRECTION('ref_axis',(0.870984468928858,0.174511027858645,-0.459273291233482));
#62347=DIRECTION('',(-0.0570786439550532,0.921346474976903,0.384529194537798));
#62348=DIRECTION('center_axis',(-0.313150259135956,0.34919794774906,-0.883174789320284));
#62349=DIRECTION('ref_axis',(-0.948683298050514,-0.158113883008419,0.273861278752584));
#62350=DIRECTION('center_axis',(0.313150259135956,-0.34919794774906,0.883174789320284));
#62351=DIRECTION('ref_axis',(0.949703593340092,0.115142691461001,-0.291213401820783));
#62352=DIRECTION('',(-0.0225789275220273,0.926947481578288,0.374511092529479));
#62353=DIRECTION('center_axis',(0.,0.374606593415912,-0.927183854566788));
#62354=DIRECTION('ref_axis',(-1.,0.,0.));
#62355=DIRECTION('',(-1.,0.,0.));
#62356=DIRECTION('',(0.0225789275220281,0.926947481578288,0.374511092529479));
#62357=DIRECTION('center_axis',(0.313150259135957,0.349197947749059,-0.883174789320284));
#62358=DIRECTION('ref_axis',(-0.948683298050513,0.15811388300842,-0.273861278752585));
#62359=DIRECTION('center_axis',(-0.313150259135957,-0.349197947749059,0.883174789320284));
#62360=DIRECTION('ref_axis',(-0.949703593340092,0.115142691461001,-0.291213401820784));
#62361=DIRECTION('',(0.0570786439550534,0.921346474976903,0.384529194537798));
#62362=DIRECTION('center_axis',(0.491310548314113,0.309369288819978,-0.814189528457783));
#62363=DIRECTION('ref_axis',(-0.86824314212446,0.248069469178416,-0.429668924423658));
#62364=DIRECTION('center_axis',(-0.491310548314113,-0.309369288819978,0.814189528457783));
#62365=DIRECTION('ref_axis',(-0.870984468928858,0.174511027858644,-0.459273291233481));
#62366=DIRECTION('',(0.0552259184163649,0.921846151116809,0.3836010578794));
#62367=DIRECTION('center_axis',(0.284551435696759,0.353724951873058,-0.891015790469123));
#62368=DIRECTION('ref_axis',(-0.957826285221151,0.143673942783173,-0.248850568624199));
#62369=DIRECTION('center_axis',(-0.284551435696759,-0.353724951873058,0.891015790469123));
#62370=DIRECTION('ref_axis',(-0.958660774436356,0.104993283944912,-0.264472928451193));
#62371=DIRECTION('',(0.0161503784824051,0.927537333400043,0.373381387356162));
#62372=DIRECTION('center_axis',(-0.0617712249622997,0.373642358743524,-0.925513751123792));
#62373=DIRECTION('ref_axis',(-0.998052578482889,-0.0311891430775903,0.0540211804549215));
#62374=DIRECTION('center_axis',(0.0617712249622997,-0.373642358743524,0.925513751123792));
#62375=DIRECTION('ref_axis',(0.998090334472114,0.0231245062698634,-0.0572795028183563));
#62376=DIRECTION('',(-0.137998583506848,0.9151812896443,0.378681393832731));
#62377=DIRECTION('center_axis',(-0.99026806874157,-0.120527440954873,-0.0695865504800329));
#62378=DIRECTION('ref_axis',(0.,-0.5,0.866025403784439));
#62379=DIRECTION('center_axis',(0.99026806874157,0.120527440954873,0.0695865504800329));
#62380=DIRECTION('ref_axis',(-0.139173100960066,0.857597304086755,0.495134034370784));
#62381=DIRECTION('',(-0.137844537491629,0.918332843924613,0.371030552991328));
#62382=DIRECTION('center_axis',(0.,0.374606593415912,-0.927183854566787));
#62383=DIRECTION('ref_axis',(-1.,0.,0.));
#62384=DIRECTION('',(-1.,0.,0.));
#62385=DIRECTION('center_axis',(0.,0.866025403784439,0.5));
#62386=DIRECTION('ref_axis',(1.,0.,0.));
#62387=DIRECTION('center_axis',(1.,0.,0.));
#62388=DIRECTION('ref_axis',(0.,1.,0.));
#62389=DIRECTION('center_axis',(1.,0.,0.));
#62390=DIRECTION('ref_axis',(0.,0.,-1.));
#62391=DIRECTION('center_axis',(0.64930555798837,0.386503331141725,-0.654994249884502));
#62392=DIRECTION('ref_axis',(-0.760527640763576,0.329979803021199,-0.559205719957048));
#62393=DIRECTION('',(1.,0.,0.));
#62394=DIRECTION('center_axis',(-0.99026806874157,0.130779935984066,0.0476000039374393));
#62395=DIRECTION('ref_axis',(0.139173100960065,0.930547596796367,0.338691626801823));
#62396=DIRECTION('center_axis',(-0.0617712249622996,0.468811987424192,-0.881135424446229));
#62397=DIRECTION('ref_axis',(0.998090334472114,0.0290144987282327,-0.0545329542285434));
#62398=DIRECTION('center_axis',(0.284551435696759,0.455187678719166,-0.843702943923494));
#62399=DIRECTION('ref_axis',(-0.958660774436356,0.135109635175349,-0.250429443236754));
#62400=DIRECTION('center_axis',(0.491310548314114,0.424846618249727,-0.760341565401402));
#62401=DIRECTION('ref_axis',(-0.870984468928858,0.239650226161174,-0.428898384218936));
#62402=DIRECTION('center_axis',(0.313150259135956,0.452091025520515,-0.835194959184317));
#62403=DIRECTION('ref_axis',(-0.949703593340092,0.149070112809494,-0.27539278542453));
#62404=DIRECTION('',(1.,0.,0.));
#62405=DIRECTION('center_axis',(-0.313150259135957,0.452091025520515,-0.835194959184317));
#62406=DIRECTION('ref_axis',(0.949703593340092,0.149070112809494,-0.275392785424531));
#62407=DIRECTION('center_axis',(-0.491310548314113,0.424846618249727,-0.760341565401403));
#62408=DIRECTION('ref_axis',(0.870984468928858,0.239650226161173,-0.428898384218935));
#62409=DIRECTION('center_axis',(-0.284551435696759,0.455187678719166,-0.843702943923494));
#62410=DIRECTION('ref_axis',(0.958660774436356,0.135109635175349,-0.250429443236754));
#62411=DIRECTION('center_axis',(0.0617712249622997,0.468811987424191,-0.881135424446229));
#62412=DIRECTION('ref_axis',(-0.998090334472114,0.0290144987282327,-0.0545329542285435));
#62413=DIRECTION('center_axis',(0.99026806874157,0.130779935984066,0.0476000039374394));
#62414=DIRECTION('ref_axis',(-0.139173100960066,0.930547596796366,0.338691626801825));
#62415=DIRECTION('',(1.,0.,0.));
#62416=DIRECTION('center_axis',(0.,-0.469471562785891,0.882947592858927));
#62417=DIRECTION('ref_axis',(1.,0.,0.));
#62418=DIRECTION('',(-0.137844537491629,0.874518866989312,0.464989929744128));
#62419=DIRECTION('center_axis',(-0.99026806874157,-0.130779935984066,-0.0476000039374394));
#62420=DIRECTION('ref_axis',(0.,-0.342020143325669,0.939692620785908));
#62421=DIRECTION('',(-0.137998583506848,0.878353971058417,0.457657833403968));
#62422=DIRECTION('center_axis',(-0.0617712249622997,-0.468811987424191,
0.881135424446229));
#62423=DIRECTION('ref_axis',(0.998052578482889,-0.0213346303712044,0.058616415197295));
#62424=DIRECTION('',(0.0161503784824051,0.882236242379483,0.470529890556386));
#62425=DIRECTION('center_axis',(0.284551435696759,-0.455187678719166,0.843702943923494));
#62426=DIRECTION('ref_axis',(0.957826285221151,0.0982787650057293,-0.270018687665128));
#62427=DIRECTION('',(0.0552259184163645,0.886406742738186,0.459601114406122));
#62428=DIRECTION('center_axis',(0.491310548314113,-0.424846618249727,0.760341565401403));
#62429=DIRECTION('ref_axis',(0.86824314212446,0.169689510806249,-0.46621809925847));
#62430=DIRECTION('',(0.057078643955053,0.886796551036219,0.458621745531673));
#62431=DIRECTION('center_axis',(0.313150259135957,-0.452091025520515,0.835194959184317));
#62432=DIRECTION('ref_axis',(0.948683298050513,0.108156265856636,-0.297156898213637));
#62433=DIRECTION('',(0.0225789275220278,0.88272249730729,0.469351877358061));
#62434=DIRECTION('center_axis',(0.,-0.469471562785891,0.882947592858927));
#62435=DIRECTION('ref_axis',(1.,0.,0.));
#62436=DIRECTION('',(-0.0225789275220274,0.88272249730729,0.469351877358061));
#62437=DIRECTION('center_axis',(-0.313150259135956,-0.452091025520515,0.835194959184317));
#62438=DIRECTION('ref_axis',(0.948683298050514,-0.108156265856635,0.297156898213636));
#62439=DIRECTION('',(-0.0570786439550527,0.886796551036219,0.458621745531673));
#62440=DIRECTION('center_axis',(-0.491310548314114,-0.424846618249727,0.760341565401402));
#62441=DIRECTION('ref_axis',(0.868243142124459,-0.169689510806249,0.466218099258471));
#62442=DIRECTION('',(-0.0552259184163635,0.886406742738186,0.459601114406122));
#62443=DIRECTION('center_axis',(-0.284551435696759,-0.455187678719166,0.843702943923494));
#62444=DIRECTION('ref_axis',(0.957826285221151,-0.0982787650057295,0.270018687665129));
#62445=DIRECTION('',(-0.0161503784824052,0.882236242379483,0.470529890556386));
#62446=DIRECTION('center_axis',(0.0617712249622996,-0.468811987424192,0.881135424446229));
#62447=DIRECTION('ref_axis',(0.998052578482889,0.0213346303712044,-0.0586164151972949));
#62448=DIRECTION('',(0.137998583506848,0.878353971058417,0.457657833403968));
#62449=DIRECTION('center_axis',(0.99026806874157,-0.130779935984066,-0.0476000039374393));
#62450=DIRECTION('ref_axis',(0.,0.342020143325669,-0.939692620785908));
#62451=DIRECTION('',(0.137844537491629,0.874518866989312,0.464989929744127));
#62452=DIRECTION('center_axis',(0.,-0.469471562785891,0.882947592858927));
#62453=DIRECTION('ref_axis',(1.,0.,0.));
#62454=DIRECTION('',(-0.0519254248777279,0.881756465810299,0.468838229299828));
#62455=DIRECTION('center_axis',(-0.64930555798837,-0.386503331141725,0.654994249884502));
#62456=DIRECTION('ref_axis',(0.755033118392644,-0.224258043872452,0.616143911670627));
#62457=DIRECTION('center_axis',(0.,0.207911690817759,-0.978147600733806));
#62458=DIRECTION('ref_axis',(-1.,0.,0.));
#62459=DIRECTION('',(-1.,0.,0.));
#62460=DIRECTION('',(0.137844537491629,0.968810083928407,0.205926940351068));
#62461=DIRECTION('center_axis',(0.99026806874157,-0.130779935984066,-0.0476000039374393));
#62462=DIRECTION('ref_axis',(0.,0.342020143325669,-0.939692620785908));
#62463=DIRECTION('center_axis',(-0.99026806874157,0.130779935984066,0.0476000039374393));
#62464=DIRECTION('ref_axis',(0.139173100960065,0.930547596796367,0.338691626801824));
#62465=DIRECTION('',(0.137998583506848,0.967034963408845,0.214008809386339));
#62466=DIRECTION('center_axis',(0.0617712249622996,0.20725211545606,-0.976335432321108));
#62467=DIRECTION('ref_axis',(-0.998052578482889,0.0213346303712044,-0.0586164151972949));
#62468=DIRECTION('center_axis',(-0.0617712249622996,-0.20725211545606,0.976335432321108));
#62469=DIRECTION('ref_axis',(-0.998090334472114,0.0128267117770656,-0.0604248268374111));
#62470=DIRECTION('',(-0.0161503784824054,0.978282954629779,0.206643717435842));
#62471=DIRECTION('center_axis',(-0.284551435696759,0.193627806751035,-0.938902951798373));
#62472=DIRECTION('ref_axis',(-0.957826285221151,-0.0982787650057295,0.270018687665129));
#62473=DIRECTION('center_axis',(0.284551435696759,-0.193627806751035,0.938902951798373));
#62474=DIRECTION('ref_axis',(0.958660774436356,0.0574729579753755,-0.278686882824878));
#62475=DIRECTION('',(-0.0552259184163638,0.974452861356161,0.21769639163261));
#62476=DIRECTION('center_axis',(-0.491310548314114,0.163286746281596,-0.855541573276281));
#62477=DIRECTION('ref_axis',(-0.868243142124459,-0.169689510806249,0.466218099258471));
#62478=DIRECTION('center_axis',(0.491310548314114,-0.163286746281596,0.855541573276281));
#62479=DIRECTION('ref_axis',(0.870984468928858,0.0921078431475352,-0.482599419928604));
#62480=DIRECTION('',(-0.0570786439550532,0.974121945658943,0.218697195660774));
#62481=DIRECTION('center_axis',(-0.313150259135956,0.190531153552383,-0.930394967059196));
#62482=DIRECTION('ref_axis',(-0.948683298050514,-0.108156265856635,0.297156898213636));
#62483=DIRECTION('center_axis',(0.313150259135956,-0.190531153552383,0.930394967059196));
#62484=DIRECTION('ref_axis',(0.949703593340092,0.0628247387151196,-0.306783534438035));
#62485=DIRECTION('',(-0.0225789275220273,0.977898235227234,0.207858686543083));
#62486=DIRECTION('center_axis',(0.,0.207911690817759,-0.978147600733806));
#62487=DIRECTION('ref_axis',(-1.,0.,0.));
#62488=DIRECTION('',(-1.,0.,0.));
#62489=DIRECTION('',(0.0225789275220281,0.977898235227234,0.207858686543083));
#62490=DIRECTION('center_axis',(0.313150259135957,0.190531153552383,-0.930394967059195));
#62491=DIRECTION('ref_axis',(-0.948683298050513,0.108156265856636,-0.297156898213637));
#62492=DIRECTION('center_axis',(-0.313150259135957,-0.190531153552383,0.930394967059195));
#62493=DIRECTION('ref_axis',(-0.949703593340092,0.0628247387151197,-0.306783534438037));
#62494=DIRECTION('',(0.0570786439550534,0.974121945658943,0.218697195660774));
#62495=DIRECTION('center_axis',(0.491310548314113,0.163286746281596,-0.855541573276282));
#62496=DIRECTION('ref_axis',(-0.86824314212446,0.169689510806249,-0.46621809925847));
#62497=DIRECTION('center_axis',(-0.491310548314113,-0.163286746281596,0.855541573276282));
#62498=DIRECTION('ref_axis',(-0.870984468928858,0.0921078431475348,-0.482599419928602));
#62499=DIRECTION('',(0.0552259184163649,0.974452861356161,0.21769639163261));
#62500=DIRECTION('center_axis',(0.284551435696759,0.193627806751035,-0.938902951798373));
#62501=DIRECTION('ref_axis',(-0.957826285221151,0.0982787650057293,-0.270018687665128));
#62502=DIRECTION('center_axis',(-0.284551435696759,-0.193627806751035,0.938902951798373));
#62503=DIRECTION('ref_axis',(-0.958660774436356,0.0574729579753754,-0.278686882824878));
#62504=DIRECTION('',(0.0161503784824051,0.978282954629779,0.206643717435842));
#62505=DIRECTION('center_axis',(-0.0617712249622997,0.20725211545606,-0.976335432321108));
#62506=DIRECTION('ref_axis',(-0.998052578482889,-0.0213346303712044,0.058616415197295));
#62507=DIRECTION('center_axis',(0.0617712249622997,-0.20725211545606,0.976335432321108));
#62508=DIRECTION('ref_axis',(0.998090334472114,0.0128267117770656,-0.0604248268374111));
#62509=DIRECTION('',(-0.137998583506848,0.967034963408845,0.214008809386339));
#62510=DIRECTION('center_axis',(-0.99026806874157,-0.130779935984066,-0.0476000039374394));
#62511=DIRECTION('ref_axis',(0.,-0.342020143325669,0.939692620785908));
#62512=DIRECTION('center_axis',(0.99026806874157,0.130779935984066,0.0476000039374394));
#62513=DIRECTION('ref_axis',(-0.139173100960066,0.930547596796366,0.338691626801825));
#62514=DIRECTION('',(-0.137844537491629,0.968810083928407,0.205926940351068));
#62515=DIRECTION('center_axis',(0.,0.207911690817759,-0.978147600733806));
#62516=DIRECTION('ref_axis',(-1.,0.,0.));
#62517=DIRECTION('',(-1.,0.,0.));
#62518=DIRECTION('center_axis',(0.,0.939692620785908,0.342020143325669));
#62519=DIRECTION('ref_axis',(1.,0.,0.));
#62520=DIRECTION('center_axis',(1.,0.,0.));
#62521=DIRECTION('ref_axis',(0.,1.,0.));
#62522=DIRECTION('center_axis',(1.,0.,0.));
#62523=DIRECTION('ref_axis',(0.,0.,-1.));
#62524=DIRECTION('center_axis',(0.64930555798837,0.266892919198654,-0.712159014579631));
#62525=DIRECTION('ref_axis',(-0.760527640763576,0.227861614141253,-0.608010520003998));
#62526=DIRECTION('',(1.,0.,0.));
#62527=DIRECTION('center_axis',(-0.99026806874157,0.137058748836223,0.0241671553619711));
#62528=DIRECTION('ref_axis',(0.139173100960065,0.975223671657125,0.171958245538723));
#62529=DIRECTION('center_axis',(-0.0617712249622996,0.308682119187541,-0.949157344732972));
#62530=DIRECTION('ref_axis',(0.998090334472114,0.0191041551727457,-0.0587427909490065));
#62531=DIRECTION('center_axis',(0.284551435696759,0.301764876373726,-0.909927711321104));
#62532=DIRECTION('ref_axis',(-0.958660774436356,0.0895703997751286,-0.27008639921553));
#62533=DIRECTION('center_axis',(0.491310548314114,0.286360316256974,-0.822564109591763));
#62534=DIRECTION('ref_axis',(-0.870984468928858,0.161531977910744,-0.463997279083573));
#62535=DIRECTION('center_axis',(0.313150259135956,0.30019266434088,-0.901011253802641));
#62536=DIRECTION('ref_axis',(-0.949703593340092,0.0989839475056044,-0.297094703643677));
#62537=DIRECTION('',(1.,0.,0.));
#62538=DIRECTION('center_axis',(-0.313150259135957,0.30019266434088,-0.901011253802641));
#62539=DIRECTION('ref_axis',(0.949703593340092,0.0989839475056049,-0.297094703643678));
#62540=DIRECTION('center_axis',(-0.491310548314113,0.286360316256975,-0.822564109591764));
#62541=DIRECTION('ref_axis',(0.870984468928858,0.161531977910744,-0.463997279083571));
#62542=DIRECTION('center_axis',(-0.284551435696759,0.301764876373726,-0.909927711321105));
#62543=DIRECTION('ref_axis',(0.958660774436356,0.0895703997751284,-0.270086399215529));
#62544=DIRECTION('center_axis',(0.0617712249622997,0.308682119187541,-0.949157344732972));
#62545=DIRECTION('ref_axis',(-0.998090334472114,0.0191041551727457,-0.0587427909490066));
#62546=DIRECTION('center_axis',(0.99026806874157,0.137058748836224,0.0241671553619711));
#62547=DIRECTION('ref_axis',(-0.139173100960066,0.975223671657125,0.171958245538724));
#62548=DIRECTION('',(1.,0.,0.));
#62549=DIRECTION('center_axis',(0.,-0.309016994374948,0.951056516295154));
#62550=DIRECTION('ref_axis',(1.,0.,0.));
#62551=DIRECTION('',(-0.137844537491629,0.941977614300068,0.306067080296576));
#62552=DIRECTION('center_axis',(-0.99026806874157,-0.137058748836224,-0.0241671553619711));
#62553=DIRECTION('ref_axis',(0.,-0.17364817766693,0.984807753012208));
#62554=DIRECTION('',(-0.137998583506848,0.944481249352984,0.298180416142191));
#62555=DIRECTION('center_axis',(-0.0617712249622997,-0.308682119187541,
0.949157344732972));
#62556=DIRECTION('ref_axis',(0.998052578482889,-0.0108318757168334,0.0614306198252359));
#62557=DIRECTION('',(0.0161503784824051,0.950539749516609,0.310182768482997));
#62558=DIRECTION('center_axis',(0.284551435696759,-0.301764876373726,0.909927711321105));
#62559=DIRECTION('ref_axis',(0.957826285221151,0.0498974366850415,-0.282982425517402));
#62560=DIRECTION('',(0.0552259184163645,0.952749128541176,0.298695825212034));
#62561=DIRECTION('center_axis',(0.491310548314113,-0.286360316256975,0.822564109591764));
#62562=DIRECTION('ref_axis',(0.86824314212446,0.0861536225152694,-0.488601473065054));
#62563=DIRECTION('',(0.057078643955053,0.952962949154956,0.297663645650825));
#62564=DIRECTION('center_axis',(0.313150259135957,-0.30019266434088,0.901011253802641));
#62565=DIRECTION('ref_axis',(0.948683298050513,0.0549123752965087,-0.311423555691114));
#62566=DIRECTION('',(0.0225789275220278,0.950814057294297,0.30893821467004));
#62567=DIRECTION('center_axis',(0.,-0.309016994374947,0.951056516295154));
#62568=DIRECTION('ref_axis',(1.,0.,0.));
#62569=DIRECTION('',(-0.0225789275220274,0.950814057294297,0.30893821467004));
#62570=DIRECTION('center_axis',(-0.313150259135956,-0.30019266434088,0.901011253802641));
#62571=DIRECTION('ref_axis',(0.948683298050514,-0.0549123752965085,0.311423555691113));
#62572=DIRECTION('',(-0.0570786439550527,0.952962949154956,0.297663645650826));
#62573=DIRECTION('center_axis',(-0.491310548314114,-0.286360316256974,0.822564109591763));
#62574=DIRECTION('ref_axis',(0.868243142124459,-0.0861536225152696,0.488601473065055));
#62575=DIRECTION('',(-0.0552259184163635,0.952749128541176,0.298695825212034));
#62576=DIRECTION('center_axis',(-0.284551435696759,-0.301764876373726,0.909927711321104));
#62577=DIRECTION('ref_axis',(0.957826285221151,-0.0498974366850416,0.282982425517402));
#62578=DIRECTION('',(-0.0161503784824052,0.950539749516609,0.310182768482997));
#62579=DIRECTION('center_axis',(0.0617712249622996,-0.308682119187541,0.949157344732972));
#62580=DIRECTION('ref_axis',(0.998052578482889,0.0108318757168334,-0.0614306198252359));
#62581=DIRECTION('',(0.137998583506848,0.944481249352984,0.298180416142191));
#62582=DIRECTION('center_axis',(0.99026806874157,-0.137058748836223,-0.0241671553619711));
#62583=DIRECTION('ref_axis',(0.,0.17364817766693,-0.984807753012208));
#62584=DIRECTION('',(0.137844537491629,0.941977614300068,0.306067080296576));
#62585=DIRECTION('center_axis',(0.,-0.309016994374948,0.951056516295154));
#62586=DIRECTION('ref_axis',(1.,0.,0.));
#62587=DIRECTION('',(-0.0519254248777279,0.949773507937132,0.308600119688995));
#62588=DIRECTION('center_axis',(-0.64930555798837,-0.266892919198654,0.712159014579631));
#62589=DIRECTION('ref_axis',(0.755033118392644,-0.113858792838765,0.645725301830105));
#62590=DIRECTION('center_axis',(0.,0.034899496702501,-0.999390827019096));
#62591=DIRECTION('ref_axis',(-1.,0.,0.));
#62592=DIRECTION('',(-1.,0.,0.));
#62593=DIRECTION('',(0.137844537491629,0.989850519773593,0.0345663418323004));
#62594=DIRECTION('center_axis',(0.99026806874157,-0.137058748836223,-0.0241671553619711));
#62595=DIRECTION('ref_axis',(0.,0.17364817766693,-0.984807753012208));
#62596=DIRECTION('center_axis',(-0.99026806874157,0.137058748836223,0.0241671553619711));
#62597=DIRECTION('ref_axis',(0.139173100960065,0.975223671657125,0.171958245538723));
#62598=DIRECTION('',(0.137998583506848,0.989505769153514,0.0428336755604258));
#62599=DIRECTION('center_axis',(0.0617712249622996,0.0345646215150941,-0.997491655456914));
#62600=DIRECTION('ref_axis',(-0.998052578482889,0.0108318757168334,-0.0614306198252359));
#62601=DIRECTION('center_axis',(-0.0617712249622996,-0.0345646215150941,
0.997491655456914));
#62602=DIRECTION('ref_axis',(-0.998090334472114,0.0021391841375509,-0.061734173069449));
#62603=DIRECTION('',(-0.0161503784824054,0.999303943318151,0.0336272827279996));
#62604=DIRECTION('center_axis',(-0.284551435696759,0.0276473787012795,-0.958262022045047));
#62605=DIRECTION('ref_axis',(-0.957826285221151,-0.0498974366850416,0.282982425517402));
#62606=DIRECTION('center_axis',(0.284551435696759,-0.0276473787012795,0.958262022045047));
#62607=DIRECTION('ref_axis',(0.958660774436356,0.00820634526047709,-0.284433077286297));
#62608=DIRECTION('',(-0.0552259184163638,0.997451314500147,0.045177130685753));
#62609=DIRECTION('center_axis',(-0.491310548314114,0.0122428185845279,-0.870898420315705));
#62610=DIRECTION('ref_axis',(-0.868243142124459,-0.0861536225152696,0.488601473065055));
#62611=DIRECTION('center_axis',(0.491310548314114,-0.0122428185845279,0.870898420315705));
#62612=DIRECTION('ref_axis',(0.870984468928858,0.00690600823120529,-0.491262009456284));
#62613=DIRECTION('',(-0.0570786439550532,0.997299213951626,0.0462201931597183));
#62614=DIRECTION('center_axis',(-0.313150259135956,0.0260751666684337,-0.949345564526583));
#62615=DIRECTION('ref_axis',(-0.948683298050514,-0.0549123752965085,0.311423555691113));
#62616=DIRECTION('center_axis',(0.313150259135956,-0.0260751666684337,0.949345564526583));
#62617=DIRECTION('ref_axis',(0.949703593340092,0.00859788807423116,-0.313032204601347));
#62618=DIRECTION('',(-0.0225789275220273,0.999136045839184,0.0348905995476465));
#62619=DIRECTION('center_axis',(0.,0.034899496702501,-0.999390827019096));
#62620=DIRECTION('ref_axis',(-1.,0.,0.));
#62621=DIRECTION('',(-1.,0.,0.));
#62622=DIRECTION('',(0.0225789275220281,0.999136045839184,0.0348905995476465));
#62623=DIRECTION('center_axis',(0.313150259135957,0.0260751666684335,-0.949345564526583));
#62624=DIRECTION('ref_axis',(-0.948683298050513,0.0549123752965087,-0.311423555691114));
#62625=DIRECTION('center_axis',(-0.313150259135957,-0.0260751666684335,
0.949345564526583));
#62626=DIRECTION('ref_axis',(-0.949703593340092,0.00859788807423112,-0.313032204601348));
#62627=DIRECTION('',(0.0570786439550533,0.997299213951626,0.0462201931597181));
#62628=DIRECTION('center_axis',(0.491310548314113,0.0122428185845279,-0.870898420315706));
#62629=DIRECTION('ref_axis',(-0.86824314212446,0.0861536225152694,-0.488601473065054));
#62630=DIRECTION('center_axis',(-0.491310548314113,-0.0122428185845279,
0.870898420315706));
#62631=DIRECTION('ref_axis',(-0.870984468928858,0.00690600823120516,-0.491262009456283));
#62632=DIRECTION('',(0.0552259184163649,0.997451314500147,0.0451771306857534));
#62633=DIRECTION('center_axis',(0.284551435696759,0.0276473787012796,-0.958262022045047));
#62634=DIRECTION('ref_axis',(-0.957826285221151,0.0498974366850415,-0.282982425517402));
#62635=DIRECTION('center_axis',(-0.284551435696759,-0.0276473787012796,
0.958262022045047));
#62636=DIRECTION('ref_axis',(-0.958660774436356,0.00820634526047708,-0.284433077286297));
#62637=DIRECTION('',(0.016150378482405,0.999303943318151,0.0336272827279996));
#62638=DIRECTION('center_axis',(-0.0617712249622997,0.0345646215150941,
-0.997491655456914));
#62639=DIRECTION('ref_axis',(-0.998052578482889,-0.0108318757168334,0.0614306198252359));
#62640=DIRECTION('center_axis',(0.0617712249622997,-0.0345646215150941,
0.997491655456914));
#62641=DIRECTION('ref_axis',(0.998090334472114,0.0021391841375509,-0.061734173069449));
#62642=DIRECTION('',(-0.137998583506848,0.989505769153514,0.0428336755604258));
#62643=DIRECTION('center_axis',(-0.99026806874157,-0.137058748836224,-0.0241671553619711));
#62644=DIRECTION('ref_axis',(0.,-0.17364817766693,0.984807753012208));
#62645=DIRECTION('center_axis',(0.99026806874157,0.137058748836224,0.0241671553619711));
#62646=DIRECTION('ref_axis',(-0.139173100960066,0.975223671657125,0.171958245538724));
#62647=DIRECTION('',(-0.137844537491629,0.989850519773593,0.0345663418323003));
#62648=DIRECTION('center_axis',(0.,0.0348994967025009,-0.999390827019096));
#62649=DIRECTION('ref_axis',(-1.,0.,0.));
#62650=DIRECTION('',(-1.,0.,0.));
#62651=DIRECTION('center_axis',(0.,0.984807753012208,0.17364817766693));
#62652=DIRECTION('ref_axis',(1.,0.,0.));
#62653=DIRECTION('center_axis',(1.,0.,0.));
#62654=DIRECTION('ref_axis',(0.,1.,0.));
#62655=DIRECTION('center_axis',(1.,0.,0.));
#62656=DIRECTION('ref_axis',(0.,0.,-1.));
#62657=DIRECTION('center_axis',(0.649305557988371,0.139173100960065,-0.747685187986609));
#62658=DIRECTION('ref_axis',(-0.760527640763576,0.118819965419165,-0.638341228068795));
#62659=DIRECTION('',(1.,0.,0.));
#62660=DIRECTION('center_axis',(-0.99026806874157,0.139173100960065,0.));
#62661=DIRECTION('ref_axis',(0.139173100960065,0.99026806874157,0.));
#62662=DIRECTION('center_axis',(-0.0617712249622996,0.139173100960065,-0.988339599396795));
#62663=DIRECTION('ref_axis',(0.998090334472114,0.00861334152950385,-0.0611677576917705));
#62664=DIRECTION('center_axis',(0.284551435696759,0.139173100960065,-0.948504785655862));
#62665=DIRECTION('ref_axis',(-0.958660774436356,0.0413096131025498,-0.281536916624453));
#62666=DIRECTION('center_axis',(0.491310548314114,0.139173100960065,-0.859793459549701));
#62667=DIRECTION('ref_axis',(-0.870984468928858,0.0785056622506209,-0.484997851417207));
#62668=DIRECTION('center_axis',(0.313150259135956,0.139173100960065,-0.939450777407866));
#62669=DIRECTION('ref_axis',(-0.949703593340092,0.0458902050450515,-0.309769549629784));
#62670=DIRECTION('',(1.,0.,0.));
#62671=DIRECTION('center_axis',(-0.313150259135957,0.139173100960066,-0.939450777407865));
#62672=DIRECTION('ref_axis',(0.949703593340092,0.0458902050450517,-0.309769549629785));
#62673=DIRECTION('center_axis',(-0.491310548314113,0.139173100960066,-0.859793459549702));
#62674=DIRECTION('ref_axis',(0.870984468928858,0.0785056622506207,-0.484997851417206));
#62675=DIRECTION('center_axis',(-0.284551435696759,0.139173100960065,-0.948504785655862));
#62676=DIRECTION('ref_axis',(0.958660774436356,0.0413096131025497,-0.281536916624453));
#62677=DIRECTION('center_axis',(0.0617712249622997,0.139173100960065,-0.988339599396795));
#62678=DIRECTION('ref_axis',(-0.998090334472114,0.00861334152950385,-0.0611677576917706));
#62679=DIRECTION('center_axis',(0.99026806874157,0.139173100960066,0.));
#62680=DIRECTION('ref_axis',(-0.139173100960066,0.99026806874157,0.));
#62681=DIRECTION('',(1.,0.,0.));
#62682=DIRECTION('center_axis',(0.,-0.139173100960065,-0.99026806874157));
#62683=DIRECTION('ref_axis',(-1.,0.,0.));
#62684=DIRECTION('',(-1.,0.,0.));
#62685=DIRECTION('',(0.137844537491629,0.980814848463989,-0.137844537491629));
#62686=DIRECTION('center_axis',(0.99026806874157,-0.139173100960065,0.));
#62687=DIRECTION('ref_axis',(0.,0.,-1.));
#62688=DIRECTION('center_axis',(-0.99026806874157,0.139173100960065,0.));
#62689=DIRECTION('ref_axis',(0.139173100960065,0.99026806874157,0.));
#62690=DIRECTION('',(0.137998583506848,0.981910942816534,-0.129642937822505));
#62691=DIRECTION('center_axis',(0.0617712249622996,-0.139173100960065,-0.988339599396795));
#62692=DIRECTION('ref_axis',(-0.998052578482889,0.,-0.0623782861551805));
#62693=DIRECTION('center_axis',(-0.0617712249622996,0.139173100960065,0.988339599396795));
#62694=DIRECTION('ref_axis',(0.998090334472114,0.00861334152950385,0.0611677576917705));
#62695=DIRECTION('',(-0.0161503784824054,0.989961587360995,-0.140410899949307));
#62696=DIRECTION('center_axis',(-0.284551435696759,-0.139173100960066,-0.948504785655862));
#62697=DIRECTION('ref_axis',(-0.957826285221151,0.,0.287347885566346));
#62698=DIRECTION('center_axis',(0.284551435696759,0.139173100960066,0.948504785655862));
#62699=DIRECTION('ref_axis',(-0.958660774436356,0.0413096131025498,0.281536916624453));
#62700=DIRECTION('',(-0.0552259184163638,0.990142714187765,-0.128714814516259));
#62701=DIRECTION('center_axis',(-0.491310548314114,-0.139173100960065,-0.859793459549701));
#62702=DIRECTION('ref_axis',(-0.868243142124459,0.,0.496138938356833));
#62703=DIRECTION('center_axis',(0.491310548314114,0.139173100960065,0.859793459549701));
#62704=DIRECTION('ref_axis',(-0.870984468928858,0.0785056622506209,0.484997851417207));
#62705=DIRECTION('',(-0.0570786439550532,0.99017405028614,-0.12766118652195));
#62706=DIRECTION('center_axis',(-0.313150259135956,-0.139173100960065,-0.939450777407866));
#62707=DIRECTION('ref_axis',(-0.948683298050514,0.,0.316227766016839));
#62708=DIRECTION('center_axis',(0.313150259135956,0.139173100960065,0.939450777407866));
#62709=DIRECTION('ref_axis',(-0.949703593340092,0.0458902050450514,0.309769549629784));
#62710=DIRECTION('',(-0.0225789275220273,0.990015613285545,-0.13913762065955));
#62711=DIRECTION('center_axis',(0.,-0.139173100960065,-0.99026806874157));
#62712=DIRECTION('ref_axis',(-1.,0.,0.));
#62713=DIRECTION('',(-1.,0.,0.));
#62714=DIRECTION('',(0.0225789275220281,0.990015613285545,-0.13913762065955));
#62715=DIRECTION('center_axis',(0.313150259135957,-0.139173100960066,-0.939450777407865));
#62716=DIRECTION('ref_axis',(-0.948683298050513,0.,-0.31622776601684));
#62717=DIRECTION('center_axis',(-0.313150259135957,0.139173100960066,0.939450777407865));
#62718=DIRECTION('ref_axis',(0.949703593340092,0.0458902050450518,0.309769549629785));
#62719=DIRECTION('',(0.0570786439550534,0.99017405028614,-0.12766118652195));
#62720=DIRECTION('center_axis',(0.491310548314113,-0.139173100960066,-0.859793459549702));
#62721=DIRECTION('ref_axis',(-0.86824314212446,0.,-0.496138938356832));
#62722=DIRECTION('center_axis',(-0.491310548314113,0.139173100960066,0.859793459549702));
#62723=DIRECTION('ref_axis',(0.870984468928858,0.0785056622506208,0.484997851417206));
#62724=DIRECTION('',(0.0552259184163649,0.990142714187765,-0.128714814516259));
#62725=DIRECTION('center_axis',(0.284551435696759,-0.139173100960065,-0.948504785655862));
#62726=DIRECTION('ref_axis',(-0.957826285221151,0.,-0.287347885566345));
#62727=DIRECTION('center_axis',(-0.284551435696759,0.139173100960065,0.948504785655862));
#62728=DIRECTION('ref_axis',(0.958660774436356,0.0413096131025497,0.281536916624453));
#62729=DIRECTION('',(0.0161503784824051,0.989961587360995,-0.140410899949307));
#62730=DIRECTION('center_axis',(-0.0617712249622997,-0.139173100960065,
-0.988339599396795));
#62731=DIRECTION('ref_axis',(-0.998052578482889,0.,0.0623782861551806));
#62732=DIRECTION('center_axis',(0.0617712249622997,0.139173100960065,0.988339599396795));
#62733=DIRECTION('ref_axis',(-0.998090334472114,0.00861334152950385,0.0611677576917706));
#62734=DIRECTION('',(-0.137998583506848,0.981910942816533,-0.129642937822505));
#62735=DIRECTION('center_axis',(-0.99026806874157,-0.139173100960066,0.));
#62736=DIRECTION('ref_axis',(0.,0.,1.));
#62737=DIRECTION('center_axis',(0.99026806874157,0.139173100960066,0.));
#62738=DIRECTION('ref_axis',(-0.139173100960066,0.99026806874157,0.));
#62739=DIRECTION('',(-0.137844537491629,0.980814848463989,-0.137844537491629));
#62740=DIRECTION('center_axis',(0.,-0.139173100960065,-0.99026806874157));
#62741=DIRECTION('ref_axis',(-1.,0.,0.));
#62742=DIRECTION('',(-1.,0.,0.));
#62743=DIRECTION('',(0.0519254248777275,0.98893216263388,-0.138985351600607));
#62744=DIRECTION('center_axis',(0.649305557988371,-0.139173100960065,-0.747685187986609));
#62745=DIRECTION('ref_axis',(-0.755033118392643,0.,-0.655686655446243));
#62746=DIRECTION('center_axis',(-0.649305557988371,0.139173100960065,0.747685187986609));
#62747=DIRECTION('ref_axis',(0.760527640763576,0.118819965419165,0.638341228068795));
#62748=DIRECTION('center_axis',(0.,-0.139173100960066,0.99026806874157));
#62749=DIRECTION('ref_axis',(1.,0.,0.));
#62750=DIRECTION('',(-0.137844537491629,0.980814848463989,0.137844537491629));
#62751=DIRECTION('center_axis',(-0.99026806874157,-0.139173100960066,0.));
#62752=DIRECTION('ref_axis',(0.,0.,1.));
#62753=DIRECTION('',(-0.137998583506848,0.981910942816533,0.129642937822505));
#62754=DIRECTION('center_axis',(-0.0617712249622997,-0.139173100960065,
0.988339599396795));
#62755=DIRECTION('ref_axis',(0.998052578482889,0.,0.0623782861551806));
#62756=DIRECTION('',(0.0161503784824051,0.989961587360995,0.140410899949307));
#62757=DIRECTION('center_axis',(0.284551435696759,-0.139173100960065,0.948504785655862));
#62758=DIRECTION('ref_axis',(0.957826285221151,0.,-0.287347885566345));
#62759=DIRECTION('',(0.0552259184163645,0.990142714187765,0.128714814516259));
#62760=DIRECTION('center_axis',(0.491310548314113,-0.139173100960066,0.859793459549702));
#62761=DIRECTION('ref_axis',(0.86824314212446,0.,-0.496138938356832));
#62762=DIRECTION('',(0.057078643955053,0.99017405028614,0.12766118652195));
#62763=DIRECTION('center_axis',(0.313150259135957,-0.139173100960066,0.939450777407865));
#62764=DIRECTION('ref_axis',(0.948683298050513,0.,-0.31622776601684));
#62765=DIRECTION('',(0.0225789275220278,0.990015613285545,0.139137620659551));
#62766=DIRECTION('center_axis',(0.,-0.139173100960065,0.99026806874157));
#62767=DIRECTION('ref_axis',(1.,0.,0.));
#62768=DIRECTION('',(-0.0225789275220274,0.990015613285545,0.139137620659551));
#62769=DIRECTION('center_axis',(-0.313150259135956,-0.139173100960065,0.939450777407866));
#62770=DIRECTION('ref_axis',(0.948683298050514,0.,0.316227766016839));
#62771=DIRECTION('',(-0.0570786439550527,0.99017405028614,0.12766118652195));
#62772=DIRECTION('center_axis',(-0.491310548314114,-0.139173100960065,0.859793459549701));
#62773=DIRECTION('ref_axis',(0.868243142124459,0.,0.496138938356833));
#62774=DIRECTION('',(-0.0552259184163635,0.990142714187765,0.12871481451626));
#62775=DIRECTION('center_axis',(-0.284551435696759,-0.139173100960065,0.948504785655862));
#62776=DIRECTION('ref_axis',(0.957826285221151,0.,0.287347885566346));
#62777=DIRECTION('',(-0.0161503784824052,0.989961587360995,0.140410899949307));
#62778=DIRECTION('center_axis',(0.0617712249622996,-0.139173100960065,0.988339599396795));
#62779=DIRECTION('ref_axis',(0.998052578482889,0.,-0.0623782861551805));
#62780=DIRECTION('',(0.137998583506848,0.981910942816534,0.129642937822505));
#62781=DIRECTION('center_axis',(0.99026806874157,-0.139173100960065,0.));
#62782=DIRECTION('ref_axis',(0.,0.,-1.));
#62783=DIRECTION('',(0.137844537491629,0.980814848463989,0.137844537491629));
#62784=DIRECTION('center_axis',(0.,-0.139173100960065,0.99026806874157));
#62785=DIRECTION('ref_axis',(1.,0.,0.));
#62786=DIRECTION('',(-0.051925424877728,0.98893216263388,0.138985351600607));
#62787=DIRECTION('center_axis',(-0.649305557988371,-0.139173100960065,0.747685187986609));
#62788=DIRECTION('ref_axis',(0.755033118392644,0.,0.655686655446243));
#62789=DIRECTION('center_axis',(-1.,0.,0.));
#62790=DIRECTION('ref_axis',(0.,1.,0.));
#62791=DIRECTION('center_axis',(1.,0.,0.));
#62792=DIRECTION('ref_axis',(0.,0.,-1.));
#62793=DIRECTION('',(-0.707106781186545,-0.70710678118655,-8.65956056235497E-17));
#62794=DIRECTION('center_axis',(1.,0.,0.));
#62795=DIRECTION('ref_axis',(0.,0.,-1.));
#62796=DIRECTION('center_axis',(-1.,0.,-7.72527832197503E-15));
#62797=DIRECTION('ref_axis',(0.,-1.,-3.07881506165609E-17));
#62798=DIRECTION('center_axis',(-1.,0.,0.));
#62799=DIRECTION('ref_axis',(0.,-1.,0.));
#62800=DIRECTION('',(-0.57864046491405,0.815582744032788,-4.34516827576256E-15));
#62801=DIRECTION('center_axis',(1.,0.,0.));
#62802=DIRECTION('ref_axis',(0.,-1.,-6.12323399573677E-17));
#62803=DIRECTION('center_axis',(1.,0.,0.));
#62804=DIRECTION('ref_axis',(0.,-1.,-6.12323399573677E-17));
#62805=DIRECTION('center_axis',(-1.,0.,0.));
#62806=DIRECTION('ref_axis',(0.,1.,0.));
#62807=DIRECTION('',(-0.943858356366018,-0.330350424728106,-4.04562590240243E-17));
#62808=DIRECTION('center_axis',(-1.,0.,0.));
#62809=DIRECTION('ref_axis',(0.,-1.,3.06161699786838E-17));
#62810=DIRECTION('center_axis',(-1.,0.,0.));
#62811=DIRECTION('ref_axis',(0.,-1.,3.06161699786838E-17));
#62812=DIRECTION('center_axis',(1.,0.,0.));
#62813=DIRECTION('ref_axis',(0.,0.,-1.));
#62814=DIRECTION('center_axis',(1.,0.,0.));
#62815=DIRECTION('ref_axis',(0.,0.,-1.));
#62816=DIRECTION('center_axis',(0.,-1.,-1.22464679914735E-16));
#62817=DIRECTION('ref_axis',(0.,-1.22464679914735E-16,1.));
#62818=DIRECTION('center_axis',(1.,0.,0.));
#62819=DIRECTION('ref_axis',(0.,-1.,1.83697019872103E-16));
#62820=DIRECTION('center_axis',(1.,0.,0.));
#62821=DIRECTION('ref_axis',(0.,-1.,1.83697019872103E-16));
#62822=DIRECTION('center_axis',(1.,0.,0.));
#62823=DIRECTION('ref_axis',(0.,1.,0.));
#62824=DIRECTION('',(-1.,0.,0.));
#62825=DIRECTION('center_axis',(1.,0.,0.));
#62826=DIRECTION('ref_axis',(0.,0.,-1.));
#62827=DIRECTION('center_axis',(1.,0.,0.));
#62828=DIRECTION('ref_axis',(0.,0.,-1.));
#62829=DIRECTION('center_axis',(1.,0.,0.));
#62830=DIRECTION('ref_axis',(0.,-1.,1.83697019872103E-16));
#62831=DIRECTION('center_axis',(0.,-1.,-1.22464679914735E-16));
#62832=DIRECTION('ref_axis',(0.,-1.22464679914735E-16,1.));
#62833=DIRECTION('center_axis',(-1.,0.,0.));
#62834=DIRECTION('ref_axis',(0.,-1.,1.83697019872103E-16));
#62835=DIRECTION('center_axis',(1.,0.,0.));
#62836=DIRECTION('ref_axis',(0.,-1.,1.83697019872103E-16));
#62837=DIRECTION('center_axis',(1.,0.,0.));
#62838=DIRECTION('ref_axis',(0.,1.,0.));
#62839=DIRECTION('',(-1.,0.,0.));
#62840=DIRECTION('center_axis',(-1.,0.,0.));
#62841=DIRECTION('ref_axis',(0.,-1.,1.83697019872103E-16));
#62842=DIRECTION('center_axis',(-1.,0.,0.));
#62843=DIRECTION('ref_axis',(0.,-1.,1.83697019872103E-16));
#62844=DIRECTION('center_axis',(-1.,0.,0.));
#62845=DIRECTION('ref_axis',(0.,0.,1.));
#62846=DIRECTION('center_axis',(1.,0.,0.));
#62847=DIRECTION('ref_axis',(0.,0.,-1.));
#62848=DIRECTION('center_axis',(1.,0.,0.));
#62849=DIRECTION('ref_axis',(0.,0.,-1.));
#62850=DIRECTION('center_axis',(1.,0.,0.));
#62851=DIRECTION('ref_axis',(0.,-1.,1.83697019872103E-16));
#62852=DIRECTION('center_axis',(0.,-1.,-1.22464679914735E-16));
#62853=DIRECTION('ref_axis',(0.,-1.22464679914735E-16,1.));
#62854=DIRECTION('center_axis',(1.,0.,0.));
#62855=DIRECTION('ref_axis',(0.,0.,-1.));
#62856=DIRECTION('center_axis',(1.,0.,0.));
#62857=DIRECTION('ref_axis',(0.,0.,-1.));
#62858=DIRECTION('center_axis',(1.,0.,0.));
#62859=DIRECTION('ref_axis',(0.,1.,0.));
#62860=DIRECTION('center_axis',(-1.,0.,0.));
#62861=DIRECTION('ref_axis',(0.,0.,1.));
#62862=DIRECTION('center_axis',(1.,0.,0.));
#62863=DIRECTION('ref_axis',(0.,0.,-1.));
#62864=DIRECTION('center_axis',(1.,0.,0.));
#62865=DIRECTION('ref_axis',(0.,1.,0.));
#62866=DIRECTION('center_axis',(1.,0.,0.));
#62867=DIRECTION('ref_axis',(0.,0.,-1.));
#62868=DIRECTION('',(-0.707106781186551,0.707106781186544,8.65956056235489E-17));
#62869=DIRECTION('center_axis',(1.,0.,0.));
#62870=DIRECTION('ref_axis',(0.,1.,0.));
#62871=DIRECTION('center_axis',(1.,0.,0.));
#62872=DIRECTION('ref_axis',(0.,0.,-1.));
#62873=DIRECTION('',(-1.,0.,0.));
#62874=DIRECTION('center_axis',(-1.,0.,0.));
#62875=DIRECTION('ref_axis',(0.,1.,0.));
#62876=DIRECTION('',(-0.707106781186549,-0.707106781186546,-8.65956056235492E-17));
#62877=DIRECTION('center_axis',(1.,0.,0.));
#62878=DIRECTION('ref_axis',(0.,1.,0.));
#62879=DIRECTION('center_axis',(1.,0.,0.));
#62880=DIRECTION('ref_axis',(0.,0.,-1.));
#62881=DIRECTION('',(-1.,0.,0.));
#62882=DIRECTION('center_axis',(1.,0.,0.));
#62883=DIRECTION('ref_axis',(0.,1.,0.));
#62884=DIRECTION('',(-0.447213595499961,0.894427190999915,1.0953573965284E-16));
#68259=CARTESIAN_POINT('',(0.,0.,0.));
#68260=CARTESIAN_POINT('Origin',(34.2,0.,0.));
#68261=CARTESIAN_POINT('',(35.,39.0489657041002,-6.5831814071929));
#68262=CARTESIAN_POINT('',(35.,38.9456055698919,-7.16936585720129));
#68263=CARTESIAN_POINT('Origin',(35.,0.,0.));
#68264=CARTESIAN_POINT('',(33.4246193974437,37.6602615890763,-5.25132148728276));
#68265=CARTESIAN_POINT('Ctrl Pts',(33.4246193974437,37.6602615890763,-5.25132148728276));
#68266=CARTESIAN_POINT('Ctrl Pts',(34.1981589442507,38.350106913703,-5.90521241418151));
#68267=CARTESIAN_POINT('Ctrl Pts',(35.,39.0489657041002,-6.5831814071929));
#68268=CARTESIAN_POINT('',(33.4246193974437,37.1851276398516,-7.94594001540395));
#68269=CARTESIAN_POINT('Ctrl Pts',(33.4246193974437,37.1851276398516,-7.94594001540396));
#68270=CARTESIAN_POINT('Ctrl Pts',(33.3753965426192,37.4226946144693,-6.59863075131265));
#68271=CARTESIAN_POINT('Ctrl Pts',(33.4246193974437,37.6602615890763,-5.25132148728276));
#68272=CARTESIAN_POINT('Ctrl Pts',(35.,38.9456055698919,-7.1693658572013));
#68273=CARTESIAN_POINT('Ctrl Pts',(34.1981589442511,38.0570140694247,-7.56742453339956));
#68274=CARTESIAN_POINT('Ctrl Pts',(33.4246193974437,37.1851276398516,-7.94594001540395));
#68275=CARTESIAN_POINT('Origin',(34.2,0.,0.));
#68276=CARTESIAN_POINT('',(35.,37.3125667178958,-13.2639498235849));
#68277=CARTESIAN_POINT('',(35.,37.1089869948545,-13.8232805156997));
#68278=CARTESIAN_POINT('Origin',(35.,0.,0.));
#68279=CARTESIAN_POINT('',(33.4246193974437,36.1762351867803,-11.7111779096387));
#68280=CARTESIAN_POINT('Ctrl Pts',(33.4246193974437,36.1762351867803,-11.7111779096387));
#68281=CARTESIAN_POINT('Ctrl Pts',(34.1981589442499,36.7420532430025,-12.4749251475656));
#68282=CARTESIAN_POINT('Ctrl Pts',(35.,37.3125667178958,-13.2639498235849));
#68283=CARTESIAN_POINT('',(33.4246193974437,35.2404039929487,-14.2823529831122));
#68284=CARTESIAN_POINT('Ctrl Pts',(33.4246193974437,35.2404039929487,-14.2823529831122));
#68285=CARTESIAN_POINT('Ctrl Pts',(33.3753965426192,35.7083195898752,-12.9967654463461));
#68286=CARTESIAN_POINT('Ctrl Pts',(33.4246193974437,36.1762351867803,-11.7111779096387));
#68287=CARTESIAN_POINT('Ctrl Pts',(35.,37.1089869948545,-13.8232805156997));
#68288=CARTESIAN_POINT('Ctrl Pts',(34.1981589442488,36.1647730322046,-14.0609894914277));
#68289=CARTESIAN_POINT('Ctrl Pts',(33.4246193974437,35.2404039929487,-14.2823529831122));
#68290=CARTESIAN_POINT('Origin',(34.2,0.,0.));
#68291=CARTESIAN_POINT('',(35.,34.4424442730379,-19.5416998364696));
#68292=CARTESIAN_POINT('',(35.,34.1448306280319,-20.0571817906459));
#68293=CARTESIAN_POINT('Origin',(35.,0.,0.));
#68294=CARTESIAN_POINT('',(33.4246193974437,33.5930121843923,-17.8151961173521));
#68295=CARTESIAN_POINT('Ctrl Pts',(33.4246193974437,33.5930121843923,-17.8151961173521));
#68296=CARTESIAN_POINT('Ctrl Pts',(34.1981589442498,34.01761087689,-18.6655935929581));
#68297=CARTESIAN_POINT('Ctrl Pts',(35.,34.4424442730379,-19.5416998364696));
#68298=CARTESIAN_POINT('',(33.4246193974437,32.224918503225,-20.1848038826479));
#68299=CARTESIAN_POINT('Ctrl Pts',(33.4246193974437,32.224918503225,-20.1848038826479));
#68300=CARTESIAN_POINT('Ctrl Pts',(33.3753965426192,32.9089653438242,-18.999999999973));
#68301=CARTESIAN_POINT('Ctrl Pts',(33.4246193974437,33.5930121843923,-17.8151961173521));
#68302=CARTESIAN_POINT('Ctrl Pts',(35.,34.1448306280319,-20.0571817906459));
#68303=CARTESIAN_POINT('Ctrl Pts',(34.1981589442497,33.1736836666627,-20.1273183989616));
#68304=CARTESIAN_POINT('Ctrl Pts',(33.4246193974437,32.224918503225,-20.1848038826479));
#68305=CARTESIAN_POINT('Origin',(34.2,0.,0.));
#68306=CARTESIAN_POINT('',(35.,30.5258055876616,-25.2256851884005));
#68307=CARTESIAN_POINT('',(35.,30.1432008606945,-25.6816557463071));
#68308=CARTESIAN_POINT('Origin',(35.,0.,0.));
#68309=CARTESIAN_POINT('',(33.4246193974437,29.989082505666,-23.3779086059641));
#68310=CARTESIAN_POINT('Ctrl Pts',(33.4246193974437,29.989082505666,-23.3779086059641));
#68311=CARTESIAN_POINT('Ctrl Pts',(34.1981589442508,30.2595606180253,-24.2891174222761));
#68312=CARTESIAN_POINT('Ctrl Pts',(35.,30.5258055876616,-25.2256851884005));
#68313=CARTESIAN_POINT('',(33.4246193974437,28.2302951713763,-25.4739497302129));
#68314=CARTESIAN_POINT('Ctrl Pts',(33.4246193974437,28.2302951713763,-25.4739497302129));
#68315=CARTESIAN_POINT('Ctrl Pts',(33.3753965426191,29.1096888385412,-24.4259291680646));
#68316=CARTESIAN_POINT('Ctrl Pts',(33.4246193974437,29.989082505666,-23.3779086059641));
#68317=CARTESIAN_POINT('Ctrl Pts',(35.,30.1432008606945,-25.6816557463071));
#68318=CARTESIAN_POINT('Ctrl Pts',(34.1981589442493,29.1746287096016,-25.5820889218577));
#68319=CARTESIAN_POINT('Ctrl Pts',(33.4246193974437,28.2302951713763,-25.4739497302129));
#68320=CARTESIAN_POINT('Origin',(34.2,0.,0.));
#68321=CARTESIAN_POINT('',(35.,25.6816557463071,-30.1432008606945));
#68322=CARTESIAN_POINT('',(35.,25.2256851884005,-30.5258055876616));
#68323=CARTESIAN_POINT('Origin',(35.,0.,0.));
#68324=CARTESIAN_POINT('',(33.4246193974437,25.4739497302129,-28.2302951713764));
#68325=CARTESIAN_POINT('Ctrl Pts',(33.4246193974437,25.4739497302129,-28.2302951713764));
#68326=CARTESIAN_POINT('Ctrl Pts',(34.198158944251,25.5820889218579,-29.1746287096037));
#68327=CARTESIAN_POINT('Ctrl Pts',(35.,25.6816557463071,-30.1432008606945));
#68328=CARTESIAN_POINT('',(33.4246193974437,23.3779086059641,-29.989082505666));
#68329=CARTESIAN_POINT('Ctrl Pts',(33.4246193974437,23.3779086059641,-29.989082505666));
#68330=CARTESIAN_POINT('Ctrl Pts',(33.3753965426192,24.4259291681124,-29.1096888385011));
#68331=CARTESIAN_POINT('Ctrl Pts',(33.4246193974437,25.4739497302129,-28.2302951713764));
#68332=CARTESIAN_POINT('Ctrl Pts',(35.,25.2256851884005,-30.5258055876616));
#68333=CARTESIAN_POINT('Ctrl Pts',(34.1981589442506,24.2891174222758,-30.2595606180253));
#68334=CARTESIAN_POINT('Ctrl Pts',(33.4246193974437,23.3779086059641,-29.989082505666));
#68335=CARTESIAN_POINT('Origin',(34.2,0.,0.));
#68336=CARTESIAN_POINT('',(35.,20.0571817906459,-34.1448306280319));
#68337=CARTESIAN_POINT('',(35.,19.5416998364696,-34.4424442730379));
#68338=CARTESIAN_POINT('Origin',(35.,0.,0.));
#68339=CARTESIAN_POINT('',(33.4246193974437,20.1848038826479,-32.224918503225));
#68340=CARTESIAN_POINT('Ctrl Pts',(33.4246193974437,20.1848038826479,-32.224918503225));
#68341=CARTESIAN_POINT('Ctrl Pts',(34.1981589442498,20.1273183989615,-33.1736836666628));
#68342=CARTESIAN_POINT('Ctrl Pts',(35.,20.0571817906459,-34.1448306280319));
#68343=CARTESIAN_POINT('',(33.4246193974437,17.8151961173521,-33.5930121843923));
#68344=CARTESIAN_POINT('Ctrl Pts',(33.4246193974437,17.8151961173521,-33.5930121843923));
#68345=CARTESIAN_POINT('Ctrl Pts',(33.3753965426191,19.000000000027,-32.9089653437931));
#68346=CARTESIAN_POINT('Ctrl Pts',(33.4246193974437,20.1848038826479,-32.224918503225));
#68347=CARTESIAN_POINT('Ctrl Pts',(35.,19.5416998364696,-34.4424442730379));
#68348=CARTESIAN_POINT('Ctrl Pts',(34.1981589442509,18.6655935929594,-34.0176108768906));
#68349=CARTESIAN_POINT('Ctrl Pts',(33.4246193974437,17.8151961173521,-33.5930121843923));
#68350=CARTESIAN_POINT('Origin',(34.2,0.,0.));
#68351=CARTESIAN_POINT('',(35.,13.8232805156996,-37.1089869948545));
#68352=CARTESIAN_POINT('',(35.,13.2639498235848,-37.3125667178958));
#68353=CARTESIAN_POINT('Origin',(35.,0.,0.));
#68354=CARTESIAN_POINT('',(33.4246193974437,14.2823529831122,-35.2404039929487));
#68355=CARTESIAN_POINT('Ctrl Pts',(33.4246193974437,14.2823529831122,-35.2404039929487));
#68356=CARTESIAN_POINT('Ctrl Pts',(34.1981589442504,14.0609894914272,-36.1647730322064));
#68357=CARTESIAN_POINT('Ctrl Pts',(35.,13.8232805156996,-37.1089869948545));
#68358=CARTESIAN_POINT('',(33.4246193974437,11.7111779096386,-36.1762351867803));
#68359=CARTESIAN_POINT('Ctrl Pts',(33.4246193974437,11.7111779096386,-36.1762351867803));
#68360=CARTESIAN_POINT('Ctrl Pts',(33.3753965426192,12.9967654464047,-35.7083195898539));
#68361=CARTESIAN_POINT('Ctrl Pts',(33.4246193974437,14.2823529831122,-35.2404039929487));
#68362=CARTESIAN_POINT('Ctrl Pts',(35.,13.2639498235848,-37.3125667178958));
#68363=CARTESIAN_POINT('Ctrl Pts',(34.1981589442509,12.4749251475665,-36.7420532430032));
#68364=CARTESIAN_POINT('Ctrl Pts',(33.4246193974437,11.7111779096386,-36.1762351867803));
#68365=CARTESIAN_POINT('Origin',(34.2,0.,0.));
#68366=CARTESIAN_POINT('',(35.,7.16936585720128,-38.9456055698919));
#68367=CARTESIAN_POINT('',(35.,6.58318140719288,-39.0489657041002));
#68368=CARTESIAN_POINT('Origin',(35.,0.,0.));
#68369=CARTESIAN_POINT('',(33.4246193974437,7.94594001540394,-37.1851276398516));
#68370=CARTESIAN_POINT('Ctrl Pts',(33.4246193974437,7.94594001540394,-37.1851276398516));
#68371=CARTESIAN_POINT('Ctrl Pts',(34.1981589442496,7.56742453340028,-38.057014069423));
#68372=CARTESIAN_POINT('Ctrl Pts',(35.,7.16936585720128,-38.9456055698919));
#68373=CARTESIAN_POINT('',(33.4246193974437,5.25132148728273,-37.6602615890763));
#68374=CARTESIAN_POINT('Ctrl Pts',(33.4246193974437,5.25132148728273,-37.6602615890763));
#68375=CARTESIAN_POINT('Ctrl Pts',(33.3753965426191,6.59863075137404,-37.4226946144585));
#68376=CARTESIAN_POINT('Ctrl Pts',(33.4246193974437,7.94594001540394,-37.1851276398516));
#68377=CARTESIAN_POINT('Ctrl Pts',(35.,6.58318140719289,-39.0489657041002));
#68378=CARTESIAN_POINT('Ctrl Pts',(34.1981589442503,5.90521241418118,-38.3501069137027));
#68379=CARTESIAN_POINT('Ctrl Pts',(33.4246193974437,5.25132148728273,-37.6602615890763));
#68380=CARTESIAN_POINT('Origin',(34.2,0.,0.));
#68381=CARTESIAN_POINT('',(35.,0.297613645006055,-39.5988816271155));
#68382=CARTESIAN_POINT('',(35.,-0.297613645006067,-39.5988816271155));
#68383=CARTESIAN_POINT('Origin',(35.,0.,0.));
#68384=CARTESIAN_POINT('',(33.4246193974437,1.36809368116733,-38.));
#68385=CARTESIAN_POINT('Ctrl Pts',(33.4246193974437,1.36809368116733,-38.));
#68386=CARTESIAN_POINT('Ctrl Pts',(34.1981589442509,0.843927210226466,-38.7929119919208));
#68387=CARTESIAN_POINT('Ctrl Pts',(35.,0.297613645006061,-39.5988816271155));
#68388=CARTESIAN_POINT('',(33.4246193974437,-1.36809368116734,-38.));
#68389=CARTESIAN_POINT('Ctrl Pts',(33.4246193974437,-1.36809368116734,-38.));
#68390=CARTESIAN_POINT('Ctrl Pts',(33.3753965426191,3.11772829775236E-11,
-38.));
#68391=CARTESIAN_POINT('Ctrl Pts',(33.4246193974437,1.36809368116733,-38.));
#68392=CARTESIAN_POINT('Ctrl Pts',(35.,-0.297613645006074,-39.5988816271155));
#68393=CARTESIAN_POINT('Ctrl Pts',(34.1981589442498,-0.843927210227242,
-38.7929119919196));
#68394=CARTESIAN_POINT('Ctrl Pts',(33.4246193974437,-1.36809368116734,-38.));
#68395=CARTESIAN_POINT('Origin',(34.2,0.,0.));
#68396=CARTESIAN_POINT('',(35.,-6.5831814071929,-39.0489657041002));
#68397=CARTESIAN_POINT('',(35.,-7.16936585720129,-38.9456055698919));
#68398=CARTESIAN_POINT('Origin',(35.,0.,0.));
#68399=CARTESIAN_POINT('',(33.4246193974437,-5.25132148728275,-37.6602615890763));
#68400=CARTESIAN_POINT('Ctrl Pts',(33.4246193974437,-5.25132148728275,-37.6602615890763));
#68401=CARTESIAN_POINT('Ctrl Pts',(34.19815894425,-5.90521241418094,-38.3501069137024));
#68402=CARTESIAN_POINT('Ctrl Pts',(35.,-6.5831814071929,-39.0489657041002));
#68403=CARTESIAN_POINT('',(33.4246193974437,-7.94594001540395,-37.1851276398516));
#68404=CARTESIAN_POINT('Ctrl Pts',(33.4246193974437,-7.94594001540395,-37.1851276398516));
#68405=CARTESIAN_POINT('Ctrl Pts',(33.3753965426192,-6.59863075131264,-37.4226946144693));
#68406=CARTESIAN_POINT('Ctrl Pts',(33.4246193974437,-5.25132148728275,-37.6602615890763));
#68407=CARTESIAN_POINT('Ctrl Pts',(35.,-7.16936585720129,-38.9456055698919));
#68408=CARTESIAN_POINT('Ctrl Pts',(34.1981589442516,-7.56742453339929,-38.0570140694253));
#68409=CARTESIAN_POINT('Ctrl Pts',(33.4246193974437,-7.94594001540395,-37.1851276398516));
#68410=CARTESIAN_POINT('Origin',(34.2,0.,0.));
#68411=CARTESIAN_POINT('',(35.,-13.2639498235849,-37.3125667178958));
#68412=CARTESIAN_POINT('',(35.,-13.8232805156997,-37.1089869948545));
#68413=CARTESIAN_POINT('Origin',(35.,0.,0.));
#68414=CARTESIAN_POINT('',(33.4246193974437,-11.7111779096387,-36.1762351867803));
#68415=CARTESIAN_POINT('Ctrl Pts',(33.4246193974437,-11.7111779096387,-36.1762351867803));
#68416=CARTESIAN_POINT('Ctrl Pts',(34.1981589442511,-12.4749251475667,-36.7420532430033));
#68417=CARTESIAN_POINT('Ctrl Pts',(35.,-13.2639498235849,-37.3125667178958));
#68418=CARTESIAN_POINT('',(33.4246193974437,-14.2823529831122,-35.2404039929487));
#68419=CARTESIAN_POINT('Ctrl Pts',(33.4246193974437,-14.2823529831122,-35.2404039929487));
#68420=CARTESIAN_POINT('Ctrl Pts',(33.3753965426192,-12.9967654463461,-35.7083195898752));
#68421=CARTESIAN_POINT('Ctrl Pts',(33.4246193974437,-11.7111779096387,-36.1762351867803));
#68422=CARTESIAN_POINT('Ctrl Pts',(35.,-13.8232805156997,-37.1089869948545));
#68423=CARTESIAN_POINT('Ctrl Pts',(34.1981589442496,-14.0609894914275,-36.1647730322054));
#68424=CARTESIAN_POINT('Ctrl Pts',(33.4246193974437,-14.2823529831122,-35.2404039929487));
#68425=CARTESIAN_POINT('Origin',(34.2,0.,0.));
#68426=CARTESIAN_POINT('',(35.,-19.5416998364696,-34.4424442730379));
#68427=CARTESIAN_POINT('',(35.,-20.0571817906459,-34.1448306280318));
#68428=CARTESIAN_POINT('Origin',(35.,0.,0.));
#68429=CARTESIAN_POINT('',(33.4246193974437,-17.8151961173521,-33.5930121843923));
#68430=CARTESIAN_POINT('Ctrl Pts',(33.4246193974437,-17.8151961173521,-33.5930121843923));
#68431=CARTESIAN_POINT('Ctrl Pts',(34.1981589442509,-18.6655935929594,-34.0176108768906));
#68432=CARTESIAN_POINT('Ctrl Pts',(35.,-19.5416998364696,-34.4424442730379));
#68433=CARTESIAN_POINT('',(33.4246193974437,-20.1848038826479,-32.224918503225));
#68434=CARTESIAN_POINT('Ctrl Pts',(33.4246193974437,-20.1848038826479,-32.224918503225));
#68435=CARTESIAN_POINT('Ctrl Pts',(33.3753965426192,-18.999999999973,-32.9089653438242));
#68436=CARTESIAN_POINT('Ctrl Pts',(33.4246193974437,-17.8151961173521,-33.5930121843923));
#68437=CARTESIAN_POINT('Ctrl Pts',(35.,-20.0571817906459,-34.1448306280319));
#68438=CARTESIAN_POINT('Ctrl Pts',(34.1981589442493,-20.1273183989616,-33.1736836666622));
#68439=CARTESIAN_POINT('Ctrl Pts',(33.4246193974437,-20.1848038826479,-32.224918503225));
#68440=CARTESIAN_POINT('Origin',(34.2,0.,0.));
#68441=CARTESIAN_POINT('',(35.,-25.2256851884005,-30.5258055876616));
#68442=CARTESIAN_POINT('',(35.,-25.6816557463071,-30.1432008606945));
#68443=CARTESIAN_POINT('Origin',(35.,0.,0.));
#68444=CARTESIAN_POINT('',(33.4246193974437,-23.3779086059641,-29.989082505666));
#68445=CARTESIAN_POINT('Ctrl Pts',(33.4246193974437,-23.3779086059641,-29.989082505666));
#68446=CARTESIAN_POINT('Ctrl Pts',(34.1981589442511,-24.2891174222764,-30.2595606180254));
#68447=CARTESIAN_POINT('Ctrl Pts',(35.,-25.2256851884005,-30.5258055876616));
#68448=CARTESIAN_POINT('',(33.4246193974437,-25.4739497302129,-28.2302951713763));
#68449=CARTESIAN_POINT('Ctrl Pts',(33.4246193974437,-25.4739497302129,-28.2302951713763));
#68450=CARTESIAN_POINT('Ctrl Pts',(33.3753965426191,-24.4259291680646,-29.1096888385412));
#68451=CARTESIAN_POINT('Ctrl Pts',(33.4246193974437,-23.3779086059641,-29.989082505666));
#68452=CARTESIAN_POINT('Ctrl Pts',(35.,-25.6816557463071,-30.1432008606945));
#68453=CARTESIAN_POINT('Ctrl Pts',(34.1981589442511,-25.582088921858,-29.1746287096039));
#68454=CARTESIAN_POINT('Ctrl Pts',(33.4246193974437,-25.4739497302129,-28.2302951713763));
#68455=CARTESIAN_POINT('Origin',(34.2,0.,0.));
#68456=CARTESIAN_POINT('',(35.,-30.1432008606945,-25.6816557463071));
#68457=CARTESIAN_POINT('',(35.,-30.5258055876616,-25.2256851884005));
#68458=CARTESIAN_POINT('Origin',(35.,0.,0.));
#68459=CARTESIAN_POINT('',(33.4246193974437,-28.2302951713764,-25.4739497302129));
#68460=CARTESIAN_POINT('Ctrl Pts',(33.4246193974437,-28.2302951713764,-25.4739497302129));
#68461=CARTESIAN_POINT('Ctrl Pts',(34.1981589442485,-29.1746287096007,-25.5820889218576));
#68462=CARTESIAN_POINT('Ctrl Pts',(35.,-30.1432008606945,-25.6816557463071));
#68463=CARTESIAN_POINT('',(33.4246193974437,-29.989082505666,-23.3779086059641));
#68464=CARTESIAN_POINT('Ctrl Pts',(33.4246193974437,-29.989082505666,-23.3779086059641));
#68465=CARTESIAN_POINT('Ctrl Pts',(33.3753965426192,-29.1096888385011,-24.4259291681124));
#68466=CARTESIAN_POINT('Ctrl Pts',(33.4246193974437,-28.2302951713764,-25.4739497302129));
#68467=CARTESIAN_POINT('Ctrl Pts',(35.,-30.5258055876616,-25.2256851884005));
#68468=CARTESIAN_POINT('Ctrl Pts',(34.1981589442495,-30.2595606180249,-24.2891174222746));
#68469=CARTESIAN_POINT('Ctrl Pts',(33.4246193974437,-29.989082505666,-23.3779086059641));
#68470=CARTESIAN_POINT('Origin',(34.2,0.,0.));
#68471=CARTESIAN_POINT('',(35.,-34.1448306280319,-20.0571817906459));
#68472=CARTESIAN_POINT('',(35.,-34.4424442730379,-19.5416998364696));
#68473=CARTESIAN_POINT('Origin',(35.,0.,0.));
#68474=CARTESIAN_POINT('',(33.4246193974437,-32.224918503225,-20.1848038826479));
#68475=CARTESIAN_POINT('Ctrl Pts',(33.4246193974437,-32.224918503225,-20.1848038826479));
#68476=CARTESIAN_POINT('Ctrl Pts',(34.1981589442514,-33.1736836666648,-20.1273183989614));
#68477=CARTESIAN_POINT('Ctrl Pts',(35.,-34.1448306280319,-20.0571817906459));
#68478=CARTESIAN_POINT('',(33.4246193974437,-33.5930121843923,-17.8151961173521));
#68479=CARTESIAN_POINT('Ctrl Pts',(33.4246193974437,-33.5930121843923,-17.8151961173521));
#68480=CARTESIAN_POINT('Ctrl Pts',(33.3753965426191,-32.9089653437931,-19.000000000027));
#68481=CARTESIAN_POINT('Ctrl Pts',(33.4246193974437,-32.224918503225,-20.1848038826479));
#68482=CARTESIAN_POINT('Ctrl Pts',(35.,-34.4424442730379,-19.5416998364696));
#68483=CARTESIAN_POINT('Ctrl Pts',(34.1981589442506,-34.0176108768905,-18.665593592959));
#68484=CARTESIAN_POINT('Ctrl Pts',(33.4246193974437,-33.5930121843923,-17.8151961173521));
#68485=CARTESIAN_POINT('Origin',(34.2,0.,0.));
#68486=CARTESIAN_POINT('',(35.,-37.1089869948545,-13.8232805156996));
#68487=CARTESIAN_POINT('',(35.,-37.3125667178958,-13.2639498235848));
#68488=CARTESIAN_POINT('Origin',(35.,0.,0.));
#68489=CARTESIAN_POINT('',(33.4246193974437,-35.2404039929487,-14.2823529831122));
#68490=CARTESIAN_POINT('Ctrl Pts',(33.4246193974437,-35.2404039929487,-14.2823529831122));
#68491=CARTESIAN_POINT('Ctrl Pts',(34.1981589442501,-36.1647730322061,-14.0609894914273));
#68492=CARTESIAN_POINT('Ctrl Pts',(35.,-37.1089869948545,-13.8232805156996));
#68493=CARTESIAN_POINT('',(33.4246193974437,-36.1762351867803,-11.7111779096386));
#68494=CARTESIAN_POINT('Ctrl Pts',(33.4246193974437,-36.1762351867803,-11.7111779096386));
#68495=CARTESIAN_POINT('Ctrl Pts',(33.3753965426192,-35.7083195898539,-12.9967654464047));
#68496=CARTESIAN_POINT('Ctrl Pts',(33.4246193974437,-35.2404039929487,-14.2823529831122));
#68497=CARTESIAN_POINT('Ctrl Pts',(35.,-37.3125667178958,-13.2639498235848));
#68498=CARTESIAN_POINT('Ctrl Pts',(34.1981589442499,-36.7420532430025,-12.4749251475656));
#68499=CARTESIAN_POINT('Ctrl Pts',(33.4246193974437,-36.1762351867803,-11.7111779096386));
#68500=CARTESIAN_POINT('Origin',(34.2,0.,0.));
#68501=CARTESIAN_POINT('',(35.,-38.9456055698919,-7.16936585720128));
#68502=CARTESIAN_POINT('',(35.,-39.0489657041002,-6.58318140719289));
#68503=CARTESIAN_POINT('Origin',(35.,0.,0.));
#68504=CARTESIAN_POINT('',(33.4246193974437,-37.1851276398516,-7.94594001540395));
#68505=CARTESIAN_POINT('Ctrl Pts',(33.4246193974437,-37.1851276398516,-7.94594001540395));
#68506=CARTESIAN_POINT('Ctrl Pts',(34.1981589442497,-38.0570140694232,-7.5674245334002));
#68507=CARTESIAN_POINT('Ctrl Pts',(35.,-38.9456055698919,-7.16936585720128));
#68508=CARTESIAN_POINT('',(33.4246193974437,-37.6602615890763,-5.25132148728274));
#68509=CARTESIAN_POINT('Ctrl Pts',(33.4246193974437,-37.6602615890763,-5.25132148728274));
#68510=CARTESIAN_POINT('Ctrl Pts',(33.3753965426191,-37.4226946144585,-6.59863075137405));
#68511=CARTESIAN_POINT('Ctrl Pts',(33.4246193974437,-37.1851276398516,-7.94594001540395));
#68512=CARTESIAN_POINT('Ctrl Pts',(35.,-39.0489657041002,-6.58318140719289));
#68513=CARTESIAN_POINT('Ctrl Pts',(34.1981589442488,-38.3501069137014,-5.90521241417989));
#68514=CARTESIAN_POINT('Ctrl Pts',(33.4246193974437,-37.6602615890763,-5.25132148728274));
#68515=CARTESIAN_POINT('Origin',(34.2,0.,0.));
#68516=CARTESIAN_POINT('',(35.,-39.5988816271155,-0.29761364500606));
#68517=CARTESIAN_POINT('',(35.,-39.5988816271155,0.297613645006073));
#68518=CARTESIAN_POINT('Origin',(35.,0.,0.));
#68519=CARTESIAN_POINT('',(33.4246193974437,-38.,-1.36809368116733));
#68520=CARTESIAN_POINT('Ctrl Pts',(33.4246193974437,-38.,-1.36809368116733));
#68521=CARTESIAN_POINT('Ctrl Pts',(34.1981589442507,-38.7929119919205,-0.843927210226627));
#68522=CARTESIAN_POINT('Ctrl Pts',(35.,-39.5988816271155,-0.297613645006064));
#68523=CARTESIAN_POINT('',(33.4246193974437,-38.,1.36809368116734));
#68524=CARTESIAN_POINT('Ctrl Pts',(33.4246193974437,-38.,1.36809368116734));
#68525=CARTESIAN_POINT('Ctrl Pts',(33.3753965426192,-38.,-3.11753400872306E-11));
#68526=CARTESIAN_POINT('Ctrl Pts',(33.4246193974437,-38.,-1.36809368116733));
#68527=CARTESIAN_POINT('Ctrl Pts',(35.,-39.5988816271155,0.297613645006073));
#68528=CARTESIAN_POINT('Ctrl Pts',(34.1981589442507,-38.7929119919206,0.843927210226618));
#68529=CARTESIAN_POINT('Ctrl Pts',(33.4246193974437,-38.,1.36809368116734));
#68530=CARTESIAN_POINT('Origin',(34.2,0.,0.));
#68531=CARTESIAN_POINT('',(35.,-39.0489657041001,6.58318140719291));
#68532=CARTESIAN_POINT('',(35.,-38.9456055698919,7.16936585720131));
#68533=CARTESIAN_POINT('Origin',(35.,0.,0.));
#68534=CARTESIAN_POINT('',(33.4246193974437,-37.6602615890763,5.25132148728276));
#68535=CARTESIAN_POINT('Ctrl Pts',(33.4246193974437,-37.6602615890763,5.25132148728276));
#68536=CARTESIAN_POINT('Ctrl Pts',(34.1981589442494,-38.3501069137019,5.90521241418043));
#68537=CARTESIAN_POINT('Ctrl Pts',(35.,-39.0489657041001,6.58318140719291));
#68538=CARTESIAN_POINT('',(33.4246193974437,-37.1851276398516,7.94594001540397));
#68539=CARTESIAN_POINT('Ctrl Pts',(33.4246193974437,-37.1851276398516,7.94594001540397));
#68540=CARTESIAN_POINT('Ctrl Pts',(33.3753965426191,-37.4226946144693,6.59863075131266));
#68541=CARTESIAN_POINT('Ctrl Pts',(33.4246193974437,-37.6602615890763,5.25132148728276));
#68542=CARTESIAN_POINT('Ctrl Pts',(35.,-38.9456055698919,7.16936585720131));
#68543=CARTESIAN_POINT('Ctrl Pts',(34.1981589442514,-38.057014069425,7.56742453339942));
#68544=CARTESIAN_POINT('Ctrl Pts',(33.4246193974437,-37.1851276398516,7.94594001540397));
#68545=CARTESIAN_POINT('Origin',(34.2,0.,0.));
#68546=CARTESIAN_POINT('',(35.,-37.3125667178958,13.2639498235848));
#68547=CARTESIAN_POINT('',(35.,-37.1089869948545,13.8232805156996));
#68548=CARTESIAN_POINT('Origin',(35.,0.,0.));
#68549=CARTESIAN_POINT('',(33.4246193974437,-36.1762351867803,11.7111779096386));
#68550=CARTESIAN_POINT('Ctrl Pts',(33.4246193974437,-36.1762351867803,11.7111779096386));
#68551=CARTESIAN_POINT('Ctrl Pts',(34.1981589442498,-36.7420532430025,12.4749251475655));
#68552=CARTESIAN_POINT('Ctrl Pts',(35.,-37.3125667178958,13.2639498235848));
#68553=CARTESIAN_POINT('',(33.4246193974437,-35.2404039929487,14.2823529831122));
#68554=CARTESIAN_POINT('Ctrl Pts',(33.4246193974437,-35.2404039929487,14.2823529831122));
#68555=CARTESIAN_POINT('Ctrl Pts',(33.3753965426191,-35.7083195898752,12.9967654463461));
#68556=CARTESIAN_POINT('Ctrl Pts',(33.4246193974437,-36.1762351867803,11.7111779096386));
#68557=CARTESIAN_POINT('Ctrl Pts',(35.,-37.1089869948545,13.8232805156996));
#68558=CARTESIAN_POINT('Ctrl Pts',(34.1981589442512,-36.1647730322074,14.060989491427));
#68559=CARTESIAN_POINT('Ctrl Pts',(33.4246193974437,-35.2404039929487,14.2823529831122));
#68560=CARTESIAN_POINT('Origin',(34.2,0.,0.));
#68561=CARTESIAN_POINT('',(35.,-34.4424442730379,19.5416998364696));
#68562=CARTESIAN_POINT('',(35.,-34.1448306280319,20.0571817906459));
#68563=CARTESIAN_POINT('Origin',(35.,0.,0.));
#68564=CARTESIAN_POINT('',(33.4246193974437,-33.5930121843923,17.8151961173521));
#68565=CARTESIAN_POINT('Ctrl Pts',(33.4246193974437,-33.5930121843923,17.8151961173521));
#68566=CARTESIAN_POINT('Ctrl Pts',(34.1981589442509,-34.0176108768906,18.6655935929593));
#68567=CARTESIAN_POINT('Ctrl Pts',(35.,-34.4424442730379,19.5416998364696));
#68568=CARTESIAN_POINT('',(33.4246193974437,-32.224918503225,20.1848038826479));
#68569=CARTESIAN_POINT('Ctrl Pts',(33.4246193974437,-32.224918503225,20.1848038826479));
#68570=CARTESIAN_POINT('Ctrl Pts',(33.3753965426192,-32.9089653438243,18.999999999973));
#68571=CARTESIAN_POINT('Ctrl Pts',(33.4246193974437,-33.5930121843923,17.8151961173521));
#68572=CARTESIAN_POINT('Ctrl Pts',(35.,-34.1448306280319,20.0571817906459));
#68573=CARTESIAN_POINT('Ctrl Pts',(34.19815894425,-33.173683666663,20.1273183989615));
#68574=CARTESIAN_POINT('Ctrl Pts',(33.4246193974437,-32.224918503225,20.1848038826479));
#68575=CARTESIAN_POINT('Origin',(34.2,0.,0.));
#68576=CARTESIAN_POINT('',(35.,-30.5258055876616,25.2256851884005));
#68577=CARTESIAN_POINT('',(35.,-30.1432008606945,25.6816557463071));
#68578=CARTESIAN_POINT('Origin',(35.,0.,0.));
#68579=CARTESIAN_POINT('',(33.4246193974437,-29.989082505666,23.3779086059641));
#68580=CARTESIAN_POINT('Ctrl Pts',(33.4246193974437,-29.989082505666,23.3779086059641));
#68581=CARTESIAN_POINT('Ctrl Pts',(34.1981589442502,-30.2595606180251,24.2891174222754));
#68582=CARTESIAN_POINT('Ctrl Pts',(35.,-30.5258055876616,25.2256851884005));
#68583=CARTESIAN_POINT('',(33.4246193974437,-28.2302951713763,25.4739497302129));
#68584=CARTESIAN_POINT('Ctrl Pts',(33.4246193974437,-28.2302951713763,25.4739497302129));
#68585=CARTESIAN_POINT('Ctrl Pts',(33.3753965426192,-29.1096888385412,24.4259291680646));
#68586=CARTESIAN_POINT('Ctrl Pts',(33.4246193974437,-29.989082505666,23.3779086059641));
#68587=CARTESIAN_POINT('Ctrl Pts',(35.,-30.1432008606945,25.6816557463071));
#68588=CARTESIAN_POINT('Ctrl Pts',(34.1981589442515,-29.1746287096043,25.582088921858));
#68589=CARTESIAN_POINT('Ctrl Pts',(33.4246193974437,-28.2302951713763,25.4739497302129));
#68590=CARTESIAN_POINT('Origin',(34.2,0.,0.));
#68591=CARTESIAN_POINT('',(35.,-25.6816557463071,30.1432008606945));
#68592=CARTESIAN_POINT('',(35.,-25.2256851884005,30.5258055876616));
#68593=CARTESIAN_POINT('Origin',(35.,0.,0.));
#68594=CARTESIAN_POINT('',(33.4246193974437,-25.4739497302129,28.2302951713764));
#68595=CARTESIAN_POINT('Ctrl Pts',(33.4246193974437,-25.4739497302129,28.2302951713764));
#68596=CARTESIAN_POINT('Ctrl Pts',(34.1981589442499,-25.5820889218578,29.1746287096024));
#68597=CARTESIAN_POINT('Ctrl Pts',(35.,-25.6816557463071,30.1432008606945));
#68598=CARTESIAN_POINT('',(33.4246193974437,-23.3779086059641,29.989082505666));
#68599=CARTESIAN_POINT('Ctrl Pts',(33.4246193974437,-23.3779086059641,29.989082505666));
#68600=CARTESIAN_POINT('Ctrl Pts',(33.3753965426191,-24.4259291681124,29.1096888385011));
#68601=CARTESIAN_POINT('Ctrl Pts',(33.4246193974437,-25.4739497302129,28.2302951713764));
#68602=CARTESIAN_POINT('Ctrl Pts',(35.,-25.2256851884005,30.5258055876616));
#68603=CARTESIAN_POINT('Ctrl Pts',(34.1981589442511,-24.2891174222765,30.2595606180255));
#68604=CARTESIAN_POINT('Ctrl Pts',(33.4246193974437,-23.3779086059641,29.989082505666));
#68605=CARTESIAN_POINT('Origin',(34.2,0.,0.));
#68606=CARTESIAN_POINT('',(35.,-20.0571817906459,34.1448306280319));
#68607=CARTESIAN_POINT('',(35.,-19.5416998364696,34.4424442730379));
#68608=CARTESIAN_POINT('Origin',(35.,0.,0.));
#68609=CARTESIAN_POINT('',(33.4246193974437,-20.1848038826479,32.224918503225));
#68610=CARTESIAN_POINT('Ctrl Pts',(33.4246193974437,-20.1848038826479,32.224918503225));
#68611=CARTESIAN_POINT('Ctrl Pts',(34.1981589442516,-20.1273183989614,33.173683666665));
#68612=CARTESIAN_POINT('Ctrl Pts',(35.,-20.0571817906459,34.1448306280319));
#68613=CARTESIAN_POINT('',(33.4246193974437,-17.8151961173521,33.5930121843923));
#68614=CARTESIAN_POINT('Ctrl Pts',(33.4246193974437,-17.8151961173521,33.5930121843923));
#68615=CARTESIAN_POINT('Ctrl Pts',(33.3753965426191,-19.000000000027,32.9089653437931));
#68616=CARTESIAN_POINT('Ctrl Pts',(33.4246193974437,-20.1848038826479,32.224918503225));
#68617=CARTESIAN_POINT('Ctrl Pts',(35.,-19.5416998364696,34.4424442730379));
#68618=CARTESIAN_POINT('Ctrl Pts',(34.1981589442509,-18.6655935929593,34.0176108768906));
#68619=CARTESIAN_POINT('Ctrl Pts',(33.4246193974437,-17.8151961173521,33.5930121843923));
#68620=CARTESIAN_POINT('Origin',(34.2,0.,0.));
#68621=CARTESIAN_POINT('',(35.,-13.8232805156996,37.1089869948545));
#68622=CARTESIAN_POINT('',(35.,-13.2639498235848,37.3125667178958));
#68623=CARTESIAN_POINT('Origin',(35.,0.,0.));
#68624=CARTESIAN_POINT('',(33.4246193974437,-14.2823529831122,35.2404039929487));
#68625=CARTESIAN_POINT('Ctrl Pts',(33.4246193974437,-14.2823529831122,35.2404039929487));
#68626=CARTESIAN_POINT('Ctrl Pts',(34.1981589442515,-14.0609894914269,36.1647730322078));
#68627=CARTESIAN_POINT('Ctrl Pts',(35.,-13.8232805156996,37.1089869948545));
#68628=CARTESIAN_POINT('',(33.4246193974437,-11.7111779096386,36.1762351867803));
#68629=CARTESIAN_POINT('Ctrl Pts',(33.4246193974437,-11.7111779096386,36.1762351867803));
#68630=CARTESIAN_POINT('Ctrl Pts',(33.3753965426191,-12.9967654464047,35.7083195898539));
#68631=CARTESIAN_POINT('Ctrl Pts',(33.4246193974437,-14.2823529831122,35.2404039929487));
#68632=CARTESIAN_POINT('Ctrl Pts',(35.,-13.2639498235848,37.3125667178958));
#68633=CARTESIAN_POINT('Ctrl Pts',(34.1981589442494,-12.4749251475651,36.7420532430021));
#68634=CARTESIAN_POINT('Ctrl Pts',(33.4246193974437,-11.7111779096386,36.1762351867803));
#68635=CARTESIAN_POINT('Origin',(34.2,0.,0.));
#68636=CARTESIAN_POINT('',(35.,-7.16936585720129,38.9456055698919));
#68637=CARTESIAN_POINT('',(35.,-6.5831814071929,39.0489657041001));
#68638=CARTESIAN_POINT('Origin',(35.,0.,0.));
#68639=CARTESIAN_POINT('',(33.4246193974437,-7.94594001540395,37.1851276398516));
#68640=CARTESIAN_POINT('Ctrl Pts',(33.4246193974437,-7.94594001540395,37.1851276398516));
#68641=CARTESIAN_POINT('Ctrl Pts',(34.1981589442492,-7.56742453340049,38.0570140694225));
#68642=CARTESIAN_POINT('Ctrl Pts',(35.,-7.16936585720129,38.9456055698919));
#68643=CARTESIAN_POINT('',(33.4246193974437,-5.25132148728275,37.6602615890763));
#68644=CARTESIAN_POINT('Ctrl Pts',(33.4246193974437,-5.25132148728275,37.6602615890763));
#68645=CARTESIAN_POINT('Ctrl Pts',(33.3753965426191,-6.59863075137406,37.4226946144585));
#68646=CARTESIAN_POINT('Ctrl Pts',(33.4246193974437,-7.94594001540395,37.1851276398516));
#68647=CARTESIAN_POINT('Ctrl Pts',(35.,-6.5831814071929,39.0489657041001));
#68648=CARTESIAN_POINT('Ctrl Pts',(34.1981589442491,-5.90521241418012,38.3501069137016));
#68649=CARTESIAN_POINT('Ctrl Pts',(33.4246193974437,-5.25132148728275,37.6602615890762));
#68650=CARTESIAN_POINT('Origin',(34.2,0.,0.));
#68651=CARTESIAN_POINT('',(35.,-0.297613645006061,39.5988816271155));
#68652=CARTESIAN_POINT('',(35.,0.29761364500607,39.5988816271155));
#68653=CARTESIAN_POINT('Origin',(35.,0.,0.));
#68654=CARTESIAN_POINT('',(33.4246193974437,-1.36809368116733,38.));
#68655=CARTESIAN_POINT('Ctrl Pts',(33.4246193974437,-1.36809368116733,38.));
#68656=CARTESIAN_POINT('Ctrl Pts',(34.1981589442505,-0.843927210226743,
38.7929119919204));
#68657=CARTESIAN_POINT('Ctrl Pts',(35.,-0.297613645006066,39.5988816271155));
#68658=CARTESIAN_POINT('',(33.4246193974437,1.36809368116733,38.));
#68659=CARTESIAN_POINT('Ctrl Pts',(33.4246193974437,1.36809368116733,38.));
#68660=CARTESIAN_POINT('Ctrl Pts',(33.3753965426191,-3.11806136465975E-11,
38.));
#68661=CARTESIAN_POINT('Ctrl Pts',(33.4246193974437,-1.36809368116733,38.));
#68662=CARTESIAN_POINT('Ctrl Pts',(35.,0.297613645006069,39.5988816271155));
#68663=CARTESIAN_POINT('Ctrl Pts',(34.1981589442504,0.843927210226807,38.7929119919203));
#68664=CARTESIAN_POINT('Ctrl Pts',(33.4246193974437,1.36809368116733,38.));
#68665=CARTESIAN_POINT('Origin',(34.2,0.,0.));
#68666=CARTESIAN_POINT('',(35.,6.5831814071929,39.0489657041002));
#68667=CARTESIAN_POINT('',(35.,7.1693658572013,38.9456055698919));
#68668=CARTESIAN_POINT('Origin',(35.,0.,0.));
#68669=CARTESIAN_POINT('',(33.4246193974437,5.25132148728276,37.6602615890763));
#68670=CARTESIAN_POINT('Ctrl Pts',(33.4246193974437,5.25132148728276,37.6602615890763));
#68671=CARTESIAN_POINT('Ctrl Pts',(34.1981589442498,5.90521241418073,38.3501069137022));
#68672=CARTESIAN_POINT('Ctrl Pts',(35.,6.5831814071929,39.0489657041002));
#68673=CARTESIAN_POINT('',(33.4246193974437,7.94594001540395,37.1851276398516));
#68674=CARTESIAN_POINT('Ctrl Pts',(33.4246193974437,7.94594001540395,37.1851276398516));
#68675=CARTESIAN_POINT('Ctrl Pts',(33.3753965426192,6.59863075131265,37.4226946144693));
#68676=CARTESIAN_POINT('Ctrl Pts',(33.4246193974437,5.25132148728276,37.6602615890763));
#68677=CARTESIAN_POINT('Ctrl Pts',(35.,7.1693658572013,38.9456055698919));
#68678=CARTESIAN_POINT('Ctrl Pts',(34.1981589442516,7.56742453339927,38.0570140694253));
#68679=CARTESIAN_POINT('Ctrl Pts',(33.4246193974437,7.94594001540395,37.1851276398516));
#68680=CARTESIAN_POINT('Origin',(34.2,0.,0.));
#68681=CARTESIAN_POINT('',(35.,13.2639498235848,37.3125667178958));
#68682=CARTESIAN_POINT('',(35.,13.8232805156997,37.1089869948545));
#68683=CARTESIAN_POINT('Origin',(35.,0.,0.));
#68684=CARTESIAN_POINT('',(33.4246193974437,11.7111779096386,36.1762351867803));
#68685=CARTESIAN_POINT('Ctrl Pts',(33.4246193974437,11.7111779096386,36.1762351867803));
#68686=CARTESIAN_POINT('Ctrl Pts',(34.1981589442503,12.4749251475659,36.7420532430028));
#68687=CARTESIAN_POINT('Ctrl Pts',(35.,13.2639498235848,37.3125667178958));
#68688=CARTESIAN_POINT('',(33.4246193974437,14.2823529831122,35.2404039929487));
#68689=CARTESIAN_POINT('Ctrl Pts',(33.4246193974437,14.2823529831122,35.2404039929487));
#68690=CARTESIAN_POINT('Ctrl Pts',(33.3753965426192,12.9967654463461,35.7083195898752));
#68691=CARTESIAN_POINT('Ctrl Pts',(33.4246193974437,11.7111779096386,36.1762351867803));
#68692=CARTESIAN_POINT('Ctrl Pts',(35.,13.8232805156996,37.1089869948545));
#68693=CARTESIAN_POINT('Ctrl Pts',(34.1981589442506,14.0609894914271,36.1647730322067));
#68694=CARTESIAN_POINT('Ctrl Pts',(33.4246193974437,14.2823529831122,35.2404039929487));
#68695=CARTESIAN_POINT('Origin',(34.2,0.,0.));
#68696=CARTESIAN_POINT('',(35.,19.5416998364696,34.4424442730379));
#68697=CARTESIAN_POINT('',(35.,20.0571817906459,34.1448306280319));
#68698=CARTESIAN_POINT('Origin',(35.,0.,0.));
#68699=CARTESIAN_POINT('',(33.4246193974437,17.8151961173521,33.5930121843923));
#68700=CARTESIAN_POINT('Ctrl Pts',(33.4246193974437,17.8151961173521,33.5930121843923));
#68701=CARTESIAN_POINT('Ctrl Pts',(34.1981589442516,18.6655935929601,34.017610876891));
#68702=CARTESIAN_POINT('Ctrl Pts',(35.,19.5416998364696,34.4424442730379));
#68703=CARTESIAN_POINT('',(33.4246193974437,20.1848038826479,32.224918503225));
#68704=CARTESIAN_POINT('Ctrl Pts',(33.4246193974437,20.1848038826479,32.224918503225));
#68705=CARTESIAN_POINT('Ctrl Pts',(33.3753965426192,18.999999999973,32.9089653438243));
#68706=CARTESIAN_POINT('Ctrl Pts',(33.4246193974437,17.8151961173521,33.5930121843923));
#68707=CARTESIAN_POINT('Ctrl Pts',(35.,20.0571817906459,34.1448306280319));
#68708=CARTESIAN_POINT('Ctrl Pts',(34.1981589442511,20.1273183989614,33.1736836666644));
#68709=CARTESIAN_POINT('Ctrl Pts',(33.4246193974437,20.1848038826479,32.224918503225));
#68710=CARTESIAN_POINT('Origin',(34.2,0.,0.));
#68711=CARTESIAN_POINT('',(35.,25.2256851884005,30.5258055876616));
#68712=CARTESIAN_POINT('',(35.,25.6816557463071,30.1432008606945));
#68713=CARTESIAN_POINT('Origin',(35.,0.,0.));
#68714=CARTESIAN_POINT('',(33.4246193974437,23.3779086059641,29.989082505666));
#68715=CARTESIAN_POINT('Ctrl Pts',(33.4246193974437,23.3779086059641,29.989082505666));
#68716=CARTESIAN_POINT('Ctrl Pts',(34.1981589442514,24.2891174222768,30.2595606180256));
#68717=CARTESIAN_POINT('Ctrl Pts',(35.,25.2256851884005,30.5258055876616));
#68718=CARTESIAN_POINT('',(33.4246193974437,25.4739497302129,28.2302951713764));
#68719=CARTESIAN_POINT('Ctrl Pts',(33.4246193974437,25.4739497302129,28.2302951713764));
#68720=CARTESIAN_POINT('Ctrl Pts',(33.3753965426192,24.4259291680646,29.1096888385412));
#68721=CARTESIAN_POINT('Ctrl Pts',(33.4246193974437,23.3779086059641,29.989082505666));
#68722=CARTESIAN_POINT('Ctrl Pts',(35.,25.6816557463071,30.1432008606945));
#68723=CARTESIAN_POINT('Ctrl Pts',(34.1981589442496,25.5820889218578,29.174628709602));
#68724=CARTESIAN_POINT('Ctrl Pts',(33.4246193974437,25.4739497302129,28.2302951713764));
#68725=CARTESIAN_POINT('Origin',(34.2,0.,0.));
#68726=CARTESIAN_POINT('',(35.,30.1432008606945,25.6816557463071));
#68727=CARTESIAN_POINT('',(35.,30.5258055876616,25.2256851884005));
#68728=CARTESIAN_POINT('Origin',(35.,0.,0.));
#68729=CARTESIAN_POINT('',(33.4246193974437,28.2302951713764,25.4739497302129));
#68730=CARTESIAN_POINT('Ctrl Pts',(33.4246193974437,28.2302951713764,25.4739497302129));
#68731=CARTESIAN_POINT('Ctrl Pts',(34.1981589442485,29.1746287096007,25.5820889218576));
#68732=CARTESIAN_POINT('Ctrl Pts',(35.,30.1432008606945,25.6816557463071));
#68733=CARTESIAN_POINT('',(33.4246193974437,29.989082505666,23.3779086059641));
#68734=CARTESIAN_POINT('Ctrl Pts',(33.4246193974437,29.989082505666,23.3779086059641));
#68735=CARTESIAN_POINT('Ctrl Pts',(33.3753965426192,29.1096888385011,24.4259291681124));
#68736=CARTESIAN_POINT('Ctrl Pts',(33.4246193974437,28.2302951713764,25.4739497302129));
#68737=CARTESIAN_POINT('Ctrl Pts',(35.,30.5258055876616,25.2256851884005));
#68738=CARTESIAN_POINT('Ctrl Pts',(34.1981589442495,30.2595606180249,24.2891174222746));
#68739=CARTESIAN_POINT('Ctrl Pts',(33.4246193974437,29.989082505666,23.3779086059641));
#68740=CARTESIAN_POINT('Origin',(34.2,0.,0.));
#68741=CARTESIAN_POINT('',(35.,34.1448306280319,20.0571817906459));
#68742=CARTESIAN_POINT('',(35.,34.4424442730379,19.5416998364696));
#68743=CARTESIAN_POINT('Origin',(35.,0.,0.));
#68744=CARTESIAN_POINT('',(33.4246193974437,32.224918503225,20.1848038826479));
#68745=CARTESIAN_POINT('Ctrl Pts',(33.4246193974437,32.224918503225,20.1848038826479));
#68746=CARTESIAN_POINT('Ctrl Pts',(34.1981589442511,33.1736836666644,20.1273183989614));
#68747=CARTESIAN_POINT('Ctrl Pts',(35.,34.1448306280319,20.0571817906459));
#68748=CARTESIAN_POINT('',(33.4246193974437,33.5930121843923,17.8151961173521));
#68749=CARTESIAN_POINT('Ctrl Pts',(33.4246193974437,33.5930121843923,17.8151961173521));
#68750=CARTESIAN_POINT('Ctrl Pts',(33.3753965426192,32.9089653437931,19.000000000027));
#68751=CARTESIAN_POINT('Ctrl Pts',(33.4246193974437,32.224918503225,20.1848038826479));
#68752=CARTESIAN_POINT('Ctrl Pts',(35.,34.4424442730379,19.5416998364696));
#68753=CARTESIAN_POINT('Ctrl Pts',(34.1981589442499,34.0176108768901,18.6655935929583));
#68754=CARTESIAN_POINT('Ctrl Pts',(33.4246193974437,33.5930121843923,17.8151961173521));
#68755=CARTESIAN_POINT('Origin',(34.2,0.,0.));
#68756=CARTESIAN_POINT('',(35.,37.1089869948545,13.8232805156996));
#68757=CARTESIAN_POINT('',(35.,37.3125667178958,13.2639498235848));
#68758=CARTESIAN_POINT('Origin',(35.,0.,0.));
#68759=CARTESIAN_POINT('',(33.4246193974437,35.2404039929487,14.2823529831122));
#68760=CARTESIAN_POINT('Ctrl Pts',(33.4246193974437,35.2404039929487,14.2823529831122));
#68761=CARTESIAN_POINT('Ctrl Pts',(34.1981589442501,36.1647730322061,14.0609894914273));
#68762=CARTESIAN_POINT('Ctrl Pts',(35.,37.1089869948545,13.8232805156996));
#68763=CARTESIAN_POINT('',(33.4246193974437,36.1762351867803,11.7111779096386));
#68764=CARTESIAN_POINT('Ctrl Pts',(33.4246193974437,36.1762351867803,11.7111779096386));
#68765=CARTESIAN_POINT('Ctrl Pts',(33.3753965426191,35.7083195898539,12.9967654464047));
#68766=CARTESIAN_POINT('Ctrl Pts',(33.4246193974437,35.2404039929487,14.2823529831122));
#68767=CARTESIAN_POINT('Ctrl Pts',(35.,37.3125667178958,13.2639498235848));
#68768=CARTESIAN_POINT('Ctrl Pts',(34.1981589442503,36.7420532430028,12.474925147566));
#68769=CARTESIAN_POINT('Ctrl Pts',(33.4246193974437,36.1762351867803,11.7111779096386));
#68770=CARTESIAN_POINT('Origin',(34.2,0.,0.));
#68771=CARTESIAN_POINT('',(35.,38.9456055698919,7.16936585720129));
#68772=CARTESIAN_POINT('',(35.,39.0489657041002,6.5831814071929));
#68773=CARTESIAN_POINT('Origin',(35.,0.,0.));
#68774=CARTESIAN_POINT('',(33.4246193974437,37.1851276398516,7.94594001540395));
#68775=CARTESIAN_POINT('Ctrl Pts',(33.4246193974437,37.1851276398516,7.94594001540395));
#68776=CARTESIAN_POINT('Ctrl Pts',(34.1981589442508,38.0570140694243,7.56742453339971));
#68777=CARTESIAN_POINT('Ctrl Pts',(35.,38.9456055698919,7.16936585720129));
#68778=CARTESIAN_POINT('',(33.4246193974437,37.6602615890763,5.25132148728275));
#68779=CARTESIAN_POINT('Ctrl Pts',(33.4246193974437,37.6602615890763,5.25132148728275));
#68780=CARTESIAN_POINT('Ctrl Pts',(33.3753965426192,37.4226946144585,6.59863075137406));
#68781=CARTESIAN_POINT('Ctrl Pts',(33.4246193974437,37.1851276398516,7.94594001540395));
#68782=CARTESIAN_POINT('Ctrl Pts',(35.,39.0489657041001,6.5831814071929));
#68783=CARTESIAN_POINT('Ctrl Pts',(34.1981589442489,38.3501069137015,5.90521241418));
#68784=CARTESIAN_POINT('Ctrl Pts',(33.4246193974437,37.6602615890763,5.25132148728275));
#68785=CARTESIAN_POINT('Origin',(34.2,0.,0.));
#68786=CARTESIAN_POINT('',(35.,39.5988816271155,0.297613645006066));
#68787=CARTESIAN_POINT('',(35.,39.5988816271155,-0.297613645006066));
#68788=CARTESIAN_POINT('Origin',(35.,0.,0.));
#68789=CARTESIAN_POINT('',(33.4246193974437,38.,1.36809368116734));
#68790=CARTESIAN_POINT('Ctrl Pts',(33.4246193974437,38.,1.36809368116734));
#68791=CARTESIAN_POINT('Ctrl Pts',(34.1981589442493,38.7929119919191,0.84392721022757));
#68792=CARTESIAN_POINT('Ctrl Pts',(35.,39.5988816271155,0.297613645006068));
#68793=CARTESIAN_POINT('',(33.4246193974437,38.,-1.36809368116733));
#68794=CARTESIAN_POINT('Ctrl Pts',(33.4246193974437,38.,-1.36809368116733));
#68795=CARTESIAN_POINT('Ctrl Pts',(33.3753965426191,38.,3.11825565368906E-11));
#68796=CARTESIAN_POINT('Ctrl Pts',(33.4246193974437,38.,1.36809368116734));
#68797=CARTESIAN_POINT('Ctrl Pts',(35.,39.5988816271155,-0.297613645006068));
#68798=CARTESIAN_POINT('Ctrl Pts',(34.1981589442501,38.7929119919199,-0.84392721022704));
#68799=CARTESIAN_POINT('Ctrl Pts',(33.4246193974437,38.,-1.36809368116733));
#68800=CARTESIAN_POINT('Origin',(17.5,38.,0.));
#68801=CARTESIAN_POINT('',(33.1,38.,1.65));
#68802=CARTESIAN_POINT('',(33.1,38.,1.65));
#68803=CARTESIAN_POINT('',(30.5,38.,1.65));
#68804=CARTESIAN_POINT('',(30.5,38.,1.65));
#68805=CARTESIAN_POINT('',(30.5,38.,1.15));
#68806=CARTESIAN_POINT('',(30.5,38.,1.15));
#68807=CARTESIAN_POINT('',(24.1,38.,0.75));
#68808=CARTESIAN_POINT('',(24.1,38.,0.75));
#68809=CARTESIAN_POINT('',(23.1,38.,1.05));
#68810=CARTESIAN_POINT('',(23.1,38.,1.05));
#68811=CARTESIAN_POINT('',(22.4,38.,1.45));
#68812=CARTESIAN_POINT('',(22.4,38.,1.45));
#68813=CARTESIAN_POINT('',(21.8,38.,1.65));
#68814=CARTESIAN_POINT('',(21.8,38.,1.65));
#68815=CARTESIAN_POINT('',(13.2,38.,1.65));
#68816=CARTESIAN_POINT('',(13.2,38.,1.65));
#68817=CARTESIAN_POINT('',(12.6,38.,1.45));
#68818=CARTESIAN_POINT('',(12.6,38.,1.45));
#68819=CARTESIAN_POINT('',(11.9,38.,1.05));
#68820=CARTESIAN_POINT('',(11.9,38.,1.05));
#68821=CARTESIAN_POINT('',(10.9,38.,0.75));
#68822=CARTESIAN_POINT('',(10.9,38.,0.75));
#68823=CARTESIAN_POINT('',(4.5,38.,1.15));
#68824=CARTESIAN_POINT('',(4.5,38.,1.15));
#68825=CARTESIAN_POINT('',(4.5,38.,1.65));
#68826=CARTESIAN_POINT('',(4.5,38.,1.65));
#68827=CARTESIAN_POINT('',(1.9,38.,1.65));
#68828=CARTESIAN_POINT('',(1.9,38.,1.65));
#68829=CARTESIAN_POINT('',(1.57538060255633,38.,1.36809368116734));
#68830=CARTESIAN_POINT('',(0.,38.,0.));
#68831=CARTESIAN_POINT('',(1.57538060255632,38.,-1.36809368116733));
#68832=CARTESIAN_POINT('Ctrl Pts',(1.57538060255633,38.,1.36809368116734));
#68833=CARTESIAN_POINT('Ctrl Pts',(1.62460345738085,38.,-3.1172564529669E-11));
#68834=CARTESIAN_POINT('Ctrl Pts',(1.57538060255632,38.,-1.36809368116733));
#68835=CARTESIAN_POINT('',(1.9,38.,-1.65));
#68836=CARTESIAN_POINT('',(1.9,38.,-1.65));
#68837=CARTESIAN_POINT('',(4.5,38.,-1.65));
#68838=CARTESIAN_POINT('',(4.5,38.,-1.65));
#68839=CARTESIAN_POINT('',(4.5,38.,-1.15));
#68840=CARTESIAN_POINT('',(4.5,38.,-1.15));
#68841=CARTESIAN_POINT('',(10.9,38.,-0.75));
#68842=CARTESIAN_POINT('',(10.9,38.,-0.75));
#68843=CARTESIAN_POINT('',(11.9,38.,-1.05));
#68844=CARTESIAN_POINT('',(11.9,38.,-1.05));
#68845=CARTESIAN_POINT('',(12.6,38.,-1.45));
#68846=CARTESIAN_POINT('',(12.6,38.,-1.45));
#68847=CARTESIAN_POINT('',(13.2,38.,-1.65));
#68848=CARTESIAN_POINT('',(13.2,38.,-1.65));
#68849=CARTESIAN_POINT('',(21.8,38.,-1.65));
#68850=CARTESIAN_POINT('',(21.8,38.,-1.65));
#68851=CARTESIAN_POINT('',(22.4,38.,-1.45));
#68852=CARTESIAN_POINT('',(22.4,38.,-1.45));
#68853=CARTESIAN_POINT('',(23.1,38.,-1.05));
#68854=CARTESIAN_POINT('',(23.1,38.,-1.05));
#68855=CARTESIAN_POINT('',(24.1,38.,-0.75));
#68856=CARTESIAN_POINT('',(24.1,38.,-0.75));
#68857=CARTESIAN_POINT('',(30.5,38.,-1.15));
#68858=CARTESIAN_POINT('',(30.5,38.,-1.15));
#68859=CARTESIAN_POINT('',(30.5,38.,-1.65));
#68860=CARTESIAN_POINT('',(30.5,38.,-1.65));
#68861=CARTESIAN_POINT('',(33.1,38.,-1.65));
#68862=CARTESIAN_POINT('',(33.1,38.,-1.65));
#68863=CARTESIAN_POINT('',(35.,38.,0.));
#68864=CARTESIAN_POINT('Origin',(35.,38.,0.));
#68865=CARTESIAN_POINT('',(35.,42.75,0.884158520433536));
#68866=CARTESIAN_POINT('',(35.,44.7655886465086,1.25933744159137));
#68867=CARTESIAN_POINT('',(34.8617922858584,42.75,1.00418100903022));
#68868=CARTESIAN_POINT('',(33.5377160618333,42.75,2.15403667726254));
#68869=CARTESIAN_POINT('',(34.4,42.2794732300362,1.31762794090604));
#68870=CARTESIAN_POINT('Ctrl Pts',(34.4,42.2794732300361,1.31762794090604));
#68871=CARTESIAN_POINT('Ctrl Pts',(34.6297825291038,42.5142243943581,1.16177621660371));
#68872=CARTESIAN_POINT('Ctrl Pts',(34.8617922858584,42.75,1.00418100903022));
#68873=CARTESIAN_POINT('',(33.322645308031,42.240333256585,2.24593997529677));
#68874=CARTESIAN_POINT('Origin',(26.8550245390365,0.,0.));
#68875=CARTESIAN_POINT('',(33.0966075166785,37.9353893420094,1.64091956419534));
#68876=CARTESIAN_POINT('Origin',(17.5,37.4226946144639,6.59863075134335));
#68877=CARTESIAN_POINT('',(33.1,37.1361751213135,8.2235635438135));
#68878=CARTESIAN_POINT('',(33.1,37.1361751213135,8.2235635438135));
#68879=CARTESIAN_POINT('',(30.5,37.1361751213135,8.2235635438135));
#68880=CARTESIAN_POINT('',(30.5,37.1361751213135,8.2235635438135));
#68881=CARTESIAN_POINT('',(30.5,37.2229992101469,7.73115966730739));
#68882=CARTESIAN_POINT('',(30.5,37.2229992101469,7.73115966730739));
#68883=CARTESIAN_POINT('',(24.1,37.2924584812137,7.33723656610251));
#68884=CARTESIAN_POINT('',(24.1,37.2924584812137,7.33723656610251));
#68885=CARTESIAN_POINT('',(23.1,37.2403640279136,7.63267889200617));
#68886=CARTESIAN_POINT('',(23.1,37.2403640279136,7.63267889200617));
#68887=CARTESIAN_POINT('',(22.4,37.1709047568469,8.02660199321105));
#68888=CARTESIAN_POINT('',(22.4,37.1709047568469,8.02660199321105));
#68889=CARTESIAN_POINT('',(21.8,37.1361751213135,8.2235635438135));
#68890=CARTESIAN_POINT('',(21.8,37.1361751213135,8.2235635438135));
#68891=CARTESIAN_POINT('',(13.2,37.1361751213135,8.2235635438135));
#68892=CARTESIAN_POINT('',(13.2,37.1361751213135,8.2235635438135));
#68893=CARTESIAN_POINT('',(12.6,37.1709047568469,8.02660199321105));
#68894=CARTESIAN_POINT('',(12.6,37.1709047568469,8.02660199321105));
#68895=CARTESIAN_POINT('',(11.9,37.2403640279136,7.63267889200617));
#68896=CARTESIAN_POINT('',(11.9,37.2403640279136,7.63267889200617));
#68897=CARTESIAN_POINT('',(10.9,37.2924584812137,7.33723656610251));
#68898=CARTESIAN_POINT('',(10.9,37.2924584812137,7.33723656610251));
#68899=CARTESIAN_POINT('',(4.5,37.2229992101469,7.73115966730739));
#68900=CARTESIAN_POINT('',(4.5,37.2229992101469,7.73115966730739));
#68901=CARTESIAN_POINT('',(4.5,37.1361751213135,8.2235635438135));
#68902=CARTESIAN_POINT('',(4.5,37.1361751213135,8.2235635438135));
#68903=CARTESIAN_POINT('',(1.9,37.1361751213135,8.2235635438135));
#68904=CARTESIAN_POINT('',(1.9,37.1361751213135,8.2235635438135));
#68905=CARTESIAN_POINT('',(1.57538060255632,37.1851276398516,7.94594001540396));
#68906=CARTESIAN_POINT('',(0.,37.4226946144639,6.59863075134335));
#68907=CARTESIAN_POINT('',(1.57538060255632,37.6602615890763,5.25132148728275));
#68908=CARTESIAN_POINT('Ctrl Pts',(1.57538060255632,37.1851276398516,7.94594001540396));
#68909=CARTESIAN_POINT('Ctrl Pts',(1.62460345738085,37.4226946144693,6.59863075131265));
#68910=CARTESIAN_POINT('Ctrl Pts',(1.57538060255632,37.6602615890763,5.25132148728275));
#68911=CARTESIAN_POINT('',(1.9,37.7092141076143,4.97369795887321));
#68912=CARTESIAN_POINT('',(1.9,37.7092141076143,4.97369795887321));
#68913=CARTESIAN_POINT('',(4.5,37.7092141076143,4.97369795887321));
#68914=CARTESIAN_POINT('',(4.5,37.7092141076143,4.97369795887321));
#68915=CARTESIAN_POINT('',(4.5,37.6223900187809,5.46610183537931));
#68916=CARTESIAN_POINT('',(4.5,37.6223900187809,5.46610183537931));
#68917=CARTESIAN_POINT('',(10.9,37.5529307477141,5.8600249365842));
#68918=CARTESIAN_POINT('',(10.9,37.5529307477141,5.8600249365842));
#68919=CARTESIAN_POINT('',(11.9,37.6050252010142,5.56458261068053));
#68920=CARTESIAN_POINT('',(11.9,37.6050252010142,5.56458261068053));
#68921=CARTESIAN_POINT('',(12.6,37.674484472081,5.17065950947565));
#68922=CARTESIAN_POINT('',(12.6,37.674484472081,5.17065950947565));
#68923=CARTESIAN_POINT('',(13.2,37.7092141076143,4.97369795887321));
#68924=CARTESIAN_POINT('',(13.2,37.7092141076143,4.97369795887321));
#68925=CARTESIAN_POINT('',(21.8,37.7092141076143,4.97369795887321));
#68926=CARTESIAN_POINT('',(21.8,37.7092141076143,4.97369795887321));
#68927=CARTESIAN_POINT('',(22.4,37.674484472081,5.17065950947565));
#68928=CARTESIAN_POINT('',(22.4,37.674484472081,5.17065950947565));
#68929=CARTESIAN_POINT('',(23.1,37.6050252010142,5.56458261068053));
#68930=CARTESIAN_POINT('',(23.1,37.6050252010142,5.56458261068053));
#68931=CARTESIAN_POINT('',(24.1,37.5529307477141,5.8600249365842));
#68932=CARTESIAN_POINT('',(24.1,37.5529307477141,5.8600249365842));
#68933=CARTESIAN_POINT('',(30.5,37.6223900187809,5.46610183537931));
#68934=CARTESIAN_POINT('',(30.5,37.6223900187809,5.46610183537931));
#68935=CARTESIAN_POINT('',(30.5,37.7092141076143,4.97369795887321));
#68936=CARTESIAN_POINT('',(30.5,37.7092141076143,4.97369795887321));
#68937=CARTESIAN_POINT('',(33.1,37.7092141076143,4.97369795887321));
#68938=CARTESIAN_POINT('',(33.1,37.7092141076143,4.97369795887321));
#68939=CARTESIAN_POINT('',(35.,37.4226946144639,6.59863075134335));
#68940=CARTESIAN_POINT('Origin',(35.,37.4226946144639,6.59863075134335));
#68941=CARTESIAN_POINT('',(35.,41.9469989254299,8.29418576107602));
#68942=CARTESIAN_POINT('',(35.,42.7295335855124,8.58745307290921));
#68943=CARTESIAN_POINT('',(34.8617922858584,41.9261572390061,8.41238483838185));
#68944=CARTESIAN_POINT('',(33.5377160618333,41.7264868976375,9.54477161530208));
#68945=CARTESIAN_POINT('',(34.4,41.4083493394303,8.63936369090333));
#68946=CARTESIAN_POINT('Ctrl Pts',(34.4,41.4083493394303,8.63936369090333));
#68947=CARTESIAN_POINT('Ctrl Pts',(34.6297825291033,41.6665974739941,8.52664381637996));
#68948=CARTESIAN_POINT('Ctrl Pts',(34.8617922858584,41.9261572390061,8.41238483838185));
#68949=CARTESIAN_POINT('',(33.3226453080309,41.2086042970448,9.54677599452213));
#68950=CARTESIAN_POINT('Origin',(26.8550245390365,0.,0.));
#68951=CARTESIAN_POINT('',(33.0966075166785,37.0741228455271,8.20340153721441));
#68952=CARTESIAN_POINT('Origin',(17.5,35.7083195898645,12.9967654463754));
#68953=CARTESIAN_POINT('',(33.1,35.1439863533772,14.5472582706722));
#68954=CARTESIAN_POINT('',(33.1,35.1439863533772,14.5472582706722));
#68955=CARTESIAN_POINT('',(30.5,35.1439863533772,14.5472582706722));
#68956=CARTESIAN_POINT('',(30.5,35.1439863533772,14.5472582706722));
#68957=CARTESIAN_POINT('',(30.5,35.31499642504,14.0774119602792));
#68958=CARTESIAN_POINT('',(30.5,35.31499642504,14.0774119602792));
#68959=CARTESIAN_POINT('',(24.1,35.4518044823703,13.7015349119648));
#68960=CARTESIAN_POINT('',(24.1,35.4518044823703,13.7015349119648));
#68961=CARTESIAN_POINT('',(23.1,35.3491984393726,13.9834426982006));
#68962=CARTESIAN_POINT('',(23.1,35.3491984393726,13.9834426982006));
#68963=CARTESIAN_POINT('',(22.4,35.2123903820423,14.359319746515));
#68964=CARTESIAN_POINT('',(22.4,35.2123903820423,14.359319746515));
#68965=CARTESIAN_POINT('',(21.8,35.1439863533772,14.5472582706722));
#68966=CARTESIAN_POINT('',(21.8,35.1439863533772,14.5472582706722));
#68967=CARTESIAN_POINT('',(13.2,35.1439863533772,14.5472582706722));
#68968=CARTESIAN_POINT('',(13.2,35.1439863533772,14.5472582706722));
#68969=CARTESIAN_POINT('',(12.6,35.2123903820423,14.359319746515));
#68970=CARTESIAN_POINT('',(12.6,35.2123903820423,14.359319746515));
#68971=CARTESIAN_POINT('',(11.9,35.3491984393726,13.9834426982006));
#68972=CARTESIAN_POINT('',(11.9,35.3491984393726,13.9834426982006));
#68973=CARTESIAN_POINT('',(10.9,35.4518044823703,13.7015349119648));
#68974=CARTESIAN_POINT('',(10.9,35.4518044823703,13.7015349119648));
#68975=CARTESIAN_POINT('',(4.5,35.31499642504,14.0774119602792));
#68976=CARTESIAN_POINT('',(4.5,35.31499642504,14.0774119602792));
#68977=CARTESIAN_POINT('',(4.5,35.1439863533772,14.5472582706722));
#68978=CARTESIAN_POINT('',(4.5,35.1439863533772,14.5472582706722));
#68979=CARTESIAN_POINT('',(1.9,35.1439863533772,14.5472582706722));
#68980=CARTESIAN_POINT('',(1.9,35.1439863533772,14.5472582706722));
#68981=CARTESIAN_POINT('',(1.57538060255633,35.2404039929487,14.2823529831122));
#68982=CARTESIAN_POINT('',(0.,35.7083195898645,12.9967654463754));
#68983=CARTESIAN_POINT('',(1.57538060255632,36.1762351867803,11.7111779096386));
#68984=CARTESIAN_POINT('Ctrl Pts',(1.57538060255633,35.2404039929487,14.2823529831122));
#68985=CARTESIAN_POINT('Ctrl Pts',(1.62460345738085,35.7083195898752,12.9967654463461));
#68986=CARTESIAN_POINT('Ctrl Pts',(1.57538060255632,36.1762351867803,11.7111779096386));
#68987=CARTESIAN_POINT('',(1.9,36.2726528263519,11.4462726220787));
#68988=CARTESIAN_POINT('',(1.9,36.2726528263519,11.4462726220787));
#68989=CARTESIAN_POINT('',(4.5,36.2726528263519,11.4462726220787));
#68990=CARTESIAN_POINT('',(4.5,36.2726528263519,11.4462726220787));
#68991=CARTESIAN_POINT('',(4.5,36.101642754689,11.9161189324716));
#68992=CARTESIAN_POINT('',(4.5,36.101642754689,11.9161189324716));
#68993=CARTESIAN_POINT('',(10.9,35.9648346973588,12.291995980786));
#68994=CARTESIAN_POINT('',(10.9,35.9648346973588,12.291995980786));
#68995=CARTESIAN_POINT('',(11.9,36.0674407403565,12.0100881945502));
#68996=CARTESIAN_POINT('',(11.9,36.0674407403565,12.0100881945502));
#68997=CARTESIAN_POINT('',(12.6,36.2042487976867,11.6342111462358));
#68998=CARTESIAN_POINT('',(12.6,36.2042487976867,11.6342111462358));
#68999=CARTESIAN_POINT('',(13.2,36.2726528263519,11.4462726220787));
#69000=CARTESIAN_POINT('',(13.2,36.2726528263519,11.4462726220787));
#69001=CARTESIAN_POINT('',(21.8,36.2726528263519,11.4462726220787));
#69002=CARTESIAN_POINT('',(21.8,36.2726528263519,11.4462726220787));
#69003=CARTESIAN_POINT('',(22.4,36.2042487976867,11.6342111462358));
#69004=CARTESIAN_POINT('',(22.4,36.2042487976867,11.6342111462358));
#69005=CARTESIAN_POINT('',(23.1,36.0674407403565,12.0100881945502));
#69006=CARTESIAN_POINT('',(23.1,36.0674407403565,12.0100881945502));
#69007=CARTESIAN_POINT('',(24.1,35.9648346973588,12.291995980786));
#69008=CARTESIAN_POINT('',(24.1,35.9648346973588,12.291995980786));
#69009=CARTESIAN_POINT('',(30.5,36.101642754689,11.9161189324716));
#69010=CARTESIAN_POINT('',(30.5,36.101642754689,11.9161189324716));
#69011=CARTESIAN_POINT('',(30.5,36.2726528263519,11.4462726220787));
#69012=CARTESIAN_POINT('',(30.5,36.2726528263519,11.4462726220787));
#69013=CARTESIAN_POINT('',(33.1,36.2726528263519,11.4462726220787));
#69014=CARTESIAN_POINT('',(33.1,36.2726528263519,11.4462726220787));
#69015=CARTESIAN_POINT('',(35.,35.7083195898645,12.9967654463754));
#69016=CARTESIAN_POINT('Origin',(35.,35.7083195898645,12.9967654463754));
#69017=CARTESIAN_POINT('',(35.,39.8694595147163,15.4521983644287));
#69018=CARTESIAN_POINT('',(35.,38.9060829772051,14.8837227771125));
#69019=CARTESIAN_POINT('',(34.8617922858584,39.8284094059642,15.5649826112914));
#69020=CARTESIAN_POINT('',(33.5377160618333,39.4351356055115,16.6454934976981));
#69021=CARTESIAN_POINT('',(34.4,39.2790537077817,15.6985967468815));
#69022=CARTESIAN_POINT('Ctrl Pts',(34.4,39.2790537077817,15.6985967468815));
#69023=CARTESIAN_POINT('Ctrl Pts',(34.6297825290998,39.5529520736946,15.6324336584862));
#69024=CARTESIAN_POINT('Ctrl Pts',(34.8617922858584,39.8284094059642,15.5649826112914));
#69025=CARTESIAN_POINT('',(33.3226453080309,38.9247727484987,16.5575380560557));
#69026=CARTESIAN_POINT('Origin',(26.8550245390365,0.,0.));
#69027=CARTESIAN_POINT('',(33.0966075166785,35.0863778867947,14.5166273056467));
#69028=CARTESIAN_POINT('Origin',(17.5,32.9089653438087,19.));
#69029=CARTESIAN_POINT('',(33.1,32.0839653438087,20.4289419162443));
#69030=CARTESIAN_POINT('',(33.1,32.0839653438087,20.4289419162443));
#69031=CARTESIAN_POINT('',(30.5,32.0839653438087,20.4289419162443));
#69032=CARTESIAN_POINT('',(30.5,32.0839653438087,20.4289419162443));
#69033=CARTESIAN_POINT('',(30.5,32.3339653438087,19.9959292143521));
#69034=CARTESIAN_POINT('',(30.5,32.3339653438087,19.9959292143521));
#69035=CARTESIAN_POINT('',(24.1,32.5339653438087,19.6495190528383));
#69036=CARTESIAN_POINT('',(24.1,32.5339653438087,19.6495190528383));
#69037=CARTESIAN_POINT('',(23.1,32.3839653438087,19.9093266739737));
#69038=CARTESIAN_POINT('',(23.1,32.3839653438087,19.9093266739737));
#69039=CARTESIAN_POINT('',(22.4,32.1839653438087,20.2557368354874));
#69040=CARTESIAN_POINT('',(22.4,32.1839653438087,20.2557368354874));
#69041=CARTESIAN_POINT('',(21.8,32.0839653438087,20.4289419162443));
#69042=CARTESIAN_POINT('',(21.8,32.0839653438087,20.4289419162443));
#69043=CARTESIAN_POINT('',(13.2,32.0839653438087,20.4289419162443));
#69044=CARTESIAN_POINT('',(13.2,32.0839653438087,20.4289419162443));
#69045=CARTESIAN_POINT('',(12.6,32.1839653438087,20.2557368354874));
#69046=CARTESIAN_POINT('',(12.6,32.1839653438087,20.2557368354874));
#69047=CARTESIAN_POINT('',(11.9,32.3839653438087,19.9093266739737));
#69048=CARTESIAN_POINT('',(11.9,32.3839653438087,19.9093266739737));
#69049=CARTESIAN_POINT('',(10.9,32.5339653438087,19.6495190528383));
#69050=CARTESIAN_POINT('',(10.9,32.5339653438087,19.6495190528383));
#69051=CARTESIAN_POINT('',(4.5,32.3339653438087,19.9959292143521));
#69052=CARTESIAN_POINT('',(4.5,32.3339653438087,19.9959292143521));
#69053=CARTESIAN_POINT('',(4.5,32.0839653438087,20.4289419162443));
#69054=CARTESIAN_POINT('',(4.5,32.0839653438087,20.4289419162443));
#69055=CARTESIAN_POINT('',(1.9,32.0839653438087,20.4289419162443));
#69056=CARTESIAN_POINT('',(1.9,32.0839653438087,20.4289419162443));
#69057=CARTESIAN_POINT('',(1.57538060255632,32.224918503225,20.1848038826479));
#69058=CARTESIAN_POINT('',(0.,32.9089653438087,19.));
#69059=CARTESIAN_POINT('',(1.57538060255632,33.5930121843923,17.8151961173521));
#69060=CARTESIAN_POINT('Ctrl Pts',(1.57538060255632,32.224918503225,20.1848038826479));
#69061=CARTESIAN_POINT('Ctrl Pts',(1.62460345738085,32.9089653438243,18.999999999973));
#69062=CARTESIAN_POINT('Ctrl Pts',(1.57538060255632,33.5930121843923,17.8151961173521));
#69063=CARTESIAN_POINT('',(1.9,33.7339653438087,17.5710580837557));
#69064=CARTESIAN_POINT('',(1.9,33.7339653438087,17.5710580837557));
#69065=CARTESIAN_POINT('',(4.5,33.7339653438087,17.5710580837557));
#69066=CARTESIAN_POINT('',(4.5,33.7339653438087,17.5710580837557));
#69067=CARTESIAN_POINT('',(4.5,33.4839653438087,18.0040707856479));
#69068=CARTESIAN_POINT('',(4.5,33.4839653438087,18.0040707856479));
#69069=CARTESIAN_POINT('',(10.9,33.2839653438087,18.3504809471617));
#69070=CARTESIAN_POINT('',(10.9,33.2839653438087,18.3504809471617));
#69071=CARTESIAN_POINT('',(11.9,33.4339653438087,18.0906733260263));
#69072=CARTESIAN_POINT('',(11.9,33.4339653438087,18.0906733260263));
#69073=CARTESIAN_POINT('',(12.6,33.6339653438087,17.7442631645126));
#69074=CARTESIAN_POINT('',(12.6,33.6339653438087,17.7442631645126));
#69075=CARTESIAN_POINT('',(13.2,33.7339653438087,17.5710580837557));
#69076=CARTESIAN_POINT('',(13.2,33.7339653438087,17.5710580837557));
#69077=CARTESIAN_POINT('',(21.8,33.7339653438087,17.5710580837557));
#69078=CARTESIAN_POINT('',(21.8,33.7339653438087,17.5710580837557));
#69079=CARTESIAN_POINT('',(22.4,33.6339653438087,17.7442631645126));
#69080=CARTESIAN_POINT('',(22.4,33.6339653438087,17.7442631645126));
#69081=CARTESIAN_POINT('',(23.1,33.4339653438087,18.0906733260263));
#69082=CARTESIAN_POINT('',(23.1,33.4339653438087,18.0906733260263));
#69083=CARTESIAN_POINT('',(24.1,33.2839653438087,18.3504809471617));
#69084=CARTESIAN_POINT('',(24.1,33.2839653438087,18.3504809471617));
#69085=CARTESIAN_POINT('',(30.5,33.4839653438087,18.0040707856479));
#69086=CARTESIAN_POINT('',(30.5,33.4839653438087,18.0040707856479));
#69087=CARTESIAN_POINT('',(30.5,33.7339653438087,17.5710580837557));
#69088=CARTESIAN_POINT('',(30.5,33.7339653438087,17.5710580837557));
#69089=CARTESIAN_POINT('',(33.1,33.7339653438087,17.5710580837557));
#69090=CARTESIAN_POINT('',(33.1,33.7339653438087,17.5710580837557));
#69091=CARTESIAN_POINT('',(35.,32.9089653438087,19.));
#69092=CARTESIAN_POINT('Origin',(35.,32.9089653438087,19.));
#69093=CARTESIAN_POINT('',(35.,36.580506751568,22.1407037396679));
#69094=CARTESIAN_POINT('',(35.,33.7283972474216,19.7009570527085));
#69095=CARTESIAN_POINT('',(34.8617922858584,36.5204955072696,22.244646263818));
#69096=CARTESIAN_POINT('',(33.5377160618333,35.9455676731535,23.2404504831928));
#69097=CARTESIAN_POINT('',(34.4,35.9562839053824,22.2808358845789));
#69098=CARTESIAN_POINT('Ctrl Pts',(34.4,35.9562839053824,22.2808358845789));
#69099=CARTESIAN_POINT('Ctrl Pts',(34.6297825291007,36.2375102394006,22.2632399142707));
#69100=CARTESIAN_POINT('Ctrl Pts',(34.8617922858584,36.5204955072696,22.244646263818));
#69101=CARTESIAN_POINT('',(33.322645308031,35.4582316768749,23.0652077022745));
#69102=CARTESIAN_POINT('Origin',(26.8550245390365,0.,0.));
#69103=CARTESIAN_POINT('',(33.0966075166785,32.0325510905359,20.3887726991648));
#69104=CARTESIAN_POINT('Origin',(17.5,29.1096888385212,24.4259291680885));
#69105=CARTESIAN_POINT('',(33.1,28.0490892825384,25.6899024992348));
#69106=CARTESIAN_POINT('',(33.1,28.0490892825384,25.6899024992348));
#69107=CARTESIAN_POINT('',(30.5,28.0490892825384,25.6899024992348));
#69108=CARTESIAN_POINT('',(30.5,28.0490892825384,25.6899024992348));
#69109=CARTESIAN_POINT('',(30.5,28.3704830873816,25.3068802776753));
#69110=CARTESIAN_POINT('',(30.5,28.3704830873816,25.3068802776753));
#69111=CARTESIAN_POINT('',(24.1,28.6275981312563,25.0004625004277));
#69112=CARTESIAN_POINT('',(24.1,28.6275981312563,25.0004625004277));
#69113=CARTESIAN_POINT('',(23.1,28.4347618483503,25.2302758333634));
#69114=CARTESIAN_POINT('',(23.1,28.4347618483503,25.2302758333634));
#69115=CARTESIAN_POINT('',(22.4,28.1776468044757,25.536693610611));
#69116=CARTESIAN_POINT('',(22.4,28.1776468044757,25.536693610611));
#69117=CARTESIAN_POINT('',(21.8,28.0490892825384,25.6899024992348));
#69118=CARTESIAN_POINT('',(21.8,28.0490892825384,25.6899024992348));
#69119=CARTESIAN_POINT('',(13.2,28.0490892825384,25.6899024992348));
#69120=CARTESIAN_POINT('',(13.2,28.0490892825384,25.6899024992348));
#69121=CARTESIAN_POINT('',(12.6,28.1776468044757,25.536693610611));
#69122=CARTESIAN_POINT('',(12.6,28.1776468044757,25.536693610611));
#69123=CARTESIAN_POINT('',(11.9,28.4347618483503,25.2302758333634));
#69124=CARTESIAN_POINT('',(11.9,28.4347618483503,25.2302758333634));
#69125=CARTESIAN_POINT('',(10.9,28.6275981312563,25.0004625004277));
#69126=CARTESIAN_POINT('',(10.9,28.6275981312563,25.0004625004277));
#69127=CARTESIAN_POINT('',(4.5,28.3704830873816,25.3068802776753));
#69128=CARTESIAN_POINT('',(4.5,28.3704830873816,25.3068802776753));
#69129=CARTESIAN_POINT('',(4.5,28.0490892825384,25.6899024992348));
#69130=CARTESIAN_POINT('',(4.5,28.0490892825384,25.6899024992348));
#69131=CARTESIAN_POINT('',(1.9,28.0490892825384,25.6899024992348));
#69132=CARTESIAN_POINT('',(1.9,28.0490892825384,25.6899024992348));
#69133=CARTESIAN_POINT('',(1.57538060255632,28.2302951713764,25.4739497302129));
#69134=CARTESIAN_POINT('',(0.,29.1096888385212,24.4259291680885));
#69135=CARTESIAN_POINT('',(1.57538060255632,29.989082505666,23.3779086059641));
#69136=CARTESIAN_POINT('Ctrl Pts',(1.57538060255632,28.2302951713764,25.4739497302129));
#69137=CARTESIAN_POINT('Ctrl Pts',(1.62460345738085,29.1096888385412,24.4259291680646));
#69138=CARTESIAN_POINT('Ctrl Pts',(1.57538060255632,29.989082505666,23.3779086059641));
#69139=CARTESIAN_POINT('',(1.9,30.170288394504,23.1619558369422));
#69140=CARTESIAN_POINT('',(1.9,30.170288394504,23.1619558369422));
#69141=CARTESIAN_POINT('',(4.5,30.170288394504,23.1619558369422));
#69142=CARTESIAN_POINT('',(4.5,30.170288394504,23.1619558369422));
#69143=CARTESIAN_POINT('',(4.5,29.8488945896607,23.5449780585017));
#69144=CARTESIAN_POINT('',(4.5,29.8488945896607,23.5449780585017));
#69145=CARTESIAN_POINT('',(10.9,29.5917795457861,23.8513958357493));
#69146=CARTESIAN_POINT('',(10.9,29.5917795457861,23.8513958357493));
#69147=CARTESIAN_POINT('',(11.9,29.784615828692,23.6215825028136));
#69148=CARTESIAN_POINT('',(11.9,29.784615828692,23.6215825028136));
#69149=CARTESIAN_POINT('',(12.6,30.0417308725667,23.315164725566));
#69150=CARTESIAN_POINT('',(12.6,30.0417308725667,23.315164725566));
#69151=CARTESIAN_POINT('',(13.2,30.170288394504,23.1619558369422));
#69152=CARTESIAN_POINT('',(13.2,30.170288394504,23.1619558369422));
#69153=CARTESIAN_POINT('',(21.8,30.170288394504,23.1619558369422));
#69154=CARTESIAN_POINT('',(21.8,30.170288394504,23.1619558369422));
#69155=CARTESIAN_POINT('',(22.4,30.0417308725667,23.315164725566));
#69156=CARTESIAN_POINT('',(22.4,30.0417308725667,23.315164725566));
#69157=CARTESIAN_POINT('',(23.1,29.784615828692,23.6215825028136));
#69158=CARTESIAN_POINT('',(23.1,29.784615828692,23.6215825028136));
#69159=CARTESIAN_POINT('',(24.1,29.5917795457861,23.8513958357493));
#69160=CARTESIAN_POINT('',(24.1,29.5917795457861,23.8513958357493));
#69161=CARTESIAN_POINT('',(30.5,29.8488945896607,23.5449780585017));
#69162=CARTESIAN_POINT('',(30.5,29.8488945896607,23.5449780585017));
#69163=CARTESIAN_POINT('',(30.5,30.170288394504,23.1619558369422));
#69164=CARTESIAN_POINT('',(30.5,30.170288394504,23.1619558369422));
#69165=CARTESIAN_POINT('',(33.1,30.170288394504,23.1619558369422));
#69166=CARTESIAN_POINT('',(33.1,30.170288394504,23.1619558369422));
#69167=CARTESIAN_POINT('',(35.,29.1096888385212,24.4259291680885));
#69168=CARTESIAN_POINT('Origin',(35.,29.1096888385212,24.4259291680885));
#69169=CARTESIAN_POINT('',(35.,32.1800738014028,28.156475035514));
#69170=CARTESIAN_POINT('',(35.,27.7391842233302,22.7607535010967));
#69171=CARTESIAN_POINT('',(34.8617922858584,32.1029248328492,28.2484175959528));
#69172=CARTESIAN_POINT('',(33.5377160618333,31.3638118563816,29.129258140991));
#69173=CARTESIAN_POINT('',(34.4,31.5410006112756,28.1860830985703));
#69174=CARTESIAN_POINT('Ctrl Pts',(34.4,31.5410006112756,28.1860830985703));
#69175=CARTESIAN_POINT('Ctrl Pts',(34.6297825290998,31.8210099935452,28.2175888910031));
#69176=CARTESIAN_POINT('Ctrl Pts',(34.8617922858584,32.1029248328492,28.2484175959527));
#69177=CARTESIAN_POINT('',(33.3226453080309,30.9143101784803,28.872052684018));
#69178=CARTESIAN_POINT('Origin',(26.8550245390365,0.,0.));
#69179=CARTESIAN_POINT('',(33.0966075166785,28.0054314386442,25.6414155514355));
#69180=CARTESIAN_POINT('Origin',(17.5,24.4259291680885,29.1096888385212));
#69181=CARTESIAN_POINT('',(33.1,23.1619558369422,30.170288394504));
#69182=CARTESIAN_POINT('',(33.1,23.1619558369422,30.170288394504));
#69183=CARTESIAN_POINT('',(30.5,23.1619558369422,30.170288394504));
#69184=CARTESIAN_POINT('',(30.5,23.1619558369422,30.170288394504));
#69185=CARTESIAN_POINT('',(30.5,23.5449780585017,29.8488945896607));
#69186=CARTESIAN_POINT('',(30.5,23.5449780585017,29.8488945896607));
#69187=CARTESIAN_POINT('',(24.1,23.8513958357493,29.5917795457861));
#69188=CARTESIAN_POINT('',(24.1,23.8513958357493,29.5917795457861));
#69189=CARTESIAN_POINT('',(23.1,23.6215825028136,29.784615828692));
#69190=CARTESIAN_POINT('',(23.1,23.6215825028136,29.784615828692));
#69191=CARTESIAN_POINT('',(22.4,23.315164725566,30.0417308725666));
#69192=CARTESIAN_POINT('',(22.4,23.315164725566,30.0417308725666));
#69193=CARTESIAN_POINT('',(21.8,23.1619558369422,30.170288394504));
#69194=CARTESIAN_POINT('',(21.8,23.1619558369422,30.170288394504));
#69195=CARTESIAN_POINT('',(13.2,23.1619558369422,30.170288394504));
#69196=CARTESIAN_POINT('',(13.2,23.1619558369422,30.170288394504));
#69197=CARTESIAN_POINT('',(12.6,23.315164725566,30.0417308725666));
#69198=CARTESIAN_POINT('',(12.6,23.315164725566,30.0417308725666));
#69199=CARTESIAN_POINT('',(11.9,23.6215825028136,29.784615828692));
#69200=CARTESIAN_POINT('',(11.9,23.6215825028136,29.784615828692));
#69201=CARTESIAN_POINT('',(10.9,23.8513958357493,29.5917795457861));
#69202=CARTESIAN_POINT('',(10.9,23.8513958357493,29.5917795457861));
#69203=CARTESIAN_POINT('',(4.5,23.5449780585017,29.8488945896607));
#69204=CARTESIAN_POINT('',(4.5,23.5449780585017,29.8488945896607));
#69205=CARTESIAN_POINT('',(4.5,23.1619558369422,30.170288394504));
#69206=CARTESIAN_POINT('',(4.5,23.1619558369422,30.170288394504));
#69207=CARTESIAN_POINT('',(1.9,23.1619558369422,30.170288394504));
#69208=CARTESIAN_POINT('',(1.9,23.1619558369422,30.170288394504));
#69209=CARTESIAN_POINT('',(1.57538060255632,23.3779086059641,29.989082505666));
#69210=CARTESIAN_POINT('',(0.,24.4259291680885,29.1096888385212));
#69211=CARTESIAN_POINT('',(1.57538060255632,25.4739497302129,28.2302951713764));
#69212=CARTESIAN_POINT('Ctrl Pts',(1.57538060255632,23.3779086059641,29.989082505666));
#69213=CARTESIAN_POINT('Ctrl Pts',(1.62460345738085,24.4259291681124,29.1096888385011));
#69214=CARTESIAN_POINT('Ctrl Pts',(1.57538060255632,25.4739497302129,28.2302951713764));
#69215=CARTESIAN_POINT('',(1.9,25.6899024992348,28.0490892825384));
#69216=CARTESIAN_POINT('',(1.9,25.6899024992348,28.0490892825384));
#69217=CARTESIAN_POINT('',(4.5,25.6899024992348,28.0490892825384));
#69218=CARTESIAN_POINT('',(4.5,25.6899024992348,28.0490892825384));
#69219=CARTESIAN_POINT('',(4.5,25.3068802776753,28.3704830873816));
#69220=CARTESIAN_POINT('',(4.5,25.3068802776753,28.3704830873816));
#69221=CARTESIAN_POINT('',(10.9,25.0004625004277,28.6275981312563));
#69222=CARTESIAN_POINT('',(10.9,25.0004625004277,28.6275981312563));
#69223=CARTESIAN_POINT('',(11.9,25.2302758333634,28.4347618483503));
#69224=CARTESIAN_POINT('',(11.9,25.2302758333634,28.4347618483503));
#69225=CARTESIAN_POINT('',(12.6,25.536693610611,28.1776468044757));
#69226=CARTESIAN_POINT('',(12.6,25.536693610611,28.1776468044757));
#69227=CARTESIAN_POINT('',(13.2,25.6899024992348,28.0490892825384));
#69228=CARTESIAN_POINT('',(13.2,25.6899024992348,28.0490892825384));
#69229=CARTESIAN_POINT('',(21.8,25.6899024992348,28.0490892825384));
#69230=CARTESIAN_POINT('',(21.8,25.6899024992348,28.0490892825384));
#69231=CARTESIAN_POINT('',(22.4,25.536693610611,28.1776468044757));
#69232=CARTESIAN_POINT('',(22.4,25.536693610611,28.1776468044757));
#69233=CARTESIAN_POINT('',(23.1,25.2302758333634,28.4347618483503));
#69234=CARTESIAN_POINT('',(23.1,25.2302758333634,28.4347618483503));
#69235=CARTESIAN_POINT('',(24.1,25.0004625004277,28.6275981312563));
#69236=CARTESIAN_POINT('',(24.1,25.0004625004277,28.6275981312563));
#69237=CARTESIAN_POINT('',(30.5,25.3068802776753,28.3704830873816));
#69238=CARTESIAN_POINT('',(30.5,25.3068802776753,28.3704830873816));
#69239=CARTESIAN_POINT('',(30.5,25.6899024992348,28.0490892825384));
#69240=CARTESIAN_POINT('',(30.5,25.6899024992348,28.0490892825384));
#69241=CARTESIAN_POINT('',(33.1,25.6899024992348,28.0490892825384));
#69242=CARTESIAN_POINT('',(33.1,25.6899024992348,28.0490892825384));
#69243=CARTESIAN_POINT('',(35.,24.4259291680885,29.1096888385212));
#69244=CARTESIAN_POINT('Origin',(35.,24.4259291680885,29.1096888385212));
#69245=CARTESIAN_POINT('',(35.,26.8018655926851,33.3167260852698));
#69246=CARTESIAN_POINT('',(35.,21.5277259351931,23.97788109181));
#69247=CARTESIAN_POINT('',(34.8617922858584,26.7099230322463,33.3938750538235));
#69248=CARTESIAN_POINT('',(33.5377160618333,25.8290824872081,34.132988030291));
#69249=CARTESIAN_POINT('',(34.4,26.1673599741116,33.234910440458));
#69250=CARTESIAN_POINT('Ctrl Pts',(34.4,26.1673599741116,33.234910440458));
#69251=CARTESIAN_POINT('Ctrl Pts',(34.6297825291018,26.4376444612473,33.314560708072));
#69252=CARTESIAN_POINT('Ctrl Pts',(34.8617922858584,26.7099230322463,33.3938750538235));
#69253=CARTESIAN_POINT('',(33.3226453080309,25.4310730087083,33.8016349549212));
#69254=CARTESIAN_POINT('Origin',(26.8550245390365,0.,0.));
#69255=CARTESIAN_POINT('',(33.0966075166785,23.1273809239214,30.1149569673582));
#69256=CARTESIAN_POINT('Origin',(17.5,19.,32.9089653438087));
#69257=CARTESIAN_POINT('',(33.1,17.5710580837557,33.7339653438087));
#69258=CARTESIAN_POINT('',(33.1,17.5710580837557,33.7339653438087));
#69259=CARTESIAN_POINT('',(30.5,17.5710580837557,33.7339653438087));
#69260=CARTESIAN_POINT('',(30.5,17.5710580837557,33.7339653438087));
#69261=CARTESIAN_POINT('',(30.5,18.0040707856479,33.4839653438087));
#69262=CARTESIAN_POINT('',(30.5,18.0040707856479,33.4839653438087));
#69263=CARTESIAN_POINT('',(24.1,18.3504809471617,33.2839653438087));
#69264=CARTESIAN_POINT('',(24.1,18.3504809471617,33.2839653438087));
#69265=CARTESIAN_POINT('',(23.1,18.0906733260263,33.4339653438087));
#69266=CARTESIAN_POINT('',(23.1,18.0906733260263,33.4339653438087));
#69267=CARTESIAN_POINT('',(22.4,17.7442631645126,33.6339653438087));
#69268=CARTESIAN_POINT('',(22.4,17.7442631645126,33.6339653438087));
#69269=CARTESIAN_POINT('',(21.8,17.5710580837557,33.7339653438087));
#69270=CARTESIAN_POINT('',(21.8,17.5710580837557,33.7339653438087));
#69271=CARTESIAN_POINT('',(13.2,17.5710580837557,33.7339653438087));
#69272=CARTESIAN_POINT('',(13.2,17.5710580837557,33.7339653438087));
#69273=CARTESIAN_POINT('',(12.6,17.7442631645126,33.6339653438087));
#69274=CARTESIAN_POINT('',(12.6,17.7442631645126,33.6339653438087));
#69275=CARTESIAN_POINT('',(11.9,18.0906733260263,33.4339653438087));
#69276=CARTESIAN_POINT('',(11.9,18.0906733260263,33.4339653438087));
#69277=CARTESIAN_POINT('',(10.9,18.3504809471617,33.2839653438087));
#69278=CARTESIAN_POINT('',(10.9,18.3504809471617,33.2839653438087));
#69279=CARTESIAN_POINT('',(4.5,18.0040707856479,33.4839653438087));
#69280=CARTESIAN_POINT('',(4.5,18.0040707856479,33.4839653438087));
#69281=CARTESIAN_POINT('',(4.5,17.5710580837557,33.7339653438087));
#69282=CARTESIAN_POINT('',(4.5,17.5710580837557,33.7339653438087));
#69283=CARTESIAN_POINT('',(1.9,17.5710580837557,33.7339653438087));
#69284=CARTESIAN_POINT('',(1.9,17.5710580837557,33.7339653438087));
#69285=CARTESIAN_POINT('',(1.57538060255632,17.8151961173521,33.5930121843923));
#69286=CARTESIAN_POINT('',(0.,19.,32.9089653438087));
#69287=CARTESIAN_POINT('',(1.57538060255632,20.1848038826479,32.224918503225));
#69288=CARTESIAN_POINT('Ctrl Pts',(1.57538060255632,17.8151961173521,33.5930121843923));
#69289=CARTESIAN_POINT('Ctrl Pts',(1.62460345738085,19.000000000027,32.9089653437931));
#69290=CARTESIAN_POINT('Ctrl Pts',(1.57538060255632,20.1848038826479,32.224918503225));
#69291=CARTESIAN_POINT('',(1.9,20.4289419162443,32.0839653438087));
#69292=CARTESIAN_POINT('',(1.9,20.4289419162443,32.0839653438087));
#69293=CARTESIAN_POINT('',(4.5,20.4289419162443,32.0839653438087));
#69294=CARTESIAN_POINT('',(4.5,20.4289419162443,32.0839653438087));
#69295=CARTESIAN_POINT('',(4.5,19.9959292143521,32.3339653438087));
#69296=CARTESIAN_POINT('',(4.5,19.9959292143521,32.3339653438087));
#69297=CARTESIAN_POINT('',(10.9,19.6495190528383,32.5339653438087));
#69298=CARTESIAN_POINT('',(10.9,19.6495190528383,32.5339653438087));
#69299=CARTESIAN_POINT('',(11.9,19.9093266739737,32.3839653438087));
#69300=CARTESIAN_POINT('',(11.9,19.9093266739737,32.3839653438087));
#69301=CARTESIAN_POINT('',(12.6,20.2557368354874,32.1839653438087));
#69302=CARTESIAN_POINT('',(12.6,20.2557368354874,32.1839653438087));
#69303=CARTESIAN_POINT('',(13.2,20.4289419162443,32.0839653438087));
#69304=CARTESIAN_POINT('',(13.2,20.4289419162443,32.0839653438087));
#69305=CARTESIAN_POINT('',(21.8,20.4289419162443,32.0839653438087));
#69306=CARTESIAN_POINT('',(21.8,20.4289419162443,32.0839653438087));
#69307=CARTESIAN_POINT('',(22.4,20.2557368354874,32.1839653438087));
#69308=CARTESIAN_POINT('',(22.4,20.2557368354874,32.1839653438087));
#69309=CARTESIAN_POINT('',(23.1,19.9093266739737,32.3839653438087));
#69310=CARTESIAN_POINT('',(23.1,19.9093266739737,32.3839653438087));
#69311=CARTESIAN_POINT('',(24.1,19.6495190528383,32.5339653438087));
#69312=CARTESIAN_POINT('',(24.1,19.6495190528383,32.5339653438087));
#69313=CARTESIAN_POINT('',(30.5,19.9959292143521,32.3339653438087));
#69314=CARTESIAN_POINT('',(30.5,19.9959292143521,32.3339653438087));
#69315=CARTESIAN_POINT('',(30.5,20.4289419162443,32.0839653438087));
#69316=CARTESIAN_POINT('',(30.5,20.4289419162443,32.0839653438087));
#69317=CARTESIAN_POINT('',(33.1,20.4289419162443,32.0839653438087));
#69318=CARTESIAN_POINT('',(33.1,20.4289419162443,32.0839653438087));
#69319=CARTESIAN_POINT('',(35.,19.,32.9089653438087));
#69320=CARTESIAN_POINT('Origin',(35.,19.,32.9089653438087));
#69321=CARTESIAN_POINT('',(35.,20.6092962603321,37.4646652720015));
#69322=CARTESIAN_POINT('',(35.,15.6628468484386,23.4619363860708));
#69323=CARTESIAN_POINT('',(34.8617922858584,20.5053537361819,37.5246765162999));
#69324=CARTESIAN_POINT('',(33.5377160618333,19.5095495168072,38.099604350416));
#69325=CARTESIAN_POINT('',(34.4,19.9986373454573,37.2739118462884));
#69326=CARTESIAN_POINT('Ctrl Pts',(34.4,19.9986373454573,37.2739118462884));
#69327=CARTESIAN_POINT('Ctrl Pts',(34.6297825291024,20.2509844800861,37.3992864560073));
#69328=CARTESIAN_POINT('Ctrl Pts',(34.8617922858584,20.5053537361819,37.5246765162999));
#69329=CARTESIAN_POINT('',(33.3226453080309,19.1751255543105,37.7041716521717));
#69330=CARTESIAN_POINT('Origin',(26.8550245390365,0.,0.));
#69331=CARTESIAN_POINT('',(33.0966075166785,17.5466166428447,33.6734706547313));
#69332=CARTESIAN_POINT('Origin',(17.5,12.9967654463754,35.7083195898645));
#69333=CARTESIAN_POINT('',(33.1,11.4462726220787,36.2726528263519));
#69334=CARTESIAN_POINT('',(33.1,11.4462726220787,36.2726528263519));
#69335=CARTESIAN_POINT('',(30.5,11.4462726220787,36.2726528263519));
#69336=CARTESIAN_POINT('',(30.5,11.4462726220787,36.2726528263519));
#69337=CARTESIAN_POINT('',(30.5,11.9161189324716,36.101642754689));
#69338=CARTESIAN_POINT('',(30.5,11.9161189324716,36.101642754689));
#69339=CARTESIAN_POINT('',(24.1,12.291995980786,35.9648346973588));
#69340=CARTESIAN_POINT('',(24.1,12.291995980786,35.9648346973588));
#69341=CARTESIAN_POINT('',(23.1,12.0100881945502,36.0674407403565));
#69342=CARTESIAN_POINT('',(23.1,12.0100881945502,36.0674407403565));
#69343=CARTESIAN_POINT('',(22.4,11.6342111462359,36.2042487976867));
#69344=CARTESIAN_POINT('',(22.4,11.6342111462359,36.2042487976867));
#69345=CARTESIAN_POINT('',(21.8,11.4462726220787,36.2726528263519));
#69346=CARTESIAN_POINT('',(21.8,11.4462726220787,36.2726528263519));
#69347=CARTESIAN_POINT('',(13.2,11.4462726220787,36.2726528263519));
#69348=CARTESIAN_POINT('',(13.2,11.4462726220787,36.2726528263519));
#69349=CARTESIAN_POINT('',(12.6,11.6342111462359,36.2042487976867));
#69350=CARTESIAN_POINT('',(12.6,11.6342111462359,36.2042487976867));
#69351=CARTESIAN_POINT('',(11.9,12.0100881945502,36.0674407403565));
#69352=CARTESIAN_POINT('',(11.9,12.0100881945502,36.0674407403565));
#69353=CARTESIAN_POINT('',(10.9,12.291995980786,35.9648346973588));
#69354=CARTESIAN_POINT('',(10.9,12.291995980786,35.9648346973588));
#69355=CARTESIAN_POINT('',(4.5,11.9161189324716,36.101642754689));
#69356=CARTESIAN_POINT('',(4.5,11.9161189324716,36.101642754689));
#69357=CARTESIAN_POINT('',(4.5,11.4462726220787,36.2726528263519));
#69358=CARTESIAN_POINT('',(4.5,11.4462726220787,36.2726528263519));
#69359=CARTESIAN_POINT('',(1.9,11.4462726220787,36.2726528263519));
#69360=CARTESIAN_POINT('',(1.9,11.4462726220787,36.2726528263519));
#69361=CARTESIAN_POINT('',(1.57538060255632,11.7111779096386,36.1762351867803));
#69362=CARTESIAN_POINT('',(0.,12.9967654463754,35.7083195898645));
#69363=CARTESIAN_POINT('',(1.57538060255633,14.2823529831122,35.2404039929487));
#69364=CARTESIAN_POINT('Ctrl Pts',(1.57538060255632,11.7111779096386,36.1762351867803));
#69365=CARTESIAN_POINT('Ctrl Pts',(1.62460345738085,12.9967654464047,35.7083195898538));
#69366=CARTESIAN_POINT('Ctrl Pts',(1.57538060255633,14.2823529831122,35.2404039929487));
#69367=CARTESIAN_POINT('',(1.9,14.5472582706722,35.1439863533772));
#69368=CARTESIAN_POINT('',(1.9,14.5472582706722,35.1439863533772));
#69369=CARTESIAN_POINT('',(4.5,14.5472582706722,35.1439863533772));
#69370=CARTESIAN_POINT('',(4.5,14.5472582706722,35.1439863533772));
#69371=CARTESIAN_POINT('',(4.5,14.0774119602792,35.31499642504));
#69372=CARTESIAN_POINT('',(4.5,14.0774119602792,35.31499642504));
#69373=CARTESIAN_POINT('',(10.9,13.7015349119648,35.4518044823703));
#69374=CARTESIAN_POINT('',(10.9,13.7015349119648,35.4518044823703));
#69375=CARTESIAN_POINT('',(11.9,13.9834426982006,35.3491984393726));
#69376=CARTESIAN_POINT('',(11.9,13.9834426982006,35.3491984393726));
#69377=CARTESIAN_POINT('',(12.6,14.359319746515,35.2123903820423));
#69378=CARTESIAN_POINT('',(12.6,14.359319746515,35.2123903820423));
#69379=CARTESIAN_POINT('',(13.2,14.5472582706722,35.1439863533772));
#69380=CARTESIAN_POINT('',(13.2,14.5472582706722,35.1439863533772));
#69381=CARTESIAN_POINT('',(21.8,14.5472582706722,35.1439863533772));
#69382=CARTESIAN_POINT('',(21.8,14.5472582706722,35.1439863533772));
#69383=CARTESIAN_POINT('',(22.4,14.359319746515,35.2123903820423));
#69384=CARTESIAN_POINT('',(22.4,14.359319746515,35.2123903820423));
#69385=CARTESIAN_POINT('',(23.1,13.9834426982006,35.3491984393726));
#69386=CARTESIAN_POINT('',(23.1,13.9834426982006,35.3491984393726));
#69387=CARTESIAN_POINT('',(24.1,13.7015349119648,35.4518044823703));
#69388=CARTESIAN_POINT('',(24.1,13.7015349119648,35.4518044823703));
#69389=CARTESIAN_POINT('',(30.5,14.0774119602792,35.31499642504));
#69390=CARTESIAN_POINT('',(30.5,14.0774119602792,35.31499642504));
#69391=CARTESIAN_POINT('',(30.5,14.5472582706722,35.1439863533772));
#69392=CARTESIAN_POINT('',(30.5,14.5472582706722,35.1439863533772));
#69393=CARTESIAN_POINT('',(33.1,14.5472582706722,35.1439863533772));
#69394=CARTESIAN_POINT('',(33.1,14.5472582706722,35.1439863533772));
#69395=CARTESIAN_POINT('',(35.,12.9967654463754,35.7083195898645));
#69396=CARTESIAN_POINT('Origin',(35.,12.9967654463754,35.7083195898645));
#69397=CARTESIAN_POINT('',(35.,13.790523889916,40.4742595624789));
#69398=CARTESIAN_POINT('',(35.,10.6297856612634,21.4963339863891));
#69399=CARTESIAN_POINT('',(34.8617922858584,13.6777396430533,40.515309671231));
#69400=CARTESIAN_POINT('',(33.5377160618333,12.5972287566465,40.9085834716837));
#69401=CARTESIAN_POINT('',(34.4,13.22226624086,40.1803643021789));
#69402=CARTESIAN_POINT('Ctrl Pts',(34.4,13.22226624086,40.1803643021789));
#69403=CARTESIAN_POINT('Ctrl Pts',(34.6297825291026,13.4490085829898,40.3476538099288));
#69404=CARTESIAN_POINT('Ctrl Pts',(34.8617922858584,13.6777396430533,40.515309671231));
#69405=CARTESIAN_POINT('',(33.3226453080309,12.3365516130268,40.4610861730024));
#69406=CARTESIAN_POINT('Origin',(26.8550245390365,0.,0.));
#69407=CARTESIAN_POINT('',(33.0966075166785,11.4327072940915,36.2088329758587));
#69408=CARTESIAN_POINT('Origin',(17.5,6.59863075134336,37.4226946144639));
#69409=CARTESIAN_POINT('',(33.1,4.97369795887321,37.7092141076143));
#69410=CARTESIAN_POINT('',(33.1,4.97369795887321,37.7092141076143));
#69411=CARTESIAN_POINT('',(30.5,4.97369795887321,37.7092141076143));
#69412=CARTESIAN_POINT('',(30.5,4.97369795887321,37.7092141076143));
#69413=CARTESIAN_POINT('',(30.5,5.46610183537932,37.6223900187809));
#69414=CARTESIAN_POINT('',(30.5,5.46610183537932,37.6223900187809));
#69415=CARTESIAN_POINT('',(24.1,5.8600249365842,37.5529307477141));
#69416=CARTESIAN_POINT('',(24.1,5.8600249365842,37.5529307477141));
#69417=CARTESIAN_POINT('',(23.1,5.56458261068054,37.6050252010142));
#69418=CARTESIAN_POINT('',(23.1,5.56458261068054,37.6050252010142));
#69419=CARTESIAN_POINT('',(22.4,5.17065950947566,37.674484472081));
#69420=CARTESIAN_POINT('',(22.4,5.17065950947566,37.674484472081));
#69421=CARTESIAN_POINT('',(21.8,4.97369795887321,37.7092141076143));
#69422=CARTESIAN_POINT('',(21.8,4.97369795887321,37.7092141076143));
#69423=CARTESIAN_POINT('',(13.2,4.97369795887321,37.7092141076143));
#69424=CARTESIAN_POINT('',(13.2,4.97369795887321,37.7092141076143));
#69425=CARTESIAN_POINT('',(12.6,5.17065950947566,37.674484472081));
#69426=CARTESIAN_POINT('',(12.6,5.17065950947566,37.674484472081));
#69427=CARTESIAN_POINT('',(11.9,5.56458261068054,37.6050252010142));
#69428=CARTESIAN_POINT('',(11.9,5.56458261068054,37.6050252010142));
#69429=CARTESIAN_POINT('',(10.9,5.8600249365842,37.5529307477141));
#69430=CARTESIAN_POINT('',(10.9,5.8600249365842,37.5529307477141));
#69431=CARTESIAN_POINT('',(4.5,5.46610183537932,37.6223900187809));
#69432=CARTESIAN_POINT('',(4.5,5.46610183537932,37.6223900187809));
#69433=CARTESIAN_POINT('',(4.5,4.97369795887321,37.7092141076143));
#69434=CARTESIAN_POINT('',(4.5,4.97369795887321,37.7092141076143));
#69435=CARTESIAN_POINT('',(1.9,4.97369795887321,37.7092141076143));
#69436=CARTESIAN_POINT('',(1.9,4.97369795887321,37.7092141076143));
#69437=CARTESIAN_POINT('',(1.57538060255632,5.25132148728276,37.6602615890763));
#69438=CARTESIAN_POINT('',(0.,6.59863075134336,37.4226946144639));
#69439=CARTESIAN_POINT('',(1.57538060255632,7.94594001540395,37.1851276398516));
#69440=CARTESIAN_POINT('Ctrl Pts',(1.57538060255632,5.25132148728276,37.6602615890763));
#69441=CARTESIAN_POINT('Ctrl Pts',(1.62460345738085,6.59863075137406,37.4226946144585));
#69442=CARTESIAN_POINT('Ctrl Pts',(1.57538060255632,7.94594001540395,37.1851276398516));
#69443=CARTESIAN_POINT('',(1.9,8.2235635438135,37.1361751213135));
#69444=CARTESIAN_POINT('',(1.9,8.2235635438135,37.1361751213135));
#69445=CARTESIAN_POINT('',(4.5,8.2235635438135,37.1361751213135));
#69446=CARTESIAN_POINT('',(4.5,8.2235635438135,37.1361751213135));
#69447=CARTESIAN_POINT('',(4.5,7.7311596673074,37.2229992101469));
#69448=CARTESIAN_POINT('',(4.5,7.7311596673074,37.2229992101469));
#69449=CARTESIAN_POINT('',(10.9,7.33723656610251,37.2924584812137));
#69450=CARTESIAN_POINT('',(10.9,7.33723656610251,37.2924584812137));
#69451=CARTESIAN_POINT('',(11.9,7.63267889200617,37.2403640279136));
#69452=CARTESIAN_POINT('',(11.9,7.63267889200617,37.2403640279136));
#69453=CARTESIAN_POINT('',(12.6,8.02660199321106,37.1709047568469));
#69454=CARTESIAN_POINT('',(12.6,8.02660199321106,37.1709047568469));
#69455=CARTESIAN_POINT('',(13.2,8.2235635438135,37.1361751213135));
#69456=CARTESIAN_POINT('',(13.2,8.2235635438135,37.1361751213135));
#69457=CARTESIAN_POINT('',(21.8,8.2235635438135,37.1361751213135));
#69458=CARTESIAN_POINT('',(21.8,8.2235635438135,37.1361751213135));
#69459=CARTESIAN_POINT('',(22.4,8.02660199321106,37.1709047568469));
#69460=CARTESIAN_POINT('',(22.4,8.02660199321106,37.1709047568469));
#69461=CARTESIAN_POINT('',(23.1,7.63267889200617,37.2403640279136));
#69462=CARTESIAN_POINT('',(23.1,7.63267889200617,37.2403640279136));
#69463=CARTESIAN_POINT('',(24.1,7.33723656610251,37.2924584812137));
#69464=CARTESIAN_POINT('',(24.1,7.33723656610251,37.2924584812137));
#69465=CARTESIAN_POINT('',(30.5,7.7311596673074,37.2229992101469));
#69466=CARTESIAN_POINT('',(30.5,7.7311596673074,37.2229992101469));
#69467=CARTESIAN_POINT('',(30.5,8.2235635438135,37.1361751213135));
#69468=CARTESIAN_POINT('',(30.5,8.2235635438135,37.1361751213135));
#69469=CARTESIAN_POINT('',(33.1,8.2235635438135,37.1361751213135));
#69470=CARTESIAN_POINT('',(33.1,8.2235635438135,37.1361751213135));
#69471=CARTESIAN_POINT('',(35.,6.59863075134336,37.4226946144639));
#69472=CARTESIAN_POINT('Origin',(35.,6.59863075134336,37.4226946144639));
#69473=CARTESIAN_POINT('',(35.,6.55273342944653,42.2540639571139));
#69474=CARTESIAN_POINT('',(35.,6.77841834076261,18.497401987115));
#69475=CARTESIAN_POINT('',(34.8617922858584,6.4345343521407,42.2749056435377));
#69476=CARTESIAN_POINT('',(33.5377160618333,5.30214757522047,42.4745759849063));
#69477=CARTESIAN_POINT('',(34.4,6.04414326732376,41.8659567209931));
#69478=CARTESIAN_POINT('Ctrl Pts',(34.4,6.04414326732376,41.8659567209931));
#69479=CARTESIAN_POINT('Ctrl Pts',(34.6297825290984,6.23839136562223,42.0700781197299));
#69480=CARTESIAN_POINT('Ctrl Pts',(34.8617922858584,6.4345343521407,42.2749056435377));
#69481=CARTESIAN_POINT('',(33.3226453080309,5.12313779357752,41.9886110647639));
#69482=CARTESIAN_POINT('Origin',(26.8550245390365,0.,0.));
#69483=CARTESIAN_POINT('',(33.0966075166785,4.97142091943645,37.6440082295681));
#69484=CARTESIAN_POINT('Origin',(17.5,2.32682891837997E-15,38.));
#69485=CARTESIAN_POINT('',(33.1,-1.65,38.));
#69486=CARTESIAN_POINT('',(33.1,-1.65,38.));
#69487=CARTESIAN_POINT('',(30.5,-1.65,38.));
#69488=CARTESIAN_POINT('',(30.5,-1.65,38.));
#69489=CARTESIAN_POINT('',(30.5,-1.15,38.));
#69490=CARTESIAN_POINT('',(30.5,-1.15,38.));
#69491=CARTESIAN_POINT('',(24.1,-0.749999999999998,38.));
#69492=CARTESIAN_POINT('',(24.1,-0.749999999999998,38.));
#69493=CARTESIAN_POINT('',(23.1,-1.05,38.));
#69494=CARTESIAN_POINT('',(23.1,-1.05,38.));
#69495=CARTESIAN_POINT('',(22.4,-1.45,38.));
#69496=CARTESIAN_POINT('',(22.4,-1.45,38.));
#69497=CARTESIAN_POINT('',(21.8,-1.65,38.));
#69498=CARTESIAN_POINT('',(21.8,-1.65,38.));
#69499=CARTESIAN_POINT('',(13.2,-1.65,38.));
#69500=CARTESIAN_POINT('',(13.2,-1.65,38.));
#69501=CARTESIAN_POINT('',(12.6,-1.45,38.));
#69502=CARTESIAN_POINT('',(12.6,-1.45,38.));
#69503=CARTESIAN_POINT('',(11.9,-1.05,38.));
#69504=CARTESIAN_POINT('',(11.9,-1.05,38.));
#69505=CARTESIAN_POINT('',(10.9,-0.749999999999998,38.));
#69506=CARTESIAN_POINT('',(10.9,-0.749999999999998,38.));
#69507=CARTESIAN_POINT('',(4.5,-1.15,38.));
#69508=CARTESIAN_POINT('',(4.5,-1.15,38.));
#69509=CARTESIAN_POINT('',(4.5,-1.65,38.));
#69510=CARTESIAN_POINT('',(4.5,-1.65,38.));
#69511=CARTESIAN_POINT('',(1.9,-1.65,38.));
#69512=CARTESIAN_POINT('',(1.9,-1.65,38.));
#69513=CARTESIAN_POINT('',(1.57538060255632,-1.36809368116733,38.));
#69514=CARTESIAN_POINT('',(0.,2.32682891837997E-15,38.));
#69515=CARTESIAN_POINT('',(1.57538060255633,1.36809368116734,38.));
#69516=CARTESIAN_POINT('Ctrl Pts',(1.57538060255632,-1.36809368116733,38.));
#69517=CARTESIAN_POINT('Ctrl Pts',(1.62460345738085,3.1181446313866E-11,
38.));
#69518=CARTESIAN_POINT('Ctrl Pts',(1.57538060255633,1.36809368116734,38.));
#69519=CARTESIAN_POINT('',(1.9,1.65,38.));
#69520=CARTESIAN_POINT('',(1.9,1.65,38.));
#69521=CARTESIAN_POINT('',(4.5,1.65,38.));
#69522=CARTESIAN_POINT('',(4.5,1.65,38.));
#69523=CARTESIAN_POINT('',(4.5,1.15,38.));
#69524=CARTESIAN_POINT('',(4.5,1.15,38.));
#69525=CARTESIAN_POINT('',(10.9,0.750000000000002,38.));
#69526=CARTESIAN_POINT('',(10.9,0.750000000000002,38.));
#69527=CARTESIAN_POINT('',(11.9,1.05,38.));
#69528=CARTESIAN_POINT('',(11.9,1.05,38.));
#69529=CARTESIAN_POINT('',(12.6,1.45,38.));
#69530=CARTESIAN_POINT('',(12.6,1.45,38.));
#69531=CARTESIAN_POINT('',(13.2,1.65,38.));
#69532=CARTESIAN_POINT('',(13.2,1.65,38.));
#69533=CARTESIAN_POINT('',(21.8,1.65,38.));
#69534=CARTESIAN_POINT('',(21.8,1.65,38.));
#69535=CARTESIAN_POINT('',(22.4,1.45,38.));
#69536=CARTESIAN_POINT('',(22.4,1.45,38.));
#69537=CARTESIAN_POINT('',(23.1,1.05,38.));
#69538=CARTESIAN_POINT('',(23.1,1.05,38.));
#69539=CARTESIAN_POINT('',(24.1,0.750000000000002,38.));
#69540=CARTESIAN_POINT('',(24.1,0.750000000000002,38.));
#69541=CARTESIAN_POINT('',(30.5,1.15,38.));
#69542=CARTESIAN_POINT('',(30.5,1.15,38.));
#69543=CARTESIAN_POINT('',(30.5,1.65,38.));
#69544=CARTESIAN_POINT('',(30.5,1.65,38.));
#69545=CARTESIAN_POINT('',(33.1,1.65,38.));
#69546=CARTESIAN_POINT('',(33.1,1.65,38.));
#69547=CARTESIAN_POINT('',(35.,2.32682891837997E-15,38.));
#69548=CARTESIAN_POINT('Origin',(35.,2.32682891837997E-15,38.));
#69549=CARTESIAN_POINT('',(35.,-0.884158520433533,42.75));
#69550=CARTESIAN_POINT('',(35.,4.28887236871593,14.95872031928));
#69551=CARTESIAN_POINT('',(34.8617922858584,-1.0041810090302,42.75));
#69552=CARTESIAN_POINT('',(33.5377160618333,-2.15403667726254,42.75));
#69553=CARTESIAN_POINT('',(34.4,-1.31762794090604,42.2794732300362));
#69554=CARTESIAN_POINT('Ctrl Pts',(34.4,-1.31762794090604,42.2794732300361));
#69555=CARTESIAN_POINT('Ctrl Pts',(34.6297825291,-1.16177621660623,42.5142243943543));
#69556=CARTESIAN_POINT('Ctrl Pts',(34.8617922858584,-1.0041810090302,42.75));
#69557=CARTESIAN_POINT('',(33.3226453080309,-2.24593997529677,42.240333256585));
#69558=CARTESIAN_POINT('Origin',(26.8550245390365,0.,0.));
#69559=CARTESIAN_POINT('',(33.0966075166785,-1.64091956419533,37.9353893420094));
#69560=CARTESIAN_POINT('Origin',(17.5,-6.59863075134335,37.4226946144639));
#69561=CARTESIAN_POINT('',(33.1,-8.22356354381349,37.1361751213135));
#69562=CARTESIAN_POINT('',(33.1,-8.22356354381349,37.1361751213135));
#69563=CARTESIAN_POINT('',(30.5,-8.22356354381349,37.1361751213135));
#69564=CARTESIAN_POINT('',(30.5,-8.22356354381349,37.1361751213135));
#69565=CARTESIAN_POINT('',(30.5,-7.73115966730739,37.2229992101469));
#69566=CARTESIAN_POINT('',(30.5,-7.73115966730739,37.2229992101469));
#69567=CARTESIAN_POINT('',(24.1,-7.33723656610251,37.2924584812137));
#69568=CARTESIAN_POINT('',(24.1,-7.33723656610251,37.2924584812137));
#69569=CARTESIAN_POINT('',(23.1,-7.63267889200617,37.2403640279136));
#69570=CARTESIAN_POINT('',(23.1,-7.63267889200617,37.2403640279136));
#69571=CARTESIAN_POINT('',(22.4,-8.02660199321105,37.1709047568469));
#69572=CARTESIAN_POINT('',(22.4,-8.02660199321105,37.1709047568469));
#69573=CARTESIAN_POINT('',(21.8,-8.22356354381349,37.1361751213135));
#69574=CARTESIAN_POINT('',(21.8,-8.22356354381349,37.1361751213135));
#69575=CARTESIAN_POINT('',(13.2,-8.22356354381349,37.1361751213135));
#69576=CARTESIAN_POINT('',(13.2,-8.22356354381349,37.1361751213135));
#69577=CARTESIAN_POINT('',(12.6,-8.02660199321105,37.1709047568469));
#69578=CARTESIAN_POINT('',(12.6,-8.02660199321105,37.1709047568469));
#69579=CARTESIAN_POINT('',(11.9,-7.63267889200617,37.2403640279136));
#69580=CARTESIAN_POINT('',(11.9,-7.63267889200617,37.2403640279136));
#69581=CARTESIAN_POINT('',(10.9,-7.33723656610251,37.2924584812137));
#69582=CARTESIAN_POINT('',(10.9,-7.33723656610251,37.2924584812137));
#69583=CARTESIAN_POINT('',(4.5,-7.73115966730739,37.2229992101469));
#69584=CARTESIAN_POINT('',(4.5,-7.73115966730739,37.2229992101469));
#69585=CARTESIAN_POINT('',(4.5,-8.22356354381349,37.1361751213135));
#69586=CARTESIAN_POINT('',(4.5,-8.22356354381349,37.1361751213135));
#69587=CARTESIAN_POINT('',(1.9,-8.22356354381349,37.1361751213135));
#69588=CARTESIAN_POINT('',(1.9,-8.22356354381349,37.1361751213135));
#69589=CARTESIAN_POINT('',(1.57538060255632,-7.94594001540396,37.1851276398516));
#69590=CARTESIAN_POINT('',(0.,-6.59863075134335,37.4226946144639));
#69591=CARTESIAN_POINT('',(1.57538060255632,-5.25132148728275,37.6602615890763));
#69592=CARTESIAN_POINT('Ctrl Pts',(1.57538060255632,-7.94594001540396,37.1851276398516));
#69593=CARTESIAN_POINT('Ctrl Pts',(1.62460345738085,-6.59863075131265,37.4226946144693));
#69594=CARTESIAN_POINT('Ctrl Pts',(1.57538060255632,-5.25132148728275,37.6602615890763));
#69595=CARTESIAN_POINT('',(1.9,-4.97369795887321,37.7092141076143));
#69596=CARTESIAN_POINT('',(1.9,-4.97369795887321,37.7092141076143));
#69597=CARTESIAN_POINT('',(4.5,-4.97369795887321,37.7092141076143));
#69598=CARTESIAN_POINT('',(4.5,-4.97369795887321,37.7092141076143));
#69599=CARTESIAN_POINT('',(4.5,-5.46610183537931,37.6223900187809));
#69600=CARTESIAN_POINT('',(4.5,-5.46610183537931,37.6223900187809));
#69601=CARTESIAN_POINT('',(10.9,-5.8600249365842,37.5529307477141));
#69602=CARTESIAN_POINT('',(10.9,-5.8600249365842,37.5529307477141));
#69603=CARTESIAN_POINT('',(11.9,-5.56458261068053,37.6050252010142));
#69604=CARTESIAN_POINT('',(11.9,-5.56458261068053,37.6050252010142));
#69605=CARTESIAN_POINT('',(12.6,-5.17065950947565,37.674484472081));
#69606=CARTESIAN_POINT('',(12.6,-5.17065950947565,37.674484472081));
#69607=CARTESIAN_POINT('',(13.2,-4.97369795887321,37.7092141076143));
#69608=CARTESIAN_POINT('',(13.2,-4.97369795887321,37.7092141076143));
#69609=CARTESIAN_POINT('',(21.8,-4.97369795887321,37.7092141076143));
#69610=CARTESIAN_POINT('',(21.8,-4.97369795887321,37.7092141076143));
#69611=CARTESIAN_POINT('',(22.4,-5.17065950947565,37.674484472081));
#69612=CARTESIAN_POINT('',(22.4,-5.17065950947565,37.674484472081));
#69613=CARTESIAN_POINT('',(23.1,-5.56458261068053,37.6050252010142));
#69614=CARTESIAN_POINT('',(23.1,-5.56458261068053,37.6050252010142));
#69615=CARTESIAN_POINT('',(24.1,-5.8600249365842,37.5529307477141));
#69616=CARTESIAN_POINT('',(24.1,-5.8600249365842,37.5529307477141));
#69617=CARTESIAN_POINT('',(30.5,-5.46610183537931,37.6223900187809));
#69618=CARTESIAN_POINT('',(30.5,-5.46610183537931,37.6223900187809));
#69619=CARTESIAN_POINT('',(30.5,-4.97369795887321,37.7092141076143));
#69620=CARTESIAN_POINT('',(30.5,-4.97369795887321,37.7092141076143));
#69621=CARTESIAN_POINT('',(33.1,-4.97369795887321,37.7092141076143));
#69622=CARTESIAN_POINT('',(33.1,-4.97369795887321,37.7092141076143));
#69623=CARTESIAN_POINT('',(35.,-6.59863075134335,37.4226946144639));
#69624=CARTESIAN_POINT('Origin',(35.,-6.59863075134335,37.4226946144639));
#69625=CARTESIAN_POINT('',(35.,-8.29418576107602,41.9469989254299));
#69626=CARTESIAN_POINT('',(35.,3.1584421883261,11.3875810911838));
#69627=CARTESIAN_POINT('',(34.8617922858584,-8.41238483838184,41.9261572390061));
#69628=CARTESIAN_POINT('',(33.5377160618333,-9.54477161530208,41.7264868976375));
#69629=CARTESIAN_POINT('',(34.4,-8.63936369090332,41.4083493394303));
#69630=CARTESIAN_POINT('Ctrl Pts',(34.4,-8.63936369090333,41.4083493394303));
#69631=CARTESIAN_POINT('Ctrl Pts',(34.6297825291073,-8.52664381637799,41.6665974739986));
#69632=CARTESIAN_POINT('Ctrl Pts',(34.8617922858584,-8.41238483838184,41.9261572390061));
#69633=CARTESIAN_POINT('',(33.3226453080309,-9.54677599452213,41.2086042970448));
#69634=CARTESIAN_POINT('Origin',(26.8550245390365,0.,0.));
#69635=CARTESIAN_POINT('',(33.0966075166785,-8.20340153721441,37.0741228455271));
#69636=CARTESIAN_POINT('Origin',(17.5,-12.9967654463754,35.7083195898645));
#69637=CARTESIAN_POINT('',(33.1,-14.5472582706722,35.1439863533772));
#69638=CARTESIAN_POINT('',(33.1,-14.5472582706722,35.1439863533772));
#69639=CARTESIAN_POINT('',(30.5,-14.5472582706722,35.1439863533772));
#69640=CARTESIAN_POINT('',(30.5,-14.5472582706722,35.1439863533772));
#69641=CARTESIAN_POINT('',(30.5,-14.0774119602792,35.31499642504));
#69642=CARTESIAN_POINT('',(30.5,-14.0774119602792,35.31499642504));
#69643=CARTESIAN_POINT('',(24.1,-13.7015349119648,35.4518044823703));
#69644=CARTESIAN_POINT('',(24.1,-13.7015349119648,35.4518044823703));
#69645=CARTESIAN_POINT('',(23.1,-13.9834426982006,35.3491984393726));
#69646=CARTESIAN_POINT('',(23.1,-13.9834426982006,35.3491984393726));
#69647=CARTESIAN_POINT('',(22.4,-14.359319746515,35.2123903820423));
#69648=CARTESIAN_POINT('',(22.4,-14.359319746515,35.2123903820423));
#69649=CARTESIAN_POINT('',(21.8,-14.5472582706722,35.1439863533772));
#69650=CARTESIAN_POINT('',(21.8,-14.5472582706722,35.1439863533772));
#69651=CARTESIAN_POINT('',(13.2,-14.5472582706722,35.1439863533772));
#69652=CARTESIAN_POINT('',(13.2,-14.5472582706722,35.1439863533772));
#69653=CARTESIAN_POINT('',(12.6,-14.359319746515,35.2123903820423));
#69654=CARTESIAN_POINT('',(12.6,-14.359319746515,35.2123903820423));
#69655=CARTESIAN_POINT('',(11.9,-13.9834426982006,35.3491984393726));
#69656=CARTESIAN_POINT('',(11.9,-13.9834426982006,35.3491984393726));
#69657=CARTESIAN_POINT('',(10.9,-13.7015349119648,35.4518044823703));
#69658=CARTESIAN_POINT('',(10.9,-13.7015349119648,35.4518044823703));
#69659=CARTESIAN_POINT('',(4.5,-14.0774119602792,35.31499642504));
#69660=CARTESIAN_POINT('',(4.5,-14.0774119602792,35.31499642504));
#69661=CARTESIAN_POINT('',(4.5,-14.5472582706722,35.1439863533772));
#69662=CARTESIAN_POINT('',(4.5,-14.5472582706722,35.1439863533772));
#69663=CARTESIAN_POINT('',(1.9,-14.5472582706722,35.1439863533772));
#69664=CARTESIAN_POINT('',(1.9,-14.5472582706722,35.1439863533772));
#69665=CARTESIAN_POINT('',(1.57538060255632,-14.2823529831122,35.2404039929487));
#69666=CARTESIAN_POINT('',(0.,-12.9967654463754,35.7083195898645));
#69667=CARTESIAN_POINT('',(1.57538060255632,-11.7111779096386,36.1762351867803));
#69668=CARTESIAN_POINT('Ctrl Pts',(1.57538060255632,-14.2823529831122,35.2404039929487));
#69669=CARTESIAN_POINT('Ctrl Pts',(1.62460345738085,-12.9967654463461,35.7083195898752));
#69670=CARTESIAN_POINT('Ctrl Pts',(1.57538060255632,-11.7111779096386,36.1762351867803));
#69671=CARTESIAN_POINT('',(1.9,-11.4462726220787,36.2726528263519));
#69672=CARTESIAN_POINT('',(1.9,-11.4462726220787,36.2726528263519));
#69673=CARTESIAN_POINT('',(4.5,-11.4462726220787,36.2726528263519));
#69674=CARTESIAN_POINT('',(4.5,-11.4462726220787,36.2726528263519));
#69675=CARTESIAN_POINT('',(4.5,-11.9161189324716,36.101642754689));
#69676=CARTESIAN_POINT('',(4.5,-11.9161189324716,36.101642754689));
#69677=CARTESIAN_POINT('',(10.9,-12.291995980786,35.9648346973588));
#69678=CARTESIAN_POINT('',(10.9,-12.291995980786,35.9648346973588));
#69679=CARTESIAN_POINT('',(11.9,-12.0100881945502,36.0674407403565));
#69680=CARTESIAN_POINT('',(11.9,-12.0100881945502,36.0674407403565));
#69681=CARTESIAN_POINT('',(12.6,-11.6342111462358,36.2042487976867));
#69682=CARTESIAN_POINT('',(12.6,-11.6342111462358,36.2042487976867));
#69683=CARTESIAN_POINT('',(13.2,-11.4462726220787,36.2726528263519));
#69684=CARTESIAN_POINT('',(13.2,-11.4462726220787,36.2726528263519));
#69685=CARTESIAN_POINT('',(21.8,-11.4462726220787,36.2726528263519));
#69686=CARTESIAN_POINT('',(21.8,-11.4462726220787,36.2726528263519));
#69687=CARTESIAN_POINT('',(22.4,-11.6342111462358,36.2042487976867));
#69688=CARTESIAN_POINT('',(22.4,-11.6342111462358,36.2042487976867));
#69689=CARTESIAN_POINT('',(23.1,-12.0100881945502,36.0674407403565));
#69690=CARTESIAN_POINT('',(23.1,-12.0100881945502,36.0674407403565));
#69691=CARTESIAN_POINT('',(24.1,-12.291995980786,35.9648346973588));
#69692=CARTESIAN_POINT('',(24.1,-12.291995980786,35.9648346973588));
#69693=CARTESIAN_POINT('',(30.5,-11.9161189324716,36.101642754689));
#69694=CARTESIAN_POINT('',(30.5,-11.9161189324716,36.101642754689));
#69695=CARTESIAN_POINT('',(30.5,-11.4462726220787,36.2726528263519));
#69696=CARTESIAN_POINT('',(30.5,-11.4462726220787,36.2726528263519));
#69697=CARTESIAN_POINT('',(33.1,-11.4462726220787,36.2726528263519));
#69698=CARTESIAN_POINT('',(33.1,-11.4462726220787,36.2726528263519));
#69699=CARTESIAN_POINT('',(35.,-12.9967654463754,35.7083195898645));
#69700=CARTESIAN_POINT('Origin',(35.,-12.9967654463754,35.7083195898645));
#69701=CARTESIAN_POINT('',(35.,-15.4521983644287,39.8694595147163));
#69702=CARTESIAN_POINT('',(35.,3.21112147516056,8.24135648498115));
#69703=CARTESIAN_POINT('',(34.8617922858584,-15.5649826112914,39.8284094059642));
#69704=CARTESIAN_POINT('',(33.5377160618333,-16.6454934976981,39.4351356055115));
#69705=CARTESIAN_POINT('',(34.4,-15.6985967468815,39.2790537077817));
#69706=CARTESIAN_POINT('Ctrl Pts',(34.4,-15.6985967468815,39.2790537077817));
#69707=CARTESIAN_POINT('Ctrl Pts',(34.6297825291032,-15.6324336584852,39.5529520736987));
#69708=CARTESIAN_POINT('Ctrl Pts',(34.8617922858584,-15.5649826112914,39.8284094059642));
#69709=CARTESIAN_POINT('',(33.3226453080309,-16.5575380560557,38.9247727484987));
#69710=CARTESIAN_POINT('Origin',(26.8550245390365,0.,0.));
#69711=CARTESIAN_POINT('',(33.0966075166785,-14.5166273056467,35.0863778867947));
#69712=CARTESIAN_POINT('Origin',(17.5,-19.,32.9089653438087));
#69713=CARTESIAN_POINT('',(33.1,-20.4289419162443,32.0839653438087));
#69714=CARTESIAN_POINT('',(33.1,-20.4289419162443,32.0839653438087));
#69715=CARTESIAN_POINT('',(30.5,-20.4289419162443,32.0839653438087));
#69716=CARTESIAN_POINT('',(30.5,-20.4289419162443,32.0839653438087));
#69717=CARTESIAN_POINT('',(30.5,-19.9959292143521,32.3339653438087));
#69718=CARTESIAN_POINT('',(30.5,-19.9959292143521,32.3339653438087));
#69719=CARTESIAN_POINT('',(24.1,-19.6495190528383,32.5339653438087));
#69720=CARTESIAN_POINT('',(24.1,-19.6495190528383,32.5339653438087));
#69721=CARTESIAN_POINT('',(23.1,-19.9093266739737,32.3839653438087));
#69722=CARTESIAN_POINT('',(23.1,-19.9093266739737,32.3839653438087));
#69723=CARTESIAN_POINT('',(22.4,-20.2557368354874,32.1839653438087));
#69724=CARTESIAN_POINT('',(22.4,-20.2557368354874,32.1839653438087));
#69725=CARTESIAN_POINT('',(21.8,-20.4289419162443,32.0839653438087));
#69726=CARTESIAN_POINT('',(21.8,-20.4289419162443,32.0839653438087));
#69727=CARTESIAN_POINT('',(13.2,-20.4289419162443,32.0839653438087));
#69728=CARTESIAN_POINT('',(13.2,-20.4289419162443,32.0839653438087));
#69729=CARTESIAN_POINT('',(12.6,-20.2557368354874,32.1839653438087));
#69730=CARTESIAN_POINT('',(12.6,-20.2557368354874,32.1839653438087));
#69731=CARTESIAN_POINT('',(11.9,-19.9093266739737,32.3839653438087));
#69732=CARTESIAN_POINT('',(11.9,-19.9093266739737,32.3839653438087));
#69733=CARTESIAN_POINT('',(10.9,-19.6495190528383,32.5339653438087));
#69734=CARTESIAN_POINT('',(10.9,-19.6495190528383,32.5339653438087));
#69735=CARTESIAN_POINT('',(4.5,-19.9959292143521,32.3339653438087));
#69736=CARTESIAN_POINT('',(4.5,-19.9959292143521,32.3339653438087));
#69737=CARTESIAN_POINT('',(4.5,-20.4289419162443,32.0839653438087));
#69738=CARTESIAN_POINT('',(4.5,-20.4289419162443,32.0839653438087));
#69739=CARTESIAN_POINT('',(1.9,-20.4289419162443,32.0839653438087));
#69740=CARTESIAN_POINT('',(1.9,-20.4289419162443,32.0839653438087));
#69741=CARTESIAN_POINT('',(1.57538060255632,-20.1848038826479,32.224918503225));
#69742=CARTESIAN_POINT('',(0.,-19.,32.9089653438087));
#69743=CARTESIAN_POINT('',(1.57538060255632,-17.8151961173521,33.5930121843923));
#69744=CARTESIAN_POINT('Ctrl Pts',(1.57538060255632,-20.1848038826479,32.224918503225));
#69745=CARTESIAN_POINT('Ctrl Pts',(1.62460345738085,-18.999999999973,32.9089653438243));
#69746=CARTESIAN_POINT('Ctrl Pts',(1.57538060255632,-17.8151961173521,33.5930121843923));
#69747=CARTESIAN_POINT('',(1.9,-17.5710580837557,33.7339653438087));
#69748=CARTESIAN_POINT('',(1.9,-17.5710580837557,33.7339653438087));
#69749=CARTESIAN_POINT('',(4.5,-17.5710580837557,33.7339653438087));
#69750=CARTESIAN_POINT('',(4.5,-17.5710580837557,33.7339653438087));
#69751=CARTESIAN_POINT('',(4.5,-18.0040707856479,33.4839653438087));
#69752=CARTESIAN_POINT('',(4.5,-18.0040707856479,33.4839653438087));
#69753=CARTESIAN_POINT('',(10.9,-18.3504809471617,33.2839653438087));
#69754=CARTESIAN_POINT('',(10.9,-18.3504809471617,33.2839653438087));
#69755=CARTESIAN_POINT('',(11.9,-18.0906733260263,33.4339653438087));
#69756=CARTESIAN_POINT('',(11.9,-18.0906733260263,33.4339653438087));
#69757=CARTESIAN_POINT('',(12.6,-17.7442631645126,33.6339653438087));
#69758=CARTESIAN_POINT('',(12.6,-17.7442631645126,33.6339653438087));
#69759=CARTESIAN_POINT('',(13.2,-17.5710580837557,33.7339653438087));
#69760=CARTESIAN_POINT('',(13.2,-17.5710580837557,33.7339653438087));
#69761=CARTESIAN_POINT('',(21.8,-17.5710580837557,33.7339653438087));
#69762=CARTESIAN_POINT('',(21.8,-17.5710580837557,33.7339653438087));
#69763=CARTESIAN_POINT('',(22.4,-17.7442631645126,33.6339653438087));
#69764=CARTESIAN_POINT('',(22.4,-17.7442631645126,33.6339653438087));
#69765=CARTESIAN_POINT('',(23.1,-18.0906733260263,33.4339653438087));
#69766=CARTESIAN_POINT('',(23.1,-18.0906733260263,33.4339653438087));
#69767=CARTESIAN_POINT('',(24.1,-18.3504809471617,33.2839653438087));
#69768=CARTESIAN_POINT('',(24.1,-18.3504809471617,33.2839653438087));
#69769=CARTESIAN_POINT('',(30.5,-18.0040707856479,33.4839653438087));
#69770=CARTESIAN_POINT('',(30.5,-18.0040707856479,33.4839653438087));
#69771=CARTESIAN_POINT('',(30.5,-17.5710580837557,33.7339653438087));
#69772=CARTESIAN_POINT('',(30.5,-17.5710580837557,33.7339653438087));
#69773=CARTESIAN_POINT('',(33.1,-17.5710580837557,33.7339653438087));
#69774=CARTESIAN_POINT('',(33.1,-17.5710580837557,33.7339653438087));
#69775=CARTESIAN_POINT('',(35.,-19.,32.9089653438087));
#69776=CARTESIAN_POINT('Origin',(35.,-19.,32.9089653438087));
#69777=CARTESIAN_POINT('',(35.,-22.1407037396679,36.580506751568));
#69778=CARTESIAN_POINT('',(35.,4.12832278188515,5.87152347586176));
#69779=CARTESIAN_POINT('',(34.8617922858584,-22.244646263818,36.5204955072697));
#69780=CARTESIAN_POINT('',(33.5377160618333,-23.2404504831928,35.9455676731535));
#69781=CARTESIAN_POINT('',(34.4,-22.2808358845789,35.9562839053824));
#69782=CARTESIAN_POINT('Ctrl Pts',(34.4,-22.2808358845789,35.9562839053824));
#69783=CARTESIAN_POINT('Ctrl Pts',(34.6297825291015,-22.2632399142706,36.2375102394016));
#69784=CARTESIAN_POINT('Ctrl Pts',(34.8617922858584,-22.244646263818,36.5204955072697));
#69785=CARTESIAN_POINT('',(33.3226453080309,-23.0652077022745,35.4582316768749));
#69786=CARTESIAN_POINT('Origin',(26.8550245390365,0.,0.));
#69787=CARTESIAN_POINT('',(33.0966075166785,-20.3887726991648,32.032551090536));
#69788=CARTESIAN_POINT('Origin',(17.5,-24.4259291680885,29.1096888385212));
#69789=CARTESIAN_POINT('',(33.1,-25.6899024992348,28.0490892825384));
#69790=CARTESIAN_POINT('',(33.1,-25.6899024992348,28.0490892825384));
#69791=CARTESIAN_POINT('',(30.5,-25.6899024992348,28.0490892825384));
#69792=CARTESIAN_POINT('',(30.5,-25.6899024992348,28.0490892825384));
#69793=CARTESIAN_POINT('',(30.5,-25.3068802776753,28.3704830873816));
#69794=CARTESIAN_POINT('',(30.5,-25.3068802776753,28.3704830873816));
#69795=CARTESIAN_POINT('',(24.1,-25.0004625004277,28.6275981312563));
#69796=CARTESIAN_POINT('',(24.1,-25.0004625004277,28.6275981312563));
#69797=CARTESIAN_POINT('',(23.1,-25.2302758333634,28.4347618483503));
#69798=CARTESIAN_POINT('',(23.1,-25.2302758333634,28.4347618483503));
#69799=CARTESIAN_POINT('',(22.4,-25.536693610611,28.1776468044757));
#69800=CARTESIAN_POINT('',(22.4,-25.536693610611,28.1776468044757));
#69801=CARTESIAN_POINT('',(21.8,-25.6899024992348,28.0490892825384));
#69802=CARTESIAN_POINT('',(21.8,-25.6899024992348,28.0490892825384));
#69803=CARTESIAN_POINT('',(13.2,-25.6899024992348,28.0490892825384));
#69804=CARTESIAN_POINT('',(13.2,-25.6899024992348,28.0490892825384));
#69805=CARTESIAN_POINT('',(12.6,-25.536693610611,28.1776468044757));
#69806=CARTESIAN_POINT('',(12.6,-25.536693610611,28.1776468044757));
#69807=CARTESIAN_POINT('',(11.9,-25.2302758333634,28.4347618483503));
#69808=CARTESIAN_POINT('',(11.9,-25.2302758333634,28.4347618483503));
#69809=CARTESIAN_POINT('',(10.9,-25.0004625004277,28.6275981312563));
#69810=CARTESIAN_POINT('',(10.9,-25.0004625004277,28.6275981312563));
#69811=CARTESIAN_POINT('',(4.5,-25.3068802776753,28.3704830873816));
#69812=CARTESIAN_POINT('',(4.5,-25.3068802776753,28.3704830873816));
#69813=CARTESIAN_POINT('',(4.5,-25.6899024992348,28.0490892825384));
#69814=CARTESIAN_POINT('',(4.5,-25.6899024992348,28.0490892825384));
#69815=CARTESIAN_POINT('',(1.9,-25.6899024992348,28.0490892825384));
#69816=CARTESIAN_POINT('',(1.9,-25.6899024992348,28.0490892825384));
#69817=CARTESIAN_POINT('',(1.57538060255633,-25.4739497302129,28.2302951713764));
#69818=CARTESIAN_POINT('',(0.,-24.4259291680885,29.1096888385212));
#69819=CARTESIAN_POINT('',(1.57538060255632,-23.3779086059641,29.989082505666));
#69820=CARTESIAN_POINT('Ctrl Pts',(1.57538060255633,-25.4739497302129,28.2302951713764));
#69821=CARTESIAN_POINT('Ctrl Pts',(1.62460345738085,-24.4259291680646,29.1096888385412));
#69822=CARTESIAN_POINT('Ctrl Pts',(1.57538060255632,-23.3779086059641,29.989082505666));
#69823=CARTESIAN_POINT('',(1.9,-23.1619558369422,30.170288394504));
#69824=CARTESIAN_POINT('',(1.9,-23.1619558369422,30.170288394504));
#69825=CARTESIAN_POINT('',(4.5,-23.1619558369422,30.170288394504));
#69826=CARTESIAN_POINT('',(4.5,-23.1619558369422,30.170288394504));
#69827=CARTESIAN_POINT('',(4.5,-23.5449780585017,29.8488945896607));
#69828=CARTESIAN_POINT('',(4.5,-23.5449780585017,29.8488945896607));
#69829=CARTESIAN_POINT('',(10.9,-23.8513958357493,29.5917795457861));
#69830=CARTESIAN_POINT('',(10.9,-23.8513958357493,29.5917795457861));
#69831=CARTESIAN_POINT('',(11.9,-23.6215825028136,29.784615828692));
#69832=CARTESIAN_POINT('',(11.9,-23.6215825028136,29.784615828692));
#69833=CARTESIAN_POINT('',(12.6,-23.315164725566,30.0417308725666));
#69834=CARTESIAN_POINT('',(12.6,-23.315164725566,30.0417308725666));
#69835=CARTESIAN_POINT('',(13.2,-23.1619558369422,30.170288394504));
#69836=CARTESIAN_POINT('',(13.2,-23.1619558369422,30.170288394504));
#69837=CARTESIAN_POINT('',(21.8,-23.1619558369422,30.170288394504));
#69838=CARTESIAN_POINT('',(21.8,-23.1619558369422,30.170288394504));
#69839=CARTESIAN_POINT('',(22.4,-23.315164725566,30.0417308725666));
#69840=CARTESIAN_POINT('',(22.4,-23.315164725566,30.0417308725666));
#69841=CARTESIAN_POINT('',(23.1,-23.6215825028136,29.784615828692));
#69842=CARTESIAN_POINT('',(23.1,-23.6215825028136,29.784615828692));
#69843=CARTESIAN_POINT('',(24.1,-23.8513958357493,29.5917795457861));
#69844=CARTESIAN_POINT('',(24.1,-23.8513958357493,29.5917795457861));
#69845=CARTESIAN_POINT('',(30.5,-23.5449780585017,29.8488945896607));
#69846=CARTESIAN_POINT('',(30.5,-23.5449780585017,29.8488945896607));
#69847=CARTESIAN_POINT('',(30.5,-23.1619558369422,30.170288394504));
#69848=CARTESIAN_POINT('',(30.5,-23.1619558369422,30.170288394504));
#69849=CARTESIAN_POINT('',(33.1,-23.1619558369422,30.170288394504));
#69850=CARTESIAN_POINT('',(33.1,-23.1619558369422,30.170288394504));
#69851=CARTESIAN_POINT('',(35.,-24.4259291680885,29.1096888385212));
#69852=CARTESIAN_POINT('Origin',(35.,-24.4259291680885,29.1096888385212));
#69853=CARTESIAN_POINT('',(35.,-28.156475035514,32.1800738014028));
#69854=CARTESIAN_POINT('',(35.,5.49679094461694,4.48212141338921));
#69855=CARTESIAN_POINT('',(34.8617922858584,-28.2484175959528,32.1029248328492));
#69856=CARTESIAN_POINT('',(33.5377160618333,-29.129258140991,31.3638118563816));
#69857=CARTESIAN_POINT('',(34.4,-28.1860830985703,31.5410006112756));
#69858=CARTESIAN_POINT('Ctrl Pts',(34.4,-28.1860830985703,31.5410006112756));
#69859=CARTESIAN_POINT('Ctrl Pts',(34.6297825290996,-28.2175888910031,31.8210099935449));
#69860=CARTESIAN_POINT('Ctrl Pts',(34.8617922858584,-28.2484175959528,32.1029248328492));
#69861=CARTESIAN_POINT('',(33.322645308031,-28.872052684018,30.9143101784803));
#69862=CARTESIAN_POINT('Origin',(26.8550245390365,0.,0.));
#69863=CARTESIAN_POINT('',(33.0966075166785,-25.6414155514355,28.0054314386442));
#69864=CARTESIAN_POINT('Origin',(17.5,-29.1096888385212,24.4259291680885));
#69865=CARTESIAN_POINT('',(33.1,-30.1702883945039,23.1619558369422));
#69866=CARTESIAN_POINT('',(33.1,-30.1702883945039,23.1619558369422));
#69867=CARTESIAN_POINT('',(30.5,-30.1702883945039,23.1619558369422));
#69868=CARTESIAN_POINT('',(30.5,-30.1702883945039,23.1619558369422));
#69869=CARTESIAN_POINT('',(30.5,-29.8488945896607,23.5449780585017));
#69870=CARTESIAN_POINT('',(30.5,-29.8488945896607,23.5449780585017));
#69871=CARTESIAN_POINT('',(24.1,-29.5917795457861,23.8513958357493));
#69872=CARTESIAN_POINT('',(24.1,-29.5917795457861,23.8513958357493));
#69873=CARTESIAN_POINT('',(23.1,-29.784615828692,23.6215825028136));
#69874=CARTESIAN_POINT('',(23.1,-29.784615828692,23.6215825028136));
#69875=CARTESIAN_POINT('',(22.4,-30.0417308725666,23.315164725566));
#69876=CARTESIAN_POINT('',(22.4,-30.0417308725666,23.315164725566));
#69877=CARTESIAN_POINT('',(21.8,-30.1702883945039,23.1619558369422));
#69878=CARTESIAN_POINT('',(21.8,-30.1702883945039,23.1619558369422));
#69879=CARTESIAN_POINT('',(13.2,-30.1702883945039,23.1619558369422));
#69880=CARTESIAN_POINT('',(13.2,-30.1702883945039,23.1619558369422));
#69881=CARTESIAN_POINT('',(12.6,-30.0417308725666,23.315164725566));
#69882=CARTESIAN_POINT('',(12.6,-30.0417308725666,23.315164725566));
#69883=CARTESIAN_POINT('',(11.9,-29.784615828692,23.6215825028136));
#69884=CARTESIAN_POINT('',(11.9,-29.784615828692,23.6215825028136));
#69885=CARTESIAN_POINT('',(10.9,-29.5917795457861,23.8513958357493));
#69886=CARTESIAN_POINT('',(10.9,-29.5917795457861,23.8513958357493));
#69887=CARTESIAN_POINT('',(4.5,-29.8488945896607,23.5449780585017));
#69888=CARTESIAN_POINT('',(4.5,-29.8488945896607,23.5449780585017));
#69889=CARTESIAN_POINT('',(4.5,-30.1702883945039,23.1619558369422));
#69890=CARTESIAN_POINT('',(4.5,-30.1702883945039,23.1619558369422));
#69891=CARTESIAN_POINT('',(1.9,-30.1702883945039,23.1619558369422));
#69892=CARTESIAN_POINT('',(1.9,-30.1702883945039,23.1619558369422));
#69893=CARTESIAN_POINT('',(1.57538060255632,-29.989082505666,23.3779086059641));
#69894=CARTESIAN_POINT('',(0.,-29.1096888385212,24.4259291680885));
#69895=CARTESIAN_POINT('',(1.57538060255632,-28.2302951713763,25.4739497302129));
#69896=CARTESIAN_POINT('Ctrl Pts',(1.57538060255632,-29.989082505666,23.3779086059641));
#69897=CARTESIAN_POINT('Ctrl Pts',(1.62460345738085,-29.1096888385011,24.4259291681124));
#69898=CARTESIAN_POINT('Ctrl Pts',(1.57538060255632,-28.2302951713763,25.4739497302129));
#69899=CARTESIAN_POINT('',(1.9,-28.0490892825384,25.6899024992348));
#69900=CARTESIAN_POINT('',(1.9,-28.0490892825384,25.6899024992348));
#69901=CARTESIAN_POINT('',(4.5,-28.0490892825384,25.6899024992348));
#69902=CARTESIAN_POINT('',(4.5,-28.0490892825384,25.6899024992348));
#69903=CARTESIAN_POINT('',(4.5,-28.3704830873816,25.3068802776753));
#69904=CARTESIAN_POINT('',(4.5,-28.3704830873816,25.3068802776753));
#69905=CARTESIAN_POINT('',(10.9,-28.6275981312563,25.0004625004277));
#69906=CARTESIAN_POINT('',(10.9,-28.6275981312563,25.0004625004277));
#69907=CARTESIAN_POINT('',(11.9,-28.4347618483503,25.2302758333634));
#69908=CARTESIAN_POINT('',(11.9,-28.4347618483503,25.2302758333634));
#69909=CARTESIAN_POINT('',(12.6,-28.1776468044757,25.536693610611));
#69910=CARTESIAN_POINT('',(12.6,-28.1776468044757,25.536693610611));
#69911=CARTESIAN_POINT('',(13.2,-28.0490892825384,25.6899024992348));
#69912=CARTESIAN_POINT('',(13.2,-28.0490892825384,25.6899024992348));
#69913=CARTESIAN_POINT('',(21.8,-28.0490892825384,25.6899024992348));
#69914=CARTESIAN_POINT('',(21.8,-28.0490892825384,25.6899024992348));
#69915=CARTESIAN_POINT('',(22.4,-28.1776468044757,25.536693610611));
#69916=CARTESIAN_POINT('',(22.4,-28.1776468044757,25.536693610611));
#69917=CARTESIAN_POINT('',(23.1,-28.4347618483503,25.2302758333634));
#69918=CARTESIAN_POINT('',(23.1,-28.4347618483503,25.2302758333634));
#69919=CARTESIAN_POINT('',(24.1,-28.6275981312563,25.0004625004277));
#69920=CARTESIAN_POINT('',(24.1,-28.6275981312563,25.0004625004277));
#69921=CARTESIAN_POINT('',(30.5,-28.3704830873816,25.3068802776753));
#69922=CARTESIAN_POINT('',(30.5,-28.3704830873816,25.3068802776753));
#69923=CARTESIAN_POINT('',(30.5,-28.0490892825384,25.6899024992348));
#69924=CARTESIAN_POINT('',(30.5,-28.0490892825384,25.6899024992348));
#69925=CARTESIAN_POINT('',(33.1,-28.0490892825384,25.6899024992348));
#69926=CARTESIAN_POINT('',(33.1,-28.0490892825384,25.6899024992348));
#69927=CARTESIAN_POINT('',(35.,-29.1096888385212,24.4259291680885));
#69928=CARTESIAN_POINT('Origin',(35.,-29.1096888385212,24.4259291680885));
#69929=CARTESIAN_POINT('',(35.,-33.3167260852698,26.8018655926852));
#69930=CARTESIAN_POINT('',(35.,6.86764292749649,4.10762723987466));
#69931=CARTESIAN_POINT('',(34.8617922858584,-33.3938750538235,26.7099230322464));
#69932=CARTESIAN_POINT('',(33.5377160618333,-34.132988030291,25.8290824872081));
#69933=CARTESIAN_POINT('',(34.4,-33.234910440458,26.1673599741116));
#69934=CARTESIAN_POINT('Ctrl Pts',(34.4,-33.234910440458,26.1673599741116));
#69935=CARTESIAN_POINT('Ctrl Pts',(34.6297825291036,-33.3145607080726,26.4376444612493));
#69936=CARTESIAN_POINT('Ctrl Pts',(34.8617922858584,-33.3938750538235,26.7099230322464));
#69937=CARTESIAN_POINT('',(33.322645308031,-33.8016349549212,25.4310730087083));
#69938=CARTESIAN_POINT('Origin',(26.8550245390365,0.,0.));
#69939=CARTESIAN_POINT('',(33.0966075166785,-30.1149569673582,23.1273809239214));
#69940=CARTESIAN_POINT('Origin',(17.5,-32.9089653438087,19.));
#69941=CARTESIAN_POINT('',(33.1,-33.7339653438087,17.5710580837557));
#69942=CARTESIAN_POINT('',(33.1,-33.7339653438087,17.5710580837557));
#69943=CARTESIAN_POINT('',(30.5,-33.7339653438087,17.5710580837557));
#69944=CARTESIAN_POINT('',(30.5,-33.7339653438087,17.5710580837557));
#69945=CARTESIAN_POINT('',(30.5,-33.4839653438087,18.0040707856479));
#69946=CARTESIAN_POINT('',(30.5,-33.4839653438087,18.0040707856479));
#69947=CARTESIAN_POINT('',(24.1,-33.2839653438087,18.3504809471617));
#69948=CARTESIAN_POINT('',(24.1,-33.2839653438087,18.3504809471617));
#69949=CARTESIAN_POINT('',(23.1,-33.4339653438087,18.0906733260263));
#69950=CARTESIAN_POINT('',(23.1,-33.4339653438087,18.0906733260263));
#69951=CARTESIAN_POINT('',(22.4,-33.6339653438087,17.7442631645126));
#69952=CARTESIAN_POINT('',(22.4,-33.6339653438087,17.7442631645126));
#69953=CARTESIAN_POINT('',(21.8,-33.7339653438087,17.5710580837557));
#69954=CARTESIAN_POINT('',(21.8,-33.7339653438087,17.5710580837557));
#69955=CARTESIAN_POINT('',(13.2,-33.7339653438087,17.5710580837557));
#69956=CARTESIAN_POINT('',(13.2,-33.7339653438087,17.5710580837557));
#69957=CARTESIAN_POINT('',(12.6,-33.6339653438087,17.7442631645126));
#69958=CARTESIAN_POINT('',(12.6,-33.6339653438087,17.7442631645126));
#69959=CARTESIAN_POINT('',(11.9,-33.4339653438087,18.0906733260263));
#69960=CARTESIAN_POINT('',(11.9,-33.4339653438087,18.0906733260263));
#69961=CARTESIAN_POINT('',(10.9,-33.2839653438087,18.3504809471617));
#69962=CARTESIAN_POINT('',(10.9,-33.2839653438087,18.3504809471617));
#69963=CARTESIAN_POINT('',(4.5,-33.4839653438087,18.0040707856479));
#69964=CARTESIAN_POINT('',(4.5,-33.4839653438087,18.0040707856479));
#69965=CARTESIAN_POINT('',(4.5,-33.7339653438087,17.5710580837557));
#69966=CARTESIAN_POINT('',(4.5,-33.7339653438087,17.5710580837557));
#69967=CARTESIAN_POINT('',(1.9,-33.7339653438087,17.5710580837557));
#69968=CARTESIAN_POINT('',(1.9,-33.7339653438087,17.5710580837557));
#69969=CARTESIAN_POINT('',(1.57538060255632,-33.5930121843923,17.8151961173521));
#69970=CARTESIAN_POINT('',(0.,-32.9089653438087,19.));
#69971=CARTESIAN_POINT('',(1.57538060255632,-32.224918503225,20.1848038826479));
#69972=CARTESIAN_POINT('Ctrl Pts',(1.57538060255632,-33.5930121843923,17.8151961173521));
#69973=CARTESIAN_POINT('Ctrl Pts',(1.62460345738084,-32.9089653437931,19.000000000027));
#69974=CARTESIAN_POINT('Ctrl Pts',(1.57538060255632,-32.224918503225,20.1848038826479));
#69975=CARTESIAN_POINT('',(1.9,-32.0839653438087,20.4289419162443));
#69976=CARTESIAN_POINT('',(1.9,-32.0839653438087,20.4289419162443));
#69977=CARTESIAN_POINT('',(4.5,-32.0839653438087,20.4289419162443));
#69978=CARTESIAN_POINT('',(4.5,-32.0839653438087,20.4289419162443));
#69979=CARTESIAN_POINT('',(4.5,-32.3339653438087,19.9959292143521));
#69980=CARTESIAN_POINT('',(4.5,-32.3339653438087,19.9959292143521));
#69981=CARTESIAN_POINT('',(10.9,-32.5339653438087,19.6495190528383));
#69982=CARTESIAN_POINT('',(10.9,-32.5339653438087,19.6495190528383));
#69983=CARTESIAN_POINT('',(11.9,-32.3839653438087,19.9093266739737));
#69984=CARTESIAN_POINT('',(11.9,-32.3839653438087,19.9093266739737));
#69985=CARTESIAN_POINT('',(12.6,-32.1839653438087,20.2557368354874));
#69986=CARTESIAN_POINT('',(12.6,-32.1839653438087,20.2557368354874));
#69987=CARTESIAN_POINT('',(13.2,-32.0839653438087,20.4289419162443));
#69988=CARTESIAN_POINT('',(13.2,-32.0839653438087,20.4289419162443));
#69989=CARTESIAN_POINT('',(21.8,-32.0839653438087,20.4289419162443));
#69990=CARTESIAN_POINT('',(21.8,-32.0839653438087,20.4289419162443));
#69991=CARTESIAN_POINT('',(22.4,-32.1839653438087,20.2557368354874));
#69992=CARTESIAN_POINT('',(22.4,-32.1839653438087,20.2557368354874));
#69993=CARTESIAN_POINT('',(23.1,-32.3839653438087,19.9093266739737));
#69994=CARTESIAN_POINT('',(23.1,-32.3839653438087,19.9093266739737));
#69995=CARTESIAN_POINT('',(24.1,-32.5339653438087,19.6495190528383));
#69996=CARTESIAN_POINT('',(24.1,-32.5339653438087,19.6495190528383));
#69997=CARTESIAN_POINT('',(30.5,-32.3339653438087,19.9959292143521));
#69998=CARTESIAN_POINT('',(30.5,-32.3339653438087,19.9959292143521));
#69999=CARTESIAN_POINT('',(30.5,-32.0839653438087,20.4289419162443));
#70000=CARTESIAN_POINT('',(30.5,-32.0839653438087,20.4289419162443));
#70001=CARTESIAN_POINT('',(33.1,-32.0839653438087,20.4289419162443));
#70002=CARTESIAN_POINT('',(33.1,-32.0839653438087,20.4289419162443));
#70003=CARTESIAN_POINT('',(35.,-32.9089653438087,19.));
#70004=CARTESIAN_POINT('Origin',(35.,-32.9089653438087,19.));
#70005=CARTESIAN_POINT('',(35.,-37.4646652720015,20.6092962603321));
#70006=CARTESIAN_POINT('',(35.,7.81913363821562,4.6128414041074));
#70007=CARTESIAN_POINT('',(34.8617922858584,-37.5246765162999,20.5053537361819));
#70008=CARTESIAN_POINT('',(33.5377160618333,-38.099604350416,19.5095495168072));
#70009=CARTESIAN_POINT('',(34.4,-37.2739118462885,19.9986373454573));
#70010=CARTESIAN_POINT('Ctrl Pts',(34.4,-37.2739118462884,19.9986373454573));
#70011=CARTESIAN_POINT('Ctrl Pts',(34.6297825291036,-37.399286456008,20.2509844800875));
#70012=CARTESIAN_POINT('Ctrl Pts',(34.8617922858584,-37.5246765162998,20.5053537361819));
#70013=CARTESIAN_POINT('',(33.322645308031,-37.7041716521717,19.1751255543105));
#70014=CARTESIAN_POINT('Origin',(26.8550245390365,0.,0.));
#70015=CARTESIAN_POINT('',(33.0966075166785,-33.6734706547313,17.5466166428447));
#70016=CARTESIAN_POINT('Origin',(17.5,-35.7083195898645,12.9967654463754));
#70017=CARTESIAN_POINT('',(33.1,-36.2726528263519,11.4462726220787));
#70018=CARTESIAN_POINT('',(33.1,-36.2726528263519,11.4462726220787));
#70019=CARTESIAN_POINT('',(30.5,-36.2726528263519,11.4462726220787));
#70020=CARTESIAN_POINT('',(30.5,-36.2726528263519,11.4462726220787));
#70021=CARTESIAN_POINT('',(30.5,-36.101642754689,11.9161189324716));
#70022=CARTESIAN_POINT('',(30.5,-36.101642754689,11.9161189324716));
#70023=CARTESIAN_POINT('',(24.1,-35.9648346973588,12.291995980786));
#70024=CARTESIAN_POINT('',(24.1,-35.9648346973588,12.291995980786));
#70025=CARTESIAN_POINT('',(23.1,-36.0674407403565,12.0100881945502));
#70026=CARTESIAN_POINT('',(23.1,-36.0674407403565,12.0100881945502));
#70027=CARTESIAN_POINT('',(22.4,-36.2042487976867,11.6342111462359));
#70028=CARTESIAN_POINT('',(22.4,-36.2042487976867,11.6342111462359));
#70029=CARTESIAN_POINT('',(21.8,-36.2726528263519,11.4462726220787));
#70030=CARTESIAN_POINT('',(21.8,-36.2726528263519,11.4462726220787));
#70031=CARTESIAN_POINT('',(13.2,-36.2726528263519,11.4462726220787));
#70032=CARTESIAN_POINT('',(13.2,-36.2726528263519,11.4462726220787));
#70033=CARTESIAN_POINT('',(12.6,-36.2042487976867,11.6342111462359));
#70034=CARTESIAN_POINT('',(12.6,-36.2042487976867,11.6342111462359));
#70035=CARTESIAN_POINT('',(11.9,-36.0674407403565,12.0100881945502));
#70036=CARTESIAN_POINT('',(11.9,-36.0674407403565,12.0100881945502));
#70037=CARTESIAN_POINT('',(10.9,-35.9648346973588,12.291995980786));
#70038=CARTESIAN_POINT('',(10.9,-35.9648346973588,12.291995980786));
#70039=CARTESIAN_POINT('',(4.5,-36.101642754689,11.9161189324716));
#70040=CARTESIAN_POINT('',(4.5,-36.101642754689,11.9161189324716));
#70041=CARTESIAN_POINT('',(4.5,-36.2726528263519,11.4462726220787));
#70042=CARTESIAN_POINT('',(4.5,-36.2726528263519,11.4462726220787));
#70043=CARTESIAN_POINT('',(1.9,-36.2726528263519,11.4462726220787));
#70044=CARTESIAN_POINT('',(1.9,-36.2726528263519,11.4462726220787));
#70045=CARTESIAN_POINT('',(1.57538060255632,-36.1762351867803,11.7111779096386));
#70046=CARTESIAN_POINT('',(0.,-35.7083195898645,12.9967654463754));
#70047=CARTESIAN_POINT('',(1.57538060255633,-35.2404039929487,14.2823529831122));
#70048=CARTESIAN_POINT('Ctrl Pts',(1.57538060255632,-36.1762351867803,11.7111779096386));
#70049=CARTESIAN_POINT('Ctrl Pts',(1.62460345738085,-35.7083195898539,12.9967654464047));
#70050=CARTESIAN_POINT('Ctrl Pts',(1.57538060255633,-35.2404039929487,14.2823529831122));
#70051=CARTESIAN_POINT('',(1.9,-35.1439863533772,14.5472582706722));
#70052=CARTESIAN_POINT('',(1.9,-35.1439863533772,14.5472582706722));
#70053=CARTESIAN_POINT('',(4.5,-35.1439863533772,14.5472582706722));
#70054=CARTESIAN_POINT('',(4.5,-35.1439863533772,14.5472582706722));
#70055=CARTESIAN_POINT('',(4.5,-35.31499642504,14.0774119602792));
#70056=CARTESIAN_POINT('',(4.5,-35.31499642504,14.0774119602792));
#70057=CARTESIAN_POINT('',(10.9,-35.4518044823703,13.7015349119648));
#70058=CARTESIAN_POINT('',(10.9,-35.4518044823703,13.7015349119648));
#70059=CARTESIAN_POINT('',(11.9,-35.3491984393726,13.9834426982006));
#70060=CARTESIAN_POINT('',(11.9,-35.3491984393726,13.9834426982006));
#70061=CARTESIAN_POINT('',(12.6,-35.2123903820423,14.359319746515));
#70062=CARTESIAN_POINT('',(12.6,-35.2123903820423,14.359319746515));
#70063=CARTESIAN_POINT('',(13.2,-35.1439863533772,14.5472582706722));
#70064=CARTESIAN_POINT('',(13.2,-35.1439863533772,14.5472582706722));
#70065=CARTESIAN_POINT('',(21.8,-35.1439863533772,14.5472582706722));
#70066=CARTESIAN_POINT('',(21.8,-35.1439863533772,14.5472582706722));
#70067=CARTESIAN_POINT('',(22.4,-35.2123903820423,14.359319746515));
#70068=CARTESIAN_POINT('',(22.4,-35.2123903820423,14.359319746515));
#70069=CARTESIAN_POINT('',(23.1,-35.3491984393726,13.9834426982006));
#70070=CARTESIAN_POINT('',(23.1,-35.3491984393726,13.9834426982006));
#70071=CARTESIAN_POINT('',(24.1,-35.4518044823703,13.7015349119648));
#70072=CARTESIAN_POINT('',(24.1,-35.4518044823703,13.7015349119648));
#70073=CARTESIAN_POINT('',(30.5,-35.31499642504,14.0774119602792));
#70074=CARTESIAN_POINT('',(30.5,-35.31499642504,14.0774119602792));
#70075=CARTESIAN_POINT('',(30.5,-35.1439863533772,14.5472582706722));
#70076=CARTESIAN_POINT('',(30.5,-35.1439863533772,14.5472582706722));
#70077=CARTESIAN_POINT('',(33.1,-35.1439863533772,14.5472582706722));
#70078=CARTESIAN_POINT('',(33.1,-35.1439863533772,14.5472582706722));
#70079=CARTESIAN_POINT('',(35.,-35.7083195898645,12.9967654463754));
#70080=CARTESIAN_POINT('Origin',(35.,-35.7083195898645,12.9967654463754));
#70081=CARTESIAN_POINT('',(35.,-40.4742595624789,13.790523889916));
#70082=CARTESIAN_POINT('',(35.,8.01531519808922,5.71467534565107));
#70083=CARTESIAN_POINT('',(34.8617922858584,-40.515309671231,13.6777396430533));
#70084=CARTESIAN_POINT('',(33.5377160618333,-40.9085834716837,12.5972287566465));
#70085=CARTESIAN_POINT('',(34.4,-40.1803643021789,13.22226624086));
#70086=CARTESIAN_POINT('Ctrl Pts',(34.4,-40.1803643021789,13.22226624086));
#70087=CARTESIAN_POINT('Ctrl Pts',(34.6297825291021,-40.3476538099285,13.4490085829893));
#70088=CARTESIAN_POINT('Ctrl Pts',(34.8617922858584,-40.515309671231,13.6777396430533));
#70089=CARTESIAN_POINT('',(33.322645308031,-40.4610861730024,12.3365516130268));
#70090=CARTESIAN_POINT('Origin',(26.8550245390365,0.,0.));
#70091=CARTESIAN_POINT('',(33.0966075166785,-36.2088329758587,11.4327072940915));
#70092=CARTESIAN_POINT('Origin',(17.5,-37.4226946144639,6.59863075134337));
#70093=CARTESIAN_POINT('',(33.1,-37.7092141076143,4.97369795887322));
#70094=CARTESIAN_POINT('',(33.1,-37.7092141076143,4.97369795887322));
#70095=CARTESIAN_POINT('',(30.5,-37.7092141076143,4.97369795887322));
#70096=CARTESIAN_POINT('',(30.5,-37.7092141076143,4.97369795887322));
#70097=CARTESIAN_POINT('',(30.5,-37.6223900187809,5.46610183537933));
#70098=CARTESIAN_POINT('',(30.5,-37.6223900187809,5.46610183537933));
#70099=CARTESIAN_POINT('',(24.1,-37.5529307477141,5.86002493658421));
#70100=CARTESIAN_POINT('',(24.1,-37.5529307477141,5.86002493658421));
#70101=CARTESIAN_POINT('',(23.1,-37.6050252010142,5.56458261068055));
#70102=CARTESIAN_POINT('',(23.1,-37.6050252010142,5.56458261068055));
#70103=CARTESIAN_POINT('',(22.4,-37.674484472081,5.17065950947566));
#70104=CARTESIAN_POINT('',(22.4,-37.674484472081,5.17065950947566));
#70105=CARTESIAN_POINT('',(21.8,-37.7092141076143,4.97369795887322));
#70106=CARTESIAN_POINT('',(21.8,-37.7092141076143,4.97369795887322));
#70107=CARTESIAN_POINT('',(13.2,-37.7092141076143,4.97369795887322));
#70108=CARTESIAN_POINT('',(13.2,-37.7092141076143,4.97369795887322));
#70109=CARTESIAN_POINT('',(12.6,-37.674484472081,5.17065950947566));
#70110=CARTESIAN_POINT('',(12.6,-37.674484472081,5.17065950947566));
#70111=CARTESIAN_POINT('',(11.9,-37.6050252010142,5.56458261068055));
#70112=CARTESIAN_POINT('',(11.9,-37.6050252010142,5.56458261068055));
#70113=CARTESIAN_POINT('',(10.9,-37.5529307477141,5.86002493658421));
#70114=CARTESIAN_POINT('',(10.9,-37.5529307477141,5.86002493658421));
#70115=CARTESIAN_POINT('',(4.5,-37.6223900187809,5.46610183537933));
#70116=CARTESIAN_POINT('',(4.5,-37.6223900187809,5.46610183537933));
#70117=CARTESIAN_POINT('',(4.5,-37.7092141076143,4.97369795887322));
#70118=CARTESIAN_POINT('',(4.5,-37.7092141076143,4.97369795887322));
#70119=CARTESIAN_POINT('',(1.9,-37.7092141076143,4.97369795887322));
#70120=CARTESIAN_POINT('',(1.9,-37.7092141076143,4.97369795887322));
#70121=CARTESIAN_POINT('',(1.57538060255632,-37.6602615890763,5.25132148728276));
#70122=CARTESIAN_POINT('',(0.,-37.4226946144639,6.59863075134337));
#70123=CARTESIAN_POINT('',(1.57538060255632,-37.1851276398516,7.94594001540397));
#70124=CARTESIAN_POINT('Ctrl Pts',(1.57538060255632,-37.6602615890763,5.25132148728276));
#70125=CARTESIAN_POINT('Ctrl Pts',(1.62460345738085,-37.4226946144585,6.59863075137407));
#70126=CARTESIAN_POINT('Ctrl Pts',(1.57538060255632,-37.1851276398516,7.94594001540397));
#70127=CARTESIAN_POINT('',(1.9,-37.1361751213135,8.22356354381351));
#70128=CARTESIAN_POINT('',(1.9,-37.1361751213135,8.22356354381351));
#70129=CARTESIAN_POINT('',(4.5,-37.1361751213135,8.22356354381351));
#70130=CARTESIAN_POINT('',(4.5,-37.1361751213135,8.22356354381351));
#70131=CARTESIAN_POINT('',(4.5,-37.2229992101469,7.73115966730741));
#70132=CARTESIAN_POINT('',(4.5,-37.2229992101469,7.73115966730741));
#70133=CARTESIAN_POINT('',(10.9,-37.2924584812137,7.33723656610252));
#70134=CARTESIAN_POINT('',(10.9,-37.2924584812137,7.33723656610252));
#70135=CARTESIAN_POINT('',(11.9,-37.2403640279136,7.63267889200618));
#70136=CARTESIAN_POINT('',(11.9,-37.2403640279136,7.63267889200618));
#70137=CARTESIAN_POINT('',(12.6,-37.1709047568469,8.02660199321107));
#70138=CARTESIAN_POINT('',(12.6,-37.1709047568469,8.02660199321107));
#70139=CARTESIAN_POINT('',(13.2,-37.1361751213135,8.22356354381351));
#70140=CARTESIAN_POINT('',(13.2,-37.1361751213135,8.22356354381351));
#70141=CARTESIAN_POINT('',(21.8,-37.1361751213135,8.22356354381351));
#70142=CARTESIAN_POINT('',(21.8,-37.1361751213135,8.22356354381351));
#70143=CARTESIAN_POINT('',(22.4,-37.1709047568469,8.02660199321107));
#70144=CARTESIAN_POINT('',(22.4,-37.1709047568469,8.02660199321107));
#70145=CARTESIAN_POINT('',(23.1,-37.2403640279136,7.63267889200618));
#70146=CARTESIAN_POINT('',(23.1,-37.2403640279136,7.63267889200618));
#70147=CARTESIAN_POINT('',(24.1,-37.2924584812137,7.33723656610252));
#70148=CARTESIAN_POINT('',(24.1,-37.2924584812137,7.33723656610252));
#70149=CARTESIAN_POINT('',(30.5,-37.2229992101469,7.73115966730741));
#70150=CARTESIAN_POINT('',(30.5,-37.2229992101469,7.73115966730741));
#70151=CARTESIAN_POINT('',(30.5,-37.1361751213135,8.22356354381351));
#70152=CARTESIAN_POINT('',(30.5,-37.1361751213135,8.22356354381351));
#70153=CARTESIAN_POINT('',(33.1,-37.1361751213135,8.22356354381351));
#70154=CARTESIAN_POINT('',(33.1,-37.1361751213135,8.22356354381351));
#70155=CARTESIAN_POINT('',(35.,-37.4226946144639,6.59863075134337));
#70156=CARTESIAN_POINT('Origin',(35.,-37.4226946144639,6.59863075134337));
#70157=CARTESIAN_POINT('',(35.,-42.2540639571139,6.55273342944654));
#70158=CARTESIAN_POINT('',(35.,7.25327777991845,7.02304613766821));
#70159=CARTESIAN_POINT('',(34.8617922858584,-42.2749056435377,6.43453435214071));
#70160=CARTESIAN_POINT('',(33.5377160618333,-42.4745759849063,5.30214757522048));
#70161=CARTESIAN_POINT('',(34.4,-41.8659567209931,6.04414326732377));
#70162=CARTESIAN_POINT('Ctrl Pts',(34.4,-41.8659567209931,6.04414326732377));
#70163=CARTESIAN_POINT('Ctrl Pts',(34.6297825291009,-42.0700781197321,6.23839136562435));
#70164=CARTESIAN_POINT('Ctrl Pts',(34.8617922858584,-42.2749056435377,6.43453435214071));
#70165=CARTESIAN_POINT('',(33.3226453080309,-41.9886110647639,5.12313779357753));
#70166=CARTESIAN_POINT('Origin',(26.8550245390365,0.,0.));
#70167=CARTESIAN_POINT('',(33.0966075166785,-37.6440082295681,4.97142091943646));
#70168=CARTESIAN_POINT('Origin',(17.5,-38.,4.65365783675994E-15));
#70169=CARTESIAN_POINT('',(33.1,-38.,-1.65));
#70170=CARTESIAN_POINT('',(33.1,-38.,-1.65));
#70171=CARTESIAN_POINT('',(30.5,-38.,-1.65));
#70172=CARTESIAN_POINT('',(30.5,-38.,-1.65));
#70173=CARTESIAN_POINT('',(30.5,-38.,-1.15));
#70174=CARTESIAN_POINT('',(30.5,-38.,-1.15));
#70175=CARTESIAN_POINT('',(24.1,-38.,-0.749999999999995));
#70176=CARTESIAN_POINT('',(24.1,-38.,-0.749999999999995));
#70177=CARTESIAN_POINT('',(23.1,-38.,-1.05));
#70178=CARTESIAN_POINT('',(23.1,-38.,-1.05));
#70179=CARTESIAN_POINT('',(22.4,-38.,-1.45));
#70180=CARTESIAN_POINT('',(22.4,-38.,-1.45));
#70181=CARTESIAN_POINT('',(21.8,-38.,-1.65));
#70182=CARTESIAN_POINT('',(21.8,-38.,-1.65));
#70183=CARTESIAN_POINT('',(13.2,-38.,-1.65));
#70184=CARTESIAN_POINT('',(13.2,-38.,-1.65));
#70185=CARTESIAN_POINT('',(12.6,-38.,-1.45));
#70186=CARTESIAN_POINT('',(12.6,-38.,-1.45));
#70187=CARTESIAN_POINT('',(11.9,-38.,-1.05));
#70188=CARTESIAN_POINT('',(11.9,-38.,-1.05));
#70189=CARTESIAN_POINT('',(10.9,-38.,-0.749999999999995));
#70190=CARTESIAN_POINT('',(10.9,-38.,-0.749999999999995));
#70191=CARTESIAN_POINT('',(4.5,-38.,-1.15));
#70192=CARTESIAN_POINT('',(4.5,-38.,-1.15));
#70193=CARTESIAN_POINT('',(4.5,-38.,-1.65));
#70194=CARTESIAN_POINT('',(4.5,-38.,-1.65));
#70195=CARTESIAN_POINT('',(1.9,-38.,-1.65));
#70196=CARTESIAN_POINT('',(1.9,-38.,-1.65));
#70197=CARTESIAN_POINT('',(1.57538060255632,-38.,-1.36809368116733));
#70198=CARTESIAN_POINT('',(0.,-38.,4.65365783675994E-15));
#70199=CARTESIAN_POINT('',(1.57538060255633,-38.,1.36809368116734));
#70200=CARTESIAN_POINT('Ctrl Pts',(1.57538060255632,-38.,-1.36809368116733));
#70201=CARTESIAN_POINT('Ctrl Pts',(1.62460345738085,-38.,3.11853320944522E-11));
#70202=CARTESIAN_POINT('Ctrl Pts',(1.57538060255633,-38.,1.36809368116734));
#70203=CARTESIAN_POINT('',(1.9,-38.,1.65));
#70204=CARTESIAN_POINT('',(1.9,-38.,1.65));
#70205=CARTESIAN_POINT('',(4.5,-38.,1.65));
#70206=CARTESIAN_POINT('',(4.5,-38.,1.65));
#70207=CARTESIAN_POINT('',(4.5,-38.,1.15));
#70208=CARTESIAN_POINT('',(4.5,-38.,1.15));
#70209=CARTESIAN_POINT('',(10.9,-38.,0.750000000000005));
#70210=CARTESIAN_POINT('',(10.9,-38.,0.750000000000005));
#70211=CARTESIAN_POINT('',(11.9,-38.,1.05));
#70212=CARTESIAN_POINT('',(11.9,-38.,1.05));
#70213=CARTESIAN_POINT('',(12.6,-38.,1.45));
#70214=CARTESIAN_POINT('',(12.6,-38.,1.45));
#70215=CARTESIAN_POINT('',(13.2,-38.,1.65));
#70216=CARTESIAN_POINT('',(13.2,-38.,1.65));
#70217=CARTESIAN_POINT('',(21.8,-38.,1.65));
#70218=CARTESIAN_POINT('',(21.8,-38.,1.65));
#70219=CARTESIAN_POINT('',(22.4,-38.,1.45));
#70220=CARTESIAN_POINT('',(22.4,-38.,1.45));
#70221=CARTESIAN_POINT('',(23.1,-38.,1.05));
#70222=CARTESIAN_POINT('',(23.1,-38.,1.05));
#70223=CARTESIAN_POINT('',(24.1,-38.,0.750000000000005));
#70224=CARTESIAN_POINT('',(24.1,-38.,0.750000000000005));
#70225=CARTESIAN_POINT('',(30.5,-38.,1.15));
#70226=CARTESIAN_POINT('',(30.5,-38.,1.15));
#70227=CARTESIAN_POINT('',(30.5,-38.,1.65));
#70228=CARTESIAN_POINT('',(30.5,-38.,1.65));
#70229=CARTESIAN_POINT('',(33.1,-38.,1.65));
#70230=CARTESIAN_POINT('',(33.1,-38.,1.65));
#70231=CARTESIAN_POINT('',(35.,-38.,4.65365783675994E-15));
#70232=CARTESIAN_POINT('Origin',(35.,-38.,4.65365783675994E-15));
#70233=CARTESIAN_POINT('',(35.,-42.75,-0.884158520433531));
#70234=CARTESIAN_POINT('',(35.,5.49306987041266,8.09574069594452));
#70235=CARTESIAN_POINT('',(34.8617922858584,-42.75,-1.0041810090302));
#70236=CARTESIAN_POINT('',(33.5377160618333,-42.75,-2.15403667726254));
#70237=CARTESIAN_POINT('',(34.4,-42.2794732300362,-1.31762794090604));
#70238=CARTESIAN_POINT('Ctrl Pts',(34.4,-42.2794732300361,-1.31762794090604));
#70239=CARTESIAN_POINT('Ctrl Pts',(34.6297825290972,-42.5142243943514,-1.16177621660812));
#70240=CARTESIAN_POINT('Ctrl Pts',(34.8617922858584,-42.75,-1.0041810090302));
#70241=CARTESIAN_POINT('',(33.3226453080309,-42.240333256585,-2.24593997529677));
#70242=CARTESIAN_POINT('Origin',(26.8550245390365,0.,0.));
#70243=CARTESIAN_POINT('',(33.0966075166785,-37.9353893420094,-1.64091956419533));
#70244=CARTESIAN_POINT('Origin',(17.5,-37.4226946144639,-6.59863075134334));
#70245=CARTESIAN_POINT('',(33.1,-37.1361751213135,-8.22356354381348));
#70246=CARTESIAN_POINT('',(33.1,-37.1361751213135,-8.22356354381348));
#70247=CARTESIAN_POINT('',(30.5,-37.1361751213135,-8.22356354381348));
#70248=CARTESIAN_POINT('',(30.5,-37.1361751213135,-8.22356354381348));
#70249=CARTESIAN_POINT('',(30.5,-37.2229992101469,-7.73115966730738));
#70250=CARTESIAN_POINT('',(30.5,-37.2229992101469,-7.73115966730738));
#70251=CARTESIAN_POINT('',(24.1,-37.2924584812137,-7.3372365661025));
#70252=CARTESIAN_POINT('',(24.1,-37.2924584812137,-7.3372365661025));
#70253=CARTESIAN_POINT('',(23.1,-37.2403640279136,-7.63267889200616));
#70254=CARTESIAN_POINT('',(23.1,-37.2403640279136,-7.63267889200616));
#70255=CARTESIAN_POINT('',(22.4,-37.1709047568469,-8.02660199321104));
#70256=CARTESIAN_POINT('',(22.4,-37.1709047568469,-8.02660199321104));
#70257=CARTESIAN_POINT('',(21.8,-37.1361751213135,-8.22356354381348));
#70258=CARTESIAN_POINT('',(21.8,-37.1361751213135,-8.22356354381348));
#70259=CARTESIAN_POINT('',(13.2,-37.1361751213135,-8.22356354381348));
#70260=CARTESIAN_POINT('',(13.2,-37.1361751213135,-8.22356354381348));
#70261=CARTESIAN_POINT('',(12.6,-37.1709047568469,-8.02660199321104));
#70262=CARTESIAN_POINT('',(12.6,-37.1709047568469,-8.02660199321104));
#70263=CARTESIAN_POINT('',(11.9,-37.2403640279136,-7.63267889200616));
#70264=CARTESIAN_POINT('',(11.9,-37.2403640279136,-7.63267889200616));
#70265=CARTESIAN_POINT('',(10.9,-37.2924584812137,-7.3372365661025));
#70266=CARTESIAN_POINT('',(10.9,-37.2924584812137,-7.3372365661025));
#70267=CARTESIAN_POINT('',(4.5,-37.2229992101469,-7.73115966730738));
#70268=CARTESIAN_POINT('',(4.5,-37.2229992101469,-7.73115966730738));
#70269=CARTESIAN_POINT('',(4.5,-37.1361751213135,-8.22356354381348));
#70270=CARTESIAN_POINT('',(4.5,-37.1361751213135,-8.22356354381348));
#70271=CARTESIAN_POINT('',(1.9,-37.1361751213135,-8.22356354381348));
#70272=CARTESIAN_POINT('',(1.9,-37.1361751213135,-8.22356354381348));
#70273=CARTESIAN_POINT('',(1.57538060255632,-37.1851276398516,-7.94594001540395));
#70274=CARTESIAN_POINT('',(0.,-37.4226946144639,-6.59863075134334));
#70275=CARTESIAN_POINT('',(1.57538060255633,-37.6602615890763,-5.25132148728274));
#70276=CARTESIAN_POINT('Ctrl Pts',(1.57538060255632,-37.1851276398516,-7.94594001540395));
#70277=CARTESIAN_POINT('Ctrl Pts',(1.62460345738085,-37.4226946144693,-6.59863075131264));
#70278=CARTESIAN_POINT('Ctrl Pts',(1.57538060255633,-37.6602615890763,-5.25132148728274));
#70279=CARTESIAN_POINT('',(1.9,-37.7092141076143,-4.9736979588732));
#70280=CARTESIAN_POINT('',(1.9,-37.7092141076143,-4.9736979588732));
#70281=CARTESIAN_POINT('',(4.5,-37.7092141076143,-4.9736979588732));
#70282=CARTESIAN_POINT('',(4.5,-37.7092141076143,-4.9736979588732));
#70283=CARTESIAN_POINT('',(4.5,-37.6223900187809,-5.4661018353793));
#70284=CARTESIAN_POINT('',(4.5,-37.6223900187809,-5.4661018353793));
#70285=CARTESIAN_POINT('',(10.9,-37.5529307477141,-5.86002493658419));
#70286=CARTESIAN_POINT('',(10.9,-37.5529307477141,-5.86002493658419));
#70287=CARTESIAN_POINT('',(11.9,-37.6050252010142,-5.56458261068052));
#70288=CARTESIAN_POINT('',(11.9,-37.6050252010142,-5.56458261068052));
#70289=CARTESIAN_POINT('',(12.6,-37.674484472081,-5.17065950947564));
#70290=CARTESIAN_POINT('',(12.6,-37.674484472081,-5.17065950947564));
#70291=CARTESIAN_POINT('',(13.2,-37.7092141076143,-4.9736979588732));
#70292=CARTESIAN_POINT('',(13.2,-37.7092141076143,-4.9736979588732));
#70293=CARTESIAN_POINT('',(21.8,-37.7092141076143,-4.9736979588732));
#70294=CARTESIAN_POINT('',(21.8,-37.7092141076143,-4.9736979588732));
#70295=CARTESIAN_POINT('',(22.4,-37.674484472081,-5.17065950947564));
#70296=CARTESIAN_POINT('',(22.4,-37.674484472081,-5.17065950947564));
#70297=CARTESIAN_POINT('',(23.1,-37.6050252010142,-5.56458261068052));
#70298=CARTESIAN_POINT('',(23.1,-37.6050252010142,-5.56458261068052));
#70299=CARTESIAN_POINT('',(24.1,-37.5529307477141,-5.86002493658419));
#70300=CARTESIAN_POINT('',(24.1,-37.5529307477141,-5.86002493658419));
#70301=CARTESIAN_POINT('',(30.5,-37.6223900187809,-5.4661018353793));
#70302=CARTESIAN_POINT('',(30.5,-37.6223900187809,-5.4661018353793));
#70303=CARTESIAN_POINT('',(30.5,-37.7092141076143,-4.9736979588732));
#70304=CARTESIAN_POINT('',(30.5,-37.7092141076143,-4.9736979588732));
#70305=CARTESIAN_POINT('',(33.1,-37.7092141076143,-4.9736979588732));
#70306=CARTESIAN_POINT('',(33.1,-37.7092141076143,-4.9736979588732));
#70307=CARTESIAN_POINT('',(35.,-37.4226946144639,-6.59863075134334));
#70308=CARTESIAN_POINT('Origin',(35.,-37.4226946144639,-6.59863075134334));
#70309=CARTESIAN_POINT('',(35.,-41.9469989254299,-8.29418576107601));
#70310=CARTESIAN_POINT('',(35.,2.8665236475809,8.50039468265471));
#70311=CARTESIAN_POINT('',(34.8617922858584,-41.9261572390061,-8.41238483838183));
#70312=CARTESIAN_POINT('',(33.5377160618333,-41.7264868976375,-9.54477161530207));
#70313=CARTESIAN_POINT('',(34.4,-41.4083493394303,-8.63936369090331));
#70314=CARTESIAN_POINT('Ctrl Pts',(34.4,-41.4083493394303,-8.63936369090331));
#70315=CARTESIAN_POINT('Ctrl Pts',(34.6297825290979,-41.666597473988,-8.52664381638261));
#70316=CARTESIAN_POINT('Ctrl Pts',(34.8617922858584,-41.9261572390061,-8.41238483838183));
#70317=CARTESIAN_POINT('',(33.322645308031,-41.2086042970448,-9.54677599452212));
#70318=CARTESIAN_POINT('Origin',(26.8550245390365,0.,0.));
#70319=CARTESIAN_POINT('',(33.0966075166785,-37.0741228455271,-8.2034015372144));
#70320=CARTESIAN_POINT('Origin',(17.5,-35.7083195898645,-12.9967654463754));
#70321=CARTESIAN_POINT('',(33.1,-35.1439863533772,-14.5472582706722));
#70322=CARTESIAN_POINT('',(33.1,-35.1439863533772,-14.5472582706722));
#70323=CARTESIAN_POINT('',(30.5,-35.1439863533772,-14.5472582706722));
#70324=CARTESIAN_POINT('',(30.5,-35.1439863533772,-14.5472582706722));
#70325=CARTESIAN_POINT('',(30.5,-35.31499642504,-14.0774119602792));
#70326=CARTESIAN_POINT('',(30.5,-35.31499642504,-14.0774119602792));
#70327=CARTESIAN_POINT('',(24.1,-35.4518044823703,-13.7015349119648));
#70328=CARTESIAN_POINT('',(24.1,-35.4518044823703,-13.7015349119648));
#70329=CARTESIAN_POINT('',(23.1,-35.3491984393726,-13.9834426982006));
#70330=CARTESIAN_POINT('',(23.1,-35.3491984393726,-13.9834426982006));
#70331=CARTESIAN_POINT('',(22.4,-35.2123903820423,-14.359319746515));
#70332=CARTESIAN_POINT('',(22.4,-35.2123903820423,-14.359319746515));
#70333=CARTESIAN_POINT('',(21.8,-35.1439863533772,-14.5472582706722));
#70334=CARTESIAN_POINT('',(21.8,-35.1439863533772,-14.5472582706722));
#70335=CARTESIAN_POINT('',(13.2,-35.1439863533772,-14.5472582706722));
#70336=CARTESIAN_POINT('',(13.2,-35.1439863533772,-14.5472582706722));
#70337=CARTESIAN_POINT('',(12.6,-35.2123903820423,-14.359319746515));
#70338=CARTESIAN_POINT('',(12.6,-35.2123903820423,-14.359319746515));
#70339=CARTESIAN_POINT('',(11.9,-35.3491984393726,-13.9834426982006));
#70340=CARTESIAN_POINT('',(11.9,-35.3491984393726,-13.9834426982006));
#70341=CARTESIAN_POINT('',(10.9,-35.4518044823703,-13.7015349119648));
#70342=CARTESIAN_POINT('',(10.9,-35.4518044823703,-13.7015349119648));
#70343=CARTESIAN_POINT('',(4.5,-35.31499642504,-14.0774119602792));
#70344=CARTESIAN_POINT('',(4.5,-35.31499642504,-14.0774119602792));
#70345=CARTESIAN_POINT('',(4.5,-35.1439863533772,-14.5472582706722));
#70346=CARTESIAN_POINT('',(4.5,-35.1439863533772,-14.5472582706722));
#70347=CARTESIAN_POINT('',(1.9,-35.1439863533772,-14.5472582706722));
#70348=CARTESIAN_POINT('',(1.9,-35.1439863533772,-14.5472582706722));
#70349=CARTESIAN_POINT('',(1.57538060255633,-35.2404039929487,-14.2823529831122));
#70350=CARTESIAN_POINT('',(0.,-35.7083195898645,-12.9967654463754));
#70351=CARTESIAN_POINT('',(1.57538060255633,-36.1762351867803,-11.7111779096386));
#70352=CARTESIAN_POINT('Ctrl Pts',(1.57538060255633,-35.2404039929487,-14.2823529831122));
#70353=CARTESIAN_POINT('Ctrl Pts',(1.62460345738085,-35.7083195898752,-12.9967654463461));
#70354=CARTESIAN_POINT('Ctrl Pts',(1.57538060255633,-36.1762351867803,-11.7111779096386));
#70355=CARTESIAN_POINT('',(1.9,-36.2726528263519,-11.4462726220787));
#70356=CARTESIAN_POINT('',(1.9,-36.2726528263519,-11.4462726220787));
#70357=CARTESIAN_POINT('',(4.5,-36.2726528263519,-11.4462726220787));
#70358=CARTESIAN_POINT('',(4.5,-36.2726528263519,-11.4462726220787));
#70359=CARTESIAN_POINT('',(4.5,-36.101642754689,-11.9161189324716));
#70360=CARTESIAN_POINT('',(4.5,-36.101642754689,-11.9161189324716));
#70361=CARTESIAN_POINT('',(10.9,-35.9648346973588,-12.291995980786));
#70362=CARTESIAN_POINT('',(10.9,-35.9648346973588,-12.291995980786));
#70363=CARTESIAN_POINT('',(11.9,-36.0674407403565,-12.0100881945502));
#70364=CARTESIAN_POINT('',(11.9,-36.0674407403565,-12.0100881945502));
#70365=CARTESIAN_POINT('',(12.6,-36.2042487976867,-11.6342111462358));
#70366=CARTESIAN_POINT('',(12.6,-36.2042487976867,-11.6342111462358));
#70367=CARTESIAN_POINT('',(13.2,-36.2726528263519,-11.4462726220787));
#70368=CARTESIAN_POINT('',(13.2,-36.2726528263519,-11.4462726220787));
#70369=CARTESIAN_POINT('',(21.8,-36.2726528263519,-11.4462726220787));
#70370=CARTESIAN_POINT('',(21.8,-36.2726528263519,-11.4462726220787));
#70371=CARTESIAN_POINT('',(22.4,-36.2042487976867,-11.6342111462358));
#70372=CARTESIAN_POINT('',(22.4,-36.2042487976867,-11.6342111462358));
#70373=CARTESIAN_POINT('',(23.1,-36.0674407403565,-12.0100881945502));
#70374=CARTESIAN_POINT('',(23.1,-36.0674407403565,-12.0100881945502));
#70375=CARTESIAN_POINT('',(24.1,-35.9648346973588,-12.291995980786));
#70376=CARTESIAN_POINT('',(24.1,-35.9648346973588,-12.291995980786));
#70377=CARTESIAN_POINT('',(30.5,-36.101642754689,-11.9161189324716));
#70378=CARTESIAN_POINT('',(30.5,-36.101642754689,-11.9161189324716));
#70379=CARTESIAN_POINT('',(30.5,-36.2726528263519,-11.4462726220787));
#70380=CARTESIAN_POINT('',(30.5,-36.2726528263519,-11.4462726220787));
#70381=CARTESIAN_POINT('',(33.1,-36.2726528263519,-11.4462726220787));
#70382=CARTESIAN_POINT('',(33.1,-36.2726528263519,-11.4462726220787));
#70383=CARTESIAN_POINT('',(35.,-35.7083195898645,-12.9967654463754));
#70384=CARTESIAN_POINT('Origin',(35.,-35.7083195898645,-12.9967654463754));
#70385=CARTESIAN_POINT('',(35.,-39.8694595147163,-15.4521983644287));
#70386=CARTESIAN_POINT('',(35.,-0.336200737254209,7.87584796738456));
#70387=CARTESIAN_POINT('',(34.8617922858584,-39.8284094059642,-15.5649826112914));
#70388=CARTESIAN_POINT('',(33.5377160618333,-39.4351356055115,-16.6454934976981));
#70389=CARTESIAN_POINT('',(34.4,-39.2790537077817,-15.6985967468815));
#70390=CARTESIAN_POINT('Ctrl Pts',(34.4,-39.2790537077817,-15.6985967468815));
#70391=CARTESIAN_POINT('Ctrl Pts',(34.6297825291028,-39.5529520736982,-15.6324336584854));
#70392=CARTESIAN_POINT('Ctrl Pts',(34.8617922858584,-39.8284094059642,-15.5649826112914));
#70393=CARTESIAN_POINT('',(33.3226453080309,-38.9247727484987,-16.5575380560557));
#70394=CARTESIAN_POINT('Origin',(26.8550245390365,0.,0.));
#70395=CARTESIAN_POINT('',(33.0966075166785,-35.0863778867947,-14.5166273056467));
#70396=CARTESIAN_POINT('Origin',(17.5,-32.9089653438087,-19.));
#70397=CARTESIAN_POINT('',(33.1,-32.0839653438087,-20.4289419162443));
#70398=CARTESIAN_POINT('',(33.1,-32.0839653438087,-20.4289419162443));
#70399=CARTESIAN_POINT('',(30.5,-32.0839653438087,-20.4289419162443));
#70400=CARTESIAN_POINT('',(30.5,-32.0839653438087,-20.4289419162443));
#70401=CARTESIAN_POINT('',(30.5,-32.3339653438087,-19.9959292143521));
#70402=CARTESIAN_POINT('',(30.5,-32.3339653438087,-19.9959292143521));
#70403=CARTESIAN_POINT('',(24.1,-32.5339653438087,-19.6495190528383));
#70404=CARTESIAN_POINT('',(24.1,-32.5339653438087,-19.6495190528383));
#70405=CARTESIAN_POINT('',(23.1,-32.3839653438087,-19.9093266739736));
#70406=CARTESIAN_POINT('',(23.1,-32.3839653438087,-19.9093266739736));
#70407=CARTESIAN_POINT('',(22.4,-32.1839653438087,-20.2557368354874));
#70408=CARTESIAN_POINT('',(22.4,-32.1839653438087,-20.2557368354874));
#70409=CARTESIAN_POINT('',(21.8,-32.0839653438087,-20.4289419162443));
#70410=CARTESIAN_POINT('',(21.8,-32.0839653438087,-20.4289419162443));
#70411=CARTESIAN_POINT('',(13.2,-32.0839653438087,-20.4289419162443));
#70412=CARTESIAN_POINT('',(13.2,-32.0839653438087,-20.4289419162443));
#70413=CARTESIAN_POINT('',(12.6,-32.1839653438087,-20.2557368354874));
#70414=CARTESIAN_POINT('',(12.6,-32.1839653438087,-20.2557368354874));
#70415=CARTESIAN_POINT('',(11.9,-32.3839653438087,-19.9093266739736));
#70416=CARTESIAN_POINT('',(11.9,-32.3839653438087,-19.9093266739736));
#70417=CARTESIAN_POINT('',(10.9,-32.5339653438087,-19.6495190528383));
#70418=CARTESIAN_POINT('',(10.9,-32.5339653438087,-19.6495190528383));
#70419=CARTESIAN_POINT('',(4.5,-32.3339653438087,-19.9959292143521));
#70420=CARTESIAN_POINT('',(4.5,-32.3339653438087,-19.9959292143521));
#70421=CARTESIAN_POINT('',(4.5,-32.0839653438087,-20.4289419162443));
#70422=CARTESIAN_POINT('',(4.5,-32.0839653438087,-20.4289419162443));
#70423=CARTESIAN_POINT('',(1.9,-32.0839653438087,-20.4289419162443));
#70424=CARTESIAN_POINT('',(1.9,-32.0839653438087,-20.4289419162443));
#70425=CARTESIAN_POINT('',(1.57538060255633,-32.224918503225,-20.1848038826479));
#70426=CARTESIAN_POINT('',(0.,-32.9089653438087,-19.));
#70427=CARTESIAN_POINT('',(1.57538060255633,-33.5930121843923,-17.8151961173521));
#70428=CARTESIAN_POINT('Ctrl Pts',(1.57538060255633,-32.224918503225,-20.1848038826479));
#70429=CARTESIAN_POINT('Ctrl Pts',(1.62460345738085,-32.9089653438243,-18.999999999973));
#70430=CARTESIAN_POINT('Ctrl Pts',(1.57538060255633,-33.5930121843923,-17.8151961173521));
#70431=CARTESIAN_POINT('',(1.9,-33.7339653438087,-17.5710580837557));
#70432=CARTESIAN_POINT('',(1.9,-33.7339653438087,-17.5710580837557));
#70433=CARTESIAN_POINT('',(4.5,-33.7339653438087,-17.5710580837557));
#70434=CARTESIAN_POINT('',(4.5,-33.7339653438087,-17.5710580837557));
#70435=CARTESIAN_POINT('',(4.5,-33.4839653438087,-18.0040707856479));
#70436=CARTESIAN_POINT('',(4.5,-33.4839653438087,-18.0040707856479));
#70437=CARTESIAN_POINT('',(10.9,-33.2839653438087,-18.3504809471617));
#70438=CARTESIAN_POINT('',(10.9,-33.2839653438087,-18.3504809471617));
#70439=CARTESIAN_POINT('',(11.9,-33.4339653438087,-18.0906733260263));
#70440=CARTESIAN_POINT('',(11.9,-33.4339653438087,-18.0906733260263));
#70441=CARTESIAN_POINT('',(12.6,-33.6339653438087,-17.7442631645126));
#70442=CARTESIAN_POINT('',(12.6,-33.6339653438087,-17.7442631645126));
#70443=CARTESIAN_POINT('',(13.2,-33.7339653438087,-17.5710580837557));
#70444=CARTESIAN_POINT('',(13.2,-33.7339653438087,-17.5710580837557));
#70445=CARTESIAN_POINT('',(21.8,-33.7339653438087,-17.5710580837557));
#70446=CARTESIAN_POINT('',(21.8,-33.7339653438087,-17.5710580837557));
#70447=CARTESIAN_POINT('',(22.4,-33.6339653438087,-17.7442631645126));
#70448=CARTESIAN_POINT('',(22.4,-33.6339653438087,-17.7442631645126));
#70449=CARTESIAN_POINT('',(23.1,-33.4339653438087,-18.0906733260263));
#70450=CARTESIAN_POINT('',(23.1,-33.4339653438087,-18.0906733260263));
#70451=CARTESIAN_POINT('',(24.1,-33.2839653438087,-18.3504809471617));
#70452=CARTESIAN_POINT('',(24.1,-33.2839653438087,-18.3504809471617));
#70453=CARTESIAN_POINT('',(30.5,-33.4839653438087,-18.0040707856479));
#70454=CARTESIAN_POINT('',(30.5,-33.4839653438087,-18.0040707856479));
#70455=CARTESIAN_POINT('',(30.5,-33.7339653438087,-17.5710580837557));
#70456=CARTESIAN_POINT('',(30.5,-33.7339653438087,-17.5710580837557));
#70457=CARTESIAN_POINT('',(33.1,-33.7339653438087,-17.5710580837557));
#70458=CARTESIAN_POINT('',(33.1,-33.7339653438087,-17.5710580837557));
#70459=CARTESIAN_POINT('',(35.,-32.9089653438087,-19.));
#70460=CARTESIAN_POINT('Origin',(35.,-32.9089653438087,-19.));
#70461=CARTESIAN_POINT('',(35.,-36.580506751568,-22.1407037396679));
#70462=CARTESIAN_POINT('',(35.,-3.70080331045544,5.98519655344499));
#70463=CARTESIAN_POINT('',(34.8617922858584,-36.5204955072697,-22.244646263818));
#70464=CARTESIAN_POINT('',(33.5377160618333,-35.9455676731535,-23.2404504831928));
#70465=CARTESIAN_POINT('',(34.4,-35.9562839053824,-22.2808358845789));
#70466=CARTESIAN_POINT('Ctrl Pts',(34.4,-35.9562839053824,-22.2808358845789));
#70467=CARTESIAN_POINT('Ctrl Pts',(34.6297825291,-36.2375102393997,-22.2632399142707));
#70468=CARTESIAN_POINT('Ctrl Pts',(34.8617922858584,-36.5204955072696,-22.244646263818));
#70469=CARTESIAN_POINT('',(33.322645308031,-35.4582316768749,-23.0652077022745));
#70470=CARTESIAN_POINT('Origin',(26.8550245390365,0.,0.));
#70471=CARTESIAN_POINT('',(33.0966075166785,-32.032551090536,-20.3887726991648));
#70472=CARTESIAN_POINT('Origin',(17.5,-29.1096888385212,-24.4259291680885));
#70473=CARTESIAN_POINT('',(33.1,-28.0490892825384,-25.6899024992348));
#70474=CARTESIAN_POINT('',(33.1,-28.0490892825384,-25.6899024992348));
#70475=CARTESIAN_POINT('',(30.5,-28.0490892825384,-25.6899024992348));
#70476=CARTESIAN_POINT('',(30.5,-28.0490892825384,-25.6899024992348));
#70477=CARTESIAN_POINT('',(30.5,-28.3704830873816,-25.3068802776753));
#70478=CARTESIAN_POINT('',(30.5,-28.3704830873816,-25.3068802776753));
#70479=CARTESIAN_POINT('',(24.1,-28.6275981312563,-25.0004625004277));
#70480=CARTESIAN_POINT('',(24.1,-28.6275981312563,-25.0004625004277));
#70481=CARTESIAN_POINT('',(23.1,-28.4347618483503,-25.2302758333634));
#70482=CARTESIAN_POINT('',(23.1,-28.4347618483503,-25.2302758333634));
#70483=CARTESIAN_POINT('',(22.4,-28.1776468044757,-25.536693610611));
#70484=CARTESIAN_POINT('',(22.4,-28.1776468044757,-25.536693610611));
#70485=CARTESIAN_POINT('',(21.8,-28.0490892825384,-25.6899024992348));
#70486=CARTESIAN_POINT('',(21.8,-28.0490892825384,-25.6899024992348));
#70487=CARTESIAN_POINT('',(13.2,-28.0490892825384,-25.6899024992348));
#70488=CARTESIAN_POINT('',(13.2,-28.0490892825384,-25.6899024992348));
#70489=CARTESIAN_POINT('',(12.6,-28.1776468044757,-25.536693610611));
#70490=CARTESIAN_POINT('',(12.6,-28.1776468044757,-25.536693610611));
#70491=CARTESIAN_POINT('',(11.9,-28.4347618483503,-25.2302758333634));
#70492=CARTESIAN_POINT('',(11.9,-28.4347618483503,-25.2302758333634));
#70493=CARTESIAN_POINT('',(10.9,-28.6275981312563,-25.0004625004277));
#70494=CARTESIAN_POINT('',(10.9,-28.6275981312563,-25.0004625004277));
#70495=CARTESIAN_POINT('',(4.5,-28.3704830873816,-25.3068802776753));
#70496=CARTESIAN_POINT('',(4.5,-28.3704830873816,-25.3068802776753));
#70497=CARTESIAN_POINT('',(4.5,-28.0490892825384,-25.6899024992348));
#70498=CARTESIAN_POINT('',(4.5,-28.0490892825384,-25.6899024992348));
#70499=CARTESIAN_POINT('',(1.9,-28.0490892825384,-25.6899024992348));
#70500=CARTESIAN_POINT('',(1.9,-28.0490892825384,-25.6899024992348));
#70501=CARTESIAN_POINT('',(1.57538060255632,-28.2302951713764,-25.4739497302129));
#70502=CARTESIAN_POINT('',(0.,-29.1096888385212,-24.4259291680885));
#70503=CARTESIAN_POINT('',(1.57538060255632,-29.989082505666,-23.3779086059641));
#70504=CARTESIAN_POINT('Ctrl Pts',(1.57538060255632,-28.2302951713764,-25.4739497302129));
#70505=CARTESIAN_POINT('Ctrl Pts',(1.62460345738085,-29.1096888385412,-24.4259291680646));
#70506=CARTESIAN_POINT('Ctrl Pts',(1.57538060255632,-29.989082505666,-23.3779086059641));
#70507=CARTESIAN_POINT('',(1.9,-30.170288394504,-23.1619558369422));
#70508=CARTESIAN_POINT('',(1.9,-30.170288394504,-23.1619558369422));
#70509=CARTESIAN_POINT('',(4.5,-30.170288394504,-23.1619558369422));
#70510=CARTESIAN_POINT('',(4.5,-30.170288394504,-23.1619558369422));
#70511=CARTESIAN_POINT('',(4.5,-29.8488945896607,-23.5449780585017));
#70512=CARTESIAN_POINT('',(4.5,-29.8488945896607,-23.5449780585017));
#70513=CARTESIAN_POINT('',(10.9,-29.5917795457861,-23.8513958357493));
#70514=CARTESIAN_POINT('',(10.9,-29.5917795457861,-23.8513958357493));
#70515=CARTESIAN_POINT('',(11.9,-29.784615828692,-23.6215825028136));
#70516=CARTESIAN_POINT('',(11.9,-29.784615828692,-23.6215825028136));
#70517=CARTESIAN_POINT('',(12.6,-30.0417308725667,-23.315164725566));
#70518=CARTESIAN_POINT('',(12.6,-30.0417308725667,-23.315164725566));
#70519=CARTESIAN_POINT('',(13.2,-30.170288394504,-23.1619558369422));
#70520=CARTESIAN_POINT('',(13.2,-30.170288394504,-23.1619558369422));
#70521=CARTESIAN_POINT('',(21.8,-30.170288394504,-23.1619558369422));
#70522=CARTESIAN_POINT('',(21.8,-30.170288394504,-23.1619558369422));
#70523=CARTESIAN_POINT('',(22.4,-30.0417308725667,-23.315164725566));
#70524=CARTESIAN_POINT('',(22.4,-30.0417308725667,-23.315164725566));
#70525=CARTESIAN_POINT('',(23.1,-29.784615828692,-23.6215825028136));
#70526=CARTESIAN_POINT('',(23.1,-29.784615828692,-23.6215825028136));
#70527=CARTESIAN_POINT('',(24.1,-29.5917795457861,-23.8513958357493));
#70528=CARTESIAN_POINT('',(24.1,-29.5917795457861,-23.8513958357493));
#70529=CARTESIAN_POINT('',(30.5,-29.8488945896607,-23.5449780585017));
#70530=CARTESIAN_POINT('',(30.5,-29.8488945896607,-23.5449780585017));
#70531=CARTESIAN_POINT('',(30.5,-30.170288394504,-23.1619558369422));
#70532=CARTESIAN_POINT('',(30.5,-30.170288394504,-23.1619558369422));
#70533=CARTESIAN_POINT('',(33.1,-30.170288394504,-23.1619558369422));
#70534=CARTESIAN_POINT('',(33.1,-30.170288394504,-23.1619558369422));
#70535=CARTESIAN_POINT('',(35.,-29.1096888385212,-24.4259291680885));
#70536=CARTESIAN_POINT('Origin',(35.,-29.1096888385212,-24.4259291680885));
#70537=CARTESIAN_POINT('',(35.,-32.1800738014028,-28.156475035514));
#70538=CARTESIAN_POINT('',(35.,-6.7396658591028,2.75385375455791));
#70539=CARTESIAN_POINT('',(34.8617922858584,-32.1029248328492,-28.2484175959528));
#70540=CARTESIAN_POINT('',(33.5377160618333,-31.3638118563816,-29.129258140991));
#70541=CARTESIAN_POINT('',(34.4,-31.5410006112756,-28.1860830985703));
#70542=CARTESIAN_POINT('Ctrl Pts',(34.4,-31.5410006112756,-28.1860830985703));
#70543=CARTESIAN_POINT('Ctrl Pts',(34.6297825290998,-31.8210099935452,-28.2175888910031));
#70544=CARTESIAN_POINT('Ctrl Pts',(34.8617922858584,-32.1029248328492,-28.2484175959527));
#70545=CARTESIAN_POINT('',(33.3226453080309,-30.9143101784803,-28.872052684018));
#70546=CARTESIAN_POINT('Origin',(26.8550245390365,0.,0.));
#70547=CARTESIAN_POINT('',(33.0966075166785,-28.0054314386442,-25.6414155514355));
#70548=CARTESIAN_POINT('Origin',(17.5,-24.4259291680885,-29.1096888385212));
#70549=CARTESIAN_POINT('',(33.1,-23.1619558369422,-30.1702883945039));
#70550=CARTESIAN_POINT('',(33.1,-23.1619558369422,-30.1702883945039));
#70551=CARTESIAN_POINT('',(30.5,-23.1619558369422,-30.1702883945039));
#70552=CARTESIAN_POINT('',(30.5,-23.1619558369422,-30.1702883945039));
#70553=CARTESIAN_POINT('',(30.5,-23.5449780585017,-29.8488945896607));
#70554=CARTESIAN_POINT('',(30.5,-23.5449780585017,-29.8488945896607));
#70555=CARTESIAN_POINT('',(24.1,-23.8513958357493,-29.5917795457861));
#70556=CARTESIAN_POINT('',(24.1,-23.8513958357493,-29.5917795457861));
#70557=CARTESIAN_POINT('',(23.1,-23.6215825028136,-29.784615828692));
#70558=CARTESIAN_POINT('',(23.1,-23.6215825028136,-29.784615828692));
#70559=CARTESIAN_POINT('',(22.4,-23.315164725566,-30.0417308725666));
#70560=CARTESIAN_POINT('',(22.4,-23.315164725566,-30.0417308725666));
#70561=CARTESIAN_POINT('',(21.8,-23.1619558369422,-30.1702883945039));
#70562=CARTESIAN_POINT('',(21.8,-23.1619558369422,-30.1702883945039));
#70563=CARTESIAN_POINT('',(13.2,-23.1619558369422,-30.1702883945039));
#70564=CARTESIAN_POINT('',(13.2,-23.1619558369422,-30.1702883945039));
#70565=CARTESIAN_POINT('',(12.6,-23.315164725566,-30.0417308725666));
#70566=CARTESIAN_POINT('',(12.6,-23.315164725566,-30.0417308725666));
#70567=CARTESIAN_POINT('',(11.9,-23.6215825028136,-29.784615828692));
#70568=CARTESIAN_POINT('',(11.9,-23.6215825028136,-29.784615828692));
#70569=CARTESIAN_POINT('',(10.9,-23.8513958357493,-29.5917795457861));
#70570=CARTESIAN_POINT('',(10.9,-23.8513958357493,-29.5917795457861));
#70571=CARTESIAN_POINT('',(4.5,-23.5449780585017,-29.8488945896607));
#70572=CARTESIAN_POINT('',(4.5,-23.5449780585017,-29.8488945896607));
#70573=CARTESIAN_POINT('',(4.5,-23.1619558369422,-30.1702883945039));
#70574=CARTESIAN_POINT('',(4.5,-23.1619558369422,-30.1702883945039));
#70575=CARTESIAN_POINT('',(1.9,-23.1619558369422,-30.1702883945039));
#70576=CARTESIAN_POINT('',(1.9,-23.1619558369422,-30.1702883945039));
#70577=CARTESIAN_POINT('',(1.57538060255632,-23.3779086059641,-29.989082505666));
#70578=CARTESIAN_POINT('',(0.,-24.4259291680885,-29.1096888385212));
#70579=CARTESIAN_POINT('',(1.57538060255632,-25.4739497302129,-28.2302951713763));
#70580=CARTESIAN_POINT('Ctrl Pts',(1.57538060255632,-23.3779086059641,-29.989082505666));
#70581=CARTESIAN_POINT('Ctrl Pts',(1.62460345738085,-24.4259291681124,-29.1096888385011));
#70582=CARTESIAN_POINT('Ctrl Pts',(1.57538060255632,-25.4739497302129,-28.2302951713763));
#70583=CARTESIAN_POINT('',(1.9,-25.6899024992348,-28.0490892825384));
#70584=CARTESIAN_POINT('',(1.9,-25.6899024992348,-28.0490892825384));
#70585=CARTESIAN_POINT('',(4.5,-25.6899024992348,-28.0490892825384));
#70586=CARTESIAN_POINT('',(4.5,-25.6899024992348,-28.0490892825384));
#70587=CARTESIAN_POINT('',(4.5,-25.3068802776753,-28.3704830873816));
#70588=CARTESIAN_POINT('',(4.5,-25.3068802776753,-28.3704830873816));
#70589=CARTESIAN_POINT('',(10.9,-25.0004625004277,-28.6275981312563));
#70590=CARTESIAN_POINT('',(10.9,-25.0004625004277,-28.6275981312563));
#70591=CARTESIAN_POINT('',(11.9,-25.2302758333634,-28.4347618483503));
#70592=CARTESIAN_POINT('',(11.9,-25.2302758333634,-28.4347618483503));
#70593=CARTESIAN_POINT('',(12.6,-25.536693610611,-28.1776468044757));
#70594=CARTESIAN_POINT('',(12.6,-25.536693610611,-28.1776468044757));
#70595=CARTESIAN_POINT('',(13.2,-25.6899024992348,-28.0490892825384));
#70596=CARTESIAN_POINT('',(13.2,-25.6899024992348,-28.0490892825384));
#70597=CARTESIAN_POINT('',(21.8,-25.6899024992348,-28.0490892825384));
#70598=CARTESIAN_POINT('',(21.8,-25.6899024992348,-28.0490892825384));
#70599=CARTESIAN_POINT('',(22.4,-25.536693610611,-28.1776468044757));
#70600=CARTESIAN_POINT('',(22.4,-25.536693610611,-28.1776468044757));
#70601=CARTESIAN_POINT('',(23.1,-25.2302758333634,-28.4347618483503));
#70602=CARTESIAN_POINT('',(23.1,-25.2302758333634,-28.4347618483503));
#70603=CARTESIAN_POINT('',(24.1,-25.0004625004277,-28.6275981312563));
#70604=CARTESIAN_POINT('',(24.1,-25.0004625004277,-28.6275981312563));
#70605=CARTESIAN_POINT('',(30.5,-25.3068802776753,-28.3704830873816));
#70606=CARTESIAN_POINT('',(30.5,-25.3068802776753,-28.3704830873816));
#70607=CARTESIAN_POINT('',(30.5,-25.6899024992348,-28.0490892825384));
#70608=CARTESIAN_POINT('',(30.5,-25.6899024992348,-28.0490892825384));
#70609=CARTESIAN_POINT('',(33.1,-25.6899024992348,-28.0490892825384));
#70610=CARTESIAN_POINT('',(33.1,-25.6899024992348,-28.0490892825384));
#70611=CARTESIAN_POINT('',(35.,-24.4259291680885,-29.1096888385212));
#70612=CARTESIAN_POINT('Origin',(35.,-24.4259291680885,-29.1096888385212));
#70613=CARTESIAN_POINT('',(35.,-26.8018655926852,-33.3167260852698));
#70614=CARTESIAN_POINT('',(35.,-8.95315125918114,-1.71225837718511));
#70615=CARTESIAN_POINT('',(34.8617922858584,-26.7099230322464,-33.3938750538235));
#70616=CARTESIAN_POINT('',(33.5377160618333,-25.8290824872081,-34.132988030291));
#70617=CARTESIAN_POINT('',(34.4,-26.1673599741116,-33.234910440458));
#70618=CARTESIAN_POINT('Ctrl Pts',(34.4,-26.1673599741116,-33.234910440458));
#70619=CARTESIAN_POINT('Ctrl Pts',(34.6297825291012,-26.4376444612465,-33.3145607080718));
#70620=CARTESIAN_POINT('Ctrl Pts',(34.8617922858584,-26.7099230322464,-33.3938750538234));
#70621=CARTESIAN_POINT('',(33.322645308031,-25.4310730087083,-33.8016349549212));
#70622=CARTESIAN_POINT('Origin',(26.8550245390365,0.,0.));
#70623=CARTESIAN_POINT('',(33.0966075166785,-23.1273809239214,-30.1149569673582));
#70624=CARTESIAN_POINT('Origin',(17.5,-19.,-32.9089653438087));
#70625=CARTESIAN_POINT('',(33.1,-17.5710580837557,-33.7339653438087));
#70626=CARTESIAN_POINT('',(33.1,-17.5710580837557,-33.7339653438087));
#70627=CARTESIAN_POINT('',(30.5,-17.5710580837557,-33.7339653438087));
#70628=CARTESIAN_POINT('',(30.5,-17.5710580837557,-33.7339653438087));
#70629=CARTESIAN_POINT('',(30.5,-18.0040707856479,-33.4839653438087));
#70630=CARTESIAN_POINT('',(30.5,-18.0040707856479,-33.4839653438087));
#70631=CARTESIAN_POINT('',(24.1,-18.3504809471617,-33.2839653438087));
#70632=CARTESIAN_POINT('',(24.1,-18.3504809471617,-33.2839653438087));
#70633=CARTESIAN_POINT('',(23.1,-18.0906733260264,-33.4339653438087));
#70634=CARTESIAN_POINT('',(23.1,-18.0906733260264,-33.4339653438087));
#70635=CARTESIAN_POINT('',(22.4,-17.7442631645126,-33.6339653438087));
#70636=CARTESIAN_POINT('',(22.4,-17.7442631645126,-33.6339653438087));
#70637=CARTESIAN_POINT('',(21.8,-17.5710580837557,-33.7339653438087));
#70638=CARTESIAN_POINT('',(21.8,-17.5710580837557,-33.7339653438087));
#70639=CARTESIAN_POINT('',(13.2,-17.5710580837557,-33.7339653438087));
#70640=CARTESIAN_POINT('',(13.2,-17.5710580837557,-33.7339653438087));
#70641=CARTESIAN_POINT('',(12.6,-17.7442631645126,-33.6339653438087));
#70642=CARTESIAN_POINT('',(12.6,-17.7442631645126,-33.6339653438087));
#70643=CARTESIAN_POINT('',(11.9,-18.0906733260264,-33.4339653438087));
#70644=CARTESIAN_POINT('',(11.9,-18.0906733260264,-33.4339653438087));
#70645=CARTESIAN_POINT('',(10.9,-18.3504809471617,-33.2839653438087));
#70646=CARTESIAN_POINT('',(10.9,-18.3504809471617,-33.2839653438087));
#70647=CARTESIAN_POINT('',(4.5,-18.0040707856479,-33.4839653438087));
#70648=CARTESIAN_POINT('',(4.5,-18.0040707856479,-33.4839653438087));
#70649=CARTESIAN_POINT('',(4.5,-17.5710580837557,-33.7339653438087));
#70650=CARTESIAN_POINT('',(4.5,-17.5710580837557,-33.7339653438087));
#70651=CARTESIAN_POINT('',(1.9,-17.5710580837557,-33.7339653438087));
#70652=CARTESIAN_POINT('',(1.9,-17.5710580837557,-33.7339653438087));
#70653=CARTESIAN_POINT('',(1.57538060255633,-17.8151961173521,-33.5930121843923));
#70654=CARTESIAN_POINT('',(0.,-19.,-32.9089653438087));
#70655=CARTESIAN_POINT('',(1.57538060255632,-20.1848038826479,-32.224918503225));
#70656=CARTESIAN_POINT('Ctrl Pts',(1.57538060255633,-17.8151961173521,-33.5930121843923));
#70657=CARTESIAN_POINT('Ctrl Pts',(1.62460345738085,-19.000000000027,-32.9089653437931));
#70658=CARTESIAN_POINT('Ctrl Pts',(1.57538060255632,-20.1848038826479,-32.224918503225));
#70659=CARTESIAN_POINT('',(1.9,-20.4289419162443,-32.0839653438087));
#70660=CARTESIAN_POINT('',(1.9,-20.4289419162443,-32.0839653438087));
#70661=CARTESIAN_POINT('',(4.5,-20.4289419162443,-32.0839653438087));
#70662=CARTESIAN_POINT('',(4.5,-20.4289419162443,-32.0839653438087));
#70663=CARTESIAN_POINT('',(4.5,-19.9959292143521,-32.3339653438087));
#70664=CARTESIAN_POINT('',(4.5,-19.9959292143521,-32.3339653438087));
#70665=CARTESIAN_POINT('',(10.9,-19.6495190528383,-32.5339653438087));
#70666=CARTESIAN_POINT('',(10.9,-19.6495190528383,-32.5339653438087));
#70667=CARTESIAN_POINT('',(11.9,-19.9093266739737,-32.3839653438087));
#70668=CARTESIAN_POINT('',(11.9,-19.9093266739737,-32.3839653438087));
#70669=CARTESIAN_POINT('',(12.6,-20.2557368354875,-32.1839653438087));
#70670=CARTESIAN_POINT('',(12.6,-20.2557368354875,-32.1839653438087));
#70671=CARTESIAN_POINT('',(13.2,-20.4289419162443,-32.0839653438087));
#70672=CARTESIAN_POINT('',(13.2,-20.4289419162443,-32.0839653438087));
#70673=CARTESIAN_POINT('',(21.8,-20.4289419162443,-32.0839653438087));
#70674=CARTESIAN_POINT('',(21.8,-20.4289419162443,-32.0839653438087));
#70675=CARTESIAN_POINT('',(22.4,-20.2557368354875,-32.1839653438087));
#70676=CARTESIAN_POINT('',(22.4,-20.2557368354875,-32.1839653438087));
#70677=CARTESIAN_POINT('',(23.1,-19.9093266739737,-32.3839653438087));
#70678=CARTESIAN_POINT('',(23.1,-19.9093266739737,-32.3839653438087));
#70679=CARTESIAN_POINT('',(24.1,-19.6495190528383,-32.5339653438087));
#70680=CARTESIAN_POINT('',(24.1,-19.6495190528383,-32.5339653438087));
#70681=CARTESIAN_POINT('',(30.5,-19.9959292143521,-32.3339653438087));
#70682=CARTESIAN_POINT('',(30.5,-19.9959292143521,-32.3339653438087));
#70683=CARTESIAN_POINT('',(30.5,-20.4289419162443,-32.0839653438087));
#70684=CARTESIAN_POINT('',(30.5,-20.4289419162443,-32.0839653438087));
#70685=CARTESIAN_POINT('',(33.1,-20.4289419162443,-32.0839653438087));
#70686=CARTESIAN_POINT('',(33.1,-20.4289419162443,-32.0839653438087));
#70687=CARTESIAN_POINT('',(35.,-19.,-32.9089653438087));
#70688=CARTESIAN_POINT('Origin',(35.,-19.,-32.9089653438087));
#70689=CARTESIAN_POINT('',(35.,-20.6092962603321,-37.4646652720015));
#70690=CARTESIAN_POINT('',(35.,-9.89391142839378,-7.13086091745311));
#70691=CARTESIAN_POINT('',(34.8617922858584,-20.505353736182,-37.5246765162998));
#70692=CARTESIAN_POINT('',(33.5377160618333,-19.5095495168072,-38.099604350416));
#70693=CARTESIAN_POINT('',(34.4,-19.9986373454573,-37.2739118462884));
#70694=CARTESIAN_POINT('Ctrl Pts',(34.4,-19.9986373454573,-37.2739118462884));
#70695=CARTESIAN_POINT('Ctrl Pts',(34.6297825290997,-20.2509844800833,-37.3992864560058));
#70696=CARTESIAN_POINT('Ctrl Pts',(34.8617922858584,-20.505353736182,-37.5246765162998));
#70697=CARTESIAN_POINT('',(33.3226453080309,-19.1751255543105,-37.7041716521717));
#70698=CARTESIAN_POINT('Origin',(26.8550245390365,0.,0.));
#70699=CARTESIAN_POINT('',(33.0966075166785,-17.5466166428447,-33.6734706547313));
#70700=CARTESIAN_POINT('Origin',(17.5,-12.9967654463754,-35.7083195898645));
#70701=CARTESIAN_POINT('',(33.1,-11.4462726220787,-36.2726528263519));
#70702=CARTESIAN_POINT('',(33.1,-11.4462726220787,-36.2726528263519));
#70703=CARTESIAN_POINT('',(30.5,-11.4462726220787,-36.2726528263519));
#70704=CARTESIAN_POINT('',(30.5,-11.4462726220787,-36.2726528263519));
#70705=CARTESIAN_POINT('',(30.5,-11.9161189324716,-36.101642754689));
#70706=CARTESIAN_POINT('',(30.5,-11.9161189324716,-36.101642754689));
#70707=CARTESIAN_POINT('',(24.1,-12.291995980786,-35.9648346973588));
#70708=CARTESIAN_POINT('',(24.1,-12.291995980786,-35.9648346973588));
#70709=CARTESIAN_POINT('',(23.1,-12.0100881945502,-36.0674407403565));
#70710=CARTESIAN_POINT('',(23.1,-12.0100881945502,-36.0674407403565));
#70711=CARTESIAN_POINT('',(22.4,-11.6342111462359,-36.2042487976867));
#70712=CARTESIAN_POINT('',(22.4,-11.6342111462359,-36.2042487976867));
#70713=CARTESIAN_POINT('',(21.8,-11.4462726220787,-36.2726528263519));
#70714=CARTESIAN_POINT('',(21.8,-11.4462726220787,-36.2726528263519));
#70715=CARTESIAN_POINT('',(13.2,-11.4462726220787,-36.2726528263519));
#70716=CARTESIAN_POINT('',(13.2,-11.4462726220787,-36.2726528263519));
#70717=CARTESIAN_POINT('',(12.6,-11.6342111462359,-36.2042487976867));
#70718=CARTESIAN_POINT('',(12.6,-11.6342111462359,-36.2042487976867));
#70719=CARTESIAN_POINT('',(11.9,-12.0100881945502,-36.0674407403565));
#70720=CARTESIAN_POINT('',(11.9,-12.0100881945502,-36.0674407403565));
#70721=CARTESIAN_POINT('',(10.9,-12.291995980786,-35.9648346973588));
#70722=CARTESIAN_POINT('',(10.9,-12.291995980786,-35.9648346973588));
#70723=CARTESIAN_POINT('',(4.5,-11.9161189324716,-36.101642754689));
#70724=CARTESIAN_POINT('',(4.5,-11.9161189324716,-36.101642754689));
#70725=CARTESIAN_POINT('',(4.5,-11.4462726220787,-36.2726528263519));
#70726=CARTESIAN_POINT('',(4.5,-11.4462726220787,-36.2726528263519));
#70727=CARTESIAN_POINT('',(1.9,-11.4462726220787,-36.2726528263519));
#70728=CARTESIAN_POINT('',(1.9,-11.4462726220787,-36.2726528263519));
#70729=CARTESIAN_POINT('',(1.57538060255632,-11.7111779096387,-36.1762351867803));
#70730=CARTESIAN_POINT('',(0.,-12.9967654463754,-35.7083195898645));
#70731=CARTESIAN_POINT('',(1.57538060255632,-14.2823529831122,-35.2404039929487));
#70732=CARTESIAN_POINT('Ctrl Pts',(1.57538060255632,-11.7111779096387,-36.1762351867803));
#70733=CARTESIAN_POINT('Ctrl Pts',(1.62460345738085,-12.9967654464047,-35.7083195898538));
#70734=CARTESIAN_POINT('Ctrl Pts',(1.57538060255632,-14.2823529831122,-35.2404039929487));
#70735=CARTESIAN_POINT('',(1.9,-14.5472582706722,-35.1439863533772));
#70736=CARTESIAN_POINT('',(1.9,-14.5472582706722,-35.1439863533772));
#70737=CARTESIAN_POINT('',(4.5,-14.5472582706722,-35.1439863533772));
#70738=CARTESIAN_POINT('',(4.5,-14.5472582706722,-35.1439863533772));
#70739=CARTESIAN_POINT('',(4.5,-14.0774119602792,-35.31499642504));
#70740=CARTESIAN_POINT('',(4.5,-14.0774119602792,-35.31499642504));
#70741=CARTESIAN_POINT('',(10.9,-13.7015349119649,-35.4518044823703));
#70742=CARTESIAN_POINT('',(10.9,-13.7015349119649,-35.4518044823703));
#70743=CARTESIAN_POINT('',(11.9,-13.9834426982006,-35.3491984393726));
#70744=CARTESIAN_POINT('',(11.9,-13.9834426982006,-35.3491984393726));
#70745=CARTESIAN_POINT('',(12.6,-14.359319746515,-35.2123903820423));
#70746=CARTESIAN_POINT('',(12.6,-14.359319746515,-35.2123903820423));
#70747=CARTESIAN_POINT('',(13.2,-14.5472582706722,-35.1439863533772));
#70748=CARTESIAN_POINT('',(13.2,-14.5472582706722,-35.1439863533772));
#70749=CARTESIAN_POINT('',(21.8,-14.5472582706722,-35.1439863533772));
#70750=CARTESIAN_POINT('',(21.8,-14.5472582706722,-35.1439863533772));
#70751=CARTESIAN_POINT('',(22.4,-14.359319746515,-35.2123903820423));
#70752=CARTESIAN_POINT('',(22.4,-14.359319746515,-35.2123903820423));
#70753=CARTESIAN_POINT('',(23.1,-13.9834426982006,-35.3491984393726));
#70754=CARTESIAN_POINT('',(23.1,-13.9834426982006,-35.3491984393726));
#70755=CARTESIAN_POINT('',(24.1,-13.7015349119649,-35.4518044823703));
#70756=CARTESIAN_POINT('',(24.1,-13.7015349119649,-35.4518044823703));
#70757=CARTESIAN_POINT('',(30.5,-14.0774119602792,-35.31499642504));
#70758=CARTESIAN_POINT('',(30.5,-14.0774119602792,-35.31499642504));
#70759=CARTESIAN_POINT('',(30.5,-14.5472582706722,-35.1439863533772));
#70760=CARTESIAN_POINT('',(30.5,-14.5472582706722,-35.1439863533772));
#70761=CARTESIAN_POINT('',(33.1,-14.5472582706722,-35.1439863533772));
#70762=CARTESIAN_POINT('',(33.1,-14.5472582706722,-35.1439863533772));
#70763=CARTESIAN_POINT('',(35.,-12.9967654463754,-35.7083195898645));
#70764=CARTESIAN_POINT('Origin',(35.,-12.9967654463754,-35.7083195898645));
#70765=CARTESIAN_POINT('',(35.,-13.790523889916,-40.4742595624789));
#70766=CARTESIAN_POINT('',(35.,-9.22632453012935,-13.0695744862984));
#70767=CARTESIAN_POINT('',(34.8617922858584,-13.6777396430533,-40.515309671231));
#70768=CARTESIAN_POINT('',(33.5377160618333,-12.5972287566466,-40.9085834716836));
#70769=CARTESIAN_POINT('',(34.4,-13.22226624086,-40.1803643021789));
#70770=CARTESIAN_POINT('Ctrl Pts',(34.4,-13.22226624086,-40.1803643021789));
#70771=CARTESIAN_POINT('Ctrl Pts',(34.6297825290994,-13.4490085829866,-40.3476538099265));
#70772=CARTESIAN_POINT('Ctrl Pts',(34.8617922858584,-13.6777396430533,-40.515309671231));
#70773=CARTESIAN_POINT('',(33.3226453080309,-12.3365516130268,-40.4610861730024));
#70774=CARTESIAN_POINT('Origin',(26.8550245390365,0.,0.));
#70775=CARTESIAN_POINT('',(33.0966075166785,-11.4327072940916,-36.2088329758586));
#70776=CARTESIAN_POINT('Origin',(17.5,-6.59863075134335,-37.4226946144639));
#70777=CARTESIAN_POINT('',(33.1,-4.97369795887321,-37.7092141076143));
#70778=CARTESIAN_POINT('',(33.1,-4.97369795887321,-37.7092141076143));
#70779=CARTESIAN_POINT('',(30.5,-4.97369795887321,-37.7092141076143));
#70780=CARTESIAN_POINT('',(30.5,-4.97369795887321,-37.7092141076143));
#70781=CARTESIAN_POINT('',(30.5,-5.46610183537931,-37.6223900187809));
#70782=CARTESIAN_POINT('',(30.5,-5.46610183537931,-37.6223900187809));
#70783=CARTESIAN_POINT('',(24.1,-5.8600249365842,-37.5529307477141));
#70784=CARTESIAN_POINT('',(24.1,-5.8600249365842,-37.5529307477141));
#70785=CARTESIAN_POINT('',(23.1,-5.56458261068053,-37.6050252010142));
#70786=CARTESIAN_POINT('',(23.1,-5.56458261068053,-37.6050252010142));
#70787=CARTESIAN_POINT('',(22.4,-5.17065950947565,-37.674484472081));
#70788=CARTESIAN_POINT('',(22.4,-5.17065950947565,-37.674484472081));
#70789=CARTESIAN_POINT('',(21.8,-4.97369795887321,-37.7092141076143));
#70790=CARTESIAN_POINT('',(21.8,-4.97369795887321,-37.7092141076143));
#70791=CARTESIAN_POINT('',(13.2,-4.97369795887321,-37.7092141076143));
#70792=CARTESIAN_POINT('',(13.2,-4.97369795887321,-37.7092141076143));
#70793=CARTESIAN_POINT('',(12.6,-5.17065950947565,-37.674484472081));
#70794=CARTESIAN_POINT('',(12.6,-5.17065950947565,-37.674484472081));
#70795=CARTESIAN_POINT('',(11.9,-5.56458261068053,-37.6050252010142));
#70796=CARTESIAN_POINT('',(11.9,-5.56458261068053,-37.6050252010142));
#70797=CARTESIAN_POINT('',(10.9,-5.8600249365842,-37.5529307477141));
#70798=CARTESIAN_POINT('',(10.9,-5.8600249365842,-37.5529307477141));
#70799=CARTESIAN_POINT('',(4.5,-5.46610183537931,-37.6223900187809));
#70800=CARTESIAN_POINT('',(4.5,-5.46610183537931,-37.6223900187809));
#70801=CARTESIAN_POINT('',(4.5,-4.97369795887321,-37.7092141076143));
#70802=CARTESIAN_POINT('',(4.5,-4.97369795887321,-37.7092141076143));
#70803=CARTESIAN_POINT('',(1.9,-4.97369795887321,-37.7092141076143));
#70804=CARTESIAN_POINT('',(1.9,-4.97369795887321,-37.7092141076143));
#70805=CARTESIAN_POINT('',(1.57538060255632,-5.25132148728275,-37.6602615890763));
#70806=CARTESIAN_POINT('',(0.,-6.59863075134335,-37.4226946144639));
#70807=CARTESIAN_POINT('',(1.57538060255633,-7.94594001540395,-37.1851276398516));
#70808=CARTESIAN_POINT('Ctrl Pts',(1.57538060255632,-5.25132148728275,-37.6602615890763));
#70809=CARTESIAN_POINT('Ctrl Pts',(1.62460345738085,-6.59863075137406,-37.4226946144585));
#70810=CARTESIAN_POINT('Ctrl Pts',(1.57538060255633,-7.94594001540395,-37.1851276398516));
#70811=CARTESIAN_POINT('',(1.9,-8.2235635438135,-37.1361751213135));
#70812=CARTESIAN_POINT('',(1.9,-8.2235635438135,-37.1361751213135));
#70813=CARTESIAN_POINT('',(4.5,-8.2235635438135,-37.1361751213135));
#70814=CARTESIAN_POINT('',(4.5,-8.2235635438135,-37.1361751213135));
#70815=CARTESIAN_POINT('',(4.5,-7.73115966730739,-37.2229992101469));
#70816=CARTESIAN_POINT('',(4.5,-7.73115966730739,-37.2229992101469));
#70817=CARTESIAN_POINT('',(10.9,-7.33723656610251,-37.2924584812137));
#70818=CARTESIAN_POINT('',(10.9,-7.33723656610251,-37.2924584812137));
#70819=CARTESIAN_POINT('',(11.9,-7.63267889200617,-37.2403640279136));
#70820=CARTESIAN_POINT('',(11.9,-7.63267889200617,-37.2403640279136));
#70821=CARTESIAN_POINT('',(12.6,-8.02660199321105,-37.1709047568469));
#70822=CARTESIAN_POINT('',(12.6,-8.02660199321105,-37.1709047568469));
#70823=CARTESIAN_POINT('',(13.2,-8.2235635438135,-37.1361751213135));
#70824=CARTESIAN_POINT('',(13.2,-8.2235635438135,-37.1361751213135));
#70825=CARTESIAN_POINT('',(21.8,-8.2235635438135,-37.1361751213135));
#70826=CARTESIAN_POINT('',(21.8,-8.2235635438135,-37.1361751213135));
#70827=CARTESIAN_POINT('',(22.4,-8.02660199321105,-37.1709047568469));
#70828=CARTESIAN_POINT('',(22.4,-8.02660199321105,-37.1709047568469));
#70829=CARTESIAN_POINT('',(23.1,-7.63267889200617,-37.2403640279136));
#70830=CARTESIAN_POINT('',(23.1,-7.63267889200617,-37.2403640279136));
#70831=CARTESIAN_POINT('',(24.1,-7.33723656610251,-37.2924584812137));
#70832=CARTESIAN_POINT('',(24.1,-7.33723656610251,-37.2924584812137));
#70833=CARTESIAN_POINT('',(30.5,-7.73115966730739,-37.2229992101469));
#70834=CARTESIAN_POINT('',(30.5,-7.73115966730739,-37.2229992101469));
#70835=CARTESIAN_POINT('',(30.5,-8.2235635438135,-37.1361751213135));
#70836=CARTESIAN_POINT('',(30.5,-8.2235635438135,-37.1361751213135));
#70837=CARTESIAN_POINT('',(33.1,-8.2235635438135,-37.1361751213135));
#70838=CARTESIAN_POINT('',(33.1,-8.2235635438135,-37.1361751213135));
#70839=CARTESIAN_POINT('',(35.,-6.59863075134335,-37.4226946144639));
#70840=CARTESIAN_POINT('Origin',(35.,-6.59863075134335,-37.4226946144639));
#70841=CARTESIAN_POINT('',(35.,-6.55273342944652,-42.2540639571139));
#70842=CARTESIAN_POINT('',(35.,-6.77372590470163,-18.9913500169872));
#70843=CARTESIAN_POINT('',(34.8617922858584,-6.4345343521407,-42.2749056435377));
#70844=CARTESIAN_POINT('',(33.5377160618333,-5.30214757522046,-42.4745759849063));
#70845=CARTESIAN_POINT('',(34.4,-6.04414326732376,-41.8659567209931));
#70846=CARTESIAN_POINT('Ctrl Pts',(34.4,-6.04414326732376,-41.8659567209931));
#70847=CARTESIAN_POINT('Ctrl Pts',(34.6297825290996,-6.23839136562319,-42.0700781197309));
#70848=CARTESIAN_POINT('Ctrl Pts',(34.8617922858584,-6.4345343521407,-42.2749056435377));
#70849=CARTESIAN_POINT('',(33.3226453080309,-5.12313779357752,-41.9886110647639));
#70850=CARTESIAN_POINT('Origin',(26.8550245390365,0.,0.));
#70851=CARTESIAN_POINT('',(33.0966075166785,-4.97142091943645,-37.6440082295681));
#70852=CARTESIAN_POINT('Origin',(17.5,-6.98048675513991E-15,-38.));
#70853=CARTESIAN_POINT('',(33.1,1.64999999999999,-38.));
#70854=CARTESIAN_POINT('',(33.1,1.64999999999999,-38.));
#70855=CARTESIAN_POINT('',(30.5,1.64999999999999,-38.));
#70856=CARTESIAN_POINT('',(30.5,1.64999999999999,-38.));
#70857=CARTESIAN_POINT('',(30.5,1.14999999999999,-38.));
#70858=CARTESIAN_POINT('',(30.5,1.14999999999999,-38.));
#70859=CARTESIAN_POINT('',(24.1,0.749999999999993,-38.));
#70860=CARTESIAN_POINT('',(24.1,0.749999999999993,-38.));
#70861=CARTESIAN_POINT('',(23.1,1.04999999999999,-38.));
#70862=CARTESIAN_POINT('',(23.1,1.04999999999999,-38.));
#70863=CARTESIAN_POINT('',(22.4,1.44999999999999,-38.));
#70864=CARTESIAN_POINT('',(22.4,1.44999999999999,-38.));
#70865=CARTESIAN_POINT('',(21.8,1.64999999999999,-38.));
#70866=CARTESIAN_POINT('',(21.8,1.64999999999999,-38.));
#70867=CARTESIAN_POINT('',(13.2,1.64999999999999,-38.));
#70868=CARTESIAN_POINT('',(13.2,1.64999999999999,-38.));
#70869=CARTESIAN_POINT('',(12.6,1.44999999999999,-38.));
#70870=CARTESIAN_POINT('',(12.6,1.44999999999999,-38.));
#70871=CARTESIAN_POINT('',(11.9,1.04999999999999,-38.));
#70872=CARTESIAN_POINT('',(11.9,1.04999999999999,-38.));
#70873=CARTESIAN_POINT('',(10.9,0.749999999999993,-38.));
#70874=CARTESIAN_POINT('',(10.9,0.749999999999993,-38.));
#70875=CARTESIAN_POINT('',(4.5,1.14999999999999,-38.));
#70876=CARTESIAN_POINT('',(4.5,1.14999999999999,-38.));
#70877=CARTESIAN_POINT('',(4.5,1.64999999999999,-38.));
#70878=CARTESIAN_POINT('',(4.5,1.64999999999999,-38.));
#70879=CARTESIAN_POINT('',(1.9,1.64999999999999,-38.));
#70880=CARTESIAN_POINT('',(1.9,1.64999999999999,-38.));
#70881=CARTESIAN_POINT('',(1.57538060255632,1.36809368116733,-38.));
#70882=CARTESIAN_POINT('',(0.,-6.98048675513991E-15,-38.));
#70883=CARTESIAN_POINT('',(1.57538060255632,-1.36809368116734,-38.));
#70884=CARTESIAN_POINT('Ctrl Pts',(1.57538060255632,1.36809368116733,-38.));
#70885=CARTESIAN_POINT('Ctrl Pts',(1.62460345738085,-3.11864423174768E-11,
-38.));
#70886=CARTESIAN_POINT('Ctrl Pts',(1.57538060255632,-1.36809368116734,-38.));
#70887=CARTESIAN_POINT('',(1.9,-1.65000000000001,-38.));
#70888=CARTESIAN_POINT('',(1.9,-1.65000000000001,-38.));
#70889=CARTESIAN_POINT('',(4.5,-1.65000000000001,-38.));
#70890=CARTESIAN_POINT('',(4.5,-1.65000000000001,-38.));
#70891=CARTESIAN_POINT('',(4.5,-1.15000000000001,-38.));
#70892=CARTESIAN_POINT('',(4.5,-1.15000000000001,-38.));
#70893=CARTESIAN_POINT('',(10.9,-0.750000000000007,-38.));
#70894=CARTESIAN_POINT('',(10.9,-0.750000000000007,-38.));
#70895=CARTESIAN_POINT('',(11.9,-1.05000000000001,-38.));
#70896=CARTESIAN_POINT('',(11.9,-1.05000000000001,-38.));
#70897=CARTESIAN_POINT('',(12.6,-1.45000000000001,-38.));
#70898=CARTESIAN_POINT('',(12.6,-1.45000000000001,-38.));
#70899=CARTESIAN_POINT('',(13.2,-1.65000000000001,-38.));
#70900=CARTESIAN_POINT('',(13.2,-1.65000000000001,-38.));
#70901=CARTESIAN_POINT('',(21.8,-1.65000000000001,-38.));
#70902=CARTESIAN_POINT('',(21.8,-1.65000000000001,-38.));
#70903=CARTESIAN_POINT('',(22.4,-1.45000000000001,-38.));
#70904=CARTESIAN_POINT('',(22.4,-1.45000000000001,-38.));
#70905=CARTESIAN_POINT('',(23.1,-1.05000000000001,-38.));
#70906=CARTESIAN_POINT('',(23.1,-1.05000000000001,-38.));
#70907=CARTESIAN_POINT('',(24.1,-0.750000000000007,-38.));
#70908=CARTESIAN_POINT('',(24.1,-0.750000000000007,-38.));
#70909=CARTESIAN_POINT('',(30.5,-1.15000000000001,-38.));
#70910=CARTESIAN_POINT('',(30.5,-1.15000000000001,-38.));
#70911=CARTESIAN_POINT('',(30.5,-1.65000000000001,-38.));
#70912=CARTESIAN_POINT('',(30.5,-1.65000000000001,-38.));
#70913=CARTESIAN_POINT('',(33.1,-1.65000000000001,-38.));
#70914=CARTESIAN_POINT('',(33.1,-1.65000000000001,-38.));
#70915=CARTESIAN_POINT('',(35.,-6.98048675513991E-15,-38.));
#70916=CARTESIAN_POINT('Origin',(35.,-6.98048675513991E-15,-38.));
#70917=CARTESIAN_POINT('',(35.,0.884158520433528,-42.75));
#70918=CARTESIAN_POINT('',(35.,-2.54753088563723,-24.3137984568159));
#70919=CARTESIAN_POINT('',(34.8617922858584,1.0041810090302,-42.75));
#70920=CARTESIAN_POINT('',(33.5377160618333,2.15403667726254,-42.75));
#70921=CARTESIAN_POINT('',(34.4,1.31762794090604,-42.2794732300362));
#70922=CARTESIAN_POINT('Ctrl Pts',(34.4,1.31762794090604,-42.2794732300361));
#70923=CARTESIAN_POINT('Ctrl Pts',(34.6297825290971,1.16177621660823,-42.5142243943513));
#70924=CARTESIAN_POINT('Ctrl Pts',(34.8617922858584,1.0041810090302,-42.75));
#70925=CARTESIAN_POINT('',(33.322645308031,2.24593997529676,-42.240333256585));
#70926=CARTESIAN_POINT('Origin',(26.8550245390365,0.,0.));
#70927=CARTESIAN_POINT('',(33.0966075166785,1.64091956419533,-37.9353893420094));
#70928=CARTESIAN_POINT('Origin',(17.5,6.59863075134334,-37.4226946144639));
#70929=CARTESIAN_POINT('',(33.1,8.22356354381348,-37.1361751213135));
#70930=CARTESIAN_POINT('',(33.1,8.22356354381348,-37.1361751213135));
#70931=CARTESIAN_POINT('',(30.5,8.22356354381348,-37.1361751213135));
#70932=CARTESIAN_POINT('',(30.5,8.22356354381348,-37.1361751213135));
#70933=CARTESIAN_POINT('',(30.5,7.73115966730738,-37.2229992101469));
#70934=CARTESIAN_POINT('',(30.5,7.73115966730738,-37.2229992101469));
#70935=CARTESIAN_POINT('',(24.1,7.33723656610249,-37.2924584812137));
#70936=CARTESIAN_POINT('',(24.1,7.33723656610249,-37.2924584812137));
#70937=CARTESIAN_POINT('',(23.1,7.63267889200616,-37.2403640279136));
#70938=CARTESIAN_POINT('',(23.1,7.63267889200616,-37.2403640279136));
#70939=CARTESIAN_POINT('',(22.4,8.02660199321104,-37.1709047568469));
#70940=CARTESIAN_POINT('',(22.4,8.02660199321104,-37.1709047568469));
#70941=CARTESIAN_POINT('',(21.8,8.22356354381348,-37.1361751213135));
#70942=CARTESIAN_POINT('',(21.8,8.22356354381348,-37.1361751213135));
#70943=CARTESIAN_POINT('',(13.2,8.22356354381348,-37.1361751213135));
#70944=CARTESIAN_POINT('',(13.2,8.22356354381348,-37.1361751213135));
#70945=CARTESIAN_POINT('',(12.6,8.02660199321104,-37.1709047568469));
#70946=CARTESIAN_POINT('',(12.6,8.02660199321104,-37.1709047568469));
#70947=CARTESIAN_POINT('',(11.9,7.63267889200616,-37.2403640279136));
#70948=CARTESIAN_POINT('',(11.9,7.63267889200616,-37.2403640279136));
#70949=CARTESIAN_POINT('',(10.9,7.33723656610249,-37.2924584812137));
#70950=CARTESIAN_POINT('',(10.9,7.33723656610249,-37.2924584812137));
#70951=CARTESIAN_POINT('',(4.5,7.73115966730738,-37.2229992101469));
#70952=CARTESIAN_POINT('',(4.5,7.73115966730738,-37.2229992101469));
#70953=CARTESIAN_POINT('',(4.5,8.22356354381348,-37.1361751213135));
#70954=CARTESIAN_POINT('',(4.5,8.22356354381348,-37.1361751213135));
#70955=CARTESIAN_POINT('',(1.9,8.22356354381348,-37.1361751213135));
#70956=CARTESIAN_POINT('',(1.9,8.22356354381348,-37.1361751213135));
#70957=CARTESIAN_POINT('',(1.57538060255632,7.94594001540394,-37.1851276398516));
#70958=CARTESIAN_POINT('',(0.,6.59863075134334,-37.4226946144639));
#70959=CARTESIAN_POINT('',(1.57538060255633,5.25132148728273,-37.6602615890763));
#70960=CARTESIAN_POINT('Ctrl Pts',(1.57538060255632,7.94594001540394,-37.1851276398516));
#70961=CARTESIAN_POINT('Ctrl Pts',(1.62460345738085,6.59863075131263,-37.4226946144693));
#70962=CARTESIAN_POINT('Ctrl Pts',(1.57538060255633,5.25132148728273,-37.6602615890763));
#70963=CARTESIAN_POINT('',(1.9,4.9736979588732,-37.7092141076143));
#70964=CARTESIAN_POINT('',(1.9,4.9736979588732,-37.7092141076143));
#70965=CARTESIAN_POINT('',(4.5,4.9736979588732,-37.7092141076143));
#70966=CARTESIAN_POINT('',(4.5,4.9736979588732,-37.7092141076143));
#70967=CARTESIAN_POINT('',(4.5,5.4661018353793,-37.6223900187809));
#70968=CARTESIAN_POINT('',(4.5,5.4661018353793,-37.6223900187809));
#70969=CARTESIAN_POINT('',(10.9,5.86002493658418,-37.5529307477141));
#70970=CARTESIAN_POINT('',(10.9,5.86002493658418,-37.5529307477141));
#70971=CARTESIAN_POINT('',(11.9,5.56458261068052,-37.6050252010142));
#70972=CARTESIAN_POINT('',(11.9,5.56458261068052,-37.6050252010142));
#70973=CARTESIAN_POINT('',(12.6,5.17065950947564,-37.674484472081));
#70974=CARTESIAN_POINT('',(12.6,5.17065950947564,-37.674484472081));
#70975=CARTESIAN_POINT('',(13.2,4.9736979588732,-37.7092141076143));
#70976=CARTESIAN_POINT('',(13.2,4.9736979588732,-37.7092141076143));
#70977=CARTESIAN_POINT('',(21.8,4.9736979588732,-37.7092141076143));
#70978=CARTESIAN_POINT('',(21.8,4.9736979588732,-37.7092141076143));
#70979=CARTESIAN_POINT('',(22.4,5.17065950947564,-37.674484472081));
#70980=CARTESIAN_POINT('',(22.4,5.17065950947564,-37.674484472081));
#70981=CARTESIAN_POINT('',(23.1,5.56458261068052,-37.6050252010142));
#70982=CARTESIAN_POINT('',(23.1,5.56458261068052,-37.6050252010142));
#70983=CARTESIAN_POINT('',(24.1,5.86002493658418,-37.5529307477141));
#70984=CARTESIAN_POINT('',(24.1,5.86002493658418,-37.5529307477141));
#70985=CARTESIAN_POINT('',(30.5,5.4661018353793,-37.6223900187809));
#70986=CARTESIAN_POINT('',(30.5,5.4661018353793,-37.6223900187809));
#70987=CARTESIAN_POINT('',(30.5,4.9736979588732,-37.7092141076143));
#70988=CARTESIAN_POINT('',(30.5,4.9736979588732,-37.7092141076143));
#70989=CARTESIAN_POINT('',(33.1,4.9736979588732,-37.7092141076143));
#70990=CARTESIAN_POINT('',(33.1,4.9736979588732,-37.7092141076143));
#70991=CARTESIAN_POINT('',(35.,6.59863075134334,-37.4226946144639));
#70992=CARTESIAN_POINT('Origin',(35.,6.59863075134334,-37.4226946144639));
#70993=CARTESIAN_POINT('',(35.,8.294185761076,-41.9469989254299));
#70994=CARTESIAN_POINT('',(35.,3.24550057858058,-28.4754288467477));
#70995=CARTESIAN_POINT('',(34.8617922858584,8.41238483838183,-41.9261572390061));
#70996=CARTESIAN_POINT('',(33.5377160618333,9.54477161530206,-41.7264868976375));
#70997=CARTESIAN_POINT('',(34.4,8.63936369090331,-41.4083493394303));
#70998=CARTESIAN_POINT('Ctrl Pts',(34.4,8.63936369090331,-41.4083493394303));
#70999=CARTESIAN_POINT('Ctrl Pts',(34.6297825290999,8.5266438163816,-41.6665974739903));
#71000=CARTESIAN_POINT('Ctrl Pts',(34.8617922858584,8.41238483838183,-41.9261572390061));
#71001=CARTESIAN_POINT('',(33.322645308031,9.54677599452212,-41.2086042970448));
#71002=CARTESIAN_POINT('Origin',(26.8550245390365,0.,0.));
#71003=CARTESIAN_POINT('',(33.0966075166785,8.2034015372144,-37.0741228455271));
#71004=CARTESIAN_POINT('Origin',(17.5,12.9967654463754,-35.7083195898645));
#71005=CARTESIAN_POINT('',(33.1,14.5472582706721,-35.1439863533772));
#71006=CARTESIAN_POINT('',(33.1,14.5472582706721,-35.1439863533772));
#71007=CARTESIAN_POINT('',(30.5,14.5472582706721,-35.1439863533772));
#71008=CARTESIAN_POINT('',(30.5,14.5472582706721,-35.1439863533772));
#71009=CARTESIAN_POINT('',(30.5,14.0774119602792,-35.31499642504));
#71010=CARTESIAN_POINT('',(30.5,14.0774119602792,-35.31499642504));
#71011=CARTESIAN_POINT('',(24.1,13.7015349119648,-35.4518044823703));
#71012=CARTESIAN_POINT('',(24.1,13.7015349119648,-35.4518044823703));
#71013=CARTESIAN_POINT('',(23.1,13.9834426982006,-35.3491984393726));
#71014=CARTESIAN_POINT('',(23.1,13.9834426982006,-35.3491984393726));
#71015=CARTESIAN_POINT('',(22.4,14.359319746515,-35.2123903820423));
#71016=CARTESIAN_POINT('',(22.4,14.359319746515,-35.2123903820423));
#71017=CARTESIAN_POINT('',(21.8,14.5472582706721,-35.1439863533772));
#71018=CARTESIAN_POINT('',(21.8,14.5472582706721,-35.1439863533772));
#71019=CARTESIAN_POINT('',(13.2,14.5472582706721,-35.1439863533772));
#71020=CARTESIAN_POINT('',(13.2,14.5472582706721,-35.1439863533772));
#71021=CARTESIAN_POINT('',(12.6,14.359319746515,-35.2123903820423));
#71022=CARTESIAN_POINT('',(12.6,14.359319746515,-35.2123903820423));
#71023=CARTESIAN_POINT('',(11.9,13.9834426982006,-35.3491984393726));
#71024=CARTESIAN_POINT('',(11.9,13.9834426982006,-35.3491984393726));
#71025=CARTESIAN_POINT('',(10.9,13.7015349119648,-35.4518044823703));
#71026=CARTESIAN_POINT('',(10.9,13.7015349119648,-35.4518044823703));
#71027=CARTESIAN_POINT('',(4.5,14.0774119602792,-35.31499642504));
#71028=CARTESIAN_POINT('',(4.5,14.0774119602792,-35.31499642504));
#71029=CARTESIAN_POINT('',(4.5,14.5472582706721,-35.1439863533772));
#71030=CARTESIAN_POINT('',(4.5,14.5472582706721,-35.1439863533772));
#71031=CARTESIAN_POINT('',(1.9,14.5472582706721,-35.1439863533772));
#71032=CARTESIAN_POINT('',(1.9,14.5472582706721,-35.1439863533772));
#71033=CARTESIAN_POINT('',(1.57538060255632,14.2823529831122,-35.2404039929487));
#71034=CARTESIAN_POINT('',(0.,12.9967654463754,-35.7083195898645));
#71035=CARTESIAN_POINT('',(1.57538060255632,11.7111779096386,-36.1762351867803));
#71036=CARTESIAN_POINT('Ctrl Pts',(1.57538060255632,14.2823529831122,-35.2404039929487));
#71037=CARTESIAN_POINT('Ctrl Pts',(1.62460345738085,12.9967654463461,-35.7083195898752));
#71038=CARTESIAN_POINT('Ctrl Pts',(1.57538060255632,11.7111779096386,-36.1762351867803));
#71039=CARTESIAN_POINT('',(1.9,11.4462726220786,-36.2726528263519));
#71040=CARTESIAN_POINT('',(1.9,11.4462726220786,-36.2726528263519));
#71041=CARTESIAN_POINT('',(4.5,11.4462726220786,-36.2726528263519));
#71042=CARTESIAN_POINT('',(4.5,11.4462726220786,-36.2726528263519));
#71043=CARTESIAN_POINT('',(4.5,11.9161189324716,-36.101642754689));
#71044=CARTESIAN_POINT('',(4.5,11.9161189324716,-36.101642754689));
#71045=CARTESIAN_POINT('',(10.9,12.291995980786,-35.9648346973588));
#71046=CARTESIAN_POINT('',(10.9,12.291995980786,-35.9648346973588));
#71047=CARTESIAN_POINT('',(11.9,12.0100881945502,-36.0674407403565));
#71048=CARTESIAN_POINT('',(11.9,12.0100881945502,-36.0674407403565));
#71049=CARTESIAN_POINT('',(12.6,11.6342111462358,-36.2042487976867));
#71050=CARTESIAN_POINT('',(12.6,11.6342111462358,-36.2042487976867));
#71051=CARTESIAN_POINT('',(13.2,11.4462726220786,-36.2726528263519));
#71052=CARTESIAN_POINT('',(13.2,11.4462726220786,-36.2726528263519));
#71053=CARTESIAN_POINT('',(21.8,11.4462726220786,-36.2726528263519));
#71054=CARTESIAN_POINT('',(21.8,11.4462726220786,-36.2726528263519));
#71055=CARTESIAN_POINT('',(22.4,11.6342111462358,-36.2042487976867));
#71056=CARTESIAN_POINT('',(22.4,11.6342111462358,-36.2042487976867));
#71057=CARTESIAN_POINT('',(23.1,12.0100881945502,-36.0674407403565));
#71058=CARTESIAN_POINT('',(23.1,12.0100881945502,-36.0674407403565));
#71059=CARTESIAN_POINT('',(24.1,12.291995980786,-35.9648346973588));
#71060=CARTESIAN_POINT('',(24.1,12.291995980786,-35.9648346973588));
#71061=CARTESIAN_POINT('',(30.5,11.9161189324716,-36.101642754689));
#71062=CARTESIAN_POINT('',(30.5,11.9161189324716,-36.101642754689));
#71063=CARTESIAN_POINT('',(30.5,11.4462726220786,-36.2726528263519));
#71064=CARTESIAN_POINT('',(30.5,11.4462726220786,-36.2726528263519));
#71065=CARTESIAN_POINT('',(33.1,11.4462726220786,-36.2726528263519));
#71066=CARTESIAN_POINT('',(33.1,11.4462726220786,-36.2726528263519));
#71067=CARTESIAN_POINT('',(35.,12.9967654463754,-35.7083195898645));
#71068=CARTESIAN_POINT('Origin',(35.,12.9967654463754,-35.7083195898645));
#71069=CARTESIAN_POINT('',(35.,15.4521983644287,-39.8694595147163));
#71070=CARTESIAN_POINT('',(35.,10.2189962848885,-31.0009272294782));
#71071=CARTESIAN_POINT('',(34.8617922858584,15.5649826112914,-39.8284094059642));
#71072=CARTESIAN_POINT('',(33.5377160618333,16.6454934976981,-39.4351356055115));
#71073=CARTESIAN_POINT('',(34.4,15.6985967468815,-39.2790537077817));
#71074=CARTESIAN_POINT('Ctrl Pts',(34.4,15.6985967468815,-39.2790537077817));
#71075=CARTESIAN_POINT('Ctrl Pts',(34.6297825291022,15.6324336584855,-39.5529520736976));
#71076=CARTESIAN_POINT('Ctrl Pts',(34.8617922858584,15.5649826112914,-39.8284094059642));
#71077=CARTESIAN_POINT('',(33.3226453080309,16.5575380560557,-38.9247727484987));
#71078=CARTESIAN_POINT('Origin',(26.8550245390365,0.,0.));
#71079=CARTESIAN_POINT('',(33.0966075166785,14.5166273056467,-35.0863778867947));
#71080=CARTESIAN_POINT('Origin',(17.5,19.,-32.9089653438087));
#71081=CARTESIAN_POINT('',(33.1,20.4289419162443,-32.0839653438087));
#71082=CARTESIAN_POINT('',(33.1,20.4289419162443,-32.0839653438087));
#71083=CARTESIAN_POINT('',(30.5,20.4289419162443,-32.0839653438087));
#71084=CARTESIAN_POINT('',(30.5,20.4289419162443,-32.0839653438087));
#71085=CARTESIAN_POINT('',(30.5,19.9959292143521,-32.3339653438087));
#71086=CARTESIAN_POINT('',(30.5,19.9959292143521,-32.3339653438087));
#71087=CARTESIAN_POINT('',(24.1,19.6495190528383,-32.5339653438087));
#71088=CARTESIAN_POINT('',(24.1,19.6495190528383,-32.5339653438087));
#71089=CARTESIAN_POINT('',(23.1,19.9093266739737,-32.3839653438087));
#71090=CARTESIAN_POINT('',(23.1,19.9093266739737,-32.3839653438087));
#71091=CARTESIAN_POINT('',(22.4,20.2557368354874,-32.1839653438087));
#71092=CARTESIAN_POINT('',(22.4,20.2557368354874,-32.1839653438087));
#71093=CARTESIAN_POINT('',(21.8,20.4289419162443,-32.0839653438087));
#71094=CARTESIAN_POINT('',(21.8,20.4289419162443,-32.0839653438087));
#71095=CARTESIAN_POINT('',(13.2,20.4289419162443,-32.0839653438087));
#71096=CARTESIAN_POINT('',(13.2,20.4289419162443,-32.0839653438087));
#71097=CARTESIAN_POINT('',(12.6,20.2557368354874,-32.1839653438087));
#71098=CARTESIAN_POINT('',(12.6,20.2557368354874,-32.1839653438087));
#71099=CARTESIAN_POINT('',(11.9,19.9093266739737,-32.3839653438087));
#71100=CARTESIAN_POINT('',(11.9,19.9093266739737,-32.3839653438087));
#71101=CARTESIAN_POINT('',(10.9,19.6495190528383,-32.5339653438087));
#71102=CARTESIAN_POINT('',(10.9,19.6495190528383,-32.5339653438087));
#71103=CARTESIAN_POINT('',(4.5,19.9959292143521,-32.3339653438087));
#71104=CARTESIAN_POINT('',(4.5,19.9959292143521,-32.3339653438087));
#71105=CARTESIAN_POINT('',(4.5,20.4289419162443,-32.0839653438087));
#71106=CARTESIAN_POINT('',(4.5,20.4289419162443,-32.0839653438087));
#71107=CARTESIAN_POINT('',(1.9,20.4289419162443,-32.0839653438087));
#71108=CARTESIAN_POINT('',(1.9,20.4289419162443,-32.0839653438087));
#71109=CARTESIAN_POINT('',(1.57538060255632,20.1848038826479,-32.224918503225));
#71110=CARTESIAN_POINT('',(0.,19.,-32.9089653438087));
#71111=CARTESIAN_POINT('',(1.57538060255632,17.8151961173521,-33.5930121843923));
#71112=CARTESIAN_POINT('Ctrl Pts',(1.57538060255632,20.1848038826479,-32.224918503225));
#71113=CARTESIAN_POINT('Ctrl Pts',(1.62460345738085,18.999999999973,-32.9089653438243));
#71114=CARTESIAN_POINT('Ctrl Pts',(1.57538060255632,17.8151961173521,-33.5930121843923));
#71115=CARTESIAN_POINT('',(1.9,17.5710580837557,-33.7339653438087));
#71116=CARTESIAN_POINT('',(1.9,17.5710580837557,-33.7339653438087));
#71117=CARTESIAN_POINT('',(4.5,17.5710580837557,-33.7339653438087));
#71118=CARTESIAN_POINT('',(4.5,17.5710580837557,-33.7339653438087));
#71119=CARTESIAN_POINT('',(4.5,18.0040707856479,-33.4839653438087));
#71120=CARTESIAN_POINT('',(4.5,18.0040707856479,-33.4839653438087));
#71121=CARTESIAN_POINT('',(10.9,18.3504809471617,-33.2839653438087));
#71122=CARTESIAN_POINT('',(10.9,18.3504809471617,-33.2839653438087));
#71123=CARTESIAN_POINT('',(11.9,18.0906733260263,-33.4339653438087));
#71124=CARTESIAN_POINT('',(11.9,18.0906733260263,-33.4339653438087));
#71125=CARTESIAN_POINT('',(12.6,17.7442631645126,-33.6339653438087));
#71126=CARTESIAN_POINT('',(12.6,17.7442631645126,-33.6339653438087));
#71127=CARTESIAN_POINT('',(13.2,17.5710580837557,-33.7339653438087));
#71128=CARTESIAN_POINT('',(13.2,17.5710580837557,-33.7339653438087));
#71129=CARTESIAN_POINT('',(21.8,17.5710580837557,-33.7339653438087));
#71130=CARTESIAN_POINT('',(21.8,17.5710580837557,-33.7339653438087));
#71131=CARTESIAN_POINT('',(22.4,17.7442631645126,-33.6339653438087));
#71132=CARTESIAN_POINT('',(22.4,17.7442631645126,-33.6339653438087));
#71133=CARTESIAN_POINT('',(23.1,18.0906733260263,-33.4339653438087));
#71134=CARTESIAN_POINT('',(23.1,18.0906733260263,-33.4339653438087));
#71135=CARTESIAN_POINT('',(24.1,18.3504809471617,-33.2839653438087));
#71136=CARTESIAN_POINT('',(24.1,18.3504809471617,-33.2839653438087));
#71137=CARTESIAN_POINT('',(30.5,18.0040707856479,-33.4839653438087));
#71138=CARTESIAN_POINT('',(30.5,18.0040707856479,-33.4839653438087));
#71139=CARTESIAN_POINT('',(30.5,17.5710580837557,-33.7339653438087));
#71140=CARTESIAN_POINT('',(30.5,17.5710580837557,-33.7339653438087));
#71141=CARTESIAN_POINT('',(33.1,17.5710580837557,-33.7339653438087));
#71142=CARTESIAN_POINT('',(33.1,17.5710580837557,-33.7339653438087));
#71143=CARTESIAN_POINT('',(35.,19.,-32.9089653438087));
#71144=CARTESIAN_POINT('Origin',(35.,19.,-32.9089653438087));
#71145=CARTESIAN_POINT('',(35.,22.1407037396679,-36.580506751568));
#71146=CARTESIAN_POINT('',(35.,17.8440832811487,-31.5576770820153));
#71147=CARTESIAN_POINT('',(34.8617922858584,22.2446462638181,-36.5204955072696));
#71148=CARTESIAN_POINT('',(33.5377160618333,23.2404504831928,-35.9455676731535));
#71149=CARTESIAN_POINT('',(34.4,22.2808358845789,-35.9562839053824));
#71150=CARTESIAN_POINT('Ctrl Pts',(34.4,22.2808358845789,-35.9562839053824));
#71151=CARTESIAN_POINT('Ctrl Pts',(34.6297825291023,22.2632399142705,-36.2375102394025));
#71152=CARTESIAN_POINT('Ctrl Pts',(34.8617922858584,22.2446462638181,-36.5204955072696));
#71153=CARTESIAN_POINT('',(33.322645308031,23.0652077022745,-35.4582316768749));
#71154=CARTESIAN_POINT('Origin',(26.8550245390365,0.,0.));
#71155=CARTESIAN_POINT('',(33.0966075166785,20.3887726991648,-32.0325510905359));
#71156=CARTESIAN_POINT('Origin',(17.5,24.4259291680885,-29.1096888385212));
#71157=CARTESIAN_POINT('',(33.1,25.6899024992348,-28.0490892825384));
#71158=CARTESIAN_POINT('',(33.1,25.6899024992348,-28.0490892825384));
#71159=CARTESIAN_POINT('',(30.5,25.6899024992348,-28.0490892825384));
#71160=CARTESIAN_POINT('',(30.5,25.6899024992348,-28.0490892825384));
#71161=CARTESIAN_POINT('',(30.5,25.3068802776753,-28.3704830873817));
#71162=CARTESIAN_POINT('',(30.5,25.3068802776753,-28.3704830873817));
#71163=CARTESIAN_POINT('',(24.1,25.0004625004277,-28.6275981312563));
#71164=CARTESIAN_POINT('',(24.1,25.0004625004277,-28.6275981312563));
#71165=CARTESIAN_POINT('',(23.1,25.2302758333634,-28.4347618483503));
#71166=CARTESIAN_POINT('',(23.1,25.2302758333634,-28.4347618483503));
#71167=CARTESIAN_POINT('',(22.4,25.536693610611,-28.1776468044757));
#71168=CARTESIAN_POINT('',(22.4,25.536693610611,-28.1776468044757));
#71169=CARTESIAN_POINT('',(21.8,25.6899024992348,-28.0490892825384));
#71170=CARTESIAN_POINT('',(21.8,25.6899024992348,-28.0490892825384));
#71171=CARTESIAN_POINT('',(13.2,25.6899024992348,-28.0490892825384));
#71172=CARTESIAN_POINT('',(13.2,25.6899024992348,-28.0490892825384));
#71173=CARTESIAN_POINT('',(12.6,25.536693610611,-28.1776468044757));
#71174=CARTESIAN_POINT('',(12.6,25.536693610611,-28.1776468044757));
#71175=CARTESIAN_POINT('',(11.9,25.2302758333634,-28.4347618483503));
#71176=CARTESIAN_POINT('',(11.9,25.2302758333634,-28.4347618483503));
#71177=CARTESIAN_POINT('',(10.9,25.0004625004277,-28.6275981312563));
#71178=CARTESIAN_POINT('',(10.9,25.0004625004277,-28.6275981312563));
#71179=CARTESIAN_POINT('',(4.5,25.3068802776753,-28.3704830873817));
#71180=CARTESIAN_POINT('',(4.5,25.3068802776753,-28.3704830873817));
#71181=CARTESIAN_POINT('',(4.5,25.6899024992348,-28.0490892825384));
#71182=CARTESIAN_POINT('',(4.5,25.6899024992348,-28.0490892825384));
#71183=CARTESIAN_POINT('',(1.9,25.6899024992348,-28.0490892825384));
#71184=CARTESIAN_POINT('',(1.9,25.6899024992348,-28.0490892825384));
#71185=CARTESIAN_POINT('',(1.57538060255632,25.4739497302129,-28.2302951713764));
#71186=CARTESIAN_POINT('',(0.,24.4259291680885,-29.1096888385212));
#71187=CARTESIAN_POINT('',(1.57538060255632,23.3779086059641,-29.989082505666));
#71188=CARTESIAN_POINT('Ctrl Pts',(1.57538060255632,25.4739497302129,-28.2302951713764));
#71189=CARTESIAN_POINT('Ctrl Pts',(1.62460345738084,24.4259291680646,-29.1096888385412));
#71190=CARTESIAN_POINT('Ctrl Pts',(1.57538060255632,23.3779086059641,-29.989082505666));
#71191=CARTESIAN_POINT('',(1.9,23.1619558369422,-30.170288394504));
#71192=CARTESIAN_POINT('',(1.9,23.1619558369422,-30.170288394504));
#71193=CARTESIAN_POINT('',(4.5,23.1619558369422,-30.170288394504));
#71194=CARTESIAN_POINT('',(4.5,23.1619558369422,-30.170288394504));
#71195=CARTESIAN_POINT('',(4.5,23.5449780585017,-29.8488945896607));
#71196=CARTESIAN_POINT('',(4.5,23.5449780585017,-29.8488945896607));
#71197=CARTESIAN_POINT('',(10.9,23.8513958357493,-29.5917795457861));
#71198=CARTESIAN_POINT('',(10.9,23.8513958357493,-29.5917795457861));
#71199=CARTESIAN_POINT('',(11.9,23.6215825028136,-29.784615828692));
#71200=CARTESIAN_POINT('',(11.9,23.6215825028136,-29.784615828692));
#71201=CARTESIAN_POINT('',(12.6,23.315164725566,-30.0417308725667));
#71202=CARTESIAN_POINT('',(12.6,23.315164725566,-30.0417308725667));
#71203=CARTESIAN_POINT('',(13.2,23.1619558369422,-30.170288394504));
#71204=CARTESIAN_POINT('',(13.2,23.1619558369422,-30.170288394504));
#71205=CARTESIAN_POINT('',(21.8,23.1619558369422,-30.170288394504));
#71206=CARTESIAN_POINT('',(21.8,23.1619558369422,-30.170288394504));
#71207=CARTESIAN_POINT('',(22.4,23.315164725566,-30.0417308725667));
#71208=CARTESIAN_POINT('',(22.4,23.315164725566,-30.0417308725667));
#71209=CARTESIAN_POINT('',(23.1,23.6215825028136,-29.784615828692));
#71210=CARTESIAN_POINT('',(23.1,23.6215825028136,-29.784615828692));
#71211=CARTESIAN_POINT('',(24.1,23.8513958357493,-29.5917795457861));
#71212=CARTESIAN_POINT('',(24.1,23.8513958357493,-29.5917795457861));
#71213=CARTESIAN_POINT('',(30.5,23.5449780585017,-29.8488945896607));
#71214=CARTESIAN_POINT('',(30.5,23.5449780585017,-29.8488945896607));
#71215=CARTESIAN_POINT('',(30.5,23.1619558369422,-30.170288394504));
#71216=CARTESIAN_POINT('',(30.5,23.1619558369422,-30.170288394504));
#71217=CARTESIAN_POINT('',(33.1,23.1619558369422,-30.170288394504));
#71218=CARTESIAN_POINT('',(33.1,23.1619558369422,-30.170288394504));
#71219=CARTESIAN_POINT('',(35.,24.4259291680885,-29.1096888385212));
#71220=CARTESIAN_POINT('Origin',(35.,24.4259291680885,-29.1096888385212));
#71221=CARTESIAN_POINT('',(35.,28.156475035514,-32.1800738014028));
#71222=CARTESIAN_POINT('',(35.,25.5036906911557,-29.9967286690438));
#71223=CARTESIAN_POINT('',(34.8617922858584,28.2484175959528,-32.1029248328492));
#71224=CARTESIAN_POINT('',(33.5377160618333,29.129258140991,-31.3638118563816));
#71225=CARTESIAN_POINT('',(34.4,28.1860830985703,-31.5410006112756));
#71226=CARTESIAN_POINT('Ctrl Pts',(34.4,28.1860830985703,-31.5410006112756));
#71227=CARTESIAN_POINT('Ctrl Pts',(34.6297825290989,28.217588891003,-31.821009993544));
#71228=CARTESIAN_POINT('Ctrl Pts',(34.8617922858584,28.2484175959528,-32.1029248328492));
#71229=CARTESIAN_POINT('',(33.3226453080309,28.872052684018,-30.9143101784803));
#71230=CARTESIAN_POINT('Origin',(26.8550245390365,0.,0.));
#71231=CARTESIAN_POINT('',(33.0966075166785,25.6414155514355,-28.0054314386442));
#71232=CARTESIAN_POINT('Origin',(17.5,29.1096888385212,-24.4259291680885));
#71233=CARTESIAN_POINT('',(33.1,30.1702883945039,-23.1619558369422));
#71234=CARTESIAN_POINT('',(33.1,30.1702883945039,-23.1619558369422));
#71235=CARTESIAN_POINT('',(30.5,30.1702883945039,-23.1619558369422));
#71236=CARTESIAN_POINT('',(30.5,30.1702883945039,-23.1619558369422));
#71237=CARTESIAN_POINT('',(30.5,29.8488945896607,-23.5449780585017));
#71238=CARTESIAN_POINT('',(30.5,29.8488945896607,-23.5449780585017));
#71239=CARTESIAN_POINT('',(24.1,29.5917795457861,-23.8513958357493));
#71240=CARTESIAN_POINT('',(24.1,29.5917795457861,-23.8513958357493));
#71241=CARTESIAN_POINT('',(23.1,29.784615828692,-23.6215825028136));
#71242=CARTESIAN_POINT('',(23.1,29.784615828692,-23.6215825028136));
#71243=CARTESIAN_POINT('',(22.4,30.0417308725666,-23.315164725566));
#71244=CARTESIAN_POINT('',(22.4,30.0417308725666,-23.315164725566));
#71245=CARTESIAN_POINT('',(21.8,30.1702883945039,-23.1619558369422));
#71246=CARTESIAN_POINT('',(21.8,30.1702883945039,-23.1619558369422));
#71247=CARTESIAN_POINT('',(13.2,30.1702883945039,-23.1619558369422));
#71248=CARTESIAN_POINT('',(13.2,30.1702883945039,-23.1619558369422));
#71249=CARTESIAN_POINT('',(12.6,30.0417308725666,-23.315164725566));
#71250=CARTESIAN_POINT('',(12.6,30.0417308725666,-23.315164725566));
#71251=CARTESIAN_POINT('',(11.9,29.784615828692,-23.6215825028136));
#71252=CARTESIAN_POINT('',(11.9,29.784615828692,-23.6215825028136));
#71253=CARTESIAN_POINT('',(10.9,29.5917795457861,-23.8513958357493));
#71254=CARTESIAN_POINT('',(10.9,29.5917795457861,-23.8513958357493));
#71255=CARTESIAN_POINT('',(4.5,29.8488945896607,-23.5449780585017));
#71256=CARTESIAN_POINT('',(4.5,29.8488945896607,-23.5449780585017));
#71257=CARTESIAN_POINT('',(4.5,30.1702883945039,-23.1619558369422));
#71258=CARTESIAN_POINT('',(4.5,30.1702883945039,-23.1619558369422));
#71259=CARTESIAN_POINT('',(1.9,30.1702883945039,-23.1619558369422));
#71260=CARTESIAN_POINT('',(1.9,30.1702883945039,-23.1619558369422));
#71261=CARTESIAN_POINT('',(1.57538060255632,29.989082505666,-23.3779086059641));
#71262=CARTESIAN_POINT('',(0.,29.1096888385212,-24.4259291680885));
#71263=CARTESIAN_POINT('',(1.57538060255632,28.2302951713763,-25.4739497302129));
#71264=CARTESIAN_POINT('Ctrl Pts',(1.57538060255632,29.989082505666,-23.3779086059641));
#71265=CARTESIAN_POINT('Ctrl Pts',(1.62460345738085,29.1096888385011,-24.4259291681124));
#71266=CARTESIAN_POINT('Ctrl Pts',(1.57538060255632,28.2302951713763,-25.4739497302129));
#71267=CARTESIAN_POINT('',(1.9,28.0490892825384,-25.6899024992348));
#71268=CARTESIAN_POINT('',(1.9,28.0490892825384,-25.6899024992348));
#71269=CARTESIAN_POINT('',(4.5,28.0490892825384,-25.6899024992348));
#71270=CARTESIAN_POINT('',(4.5,28.0490892825384,-25.6899024992348));
#71271=CARTESIAN_POINT('',(4.5,28.3704830873816,-25.3068802776753));
#71272=CARTESIAN_POINT('',(4.5,28.3704830873816,-25.3068802776753));
#71273=CARTESIAN_POINT('',(10.9,28.6275981312562,-25.0004625004277));
#71274=CARTESIAN_POINT('',(10.9,28.6275981312562,-25.0004625004277));
#71275=CARTESIAN_POINT('',(11.9,28.4347618483503,-25.2302758333634));
#71276=CARTESIAN_POINT('',(11.9,28.4347618483503,-25.2302758333634));
#71277=CARTESIAN_POINT('',(12.6,28.1776468044757,-25.536693610611));
#71278=CARTESIAN_POINT('',(12.6,28.1776468044757,-25.536693610611));
#71279=CARTESIAN_POINT('',(13.2,28.0490892825384,-25.6899024992348));
#71280=CARTESIAN_POINT('',(13.2,28.0490892825384,-25.6899024992348));
#71281=CARTESIAN_POINT('',(21.8,28.0490892825384,-25.6899024992348));
#71282=CARTESIAN_POINT('',(21.8,28.0490892825384,-25.6899024992348));
#71283=CARTESIAN_POINT('',(22.4,28.1776468044757,-25.536693610611));
#71284=CARTESIAN_POINT('',(22.4,28.1776468044757,-25.536693610611));
#71285=CARTESIAN_POINT('',(23.1,28.4347618483503,-25.2302758333634));
#71286=CARTESIAN_POINT('',(23.1,28.4347618483503,-25.2302758333634));
#71287=CARTESIAN_POINT('',(24.1,28.6275981312562,-25.0004625004277));
#71288=CARTESIAN_POINT('',(24.1,28.6275981312562,-25.0004625004277));
#71289=CARTESIAN_POINT('',(30.5,28.3704830873816,-25.3068802776753));
#71290=CARTESIAN_POINT('',(30.5,28.3704830873816,-25.3068802776753));
#71291=CARTESIAN_POINT('',(30.5,28.0490892825384,-25.6899024992348));
#71292=CARTESIAN_POINT('',(30.5,28.0490892825384,-25.6899024992348));
#71293=CARTESIAN_POINT('',(33.1,28.0490892825384,-25.6899024992348));
#71294=CARTESIAN_POINT('',(33.1,28.0490892825384,-25.6899024992348));
#71295=CARTESIAN_POINT('',(35.,29.1096888385212,-24.4259291680885));
#71296=CARTESIAN_POINT('Origin',(35.,29.1096888385212,-24.4259291680885));
#71297=CARTESIAN_POINT('',(35.,33.3167260852698,-26.8018655926852));
#71298=CARTESIAN_POINT('',(35.,32.5577823964916,-26.3732499544995));
#71299=CARTESIAN_POINT('',(34.8617922858584,33.3938750538235,-26.7099230322464));
#71300=CARTESIAN_POINT('',(33.5377160618333,34.132988030291,-25.8290824872081));
#71301=CARTESIAN_POINT('',(34.4,33.234910440458,-26.1673599741116));
#71302=CARTESIAN_POINT('Ctrl Pts',(34.4,33.234910440458,-26.1673599741116));
#71303=CARTESIAN_POINT('Ctrl Pts',(34.629782529103,33.3145607080724,-26.4376444612486));
#71304=CARTESIAN_POINT('Ctrl Pts',(34.8617922858584,33.3938750538235,-26.7099230322464));
#71305=CARTESIAN_POINT('',(33.3226453080309,33.8016349549212,-25.4310730087083));
#71306=CARTESIAN_POINT('Origin',(26.8550245390365,0.,0.));
#71307=CARTESIAN_POINT('',(33.0966075166785,30.1149569673582,-23.1273809239214));
#71308=CARTESIAN_POINT('Origin',(17.5,32.9089653438087,-19.));
#71309=CARTESIAN_POINT('',(33.1,33.7339653438087,-17.5710580837557));
#71310=CARTESIAN_POINT('',(33.1,33.7339653438087,-17.5710580837557));
#71311=CARTESIAN_POINT('',(30.5,33.7339653438087,-17.5710580837557));
#71312=CARTESIAN_POINT('',(30.5,33.7339653438087,-17.5710580837557));
#71313=CARTESIAN_POINT('',(30.5,33.4839653438087,-18.0040707856479));
#71314=CARTESIAN_POINT('',(30.5,33.4839653438087,-18.0040707856479));
#71315=CARTESIAN_POINT('',(24.1,33.2839653438087,-18.3504809471617));
#71316=CARTESIAN_POINT('',(24.1,33.2839653438087,-18.3504809471617));
#71317=CARTESIAN_POINT('',(23.1,33.4339653438087,-18.0906733260264));
#71318=CARTESIAN_POINT('',(23.1,33.4339653438087,-18.0906733260264));
#71319=CARTESIAN_POINT('',(22.4,33.6339653438087,-17.7442631645126));
#71320=CARTESIAN_POINT('',(22.4,33.6339653438087,-17.7442631645126));
#71321=CARTESIAN_POINT('',(21.8,33.7339653438087,-17.5710580837557));
#71322=CARTESIAN_POINT('',(21.8,33.7339653438087,-17.5710580837557));
#71323=CARTESIAN_POINT('',(13.2,33.7339653438087,-17.5710580837557));
#71324=CARTESIAN_POINT('',(13.2,33.7339653438087,-17.5710580837557));
#71325=CARTESIAN_POINT('',(12.6,33.6339653438087,-17.7442631645126));
#71326=CARTESIAN_POINT('',(12.6,33.6339653438087,-17.7442631645126));
#71327=CARTESIAN_POINT('',(11.9,33.4339653438087,-18.0906733260264));
#71328=CARTESIAN_POINT('',(11.9,33.4339653438087,-18.0906733260264));
#71329=CARTESIAN_POINT('',(10.9,33.2839653438087,-18.3504809471617));
#71330=CARTESIAN_POINT('',(10.9,33.2839653438087,-18.3504809471617));
#71331=CARTESIAN_POINT('',(4.5,33.4839653438087,-18.0040707856479));
#71332=CARTESIAN_POINT('',(4.5,33.4839653438087,-18.0040707856479));
#71333=CARTESIAN_POINT('',(4.5,33.7339653438087,-17.5710580837557));
#71334=CARTESIAN_POINT('',(4.5,33.7339653438087,-17.5710580837557));
#71335=CARTESIAN_POINT('',(1.9,33.7339653438087,-17.5710580837557));
#71336=CARTESIAN_POINT('',(1.9,33.7339653438087,-17.5710580837557));
#71337=CARTESIAN_POINT('',(1.57538060255633,33.5930121843923,-17.8151961173521));
#71338=CARTESIAN_POINT('',(0.,32.9089653438087,-19.));
#71339=CARTESIAN_POINT('',(1.57538060255632,32.224918503225,-20.1848038826479));
#71340=CARTESIAN_POINT('Ctrl Pts',(1.57538060255633,33.5930121843923,-17.8151961173521));
#71341=CARTESIAN_POINT('Ctrl Pts',(1.62460345738085,32.9089653437931,-19.000000000027));
#71342=CARTESIAN_POINT('Ctrl Pts',(1.57538060255632,32.224918503225,-20.1848038826479));
#71343=CARTESIAN_POINT('',(1.9,32.0839653438087,-20.4289419162443));
#71344=CARTESIAN_POINT('',(1.9,32.0839653438087,-20.4289419162443));
#71345=CARTESIAN_POINT('',(4.5,32.0839653438087,-20.4289419162443));
#71346=CARTESIAN_POINT('',(4.5,32.0839653438087,-20.4289419162443));
#71347=CARTESIAN_POINT('',(4.5,32.3339653438087,-19.9959292143521));
#71348=CARTESIAN_POINT('',(4.5,32.3339653438087,-19.9959292143521));
#71349=CARTESIAN_POINT('',(10.9,32.5339653438087,-19.6495190528383));
#71350=CARTESIAN_POINT('',(10.9,32.5339653438087,-19.6495190528383));
#71351=CARTESIAN_POINT('',(11.9,32.3839653438087,-19.9093266739737));
#71352=CARTESIAN_POINT('',(11.9,32.3839653438087,-19.9093266739737));
#71353=CARTESIAN_POINT('',(12.6,32.1839653438087,-20.2557368354875));
#71354=CARTESIAN_POINT('',(12.6,32.1839653438087,-20.2557368354875));
#71355=CARTESIAN_POINT('',(13.2,32.0839653438087,-20.4289419162443));
#71356=CARTESIAN_POINT('',(13.2,32.0839653438087,-20.4289419162443));
#71357=CARTESIAN_POINT('',(21.8,32.0839653438087,-20.4289419162443));
#71358=CARTESIAN_POINT('',(21.8,32.0839653438087,-20.4289419162443));
#71359=CARTESIAN_POINT('',(22.4,32.1839653438087,-20.2557368354875));
#71360=CARTESIAN_POINT('',(22.4,32.1839653438087,-20.2557368354875));
#71361=CARTESIAN_POINT('',(23.1,32.3839653438087,-19.9093266739737));
#71362=CARTESIAN_POINT('',(23.1,32.3839653438087,-19.9093266739737));
#71363=CARTESIAN_POINT('',(24.1,32.5339653438087,-19.6495190528383));
#71364=CARTESIAN_POINT('',(24.1,32.5339653438087,-19.6495190528383));
#71365=CARTESIAN_POINT('',(30.5,32.3339653438087,-19.9959292143521));
#71366=CARTESIAN_POINT('',(30.5,32.3339653438087,-19.9959292143521));
#71367=CARTESIAN_POINT('',(30.5,32.0839653438087,-20.4289419162443));
#71368=CARTESIAN_POINT('',(30.5,32.0839653438087,-20.4289419162443));
#71369=CARTESIAN_POINT('',(33.1,32.0839653438087,-20.4289419162443));
#71370=CARTESIAN_POINT('',(33.1,32.0839653438087,-20.4289419162443));
#71371=CARTESIAN_POINT('',(35.,32.9089653438087,-19.));
#71372=CARTESIAN_POINT('Origin',(35.,32.9089653438087,-19.));
#71373=CARTESIAN_POINT('',(35.,37.4646652720015,-20.6092962603321));
#71374=CARTESIAN_POINT('',(35.,38.4119309417395,-20.943916872725));
#71375=CARTESIAN_POINT('',(34.8617922858584,37.5246765162998,-20.505353736182));
#71376=CARTESIAN_POINT('',(33.5377160618333,38.099604350416,-19.5095495168072));
#71377=CARTESIAN_POINT('',(34.4,37.2739118462884,-19.9986373454573));
#71378=CARTESIAN_POINT('Ctrl Pts',(34.4,37.2739118462884,-19.9986373454573));
#71379=CARTESIAN_POINT('Ctrl Pts',(34.6297825290997,37.3992864560058,-20.2509844800833));
#71380=CARTESIAN_POINT('Ctrl Pts',(34.8617922858584,37.5246765162998,-20.505353736182));
#71381=CARTESIAN_POINT('',(33.3226453080309,37.7041716521717,-19.1751255543105));
#71382=CARTESIAN_POINT('Origin',(26.8550245390365,0.,0.));
#71383=CARTESIAN_POINT('',(33.0966075166785,33.6734706547313,-17.5466166428447));
#71384=CARTESIAN_POINT('Origin',(17.5,35.7083195898645,-12.9967654463754));
#71385=CARTESIAN_POINT('',(33.1,36.2726528263519,-11.4462726220787));
#71386=CARTESIAN_POINT('',(33.1,36.2726528263519,-11.4462726220787));
#71387=CARTESIAN_POINT('',(30.5,36.2726528263519,-11.4462726220787));
#71388=CARTESIAN_POINT('',(30.5,36.2726528263519,-11.4462726220787));
#71389=CARTESIAN_POINT('',(30.5,36.101642754689,-11.9161189324716));
#71390=CARTESIAN_POINT('',(30.5,36.101642754689,-11.9161189324716));
#71391=CARTESIAN_POINT('',(24.1,35.9648346973588,-12.291995980786));
#71392=CARTESIAN_POINT('',(24.1,35.9648346973588,-12.291995980786));
#71393=CARTESIAN_POINT('',(23.1,36.0674407403565,-12.0100881945502));
#71394=CARTESIAN_POINT('',(23.1,36.0674407403565,-12.0100881945502));
#71395=CARTESIAN_POINT('',(22.4,36.2042487976867,-11.6342111462359));
#71396=CARTESIAN_POINT('',(22.4,36.2042487976867,-11.6342111462359));
#71397=CARTESIAN_POINT('',(21.8,36.2726528263519,-11.4462726220787));
#71398=CARTESIAN_POINT('',(21.8,36.2726528263519,-11.4462726220787));
#71399=CARTESIAN_POINT('',(13.2,36.2726528263519,-11.4462726220787));
#71400=CARTESIAN_POINT('',(13.2,36.2726528263519,-11.4462726220787));
#71401=CARTESIAN_POINT('',(12.6,36.2042487976867,-11.6342111462359));
#71402=CARTESIAN_POINT('',(12.6,36.2042487976867,-11.6342111462359));
#71403=CARTESIAN_POINT('',(11.9,36.0674407403565,-12.0100881945502));
#71404=CARTESIAN_POINT('',(11.9,36.0674407403565,-12.0100881945502));
#71405=CARTESIAN_POINT('',(10.9,35.9648346973588,-12.291995980786));
#71406=CARTESIAN_POINT('',(10.9,35.9648346973588,-12.291995980786));
#71407=CARTESIAN_POINT('',(4.5,36.101642754689,-11.9161189324716));
#71408=CARTESIAN_POINT('',(4.5,36.101642754689,-11.9161189324716));
#71409=CARTESIAN_POINT('',(4.5,36.2726528263519,-11.4462726220787));
#71410=CARTESIAN_POINT('',(4.5,36.2726528263519,-11.4462726220787));
#71411=CARTESIAN_POINT('',(1.9,36.2726528263519,-11.4462726220787));
#71412=CARTESIAN_POINT('',(1.9,36.2726528263519,-11.4462726220787));
#71413=CARTESIAN_POINT('',(1.57538060255633,36.1762351867803,-11.7111779096387));
#71414=CARTESIAN_POINT('',(0.,35.7083195898645,-12.9967654463754));
#71415=CARTESIAN_POINT('',(1.57538060255633,35.2404039929487,-14.2823529831122));
#71416=CARTESIAN_POINT('Ctrl Pts',(1.57538060255633,36.1762351867803,-11.7111779096387));
#71417=CARTESIAN_POINT('Ctrl Pts',(1.62460345738085,35.7083195898538,-12.9967654464047));
#71418=CARTESIAN_POINT('Ctrl Pts',(1.57538060255633,35.2404039929487,-14.2823529831122));
#71419=CARTESIAN_POINT('',(1.9,35.1439863533772,-14.5472582706722));
#71420=CARTESIAN_POINT('',(1.9,35.1439863533772,-14.5472582706722));
#71421=CARTESIAN_POINT('',(4.5,35.1439863533772,-14.5472582706722));
#71422=CARTESIAN_POINT('',(4.5,35.1439863533772,-14.5472582706722));
#71423=CARTESIAN_POINT('',(4.5,35.31499642504,-14.0774119602792));
#71424=CARTESIAN_POINT('',(4.5,35.31499642504,-14.0774119602792));
#71425=CARTESIAN_POINT('',(10.9,35.4518044823703,-13.7015349119649));
#71426=CARTESIAN_POINT('',(10.9,35.4518044823703,-13.7015349119649));
#71427=CARTESIAN_POINT('',(11.9,35.3491984393726,-13.9834426982006));
#71428=CARTESIAN_POINT('',(11.9,35.3491984393726,-13.9834426982006));
#71429=CARTESIAN_POINT('',(12.6,35.2123903820423,-14.359319746515));
#71430=CARTESIAN_POINT('',(12.6,35.2123903820423,-14.359319746515));
#71431=CARTESIAN_POINT('',(13.2,35.1439863533772,-14.5472582706722));
#71432=CARTESIAN_POINT('',(13.2,35.1439863533772,-14.5472582706722));
#71433=CARTESIAN_POINT('',(21.8,35.1439863533772,-14.5472582706722));
#71434=CARTESIAN_POINT('',(21.8,35.1439863533772,-14.5472582706722));
#71435=CARTESIAN_POINT('',(22.4,35.2123903820423,-14.359319746515));
#71436=CARTESIAN_POINT('',(22.4,35.2123903820423,-14.359319746515));
#71437=CARTESIAN_POINT('',(23.1,35.3491984393726,-13.9834426982006));
#71438=CARTESIAN_POINT('',(23.1,35.3491984393726,-13.9834426982006));
#71439=CARTESIAN_POINT('',(24.1,35.4518044823703,-13.7015349119649));
#71440=CARTESIAN_POINT('',(24.1,35.4518044823703,-13.7015349119649));
#71441=CARTESIAN_POINT('',(30.5,35.31499642504,-14.0774119602792));
#71442=CARTESIAN_POINT('',(30.5,35.31499642504,-14.0774119602792));
#71443=CARTESIAN_POINT('',(30.5,35.1439863533772,-14.5472582706722));
#71444=CARTESIAN_POINT('',(30.5,35.1439863533772,-14.5472582706722));
#71445=CARTESIAN_POINT('',(33.1,35.1439863533772,-14.5472582706722));
#71446=CARTESIAN_POINT('',(33.1,35.1439863533772,-14.5472582706722));
#71447=CARTESIAN_POINT('',(35.,35.7083195898645,-12.9967654463754));
#71448=CARTESIAN_POINT('Origin',(35.,35.7083195898645,-12.9967654463754));
#71449=CARTESIAN_POINT('',(35.,40.4742595624789,-13.790523889916));
#71450=CARTESIAN_POINT('',(35.,42.5812236707767,-14.1414348457417));
#71451=CARTESIAN_POINT('',(34.8617922858584,40.515309671231,-13.6777396430533));
#71452=CARTESIAN_POINT('',(33.5377160618333,40.9085834716836,-12.5972287566466));
#71453=CARTESIAN_POINT('',(34.4,40.1803643021789,-13.22226624086));
#71454=CARTESIAN_POINT('Ctrl Pts',(34.4,40.1803643021789,-13.22226624086));
#71455=CARTESIAN_POINT('Ctrl Pts',(34.6297825290978,40.3476538099254,-13.4490085829851));
#71456=CARTESIAN_POINT('Ctrl Pts',(34.8617922858584,40.515309671231,-13.6777396430533));
#71457=CARTESIAN_POINT('',(33.322645308031,40.4610861730024,-12.3365516130268));
#71458=CARTESIAN_POINT('Origin',(26.8550245390365,0.,0.));
#71459=CARTESIAN_POINT('',(33.0966075166785,36.2088329758586,-11.4327072940916));
#71460=CARTESIAN_POINT('Origin',(17.5,37.4226946144639,-6.59863075134336));
#71461=CARTESIAN_POINT('',(33.1,37.7092141076143,-4.97369795887321));
#71462=CARTESIAN_POINT('',(33.1,37.7092141076143,-4.97369795887321));
#71463=CARTESIAN_POINT('',(30.5,37.7092141076143,-4.97369795887321));
#71464=CARTESIAN_POINT('',(30.5,37.7092141076143,-4.97369795887321));
#71465=CARTESIAN_POINT('',(30.5,37.6223900187809,-5.46610183537932));
#71466=CARTESIAN_POINT('',(30.5,37.6223900187809,-5.46610183537932));
#71467=CARTESIAN_POINT('',(24.1,37.5529307477141,-5.8600249365842));
#71468=CARTESIAN_POINT('',(24.1,37.5529307477141,-5.8600249365842));
#71469=CARTESIAN_POINT('',(23.1,37.6050252010142,-5.56458261068054));
#71470=CARTESIAN_POINT('',(23.1,37.6050252010142,-5.56458261068054));
#71471=CARTESIAN_POINT('',(22.4,37.674484472081,-5.17065950947565));
#71472=CARTESIAN_POINT('',(22.4,37.674484472081,-5.17065950947565));
#71473=CARTESIAN_POINT('',(21.8,37.7092141076143,-4.97369795887321));
#71474=CARTESIAN_POINT('',(21.8,37.7092141076143,-4.97369795887321));
#71475=CARTESIAN_POINT('',(13.2,37.7092141076143,-4.97369795887321));
#71476=CARTESIAN_POINT('',(13.2,37.7092141076143,-4.97369795887321));
#71477=CARTESIAN_POINT('',(12.6,37.674484472081,-5.17065950947565));
#71478=CARTESIAN_POINT('',(12.6,37.674484472081,-5.17065950947565));
#71479=CARTESIAN_POINT('',(11.9,37.6050252010142,-5.56458261068054));
#71480=CARTESIAN_POINT('',(11.9,37.6050252010142,-5.56458261068054));
#71481=CARTESIAN_POINT('',(10.9,37.5529307477141,-5.8600249365842));
#71482=CARTESIAN_POINT('',(10.9,37.5529307477141,-5.8600249365842));
#71483=CARTESIAN_POINT('',(4.5,37.6223900187809,-5.46610183537932));
#71484=CARTESIAN_POINT('',(4.5,37.6223900187809,-5.46610183537932));
#71485=CARTESIAN_POINT('',(4.5,37.7092141076143,-4.97369795887321));
#71486=CARTESIAN_POINT('',(4.5,37.7092141076143,-4.97369795887321));
#71487=CARTESIAN_POINT('',(1.9,37.7092141076143,-4.97369795887321));
#71488=CARTESIAN_POINT('',(1.9,37.7092141076143,-4.97369795887321));
#71489=CARTESIAN_POINT('',(1.57538060255632,37.6602615890763,-5.25132148728275));
#71490=CARTESIAN_POINT('',(0.,37.4226946144639,-6.59863075134336));
#71491=CARTESIAN_POINT('',(1.57538060255632,37.1851276398516,-7.94594001540395));
#71492=CARTESIAN_POINT('Ctrl Pts',(1.57538060255632,37.6602615890763,-5.25132148728275));
#71493=CARTESIAN_POINT('Ctrl Pts',(1.62460345738085,37.4226946144585,-6.59863075137406));
#71494=CARTESIAN_POINT('Ctrl Pts',(1.57538060255632,37.1851276398516,-7.94594001540395));
#71495=CARTESIAN_POINT('',(1.9,37.1361751213135,-8.2235635438135));
#71496=CARTESIAN_POINT('',(1.9,37.1361751213135,-8.2235635438135));
#71497=CARTESIAN_POINT('',(4.5,37.1361751213135,-8.2235635438135));
#71498=CARTESIAN_POINT('',(4.5,37.1361751213135,-8.2235635438135));
#71499=CARTESIAN_POINT('',(4.5,37.2229992101469,-7.7311596673074));
#71500=CARTESIAN_POINT('',(4.5,37.2229992101469,-7.7311596673074));
#71501=CARTESIAN_POINT('',(10.9,37.2924584812137,-7.33723656610251));
#71502=CARTESIAN_POINT('',(10.9,37.2924584812137,-7.33723656610251));
#71503=CARTESIAN_POINT('',(11.9,37.2403640279136,-7.63267889200617));
#71504=CARTESIAN_POINT('',(11.9,37.2403640279136,-7.63267889200617));
#71505=CARTESIAN_POINT('',(12.6,37.1709047568469,-8.02660199321106));
#71506=CARTESIAN_POINT('',(12.6,37.1709047568469,-8.02660199321106));
#71507=CARTESIAN_POINT('',(13.2,37.1361751213135,-8.2235635438135));
#71508=CARTESIAN_POINT('',(13.2,37.1361751213135,-8.2235635438135));
#71509=CARTESIAN_POINT('',(21.8,37.1361751213135,-8.2235635438135));
#71510=CARTESIAN_POINT('',(21.8,37.1361751213135,-8.2235635438135));
#71511=CARTESIAN_POINT('',(22.4,37.1709047568469,-8.02660199321106));
#71512=CARTESIAN_POINT('',(22.4,37.1709047568469,-8.02660199321106));
#71513=CARTESIAN_POINT('',(23.1,37.2403640279136,-7.63267889200617));
#71514=CARTESIAN_POINT('',(23.1,37.2403640279136,-7.63267889200617));
#71515=CARTESIAN_POINT('',(24.1,37.2924584812137,-7.33723656610251));
#71516=CARTESIAN_POINT('',(24.1,37.2924584812137,-7.33723656610251));
#71517=CARTESIAN_POINT('',(30.5,37.2229992101469,-7.7311596673074));
#71518=CARTESIAN_POINT('',(30.5,37.2229992101469,-7.7311596673074));
#71519=CARTESIAN_POINT('',(30.5,37.1361751213135,-8.2235635438135));
#71520=CARTESIAN_POINT('',(30.5,37.1361751213135,-8.2235635438135));
#71521=CARTESIAN_POINT('',(33.1,37.1361751213135,-8.2235635438135));
#71522=CARTESIAN_POINT('',(33.1,37.1361751213135,-8.2235635438135));
#71523=CARTESIAN_POINT('',(35.,37.4226946144639,-6.59863075134336));
#71524=CARTESIAN_POINT('Origin',(35.,37.4226946144639,-6.59863075134336));
#71525=CARTESIAN_POINT('',(35.,42.2540639571139,-6.55273342944653));
#71526=CARTESIAN_POINT('',(35.,44.7420297840206,-6.52909810779604));
#71527=CARTESIAN_POINT('',(34.8617922858584,42.2749056435377,-6.4345343521407));
#71528=CARTESIAN_POINT('',(33.5377160618333,42.4745759849063,-5.30214757522046));
#71529=CARTESIAN_POINT('',(34.4,41.8659567209931,-6.04414326732376));
#71530=CARTESIAN_POINT('Ctrl Pts',(34.4,41.8659567209931,-6.04414326732376));
#71531=CARTESIAN_POINT('Ctrl Pts',(34.6297825290999,42.0700781197312,-6.23839136562344));
#71532=CARTESIAN_POINT('Ctrl Pts',(34.8617922858584,42.2749056435377,-6.4345343521407));
#71533=CARTESIAN_POINT('',(33.3226453080309,41.9886110647639,-5.12313779357752));
#71534=CARTESIAN_POINT('Origin',(26.8550245390365,0.,0.));
#71535=CARTESIAN_POINT('',(33.0966075166785,37.6440082295681,-4.97142091943645));
#71536=CARTESIAN_POINT('Origin',(0.8,0.,0.));
#71537=CARTESIAN_POINT('',(0.,38.9456055698919,-7.1693658572013));
#71538=CARTESIAN_POINT('',(2.77555756156289E-16,39.0489657041001,-6.5831814071929));
#71539=CARTESIAN_POINT('Origin',(0.,0.,0.));
#71540=CARTESIAN_POINT('Ctrl Pts',(1.57538060255632,37.1851276398516,-7.94594001540395));
#71541=CARTESIAN_POINT('Ctrl Pts',(0.801841055748964,38.0570140694246,-7.56742453339957));
#71542=CARTESIAN_POINT('Ctrl Pts',(-5.55111512312578E-16,38.9456055698919,
-7.1693658572013));
#71543=CARTESIAN_POINT('Ctrl Pts',(-1.38777878078145E-16,39.0489657041001,
-6.5831814071929));
#71544=CARTESIAN_POINT('Ctrl Pts',(0.801841055750455,38.350106913702,-5.90521241418052));
#71545=CARTESIAN_POINT('Ctrl Pts',(1.57538060255632,37.6602615890763,-5.25132148728275));
#71546=CARTESIAN_POINT('Origin',(0.8,0.,0.));
#71547=CARTESIAN_POINT('',(-1.38777878078145E-16,37.1089869948545,-13.8232805156997));
#71548=CARTESIAN_POINT('',(2.77555756156289E-16,37.3125667178958,-13.2639498235849));
#71549=CARTESIAN_POINT('Origin',(0.,0.,0.));
#71550=CARTESIAN_POINT('Ctrl Pts',(1.57538060255633,35.2404039929487,-14.2823529831122));
#71551=CARTESIAN_POINT('Ctrl Pts',(0.801841055749845,36.1647730322062,-14.0609894914273));
#71552=CARTESIAN_POINT('Ctrl Pts',(-2.77555756156289E-16,37.1089869948545,
-13.8232805156997));
#71553=CARTESIAN_POINT('Ctrl Pts',(9.71445146547012E-16,37.3125667178958,
-13.2639498235849));
#71554=CARTESIAN_POINT('Ctrl Pts',(0.801841055750823,36.742053243002,-12.4749251475649));
#71555=CARTESIAN_POINT('Ctrl Pts',(1.57538060255633,36.1762351867803,-11.7111779096387));
#71556=CARTESIAN_POINT('Origin',(0.8,0.,0.));
#71557=CARTESIAN_POINT('',(-6.93889390390723E-16,34.1448306280318,-20.0571817906459));
#71558=CARTESIAN_POINT('',(-5.55111512312578E-16,34.4424442730379,-19.5416998364696));
#71559=CARTESIAN_POINT('Origin',(0.,0.,0.));
#71560=CARTESIAN_POINT('Ctrl Pts',(1.57538060255632,32.224918503225,-20.1848038826479));
#71561=CARTESIAN_POINT('Ctrl Pts',(0.801841055749468,33.1736836666637,-20.1273183989615));
#71562=CARTESIAN_POINT('Ctrl Pts',(-1.11022302462516E-15,34.1448306280318,
-20.0571817906459));
#71563=CARTESIAN_POINT('Ctrl Pts',(-8.32667268468867E-16,34.4424442730379,
-19.5416998364696));
#71564=CARTESIAN_POINT('Ctrl Pts',(0.801841055749988,34.0176108768901,-18.6655935929584));
#71565=CARTESIAN_POINT('Ctrl Pts',(1.57538060255633,33.5930121843923,-17.8151961173521));
#71566=CARTESIAN_POINT('Origin',(0.8,0.,0.));
#71567=CARTESIAN_POINT('',(2.77555756156289E-16,30.1432008606945,-25.6816557463071));
#71568=CARTESIAN_POINT('',(-4.16333634234434E-16,30.5258055876616,-25.2256851884005));
#71569=CARTESIAN_POINT('Origin',(0.,0.,0.));
#71570=CARTESIAN_POINT('Ctrl Pts',(1.57538060255632,28.2302951713763,-25.4739497302129));
#71571=CARTESIAN_POINT('Ctrl Pts',(0.801841055749793,29.1746287096027,-25.5820889218578));
#71572=CARTESIAN_POINT('Ctrl Pts',(-1.11022302462516E-15,30.1432008606945,
-25.6816557463071));
#71573=CARTESIAN_POINT('Ctrl Pts',(-1.38777878078145E-16,30.5258055876616,
-25.2256851884005));
#71574=CARTESIAN_POINT('Ctrl Pts',(0.801841055749945,30.2595606180251,-24.2891174222752));
#71575=CARTESIAN_POINT('Ctrl Pts',(1.57538060255632,29.989082505666,-23.3779086059641));
#71576=CARTESIAN_POINT('Origin',(0.8,0.,0.));
#71577=CARTESIAN_POINT('',(-4.16333634234434E-16,25.2256851884005,-30.5258055876616));
#71578=CARTESIAN_POINT('',(4.16333634234434E-16,25.6816557463071,-30.1432008606945));
#71579=CARTESIAN_POINT('Origin',(0.,0.,0.));
#71580=CARTESIAN_POINT('Ctrl Pts',(1.57538060255632,23.3779086059641,-29.989082505666));
#71581=CARTESIAN_POINT('Ctrl Pts',(0.801841055749821,24.2891174222753,-30.2595606180251));
#71582=CARTESIAN_POINT('Ctrl Pts',(-2.77555756156289E-16,25.2256851884005,
-30.5258055876616));
#71583=CARTESIAN_POINT('Ctrl Pts',(6.93889390390723E-16,25.6816557463071,
-30.1432008606945));
#71584=CARTESIAN_POINT('Ctrl Pts',(0.80184105574966,25.5820889218578,-29.1746287096029));
#71585=CARTESIAN_POINT('Ctrl Pts',(1.57538060255632,25.4739497302129,-28.2302951713764));
#71586=CARTESIAN_POINT('Origin',(0.8,0.,0.));
#71587=CARTESIAN_POINT('',(-2.77555756156289E-16,19.5416998364696,-34.4424442730379));
#71588=CARTESIAN_POINT('',(1.38777878078145E-16,20.0571817906459,-34.1448306280319));
#71589=CARTESIAN_POINT('Origin',(0.,0.,0.));
#71590=CARTESIAN_POINT('Ctrl Pts',(1.57538060255632,17.8151961173521,-33.5930121843923));
#71591=CARTESIAN_POINT('Ctrl Pts',(0.801841055750877,18.6655935929574,-34.0176108768897));
#71592=CARTESIAN_POINT('Ctrl Pts',(-2.77555756156289E-16,19.5416998364696,
-34.4424442730379));
#71593=CARTESIAN_POINT('Ctrl Pts',(1.38777878078145E-16,20.0571817906459,
-34.1448306280319));
#71594=CARTESIAN_POINT('Ctrl Pts',(0.801841055749399,20.1273183989615,-33.1736836666638));
#71595=CARTESIAN_POINT('Ctrl Pts',(1.57538060255632,20.1848038826479,-32.224918503225));
#71596=CARTESIAN_POINT('Origin',(0.8,0.,0.));
#71597=CARTESIAN_POINT('',(-1.38777878078145E-16,13.2639498235848,-37.3125667178958));
#71598=CARTESIAN_POINT('',(-2.77555756156289E-16,13.8232805156996,-37.1089869948545));
#71599=CARTESIAN_POINT('Origin',(0.,0.,0.));
#71600=CARTESIAN_POINT('Ctrl Pts',(1.57538060255632,11.7111779096386,-36.1762351867803));
#71601=CARTESIAN_POINT('Ctrl Pts',(0.801841055749469,12.4749251475662,-36.7420532430029));
#71602=CARTESIAN_POINT('Ctrl Pts',(1.38777878078145E-16,13.2639498235848,
-37.3125667178958));
#71603=CARTESIAN_POINT('Ctrl Pts',(4.16333634234434E-16,13.8232805156996,
-37.1089869948545));
#71604=CARTESIAN_POINT('Ctrl Pts',(0.801841055749681,14.0609894914272,-36.1647730322064));
#71605=CARTESIAN_POINT('Ctrl Pts',(1.57538060255632,14.2823529831122,-35.2404039929487));
#71606=CARTESIAN_POINT('Origin',(0.8,0.,0.));
#71607=CARTESIAN_POINT('',(1.38777878078145E-16,6.58318140719289,-39.0489657041002));
#71608=CARTESIAN_POINT('',(1.38777878078145E-16,7.16936585720128,-38.9456055698919));
#71609=CARTESIAN_POINT('Origin',(0.,0.,0.));
#71610=CARTESIAN_POINT('Ctrl Pts',(1.57538060255633,5.25132148728273,-37.6602615890763));
#71611=CARTESIAN_POINT('Ctrl Pts',(0.801841055749878,5.90521241418099,-38.3501069137025));
#71612=CARTESIAN_POINT('Ctrl Pts',(1.38777878078145E-16,6.58318140719289,
-39.0489657041002));
#71613=CARTESIAN_POINT('Ctrl Pts',(0.,7.16936585720128,-38.9456055698919));
#71614=CARTESIAN_POINT('Ctrl Pts',(0.80184105575087,7.5674245334005,-38.0570140694225));
#71615=CARTESIAN_POINT('Ctrl Pts',(1.57538060255632,7.94594001540394,-37.1851276398516));
#71616=CARTESIAN_POINT('Origin',(0.8,0.,0.));
#71617=CARTESIAN_POINT('',(-2.77555756156289E-16,-0.297613645006075,-39.5988816271155));
#71618=CARTESIAN_POINT('',(-2.77555756156289E-16,0.297613645006066,-39.5988816271155));
#71619=CARTESIAN_POINT('Origin',(0.,0.,0.));
#71620=CARTESIAN_POINT('Ctrl Pts',(1.57538060255632,-1.36809368116734,-38.));
#71621=CARTESIAN_POINT('Ctrl Pts',(0.801841055749771,-0.843927210226931,
-38.7929119919201));
#71622=CARTESIAN_POINT('Ctrl Pts',(-4.16333634234434E-16,-0.297613645006074,
-39.5988816271155));
#71623=CARTESIAN_POINT('Ctrl Pts',(-1.38777878078145E-16,0.29761364500606,
-39.5988816271155));
#71624=CARTESIAN_POINT('Ctrl Pts',(0.801841055750365,0.843927210227319,
-38.7929119919195));
#71625=CARTESIAN_POINT('Ctrl Pts',(1.57538060255632,1.36809368116733,-38.));
#71626=CARTESIAN_POINT('Origin',(0.8,0.,0.));
#71627=CARTESIAN_POINT('',(6.93889390390723E-16,-7.16936585720129,-38.9456055698919));
#71628=CARTESIAN_POINT('',(-2.77555756156289E-16,-6.5831814071929,-39.0489657041002));
#71629=CARTESIAN_POINT('Origin',(0.,0.,0.));
#71630=CARTESIAN_POINT('Ctrl Pts',(1.57538060255633,-7.94594001540395,-37.1851276398516));
#71631=CARTESIAN_POINT('Ctrl Pts',(0.80184105574994,-7.56742453340005,-38.0570140694235));
#71632=CARTESIAN_POINT('Ctrl Pts',(-2.77555756156289E-16,-7.16936585720129,
-38.9456055698919));
#71633=CARTESIAN_POINT('Ctrl Pts',(-2.77555756156289E-16,-6.5831814071929,
-39.0489657041001));
#71634=CARTESIAN_POINT('Ctrl Pts',(0.80184105575081,-5.90521241418022,-38.3501069137017));
#71635=CARTESIAN_POINT('Ctrl Pts',(1.57538060255632,-5.25132148728275,-37.6602615890763));
#71636=CARTESIAN_POINT('Origin',(0.8,0.,0.));
#71637=CARTESIAN_POINT('',(1.38777878078145E-16,-13.8232805156997,-37.1089869948545));
#71638=CARTESIAN_POINT('',(1.38777878078145E-16,-13.2639498235849,-37.3125667178958));
#71639=CARTESIAN_POINT('Origin',(0.,0.,0.));
#71640=CARTESIAN_POINT('Ctrl Pts',(1.57538060255632,-14.2823529831122,-35.2404039929487));
#71641=CARTESIAN_POINT('Ctrl Pts',(0.801841055750031,-14.0609894914273,
-36.1647730322059));
#71642=CARTESIAN_POINT('Ctrl Pts',(-1.38777878078145E-16,-13.8232805156997,
-37.1089869948545));
#71643=CARTESIAN_POINT('Ctrl Pts',(9.71445146547012E-16,-13.2639498235849,
-37.3125667178958));
#71644=CARTESIAN_POINT('Ctrl Pts',(0.801841055748983,-12.4749251475667,
-36.7420532430033));
#71645=CARTESIAN_POINT('Ctrl Pts',(1.57538060255632,-11.7111779096387,-36.1762351867803));
#71646=CARTESIAN_POINT('Origin',(0.8,0.,0.));
#71647=CARTESIAN_POINT('',(-1.2490009027033E-15,-20.0571817906459,-34.1448306280318));
#71648=CARTESIAN_POINT('',(-6.93889390390723E-16,-19.5416998364696,-34.4424442730379));
#71649=CARTESIAN_POINT('Origin',(0.,0.,0.));
#71650=CARTESIAN_POINT('Ctrl Pts',(1.57538060255632,-20.1848038826479,-32.224918503225));
#71651=CARTESIAN_POINT('Ctrl Pts',(0.801841055749729,-20.1273183989615,
-33.1736836666634));
#71652=CARTESIAN_POINT('Ctrl Pts',(-6.93889390390723E-16,-20.0571817906459,
-34.1448306280318));
#71653=CARTESIAN_POINT('Ctrl Pts',(-5.55111512312578E-16,-19.5416998364696,
-34.4424442730379));
#71654=CARTESIAN_POINT('Ctrl Pts',(0.801841055748299,-18.6655935929602,
-34.017610876891));
#71655=CARTESIAN_POINT('Ctrl Pts',(1.57538060255633,-17.8151961173521,-33.5930121843923));
#71656=CARTESIAN_POINT('Origin',(0.8,0.,0.));
#71657=CARTESIAN_POINT('',(1.2490009027033E-15,-25.6816557463071,-30.1432008606945));
#71658=CARTESIAN_POINT('',(-4.16333634234434E-16,-25.2256851884005,-30.5258055876616));
#71659=CARTESIAN_POINT('Origin',(0.,0.,0.));
#71660=CARTESIAN_POINT('Ctrl Pts',(1.57538060255632,-25.4739497302129,-28.2302951713763));
#71661=CARTESIAN_POINT('Ctrl Pts',(0.801841055750148,-25.5820889218578,
-29.1746287096023));
#71662=CARTESIAN_POINT('Ctrl Pts',(2.77555756156289E-16,-25.6816557463071,
-30.1432008606945));
#71663=CARTESIAN_POINT('Ctrl Pts',(1.38777878078145E-16,-25.2256851884005,
-30.5258055876616));
#71664=CARTESIAN_POINT('Ctrl Pts',(0.801841055749258,-24.289117422276,-30.2595606180253));
#71665=CARTESIAN_POINT('Ctrl Pts',(1.57538060255632,-23.3779086059641,-29.989082505666));
#71666=CARTESIAN_POINT('Origin',(0.8,0.,0.));
#71667=CARTESIAN_POINT('',(-4.16333634234434E-16,-30.5258055876616,-25.2256851884005));
#71668=CARTESIAN_POINT('',(1.2490009027033E-15,-30.1432008606945,-25.6816557463071));
#71669=CARTESIAN_POINT('Origin',(0.,0.,0.));
#71670=CARTESIAN_POINT('Ctrl Pts',(1.57538060255632,-29.989082505666,-23.3779086059641));
#71671=CARTESIAN_POINT('Ctrl Pts',(0.801841055748062,-30.2595606180257,
-24.2891174222774));
#71672=CARTESIAN_POINT('Ctrl Pts',(-1.11022302462516E-15,-30.5258055876616,
-25.2256851884005));
#71673=CARTESIAN_POINT('Ctrl Pts',(6.93889390390723E-16,-30.1432008606945,
-25.6816557463071));
#71674=CARTESIAN_POINT('Ctrl Pts',(0.801841055750156,-29.1746287096023,
-25.5820889218578));
#71675=CARTESIAN_POINT('Ctrl Pts',(1.57538060255632,-28.2302951713764,-25.4739497302129));
#71676=CARTESIAN_POINT('Origin',(0.8,0.,0.));
#71677=CARTESIAN_POINT('',(-9.71445146547012E-16,-34.4424442730379,-19.5416998364696));
#71678=CARTESIAN_POINT('',(-9.71445146547012E-16,-34.1448306280319,-20.0571817906459));
#71679=CARTESIAN_POINT('Origin',(0.,0.,0.));
#71680=CARTESIAN_POINT('Ctrl Pts',(1.57538060255633,-33.5930121843923,-17.8151961173521));
#71681=CARTESIAN_POINT('Ctrl Pts',(0.801841055749805,-34.0176108768902,
-18.6655935929586));
#71682=CARTESIAN_POINT('Ctrl Pts',(0.,-34.4424442730379,-19.5416998364696));
#71683=CARTESIAN_POINT('Ctrl Pts',(6.93889390390723E-16,-34.1448306280319,
-20.0571817906459));
#71684=CARTESIAN_POINT('Ctrl Pts',(0.801841055748204,-33.1736836666653,
-20.1273183989614));
#71685=CARTESIAN_POINT('Ctrl Pts',(1.57538060255633,-32.224918503225,-20.1848038826479));
#71686=CARTESIAN_POINT('Origin',(0.8,0.,0.));
#71687=CARTESIAN_POINT('',(-1.38777878078145E-16,-37.3125667178958,-13.2639498235848));
#71688=CARTESIAN_POINT('',(-4.16333634234434E-16,-37.1089869948545,-13.8232805156996));
#71689=CARTESIAN_POINT('Origin',(0.,0.,0.));
#71690=CARTESIAN_POINT('Ctrl Pts',(1.57538060255633,-36.1762351867803,-11.7111779096386));
#71691=CARTESIAN_POINT('Ctrl Pts',(0.801841055749638,-36.7420532430028,
-12.474925147566));
#71692=CARTESIAN_POINT('Ctrl Pts',(2.77555756156289E-16,-37.3125667178958,
-13.2639498235848));
#71693=CARTESIAN_POINT('Ctrl Pts',(-6.93889390390723E-16,-37.1089869948545,
-13.8232805156996));
#71694=CARTESIAN_POINT('Ctrl Pts',(0.801841055748945,-36.1647730322072,
-14.060989491427));
#71695=CARTESIAN_POINT('Ctrl Pts',(1.57538060255633,-35.2404039929487,-14.2823529831122));
#71696=CARTESIAN_POINT('Origin',(0.8,0.,0.));
#71697=CARTESIAN_POINT('',(0.,-39.0489657041002,-6.58318140719289));
#71698=CARTESIAN_POINT('',(-1.38777878078145E-16,-38.9456055698919,-7.16936585720128));
#71699=CARTESIAN_POINT('Origin',(0.,0.,0.));
#71700=CARTESIAN_POINT('Ctrl Pts',(1.57538060255633,-37.6602615890763,-5.25132148728274));
#71701=CARTESIAN_POINT('Ctrl Pts',(0.801841055749013,-38.3501069137033,
-5.90521241418173));
#71702=CARTESIAN_POINT('Ctrl Pts',(-5.55111512312578E-16,-39.0489657041002,
-6.58318140719289));
#71703=CARTESIAN_POINT('Ctrl Pts',(2.77555756156289E-16,-38.9456055698919,
-7.16936585720128));
#71704=CARTESIAN_POINT('Ctrl Pts',(0.801841055749582,-38.0570140694239,
-7.56742453339987));
#71705=CARTESIAN_POINT('Ctrl Pts',(1.57538060255632,-37.1851276398516,-7.94594001540395));
#71706=CARTESIAN_POINT('Origin',(0.8,0.,0.));
#71707=CARTESIAN_POINT('',(0.,-39.5988816271155,0.297613645006073));
#71708=CARTESIAN_POINT('',(1.38777878078145E-16,-39.5988816271155,-0.29761364500606));
#71709=CARTESIAN_POINT('Origin',(0.,0.,0.));
#71710=CARTESIAN_POINT('Ctrl Pts',(1.57538060255633,-38.,1.36809368116734));
#71711=CARTESIAN_POINT('Ctrl Pts',(0.801841055749649,-38.7929119919202,
0.843927210226842));
#71712=CARTESIAN_POINT('Ctrl Pts',(-1.38777878078145E-16,-39.5988816271155,
0.29761364500607));
#71713=CARTESIAN_POINT('Ctrl Pts',(-1.38777878078145E-16,-39.5988816271155,
-0.297613645006064));
#71714=CARTESIAN_POINT('Ctrl Pts',(0.801841055749106,-38.7929119919208,
-0.843927210226466));
#71715=CARTESIAN_POINT('Ctrl Pts',(1.57538060255632,-38.,-1.36809368116733));
#71716=CARTESIAN_POINT('Origin',(0.8,0.,0.));
#71717=CARTESIAN_POINT('',(-1.38777878078145E-16,-38.9456055698919,7.16936585720131));
#71718=CARTESIAN_POINT('',(2.77555756156289E-16,-39.0489657041001,6.58318140719291));
#71719=CARTESIAN_POINT('Origin',(0.,0.,0.));
#71720=CARTESIAN_POINT('Ctrl Pts',(1.57538060255632,-37.1851276398516,7.94594001540397));
#71721=CARTESIAN_POINT('Ctrl Pts',(0.801841055749284,-38.0570140694243,
7.56742453339975));
#71722=CARTESIAN_POINT('Ctrl Pts',(0.,-38.9456055698919,7.16936585720131));
#71723=CARTESIAN_POINT('Ctrl Pts',(0.,-39.0489657041001,6.58318140719291));
#71724=CARTESIAN_POINT('Ctrl Pts',(0.80184105575133,-38.3501069137012,5.90521241417979));
#71725=CARTESIAN_POINT('Ctrl Pts',(1.57538060255632,-37.6602615890763,5.25132148728276));
#71726=CARTESIAN_POINT('Origin',(0.8,0.,0.));
#71727=CARTESIAN_POINT('',(1.38777878078145E-16,-37.1089869948545,13.8232805156996));
#71728=CARTESIAN_POINT('',(1.38777878078145E-16,-37.3125667178958,13.2639498235848));
#71729=CARTESIAN_POINT('Origin',(0.,0.,0.));
#71730=CARTESIAN_POINT('Ctrl Pts',(1.57538060255633,-35.2404039929487,14.2823529831122));
#71731=CARTESIAN_POINT('Ctrl Pts',(0.8018410557497,-36.1647730322063,14.0609894914272));
#71732=CARTESIAN_POINT('Ctrl Pts',(1.38777878078145E-16,-37.1089869948545,
13.8232805156996));
#71733=CARTESIAN_POINT('Ctrl Pts',(9.71445146547012E-16,-37.3125667178958,
13.2639498235848));
#71734=CARTESIAN_POINT('Ctrl Pts',(0.801841055750097,-36.7420532430025,
12.4749251475656));
#71735=CARTESIAN_POINT('Ctrl Pts',(1.57538060255632,-36.1762351867803,11.7111779096386));
#71736=CARTESIAN_POINT('Origin',(0.8,0.,0.));
#71737=CARTESIAN_POINT('',(1.52655665885959E-15,-34.1448306280319,20.0571817906459));
#71738=CARTESIAN_POINT('',(-4.16333634234434E-16,-34.4424442730379,19.5416998364696));
#71739=CARTESIAN_POINT('Origin',(0.,0.,0.));
#71740=CARTESIAN_POINT('Ctrl Pts',(1.57538060255632,-32.224918503225,20.1848038826479));
#71741=CARTESIAN_POINT('Ctrl Pts',(0.801841055750799,-33.1736836666621,
20.1273183989616));
#71742=CARTESIAN_POINT('Ctrl Pts',(6.93889390390723E-16,-34.1448306280319,
20.0571817906459));
#71743=CARTESIAN_POINT('Ctrl Pts',(-2.77555756156289E-16,-34.4424442730379,
19.5416998364696));
#71744=CARTESIAN_POINT('Ctrl Pts',(0.801841055749465,-34.0176108768904,
18.6655935929589));
#71745=CARTESIAN_POINT('Ctrl Pts',(1.57538060255632,-33.5930121843923,17.8151961173521));
#71746=CARTESIAN_POINT('Origin',(0.8,0.,0.));
#71747=CARTESIAN_POINT('',(1.2490009027033E-15,-30.1432008606945,25.6816557463071));
#71748=CARTESIAN_POINT('',(-1.38777878078145E-16,-30.5258055876616,25.2256851884005));
#71749=CARTESIAN_POINT('Origin',(0.,0.,0.));
#71750=CARTESIAN_POINT('Ctrl Pts',(1.57538060255632,-28.2302951713763,25.4739497302129));
#71751=CARTESIAN_POINT('Ctrl Pts',(0.801841055750152,-29.1746287096023,
25.5820889218578));
#71752=CARTESIAN_POINT('Ctrl Pts',(1.38777878078145E-16,-30.1432008606945,
25.6816557463071));
#71753=CARTESIAN_POINT('Ctrl Pts',(1.38777878078145E-16,-30.5258055876616,
25.2256851884005));
#71754=CARTESIAN_POINT('Ctrl Pts',(0.80184105574948,-30.2595606180252,24.2891174222757));
#71755=CARTESIAN_POINT('Ctrl Pts',(1.57538060255632,-29.989082505666,23.3779086059641));
#71756=CARTESIAN_POINT('Origin',(0.8,0.,0.));
#71757=CARTESIAN_POINT('',(2.77555756156289E-16,-25.2256851884005,30.5258055876616));
#71758=CARTESIAN_POINT('',(-6.93889390390723E-16,-25.6816557463071,30.1432008606945));
#71759=CARTESIAN_POINT('Origin',(0.,0.,0.));
#71760=CARTESIAN_POINT('Ctrl Pts',(1.57538060255632,-23.3779086059641,29.989082505666));
#71761=CARTESIAN_POINT('Ctrl Pts',(0.801841055750737,-24.2891174222742,
30.2595606180248));
#71762=CARTESIAN_POINT('Ctrl Pts',(-1.52655665885959E-15,-25.2256851884005,
30.5258055876616));
#71763=CARTESIAN_POINT('Ctrl Pts',(1.38777878078145E-16,-25.6816557463071,
30.1432008606945));
#71764=CARTESIAN_POINT('Ctrl Pts',(0.801841055749893,-25.5820889218578,
29.1746287096026));
#71765=CARTESIAN_POINT('Ctrl Pts',(1.57538060255633,-25.4739497302129,28.2302951713764));
#71766=CARTESIAN_POINT('Origin',(0.8,0.,0.));
#71767=CARTESIAN_POINT('',(0.,-19.5416998364696,34.4424442730379));
#71768=CARTESIAN_POINT('',(2.08166817117217E-15,-20.0571817906459,34.1448306280319));
#71769=CARTESIAN_POINT('Origin',(0.,0.,0.));
#71770=CARTESIAN_POINT('Ctrl Pts',(1.57538060255632,-17.8151961173521,33.5930121843923));
#71771=CARTESIAN_POINT('Ctrl Pts',(0.801841055749172,-18.6655935929592,
34.0176108768906));
#71772=CARTESIAN_POINT('Ctrl Pts',(1.38777878078145E-16,-19.5416998364696,
34.4424442730379));
#71773=CARTESIAN_POINT('Ctrl Pts',(8.32667268468867E-16,-20.0571817906459,
34.1448306280319));
#71774=CARTESIAN_POINT('Ctrl Pts',(0.801841055749073,-20.1273183989614,
33.1736836666642));
#71775=CARTESIAN_POINT('Ctrl Pts',(1.57538060255632,-20.1848038826479,32.224918503225));
#71776=CARTESIAN_POINT('Origin',(0.8,0.,0.));
#71777=CARTESIAN_POINT('',(4.16333634234434E-16,-13.2639498235848,37.3125667178958));
#71778=CARTESIAN_POINT('',(-1.38777878078145E-16,-13.8232805156996,37.1089869948545));
#71779=CARTESIAN_POINT('Origin',(0.,0.,0.));
#71780=CARTESIAN_POINT('Ctrl Pts',(1.57538060255632,-11.7111779096386,36.1762351867803));
#71781=CARTESIAN_POINT('Ctrl Pts',(0.801841055748783,-12.4749251475669,
36.7420532430035));
#71782=CARTESIAN_POINT('Ctrl Pts',(5.55111512312578E-16,-13.2639498235848,
37.3125667178958));
#71783=CARTESIAN_POINT('Ctrl Pts',(1.38777878078145E-16,-13.8232805156996,
37.1089869948545));
#71784=CARTESIAN_POINT('Ctrl Pts',(0.801841055750372,-14.0609894914274,
36.1647730322055));
#71785=CARTESIAN_POINT('Ctrl Pts',(1.57538060255632,-14.2823529831122,35.2404039929487));
#71786=CARTESIAN_POINT('Origin',(0.8,0.,0.));
#71787=CARTESIAN_POINT('',(1.38777878078145E-16,-6.5831814071929,39.0489657041001));
#71788=CARTESIAN_POINT('',(-5.55111512312578E-16,-7.16936585720129,38.9456055698919));
#71789=CARTESIAN_POINT('Origin',(0.,0.,0.));
#71790=CARTESIAN_POINT('Ctrl Pts',(1.57538060255632,-5.25132148728275,37.6602615890763));
#71791=CARTESIAN_POINT('Ctrl Pts',(0.801841055749745,-5.90521241418111,
38.3501069137026));
#71792=CARTESIAN_POINT('Ctrl Pts',(4.16333634234434E-16,-6.5831814071929,
39.0489657041001));
#71793=CARTESIAN_POINT('Ctrl Pts',(5.55111512312578E-16,-7.16936585720129,
38.9456055698919));
#71794=CARTESIAN_POINT('Ctrl Pts',(0.801841055751039,-7.5674245334006,38.0570140694223));
#71795=CARTESIAN_POINT('Ctrl Pts',(1.57538060255632,-7.94594001540396,37.1851276398516));
#71796=CARTESIAN_POINT('Origin',(0.8,0.,0.));
#71797=CARTESIAN_POINT('',(1.38777878078145E-16,0.297613645006065,39.5988816271155));
#71798=CARTESIAN_POINT('',(0.,-0.297613645006066,39.5988816271155));
#71799=CARTESIAN_POINT('Origin',(0.,0.,0.));
#71800=CARTESIAN_POINT('Ctrl Pts',(1.57538060255633,1.36809368116734,38.));
#71801=CARTESIAN_POINT('Ctrl Pts',(0.801841055749075,0.843927210226451,
38.7929119919208));
#71802=CARTESIAN_POINT('Ctrl Pts',(-2.77555756156289E-16,0.297613645006067,
39.5988816271155));
#71803=CARTESIAN_POINT('Ctrl Pts',(0.,-0.297613645006065,39.5988816271155));
#71804=CARTESIAN_POINT('Ctrl Pts',(0.801841055749647,-0.84392721022684,
38.7929119919202));
#71805=CARTESIAN_POINT('Ctrl Pts',(1.57538060255632,-1.36809368116733,38.));
#71806=CARTESIAN_POINT('Origin',(0.8,0.,0.));
#71807=CARTESIAN_POINT('',(1.38777878078145E-16,7.16936585720129,38.9456055698919));
#71808=CARTESIAN_POINT('',(-1.38777878078145E-16,6.5831814071929,39.0489657041002));
#71809=CARTESIAN_POINT('Origin',(0.,0.,0.));
#71810=CARTESIAN_POINT('Ctrl Pts',(1.57538060255632,7.94594001540395,37.1851276398516));
#71811=CARTESIAN_POINT('Ctrl Pts',(0.801841055750375,7.56742453340027,38.0570140694231));
#71812=CARTESIAN_POINT('Ctrl Pts',(-5.55111512312578E-16,7.1693658572013,
38.9456055698919));
#71813=CARTESIAN_POINT('Ctrl Pts',(0.,6.5831814071929,39.0489657041001));
#71814=CARTESIAN_POINT('Ctrl Pts',(0.801841055750716,5.9052124141803,38.3501069137018));
#71815=CARTESIAN_POINT('Ctrl Pts',(1.57538060255632,5.25132148728276,37.6602615890763));
#71816=CARTESIAN_POINT('Origin',(0.8,0.,0.));
#71817=CARTESIAN_POINT('',(-2.77555756156289E-16,13.8232805156996,37.1089869948545));
#71818=CARTESIAN_POINT('',(1.38777878078145E-16,13.2639498235848,37.3125667178958));
#71819=CARTESIAN_POINT('Origin',(0.,0.,0.));
#71820=CARTESIAN_POINT('Ctrl Pts',(1.57538060255633,14.2823529831122,35.2404039929487));
#71821=CARTESIAN_POINT('Ctrl Pts',(0.801841055750263,14.0609894914274,36.1647730322056));
#71822=CARTESIAN_POINT('Ctrl Pts',(1.38777878078145E-16,13.8232805156996,
37.1089869948545));
#71823=CARTESIAN_POINT('Ctrl Pts',(5.55111512312578E-16,13.2639498235848,
37.3125667178958));
#71824=CARTESIAN_POINT('Ctrl Pts',(0.801841055750114,12.4749251475656,36.7420532430025));
#71825=CARTESIAN_POINT('Ctrl Pts',(1.57538060255632,11.7111779096386,36.1762351867803));
#71826=CARTESIAN_POINT('Origin',(0.8,0.,0.));
#71827=CARTESIAN_POINT('',(0.,20.0571817906459,34.1448306280319));
#71828=CARTESIAN_POINT('',(-2.77555756156289E-16,19.5416998364696,34.4424442730379));
#71829=CARTESIAN_POINT('Origin',(0.,0.,0.));
#71830=CARTESIAN_POINT('Ctrl Pts',(1.57538060255632,20.1848038826479,32.224918503225));
#71831=CARTESIAN_POINT('Ctrl Pts',(0.801841055749837,20.1273183989615,33.1736836666633));
#71832=CARTESIAN_POINT('Ctrl Pts',(5.55111512312578E-16,20.0571817906459,
34.1448306280319));
#71833=CARTESIAN_POINT('Ctrl Pts',(0.,19.5416998364696,34.4424442730379));
#71834=CARTESIAN_POINT('Ctrl Pts',(0.801841055750045,18.6655935929583,34.0176108768901));
#71835=CARTESIAN_POINT('Ctrl Pts',(1.57538060255632,17.8151961173521,33.5930121843923));
#71836=CARTESIAN_POINT('Origin',(0.8,0.,0.));
#71837=CARTESIAN_POINT('',(-1.38777878078145E-16,25.6816557463071,30.1432008606945));
#71838=CARTESIAN_POINT('',(4.16333634234434E-16,25.2256851884005,30.5258055876616));
#71839=CARTESIAN_POINT('Origin',(0.,0.,0.));
#71840=CARTESIAN_POINT('Ctrl Pts',(1.57538060255632,25.4739497302129,28.2302951713764));
#71841=CARTESIAN_POINT('Ctrl Pts',(0.801841055750649,25.5820889218577,29.1746287096017));
#71842=CARTESIAN_POINT('Ctrl Pts',(-9.71445146547012E-16,25.6816557463071,
30.1432008606945));
#71843=CARTESIAN_POINT('Ctrl Pts',(4.16333634234434E-16,25.2256851884005,
30.5258055876616));
#71844=CARTESIAN_POINT('Ctrl Pts',(0.801841055749584,24.2891174222756,30.2595606180252));
#71845=CARTESIAN_POINT('Ctrl Pts',(1.57538060255632,23.3779086059641,29.989082505666));
#71846=CARTESIAN_POINT('Origin',(0.8,0.,0.));
#71847=CARTESIAN_POINT('',(0.,30.5258055876616,25.2256851884005));
#71848=CARTESIAN_POINT('',(8.32667268468867E-16,30.1432008606945,25.6816557463071));
#71849=CARTESIAN_POINT('Origin',(0.,0.,0.));
#71850=CARTESIAN_POINT('Ctrl Pts',(1.57538060255632,29.989082505666,23.3779086059641));
#71851=CARTESIAN_POINT('Ctrl Pts',(0.801841055748062,30.2595606180257,24.2891174222774));
#71852=CARTESIAN_POINT('Ctrl Pts',(-1.11022302462516E-15,30.5258055876616,
25.2256851884005));
#71853=CARTESIAN_POINT('Ctrl Pts',(6.93889390390723E-16,30.1432008606945,
25.6816557463071));
#71854=CARTESIAN_POINT('Ctrl Pts',(0.801841055750156,29.1746287096023,25.5820889218578));
#71855=CARTESIAN_POINT('Ctrl Pts',(1.57538060255632,28.2302951713764,25.4739497302129));
#71856=CARTESIAN_POINT('Origin',(0.8,0.,0.));
#71857=CARTESIAN_POINT('',(2.77555756156289E-16,34.4424442730379,19.5416998364696));
#71858=CARTESIAN_POINT('',(1.38777878078145E-16,34.1448306280319,20.0571817906459));
#71859=CARTESIAN_POINT('Origin',(0.,0.,0.));
#71860=CARTESIAN_POINT('Ctrl Pts',(1.57538060255632,33.5930121843923,17.8151961173521));
#71861=CARTESIAN_POINT('Ctrl Pts',(0.801841055749312,34.0176108768905,18.6655935929591));
#71862=CARTESIAN_POINT('Ctrl Pts',(2.77555756156289E-16,34.4424442730379,
19.5416998364696));
#71863=CARTESIAN_POINT('Ctrl Pts',(-8.32667268468867E-16,34.1448306280319,
20.0571817906459));
#71864=CARTESIAN_POINT('Ctrl Pts',(0.801841055749606,33.1736836666635,20.1273183989615));
#71865=CARTESIAN_POINT('Ctrl Pts',(1.57538060255632,32.224918503225,20.1848038826479));
#71866=CARTESIAN_POINT('Origin',(0.8,0.,0.));
#71867=CARTESIAN_POINT('',(-2.77555756156289E-16,37.3125667178958,13.2639498235848));
#71868=CARTESIAN_POINT('',(-1.38777878078145E-16,37.1089869948545,13.8232805156996));
#71869=CARTESIAN_POINT('Origin',(0.,0.,0.));
#71870=CARTESIAN_POINT('Ctrl Pts',(1.57538060255632,36.1762351867803,11.7111779096386));
#71871=CARTESIAN_POINT('Ctrl Pts',(0.801841055749034,36.7420532430033,12.4749251475666));
#71872=CARTESIAN_POINT('Ctrl Pts',(5.55111512312578E-16,37.3125667178958,
13.2639498235848));
#71873=CARTESIAN_POINT('Ctrl Pts',(1.38777878078145E-16,37.1089869948545,
13.8232805156996));
#71874=CARTESIAN_POINT('Ctrl Pts',(0.801841055750194,36.1647730322057,14.0609894914274));
#71875=CARTESIAN_POINT('Ctrl Pts',(1.57538060255633,35.2404039929487,14.2823529831122));
#71876=CARTESIAN_POINT('Origin',(0.8,0.,0.));
#71877=CARTESIAN_POINT('',(-2.77555756156289E-16,39.0489657041001,6.5831814071929));
#71878=CARTESIAN_POINT('',(0.,38.9456055698919,7.16936585720129));
#71879=CARTESIAN_POINT('Origin',(0.,0.,0.));
#71880=CARTESIAN_POINT('Ctrl Pts',(1.57538060255632,37.6602615890763,5.25132148728275));
#71881=CARTESIAN_POINT('Ctrl Pts',(0.801841055750208,38.3501069137022,5.90521241418072));
#71882=CARTESIAN_POINT('Ctrl Pts',(-4.16333634234434E-16,39.0489657041001,
6.5831814071929));
#71883=CARTESIAN_POINT('Ctrl Pts',(5.55111512312578E-16,38.9456055698919,
7.16936585720129));
#71884=CARTESIAN_POINT('Ctrl Pts',(0.801841055749313,38.0570140694242,7.56742453339975));
#71885=CARTESIAN_POINT('Ctrl Pts',(1.57538060255632,37.1851276398516,7.94594001540396));
#71886=CARTESIAN_POINT('Origin',(0.8,0.,0.));
#71887=CARTESIAN_POINT('',(4.16333634234434E-16,39.5988816271155,-0.297613645006065));
#71888=CARTESIAN_POINT('',(-1.38777878078145E-16,39.5988816271155,0.297613645006066));
#71889=CARTESIAN_POINT('Origin',(0.,0.,0.));
#71890=CARTESIAN_POINT('Ctrl Pts',(1.57538060255632,38.,-1.36809368116733));
#71891=CARTESIAN_POINT('Ctrl Pts',(0.801841055749355,38.7929119919205,-0.843927210226636));
#71892=CARTESIAN_POINT('Ctrl Pts',(-2.77555756156289E-16,39.5988816271155,
-0.297613645006065));
#71893=CARTESIAN_POINT('Ctrl Pts',(0.,39.5988816271155,0.297613645006068));
#71894=CARTESIAN_POINT('Ctrl Pts',(0.801841055750186,38.7929119919197,0.843927210227206));
#71895=CARTESIAN_POINT('Ctrl Pts',(1.57538060255633,38.,1.36809368116734));
#71896=CARTESIAN_POINT('Origin',(0.,38.,0.));
#71897=CARTESIAN_POINT('',(0.,42.75,-0.884158520433537));
#71898=CARTESIAN_POINT('',(0.,37.5167436681065,0.0899526743993834));
#71899=CARTESIAN_POINT('',(0.13820771414163,42.75,-1.00418100903022));
#71900=CARTESIAN_POINT('',(1.46228393816674,42.75,-2.15403667726254));
#71901=CARTESIAN_POINT('',(0.600000000000001,42.2794732300361,-1.31762794090604));
#71902=CARTESIAN_POINT('Ctrl Pts',(0.600000000000001,42.2794732300362,-1.31762794090604));
#71903=CARTESIAN_POINT('Ctrl Pts',(0.370217470899393,42.5142243943549,-1.16177621660585));
#71904=CARTESIAN_POINT('Ctrl Pts',(0.13820771414163,42.75,-1.00418100903022));
#71905=CARTESIAN_POINT('',(1.67735469196904,42.240333256585,-2.24593997529677));
#71906=CARTESIAN_POINT('Origin',(8.1449754609635,0.,0.));
#71907=CARTESIAN_POINT('',(1.90339248332146,37.9353893420094,-1.64091956419534));
#71908=CARTESIAN_POINT('Origin',(0.,37.4226946144639,6.59863075134335));
#71909=CARTESIAN_POINT('',(0.,42.2540639571139,6.55273342944652));
#71910=CARTESIAN_POINT('',(0.,37.2427065776832,6.60034061210452));
#71911=CARTESIAN_POINT('',(0.138207714141617,42.2749056435377,6.4345343521407));
#71912=CARTESIAN_POINT('',(1.46228393816674,42.4745759849063,5.30214757522046));
#71913=CARTESIAN_POINT('',(0.600000000000001,41.8659567209931,6.04414326732376));
#71914=CARTESIAN_POINT('Ctrl Pts',(0.6,41.8659567209931,6.04414326732376));
#71915=CARTESIAN_POINT('Ctrl Pts',(0.370217470897594,42.0700781197334,6.23839136562556));
#71916=CARTESIAN_POINT('Ctrl Pts',(0.138207714141617,42.2749056435377,6.4345343521407));
#71917=CARTESIAN_POINT('',(1.67735469196904,41.9886110647639,5.12313779357752));
#71918=CARTESIAN_POINT('Origin',(8.1449754609635,0.,0.));
#71919=CARTESIAN_POINT('',(1.90339248332146,37.6440082295681,4.97142091943645));
#71920=CARTESIAN_POINT('Origin',(0.,35.7083195898645,12.9967654463754));
#71921=CARTESIAN_POINT('',(0.,40.4742595624789,13.790523889916));
#71922=CARTESIAN_POINT('',(0.,35.2836459493057,12.9260368409209));
#71923=CARTESIAN_POINT('',(0.138207714141626,40.515309671231,13.6777396430533));
#71924=CARTESIAN_POINT('',(1.46228393816674,40.9085834716837,12.5972287566465));
#71925=CARTESIAN_POINT('',(0.600000000000001,40.1803643021789,13.22226624086));
#71926=CARTESIAN_POINT('Ctrl Pts',(0.600000000000002,40.1803643021789,13.22226624086));
#71927=CARTESIAN_POINT('Ctrl Pts',(0.37021747089599,40.3476538099299,13.4490085829912));
#71928=CARTESIAN_POINT('Ctrl Pts',(0.138207714141626,40.515309671231,13.6777396430533));
#71929=CARTESIAN_POINT('',(1.67735469196904,40.4610861730024,12.3365516130268));
#71930=CARTESIAN_POINT('Origin',(8.1449754609635,0.,0.));
#71931=CARTESIAN_POINT('',(1.90339248332146,36.2088329758587,11.4327072940915));
#71932=CARTESIAN_POINT('Origin',(0.,32.9089653438087,19.));
#71933=CARTESIAN_POINT('',(0.,37.4646652720015,20.6092962603321));
#71934=CARTESIAN_POINT('',(0.,31.7439889350152,18.5884732955206));
#71935=CARTESIAN_POINT('',(0.138207714141626,37.5246765162999,20.5053537361819));
#71936=CARTESIAN_POINT('',(1.46228393816674,38.099604350416,19.5095495168072));
#71937=CARTESIAN_POINT('',(0.600000000000001,37.2739118462884,19.9986373454573));
#71938=CARTESIAN_POINT('Ctrl Pts',(0.600000000000003,37.2739118462884,19.9986373454573));
#71939=CARTESIAN_POINT('Ctrl Pts',(0.370217470897655,37.3992864560072,20.2509844800861));
#71940=CARTESIAN_POINT('Ctrl Pts',(0.138207714141626,37.5246765162998,20.5053537361819));
#71941=CARTESIAN_POINT('',(1.67735469196904,37.7041716521717,19.1751255543105));
#71942=CARTESIAN_POINT('Origin',(8.1449754609635,0.,0.));
#71943=CARTESIAN_POINT('',(1.90339248332146,33.6734706547313,17.5466166428447));
#71944=CARTESIAN_POINT('Origin',(0.,29.1096888385212,24.4259291680885));
#71945=CARTESIAN_POINT('',(0.,33.3167260852698,26.8018655926851));
#71946=CARTESIAN_POINT('',(0.,26.8714229747626,23.1618620629671));
#71947=CARTESIAN_POINT('',(0.138207714141623,33.3938750538235,26.7099230322464));
#71948=CARTESIAN_POINT('',(1.46228393816674,34.132988030291,25.8290824872081));
#71949=CARTESIAN_POINT('',(0.600000000000001,33.234910440458,26.1673599741116));
#71950=CARTESIAN_POINT('Ctrl Pts',(0.600000000000003,33.234910440458,26.1673599741116));
#71951=CARTESIAN_POINT('Ctrl Pts',(0.370217470903501,33.3145607080702,26.437644461241));
#71952=CARTESIAN_POINT('Ctrl Pts',(0.138207714141623,33.3938750538235,26.7099230322464));
#71953=CARTESIAN_POINT('',(1.67735469196904,33.8016349549212,25.4310730087083));
#71954=CARTESIAN_POINT('Origin',(8.1449754609635,0.,0.));
#71955=CARTESIAN_POINT('',(1.90339248332146,30.1149569673582,23.1273809239214));
#71956=CARTESIAN_POINT('Origin',(0.,24.4259291680885,29.1096888385212));
#71957=CARTESIAN_POINT('',(0.,28.156475035514,32.1800738014028));
#71958=CARTESIAN_POINT('',(0.,21.0324673783039,26.3167372379398));
#71959=CARTESIAN_POINT('',(0.138207714141625,28.2484175959528,32.1029248328492));
#71960=CARTESIAN_POINT('',(1.46228393816674,29.129258140991,31.3638118563816));
#71961=CARTESIAN_POINT('',(0.600000000000001,28.1860830985703,31.5410006112756));
#71962=CARTESIAN_POINT('Ctrl Pts',(0.600000000000002,28.1860830985703,31.5410006112756));
#71963=CARTESIAN_POINT('Ctrl Pts',(0.370217470900064,28.2175888910031,31.8210099935453));
#71964=CARTESIAN_POINT('Ctrl Pts',(0.138207714141625,28.2484175959528,32.1029248328492));
#71965=CARTESIAN_POINT('',(1.67735469196904,28.872052684018,30.9143101784803));
#71966=CARTESIAN_POINT('Origin',(8.1449754609635,0.,0.));
#71967=CARTESIAN_POINT('',(1.90339248332146,25.6414155514355,28.0054314386442));
#71968=CARTESIAN_POINT('Origin',(0.,19.,32.9089653438087));
#71969=CARTESIAN_POINT('',(0.,22.1407037396679,36.580506751568));
#71970=CARTESIAN_POINT('',(0.,14.6749862528265,27.8529433888201));
#71971=CARTESIAN_POINT('',(0.138207714141622,22.2446462638181,36.5204955072696));
#71972=CARTESIAN_POINT('',(1.46228393816674,23.2404504831928,35.9455676731535));
#71973=CARTESIAN_POINT('',(0.600000000000001,22.2808358845789,35.9562839053824));
#71974=CARTESIAN_POINT('Ctrl Pts',(0.600000000000003,22.2808358845789,35.9562839053824));
#71975=CARTESIAN_POINT('Ctrl Pts',(0.370217470897647,22.2632399142705,36.2375102394026));
#71976=CARTESIAN_POINT('Ctrl Pts',(0.138207714141622,22.2446462638181,36.5204955072696));
#71977=CARTESIAN_POINT('',(1.67735469196904,23.0652077022745,35.4582316768749));
#71978=CARTESIAN_POINT('Origin',(8.1449754609635,0.,0.));
#71979=CARTESIAN_POINT('',(1.90339248332146,20.3887726991648,32.0325510905359));
#71980=CARTESIAN_POINT('Origin',(0.,12.9967654463754,35.7083195898645));
#71981=CARTESIAN_POINT('',(0.,15.4521983644287,39.8694595147163));
#71982=CARTESIAN_POINT('',(0.,8.28196006949682,27.7182968336373));
#71983=CARTESIAN_POINT('',(0.138207714141624,15.5649826112914,39.8284094059642));
#71984=CARTESIAN_POINT('',(1.46228393816674,16.6454934976982,39.4351356055115));
#71985=CARTESIAN_POINT('',(0.600000000000001,15.6985967468815,39.2790537077817));
#71986=CARTESIAN_POINT('Ctrl Pts',(0.600000000000003,15.6985967468815,39.2790537077817));
#71987=CARTESIAN_POINT('Ctrl Pts',(0.37021747089523,15.6324336584848,39.5529520737006));
#71988=CARTESIAN_POINT('Ctrl Pts',(0.138207714141624,15.5649826112914,39.8284094059641));
#71989=CARTESIAN_POINT('',(1.67735469196904,16.5575380560557,38.9247727484987));
#71990=CARTESIAN_POINT('Origin',(8.14497546096349,0.,0.));
#71991=CARTESIAN_POINT('',(1.90339248332146,14.5166273056467,35.0863778867947));
#71992=CARTESIAN_POINT('Origin',(0.,6.59863075134336,37.4226946144639));
#71993=CARTESIAN_POINT('',(0.,8.29418576107603,41.9469989254299));
#71994=CARTESIAN_POINT('',(0.,2.32185498719982,26.0108354204645));
#71995=CARTESIAN_POINT('',(0.138207714141621,8.41238483838185,41.9261572390061));
#71996=CARTESIAN_POINT('',(1.46228393816674,9.54477161530209,41.7264868976375));
#71997=CARTESIAN_POINT('',(0.600000000000001,8.63936369090333,41.4083493394303));
#71998=CARTESIAN_POINT('Ctrl Pts',(0.600000000000004,8.63936369090333,41.4083493394303));
#71999=CARTESIAN_POINT('Ctrl Pts',(0.370217470893892,8.5266438163786,41.6665974739972));
#72000=CARTESIAN_POINT('Ctrl Pts',(0.138207714141621,8.41238483838185,41.9261572390061));
#72001=CARTESIAN_POINT('',(1.67735469196904,9.54677599452213,41.2086042970448));
#72002=CARTESIAN_POINT('Origin',(8.1449754609635,0.,0.));
#72003=CARTESIAN_POINT('',(1.90339248332146,8.20340153721441,37.0741228455271));
#72004=CARTESIAN_POINT('Origin',(0.,2.32682891837997E-15,38.));
#72005=CARTESIAN_POINT('',(0.,0.884158520433539,42.75));
#72006=CARTESIAN_POINT('',(0.,-2.79868590723512,22.9645083408252));
#72007=CARTESIAN_POINT('',(0.138207714141629,1.00418100903022,42.75));
#72008=CARTESIAN_POINT('',(1.46228393816674,2.15403667726255,42.75));
#72009=CARTESIAN_POINT('',(0.600000000000001,1.31762794090604,42.2794732300361));
#72010=CARTESIAN_POINT('Ctrl Pts',(0.600000000000004,1.31762794090604,42.2794732300361));
#72011=CARTESIAN_POINT('Ctrl Pts',(0.37021747089638,1.1617762166038,42.5142243943579));
#72012=CARTESIAN_POINT('Ctrl Pts',(0.138207714141629,1.00418100903022,42.75));
#72013=CARTESIAN_POINT('',(1.67735469196904,2.24593997529677,42.240333256585));
#72014=CARTESIAN_POINT('Origin',(8.1449754609635,0.,0.));
#72015=CARTESIAN_POINT('',(1.90339248332146,1.64091956419534,37.9353893420094));
#72016=CARTESIAN_POINT('Origin',(0.,-6.59863075134335,37.4226946144639));
#72017=CARTESIAN_POINT('',(0.,-6.55273342944652,42.2540639571139));
#72018=CARTESIAN_POINT('',(0.,-6.77440269836428,18.9201075126787));
#72019=CARTESIAN_POINT('',(0.138207714141616,-6.4345343521407,42.2749056435377));
#72020=CARTESIAN_POINT('',(1.46228393816674,-5.30214757522046,42.4745759849063));
#72021=CARTESIAN_POINT('',(0.600000000000001,-6.04414326732376,41.8659567209931));
#72022=CARTESIAN_POINT('Ctrl Pts',(0.600000000000004,-6.04414326732376,
41.8659567209931));
#72023=CARTESIAN_POINT('Ctrl Pts',(0.370217470895893,-6.23839136562701,
42.0700781197349));
#72024=CARTESIAN_POINT('Ctrl Pts',(0.138207714141616,-6.4345343521407,42.2749056435377));
#72025=CARTESIAN_POINT('',(1.67735469196904,-5.12313779357752,41.9886110647639));
#72026=CARTESIAN_POINT('Origin',(8.1449754609635,0.,0.));
#72027=CARTESIAN_POINT('',(1.90339248332146,-4.97142091943645,37.6440082295681));
#72028=CARTESIAN_POINT('Origin',(0.,-12.9967654463754,35.7083195898645));
#72029=CARTESIAN_POINT('',(0.,-13.790523889916,40.4742595624789));
#72030=CARTESIAN_POINT('',(0.,-9.42874680865831,14.2849724911192));
#72031=CARTESIAN_POINT('',(0.138207714141626,-13.6777396430533,40.515309671231));
#72032=CARTESIAN_POINT('',(1.46228393816674,-12.5972287566465,40.9085834716837));
#72033=CARTESIAN_POINT('',(0.600000000000001,-13.22226624086,40.1803643021789));
#72034=CARTESIAN_POINT('Ctrl Pts',(0.600000000000004,-13.22226624086,40.1803643021789));
#72035=CARTESIAN_POINT('Ctrl Pts',(0.370217470891807,-13.4490085829953,
40.3476538099329));
#72036=CARTESIAN_POINT('Ctrl Pts',(0.138207714141626,-13.6777396430533,
40.515309671231));
#72037=CARTESIAN_POINT('',(1.67735469196904,-12.3365516130268,40.4610861730024));
#72038=CARTESIAN_POINT('Origin',(8.1449754609635,0.,0.));
#72039=CARTESIAN_POINT('',(1.90339248332146,-11.4327072940915,36.2088329758587));
#72040=CARTESIAN_POINT('Origin',(0.,-19.,32.9089653438087));
#72041=CARTESIAN_POINT('',(0.,-20.6092962603321,37.4646652720015));
#72042=CARTESIAN_POINT('',(0.,-10.7259694216695,9.48630449465761));
#72043=CARTESIAN_POINT('',(0.138207714141623,-20.5053537361819,37.5246765162999));
#72044=CARTESIAN_POINT('',(1.46228393816674,-19.5095495168072,38.099604350416));
#72045=CARTESIAN_POINT('',(0.600000000000001,-19.9986373454573,37.2739118462884));
#72046=CARTESIAN_POINT('Ctrl Pts',(0.600000000000005,-19.9986373454573,
37.2739118462884));
#72047=CARTESIAN_POINT('Ctrl Pts',(0.370217470900507,-20.250984480083,37.3992864560057));
#72048=CARTESIAN_POINT('Ctrl Pts',(0.138207714141623,-20.5053537361819,
37.5246765162998));
#72049=CARTESIAN_POINT('',(1.67735469196904,-19.1751255543105,37.7041716521717));
#72050=CARTESIAN_POINT('Origin',(8.1449754609635,0.,0.));
#72051=CARTESIAN_POINT('',(1.90339248332146,-17.5466166428447,33.6734706547313));
#72052=CARTESIAN_POINT('Origin',(0.,-24.4259291680885,29.1096888385212));
#72053=CARTESIAN_POINT('',(0.,-26.8018655926851,33.3167260852698));
#72054=CARTESIAN_POINT('',(0.,-10.7667918374521,4.92364626871755));
#72055=CARTESIAN_POINT('',(0.138207714141626,-26.7099230322463,33.3938750538235));
#72056=CARTESIAN_POINT('',(1.46228393816674,-25.8290824872081,34.132988030291));
#72057=CARTESIAN_POINT('',(0.600000000000001,-26.1673599741116,33.234910440458));
#72058=CARTESIAN_POINT('Ctrl Pts',(0.600000000000004,-26.1673599741116,
33.234910440458));
#72059=CARTESIAN_POINT('Ctrl Pts',(0.370217470899579,-26.4376444612456,
33.3145607080715));
#72060=CARTESIAN_POINT('Ctrl Pts',(0.138207714141626,-26.7099230322463,
33.3938750538235));
#72061=CARTESIAN_POINT('',(1.67735469196904,-25.4310730087083,33.8016349549212));
#72062=CARTESIAN_POINT('Origin',(8.1449754609635,0.,0.));
#72063=CARTESIAN_POINT('',(1.90339248332146,-23.1273809239214,30.1149569673582));
#72064=CARTESIAN_POINT('Origin',(0.,-29.1096888385212,24.4259291680885));
#72065=CARTESIAN_POINT('',(0.,-32.1800738014028,28.156475035514));
#72066=CARTESIAN_POINT('',(0.,-9.76844254625099,0.92613767654611));
#72067=CARTESIAN_POINT('',(0.138207714141625,-32.1029248328492,28.2484175959528));
#72068=CARTESIAN_POINT('',(1.46228393816674,-31.3638118563816,29.129258140991));
#72069=CARTESIAN_POINT('',(0.600000000000001,-31.5410006112756,28.1860830985703));
#72070=CARTESIAN_POINT('Ctrl Pts',(0.600000000000004,-31.5410006112756,
28.1860830985703));
#72071=CARTESIAN_POINT('Ctrl Pts',(0.370217470900199,-31.8210099935451,
28.2175888910031));
#72072=CARTESIAN_POINT('Ctrl Pts',(0.138207714141625,-32.1029248328492,
28.2484175959528));
#72073=CARTESIAN_POINT('',(1.67735469196904,-30.9143101784803,28.872052684018));
#72074=CARTESIAN_POINT('Origin',(8.1449754609635,0.,0.));
#72075=CARTESIAN_POINT('',(1.90339248332146,-28.0054314386442,25.6414155514355));
#72076=CARTESIAN_POINT('Origin',(0.,-32.9089653438087,19.));
#72077=CARTESIAN_POINT('',(0.,-36.580506751568,22.1407037396679));
#72078=CARTESIAN_POINT('',(0.,-8.03170628213326,-2.28046286024977));
#72079=CARTESIAN_POINT('',(0.138207714141621,-36.5204955072697,22.244646263818));
#72080=CARTESIAN_POINT('',(1.46228393816674,-35.9455676731535,23.2404504831928));
#72081=CARTESIAN_POINT('',(0.600000000000001,-35.9562839053824,22.2808358845789));
#72082=CARTESIAN_POINT('Ctrl Pts',(0.600000000000004,-35.9562839053824,
22.2808358845789));
#72083=CARTESIAN_POINT('Ctrl Pts',(0.370217470899393,-36.2375102394005,
22.2632399142707));
#72084=CARTESIAN_POINT('Ctrl Pts',(0.138207714141621,-36.5204955072697,
22.244646263818));
#72085=CARTESIAN_POINT('',(1.67735469196904,-35.4582316768749,23.0652077022745));
#72086=CARTESIAN_POINT('Origin',(8.1449754609635,0.,0.));
#72087=CARTESIAN_POINT('',(1.90339248332146,-32.0325510905359,20.3887726991648));
#72088=CARTESIAN_POINT('Origin',(0.,-35.7083195898645,12.9967654463754));
#72089=CARTESIAN_POINT('',(0.,-39.8694595147163,15.4521983644287));
#72090=CARTESIAN_POINT('',(0.,-5.89916452186253,-4.59321757154364));
#72091=CARTESIAN_POINT('',(0.138207714141621,-39.8284094059642,15.5649826112914));
#72092=CARTESIAN_POINT('',(1.46228393816674,-39.4351356055115,16.6454934976982));
#72093=CARTESIAN_POINT('',(0.600000000000001,-39.2790537077817,15.6985967468815));
#72094=CARTESIAN_POINT('Ctrl Pts',(0.600000000000005,-39.2790537077817,
15.6985967468815));
#72095=CARTESIAN_POINT('Ctrl Pts',(0.370217470897566,-39.5529520736978,
15.6324336584854));
#72096=CARTESIAN_POINT('Ctrl Pts',(0.138207714141621,-39.8284094059642,
15.5649826112914));
#72097=CARTESIAN_POINT('',(1.67735469196904,-38.9247727484987,16.5575380560557));
#72098=CARTESIAN_POINT('Origin',(8.1449754609635,0.,0.));
#72099=CARTESIAN_POINT('',(1.90339248332146,-35.0863778867947,14.5166273056467));
#72100=CARTESIAN_POINT('Origin',(0.,-37.4226946144639,6.59863075134337));
#72101=CARTESIAN_POINT('',(0.,-41.9469989254299,8.29418576107604));
#72102=CARTESIAN_POINT('',(0.,-3.70983076103834,-6.03580125637146));
#72103=CARTESIAN_POINT('',(0.138207714141622,-41.9261572390061,8.41238483838186));
#72104=CARTESIAN_POINT('',(1.46228393816674,-41.7264868976375,9.5447716153021));
#72105=CARTESIAN_POINT('',(0.600000000000001,-41.4083493394303,8.63936369090334));
#72106=CARTESIAN_POINT('Ctrl Pts',(0.600000000000005,-41.4083493394303,
8.63936369090334));
#72107=CARTESIAN_POINT('Ctrl Pts',(0.370217470898631,-41.6665974739919,
8.52664381638094));
#72108=CARTESIAN_POINT('Ctrl Pts',(0.138207714141622,-41.9261572390061,
8.41238483838186));
#72109=CARTESIAN_POINT('',(1.67735469196904,-41.2086042970448,9.54677599452215));
#72110=CARTESIAN_POINT('Origin',(8.1449754609635,0.,0.));
#72111=CARTESIAN_POINT('',(1.90339248332146,-37.074122845527,8.20340153721442));
#72112=CARTESIAN_POINT('Origin',(0.,-38.,4.65365783675994E-15));
#72113=CARTESIAN_POINT('',(0.,-42.75,0.884158520433542));
#72114=CARTESIAN_POINT('',(0.,-1.75577510798945,-6.74645057995377));
#72115=CARTESIAN_POINT('',(0.13820771414162,-42.75,1.00418100903021));
#72116=CARTESIAN_POINT('',(1.46228393816674,-42.75,2.15403667726255));
#72117=CARTESIAN_POINT('',(0.600000000000001,-42.2794732300361,1.31762794090605));
#72118=CARTESIAN_POINT('Ctrl Pts',(0.600000000000006,-42.2794732300361,
1.31762794090605));
#72119=CARTESIAN_POINT('Ctrl Pts',(0.370217470900961,-42.5142243943533,
1.16177621660692));
#72120=CARTESIAN_POINT('Ctrl Pts',(0.13820771414162,-42.75,1.00418100903021));
#72121=CARTESIAN_POINT('',(1.67735469196904,-42.240333256585,2.24593997529678));
#72122=CARTESIAN_POINT('Origin',(8.1449754609635,0.,0.));
#72123=CARTESIAN_POINT('',(1.90339248332146,-37.9353893420094,1.64091956419534));
#72124=CARTESIAN_POINT('Origin',(0.,-37.4226946144639,-6.59863075134334));
#72125=CARTESIAN_POINT('',(0.,-42.2540639571139,-6.55273342944651));
#72126=CARTESIAN_POINT('',(0.,-0.246045426418917,-6.95180363335973));
#72127=CARTESIAN_POINT('',(0.138207714141624,-42.2749056435377,-6.43453435214068));
#72128=CARTESIAN_POINT('',(1.46228393816674,-42.4745759849063,-5.30214757522045));
#72129=CARTESIAN_POINT('',(0.600000000000001,-41.8659567209931,-6.04414326732375));
#72130=CARTESIAN_POINT('Ctrl Pts',(0.600000000000006,-41.8659567209931,
-6.04414326732374));
#72131=CARTESIAN_POINT('Ctrl Pts',(0.370217470894059,-42.0700781197365,
-6.23839136562854));
#72132=CARTESIAN_POINT('Ctrl Pts',(0.138207714141624,-42.2749056435377,
-6.43453435214068));
#72133=CARTESIAN_POINT('',(1.67735469196904,-41.9886110647639,-5.1231377935775));
#72134=CARTESIAN_POINT('Origin',(8.1449754609635,0.,0.));
#72135=CARTESIAN_POINT('',(1.90339248332146,-37.6440082295681,-4.97142091943644));
#72136=CARTESIAN_POINT('Origin',(0.,-35.7083195898645,-12.9967654463754));
#72137=CARTESIAN_POINT('',(0.,-40.4742595624789,-13.790523889916));
#72138=CARTESIAN_POINT('',(0.,0.717737476618173,-6.93007335047185));
#72139=CARTESIAN_POINT('',(0.138207714141626,-40.515309671231,-13.6777396430533));
#72140=CARTESIAN_POINT('',(1.46228393816674,-40.9085834716837,-12.5972287566465));
#72141=CARTESIAN_POINT('',(0.600000000000001,-40.1803643021789,-13.22226624086));
#72142=CARTESIAN_POINT('Ctrl Pts',(0.600000000000006,-40.1803643021789,
-13.22226624086));
#72143=CARTESIAN_POINT('Ctrl Pts',(0.370217470897712,-40.3476538099286,
-13.4490085829895));
#72144=CARTESIAN_POINT('Ctrl Pts',(0.138207714141626,-40.515309671231,-13.6777396430533));
#72145=CARTESIAN_POINT('',(1.67735469196904,-40.4610861730024,-12.3365516130268));
#72146=CARTESIAN_POINT('Origin',(8.1449754609635,0.,0.));
#72147=CARTESIAN_POINT('',(1.90339248332146,-36.2088329758587,-11.4327072940915));
#72148=CARTESIAN_POINT('Origin',(0.,-32.9089653438087,-19.));
#72149=CARTESIAN_POINT('',(0.,-37.4646652720015,-20.6092962603321));
#72150=CARTESIAN_POINT('',(0.,1.15119163149133,-6.96828498131187));
#72151=CARTESIAN_POINT('',(0.138207714141633,-37.5246765162999,-20.5053537361819));
#72152=CARTESIAN_POINT('',(1.46228393816674,-38.099604350416,-19.5095495168072));
#72153=CARTESIAN_POINT('',(0.600000000000001,-37.2739118462884,-19.9986373454573));
#72154=CARTESIAN_POINT('Ctrl Pts',(0.600000000000006,-37.2739118462884,
-19.9986373454572));
#72155=CARTESIAN_POINT('Ctrl Pts',(0.370217470897372,-37.3992864560074,
-20.2509844800864));
#72156=CARTESIAN_POINT('Ctrl Pts',(0.138207714141633,-37.5246765162999,
-20.5053537361819));
#72157=CARTESIAN_POINT('',(1.67735469196904,-37.7041716521717,-19.1751255543105));
#72158=CARTESIAN_POINT('Origin',(8.1449754609635,0.,0.));
#72159=CARTESIAN_POINT('',(1.90339248332146,-33.6734706547313,-17.5466166428447));
#72160=CARTESIAN_POINT('Origin',(0.,-29.1096888385212,-24.4259291680885));
#72161=CARTESIAN_POINT('',(0.,-33.3167260852698,-26.8018655926851));
#72162=CARTESIAN_POINT('',(0.,1.18128350576745,-7.31901513140711));
#72163=CARTESIAN_POINT('',(0.138207714141623,-33.3938750538235,-26.7099230322464));
#72164=CARTESIAN_POINT('',(1.46228393816674,-34.132988030291,-25.8290824872081));
#72165=CARTESIAN_POINT('',(0.600000000000001,-33.234910440458,-26.1673599741116));
#72166=CARTESIAN_POINT('Ctrl Pts',(0.600000000000006,-33.234910440458,-26.1673599741116));
#72167=CARTESIAN_POINT('Ctrl Pts',(0.370217470902497,-33.3145607080705,
-26.4376444612422));
#72168=CARTESIAN_POINT('Ctrl Pts',(0.138207714141623,-33.3938750538235,
-26.7099230322464));
#72169=CARTESIAN_POINT('',(1.67735469196904,-33.8016349549212,-25.4310730087083));
#72170=CARTESIAN_POINT('Origin',(8.1449754609635,0.,0.));
#72171=CARTESIAN_POINT('',(1.90339248332146,-30.1149569673582,-23.1273809239214));
#72172=CARTESIAN_POINT('Origin',(0.,-24.4259291680885,-29.1096888385212));
#72173=CARTESIAN_POINT('',(0.,-28.156475035514,-32.1800738014028));
#72174=CARTESIAN_POINT('',(0.,1.02556763176512,-8.16211284449324));
#72175=CARTESIAN_POINT('',(0.138207714141625,-28.2484175959528,-32.1029248328492));
#72176=CARTESIAN_POINT('',(1.46228393816674,-29.129258140991,-31.3638118563816));
#72177=CARTESIAN_POINT('',(0.600000000000001,-28.1860830985703,-31.5410006112756));
#72178=CARTESIAN_POINT('Ctrl Pts',(0.600000000000006,-28.1860830985703,
-31.5410006112756));
#72179=CARTESIAN_POINT('Ctrl Pts',(0.370217470901873,-28.2175888910029,
-31.8210099935431));
#72180=CARTESIAN_POINT('Ctrl Pts',(0.138207714141625,-28.2484175959528,
-32.1029248328492));
#72181=CARTESIAN_POINT('',(1.67735469196904,-28.872052684018,-30.9143101784803));
#72182=CARTESIAN_POINT('Origin',(8.1449754609635,0.,0.));
#72183=CARTESIAN_POINT('',(1.90339248332146,-25.6414155514355,-28.0054314386442));
#72184=CARTESIAN_POINT('Origin',(0.,-19.,-32.9089653438087));
#72185=CARTESIAN_POINT('',(0.,-22.1407037396679,-36.580506751568));
#72186=CARTESIAN_POINT('',(0.,0.959225753562968,-9.57625716905698));
#72187=CARTESIAN_POINT('',(0.138207714141625,-22.2446462638181,-36.5204955072696));
#72188=CARTESIAN_POINT('',(1.46228393816674,-23.2404504831928,-35.9455676731535));
#72189=CARTESIAN_POINT('',(0.600000000000001,-22.2808358845789,-35.9562839053824));
#72190=CARTESIAN_POINT('Ctrl Pts',(0.600000000000006,-22.2808358845789,
-35.9562839053824));
#72191=CARTESIAN_POINT('Ctrl Pts',(0.37021747090221,-22.2632399142709,-36.237510239397));
#72192=CARTESIAN_POINT('Ctrl Pts',(0.138207714141625,-22.2446462638181,
-36.5204955072696));
#72193=CARTESIAN_POINT('',(1.67735469196904,-23.0652077022745,-35.4582316768749));
#72194=CARTESIAN_POINT('Origin',(8.14497546096349,0.,0.));
#72195=CARTESIAN_POINT('',(1.90339248332146,-20.3887726991648,-32.0325510905359));
#72196=CARTESIAN_POINT('Origin',(0.,-12.9967654463754,-35.7083195898645));
#72197=CARTESIAN_POINT('',(0.,-15.4521983644287,-39.8694595147163));
#72198=CARTESIAN_POINT('',(0.,1.27408525976888,-11.5239868808221));
#72199=CARTESIAN_POINT('',(0.138207714141625,-15.5649826112914,-39.8284094059641));
#72200=CARTESIAN_POINT('',(1.46228393816674,-16.6454934976982,-39.4351356055115));
#72201=CARTESIAN_POINT('',(0.600000000000001,-15.6985967468815,-39.2790537077817));
#72202=CARTESIAN_POINT('Ctrl Pts',(0.600000000000006,-15.6985967468815,
-39.2790537077817));
#72203=CARTESIAN_POINT('Ctrl Pts',(0.370217470897549,-15.6324336584855,
-39.5529520736978));
#72204=CARTESIAN_POINT('Ctrl Pts',(0.138207714141625,-15.5649826112914,
-39.8284094059641));
#72205=CARTESIAN_POINT('',(1.67735469196904,-16.5575380560557,-38.9247727484987));
#72206=CARTESIAN_POINT('Origin',(8.1449754609635,0.,0.));
#72207=CARTESIAN_POINT('',(1.90339248332146,-14.5166273056467,-35.0863778867947));
#72208=CARTESIAN_POINT('Origin',(0.,-6.59863075134335,-37.4226946144639));
#72209=CARTESIAN_POINT('',(0.,-8.29418576107602,-41.9469989254299));
#72210=CARTESIAN_POINT('',(0.,2.23479659694533,-13.8521745174671));
#72211=CARTESIAN_POINT('',(0.138207714141623,-8.41238483838184,-41.9261572390061));
#72212=CARTESIAN_POINT('',(1.46228393816674,-9.54477161530208,-41.7264868976375));
#72213=CARTESIAN_POINT('',(0.600000000000001,-8.63936369090332,-41.4083493394303));
#72214=CARTESIAN_POINT('Ctrl Pts',(0.600000000000007,-8.63936369090333,
-41.4083493394303));
#72215=CARTESIAN_POINT('Ctrl Pts',(0.370217470894352,-8.52664381637882,
-41.6665974739967));
#72216=CARTESIAN_POINT('Ctrl Pts',(0.138207714141623,-8.41238483838184,
-41.9261572390061));
#72217=CARTESIAN_POINT('',(1.67735469196904,-9.54677599452213,-41.2086042970448));
#72218=CARTESIAN_POINT('Origin',(8.1449754609635,0.,0.));
#72219=CARTESIAN_POINT('',(1.90339248332146,-8.20340153721441,-37.0741228455271));
#72220=CARTESIAN_POINT('Origin',(0.,-6.98048675513991E-15,-38.));
#72221=CARTESIAN_POINT('',(0.,-0.884158520433544,-42.75));
#72222=CARTESIAN_POINT('',(0.,4.03771734711804,-16.3080104352708));
#72223=CARTESIAN_POINT('',(0.138207714141621,-1.00418100903022,-42.75));
#72224=CARTESIAN_POINT('',(1.46228393816674,-2.15403667726255,-42.75));
#72225=CARTESIAN_POINT('',(0.600000000000001,-1.31762794090605,-42.2794732300361));
#72226=CARTESIAN_POINT('Ctrl Pts',(0.600000000000007,-1.31762794090605,
-42.2794732300361));
#72227=CARTESIAN_POINT('Ctrl Pts',(0.37021747090171,-1.16177621660743,-42.5142243943525));
#72228=CARTESIAN_POINT('Ctrl Pts',(0.138207714141621,-1.00418100903022,
-42.75));
#72229=CARTESIAN_POINT('',(1.67735469196904,-2.24593997529678,-42.240333256585));
#72230=CARTESIAN_POINT('Origin',(8.1449754609635,0.,0.));
#72231=CARTESIAN_POINT('',(1.90339248332146,-1.64091956419534,-37.9353893420094));
#72232=CARTESIAN_POINT('Origin',(0.,6.59863075134334,-37.4226946144639));
#72233=CARTESIAN_POINT('',(0.,6.5527334294465,-42.2540639571139));
#72234=CARTESIAN_POINT('',(0.,6.77774154709997,-18.5686444914235));
#72235=CARTESIAN_POINT('',(0.138207714141623,6.43453435214068,-42.2749056435377));
#72236=CARTESIAN_POINT('',(1.46228393816674,5.30214757522045,-42.4745759849063));
#72237=CARTESIAN_POINT('',(0.600000000000001,6.04414326732375,-41.8659567209931));
#72238=CARTESIAN_POINT('Ctrl Pts',(0.600000000000007,6.04414326732374,-41.8659567209931));
#72239=CARTESIAN_POINT('Ctrl Pts',(0.370217470894012,6.23839136562858,-42.0700781197365));
#72240=CARTESIAN_POINT('Ctrl Pts',(0.138207714141623,6.43453435214068,-42.2749056435377));
#72241=CARTESIAN_POINT('',(1.67735469196904,5.1231377935775,-41.9886110647639));
#72242=CARTESIAN_POINT('Origin',(8.1449754609635,0.,0.));
#72243=CARTESIAN_POINT('',(1.90339248332146,4.97142091943644,-37.6440082295681));
#72244=CARTESIAN_POINT('Origin',(0.,12.9967654463754,-35.7083195898645));
#72245=CARTESIAN_POINT('',(0.,13.7905238899159,-40.4742595624789));
#72246=CARTESIAN_POINT('',(0.,10.4273633827345,-20.2809359815683));
#72247=CARTESIAN_POINT('',(0.138207714141626,13.6777396430533,-40.515309671231));
#72248=CARTESIAN_POINT('',(1.46228393816674,12.5972287566465,-40.9085834716837));
#72249=CARTESIAN_POINT('',(0.600000000000001,13.22226624086,-40.1803643021789));
#72250=CARTESIAN_POINT('Ctrl Pts',(0.600000000000008,13.22226624086,-40.1803643021789));
#72251=CARTESIAN_POINT('Ctrl Pts',(0.370217470897429,13.4490085829897,-40.3476538099288));
#72252=CARTESIAN_POINT('Ctrl Pts',(0.138207714141626,13.6777396430533,-40.515309671231));
#72253=CARTESIAN_POINT('',(1.67735469196904,12.3365516130267,-40.4610861730024));
#72254=CARTESIAN_POINT('Origin',(8.1449754609635,0.,0.));
#72255=CARTESIAN_POINT('',(1.90339248332146,11.4327072940915,-36.2088329758587));
#72256=CARTESIAN_POINT('Origin',(0.,19.,-32.9089653438087));
#72257=CARTESIAN_POINT('',(0.,20.6092962603321,-37.4646652720015));
#72258=CARTESIAN_POINT('',(0.,14.8307888551629,-21.1064928088663));
#72259=CARTESIAN_POINT('',(0.138207714141623,20.505353736182,-37.5246765162999));
#72260=CARTESIAN_POINT('',(1.46228393816674,19.5095495168072,-38.099604350416));
#72261=CARTESIAN_POINT('',(0.600000000000001,19.9986373454573,-37.2739118462884));
#72262=CARTESIAN_POINT('Ctrl Pts',(0.600000000000008,19.9986373454573,-37.2739118462884));
#72263=CARTESIAN_POINT('Ctrl Pts',(0.370217470899336,20.2509844800843,-37.3992864560063));
#72264=CARTESIAN_POINT('Ctrl Pts',(0.138207714141623,20.505353736182,-37.5246765162999));
#72265=CARTESIAN_POINT('',(1.67735469196904,19.1751255543105,-37.7041716521717));
#72266=CARTESIAN_POINT('Origin',(8.1449754609635,0.,0.));
#72267=CARTESIAN_POINT('',(1.90339248332146,17.5466166428447,-33.6734706547313));
#72268=CARTESIAN_POINT('Origin',(0.,24.4259291680885,-29.1096888385212));
#72269=CARTESIAN_POINT('',(0.,26.8018655926851,-33.3167260852698));
#72270=CARTESIAN_POINT('',(0.,19.7140853569221,-20.7664932002776));
#72271=CARTESIAN_POINT('',(0.138207714141623,26.7099230322463,-33.3938750538235));
#72272=CARTESIAN_POINT('',(1.46228393816674,25.8290824872081,-34.132988030291));
#72273=CARTESIAN_POINT('',(0.600000000000001,26.1673599741116,-33.234910440458));
#72274=CARTESIAN_POINT('Ctrl Pts',(0.600000000000008,26.1673599741116,-33.234910440458));
#72275=CARTESIAN_POINT('Ctrl Pts',(0.370217470904163,26.4376444612402,-33.3145607080699));
#72276=CARTESIAN_POINT('Ctrl Pts',(0.138207714141623,26.7099230322463,-33.3938750538235));
#72277=CARTESIAN_POINT('',(1.67735469196904,25.4310730087083,-33.8016349549212));
#72278=CARTESIAN_POINT('Origin',(8.1449754609635,0.,0.));
#72279=CARTESIAN_POINT('',(1.90339248332146,23.1273809239214,-30.1149569673582));
#72280=CARTESIAN_POINT('Origin',(0.,29.1096888385212,-24.4259291680885));
#72281=CARTESIAN_POINT('',(0.,32.1800738014028,-28.156475035514));
#72282=CARTESIAN_POINT('',(0.,24.710407536182,-19.0807620699926));
#72283=CARTESIAN_POINT('',(0.13820771414163,32.1029248328491,-28.2484175959528));
#72284=CARTESIAN_POINT('',(1.46228393816674,31.3638118563816,-29.129258140991));
#72285=CARTESIAN_POINT('',(0.600000000000001,31.5410006112756,-28.1860830985703));
#72286=CARTESIAN_POINT('Ctrl Pts',(0.600000000000009,31.5410006112756,-28.1860830985703));
#72287=CARTESIAN_POINT('Ctrl Pts',(0.370217470894748,31.8210099935517,-28.2175888910039));
#72288=CARTESIAN_POINT('Ctrl Pts',(0.13820771414163,32.1029248328491,-28.2484175959528));
#72289=CARTESIAN_POINT('',(1.67735469196904,30.9143101784803,-28.872052684018));
#72290=CARTESIAN_POINT('Origin',(8.1449754609635,0.,0.));
#72291=CARTESIAN_POINT('',(1.90339248332146,28.0054314386442,-25.6414155514355));
#72292=CARTESIAN_POINT('Origin',(0.,32.9089653438087,-19.));
#72293=CARTESIAN_POINT('',(0.,36.580506751568,-22.1407037396679));
#72294=CARTESIAN_POINT('',(0.,29.3974942757438,-15.9962233595133));
#72295=CARTESIAN_POINT('',(0.138207714141626,36.5204955072696,-22.2446462638181));
#72296=CARTESIAN_POINT('',(1.46228393816674,35.9455676731535,-23.2404504831928));
#72297=CARTESIAN_POINT('',(0.600000000000001,35.9562839053824,-22.2808358845789));
#72298=CARTESIAN_POINT('Ctrl Pts',(0.600000000000009,35.9562839053824,-22.2808358845789));
#72299=CARTESIAN_POINT('Ctrl Pts',(0.370217470898111,36.237510239402,-22.2632399142706));
#72300=CARTESIAN_POINT('Ctrl Pts',(0.138207714141626,36.5204955072696,-22.2446462638181));
#72301=CARTESIAN_POINT('',(1.67735469196904,35.4582316768749,-23.0652077022745));
#72302=CARTESIAN_POINT('Origin',(8.1449754609635,0.,0.));
#72303=CARTESIAN_POINT('',(1.90339248332146,32.0325510905359,-20.3887726991648));
#72304=CARTESIAN_POINT('Origin',(0.,35.7083195898645,-12.9967654463754));
#72305=CARTESIAN_POINT('',(0.,39.8694595147163,-15.4521983644287));
#72306=CARTESIAN_POINT('',(0.,33.3431191925968,-11.6010923812716));
#72307=CARTESIAN_POINT('',(0.138207714141623,39.8284094059641,-15.5649826112914));
#72308=CARTESIAN_POINT('',(1.46228393816674,39.4351356055115,-16.6454934976982));
#72309=CARTESIAN_POINT('',(0.600000000000001,39.2790537077817,-15.6985967468815));
#72310=CARTESIAN_POINT('Ctrl Pts',(0.600000000000009,39.2790537077817,-15.6985967468815));
#72311=CARTESIAN_POINT('Ctrl Pts',(0.370217470896577,39.552952073699,-15.6324336584852));
#72312=CARTESIAN_POINT('Ctrl Pts',(0.138207714141623,39.8284094059641,-15.5649826112914));
#72313=CARTESIAN_POINT('',(1.67735469196904,38.9247727484987,-16.5575380560557));
#72314=CARTESIAN_POINT('Origin',(8.1449754609635,0.,0.));
#72315=CARTESIAN_POINT('',(1.90339248332146,35.0863778867947,-14.5166273056467));
#72316=CARTESIAN_POINT('Origin',(0.,37.4226946144639,-6.59863075134336));
#72317=CARTESIAN_POINT('',(0.,41.9469989254299,-8.29418576107603));
#72318=CARTESIAN_POINT('',(0.,36.1531791768932,-6.12285964662596));
#72319=CARTESIAN_POINT('',(0.138207714141624,41.9261572390061,-8.41238483838185));
#72320=CARTESIAN_POINT('',(1.46228393816674,41.7264868976375,-9.54477161530208));
#72321=CARTESIAN_POINT('',(0.600000000000001,41.4083493394303,-8.63936369090333));
#72322=CARTESIAN_POINT('Ctrl Pts',(0.600000000000009,41.4083493394303,-8.63936369090333));
#72323=CARTESIAN_POINT('Ctrl Pts',(0.370217470894459,41.6665974739965,-8.52664381637888));
#72324=CARTESIAN_POINT('Ctrl Pts',(0.138207714141624,41.9261572390061,-8.41238483838185));
#72325=CARTESIAN_POINT('',(1.67735469196904,41.2086042970448,-9.54677599452213));
#72326=CARTESIAN_POINT('Origin',(8.1449754609635,0.,0.));
#72327=CARTESIAN_POINT('',(1.90339248332146,37.0741228455271,-8.20340153721441));
#72328=CARTESIAN_POINT('Origin',(35.,52.,0.));
#72329=CARTESIAN_POINT('',(35.,42.75,-0.884158520433536));
#72330=CARTESIAN_POINT('',(35.,44.9140105592676,-1.28696449396714));
#72331=CARTESIAN_POINT('',(35.,42.75,0.));
#72332=CARTESIAN_POINT('Origin',(35.,52.,0.));
#72333=CARTESIAN_POINT('',(35.,42.2540639571139,6.55273342944652));
#72334=CARTESIAN_POINT('',(35.,44.8929942217219,6.52766396709994));
#72335=CARTESIAN_POINT('',(35.,42.8845273710551,2.97719773202758));
#72336=CARTESIAN_POINT('Origin',(35.,52.,0.));
#72337=CARTESIAN_POINT('',(35.,40.4742595624789,13.790523889916));
#72338=CARTESIAN_POINT('',(35.,42.7301436553725,14.1662371923646));
#72339=CARTESIAN_POINT('',(35.,43.2132817780509,6.26512220124733));
#72340=CARTESIAN_POINT('Origin',(35.,52.,0.));
#72341=CARTESIAN_POINT('',(35.,37.4646652720015,20.6092962603321));
#72342=CARTESIAN_POINT('',(35.,38.554281614855,20.9942020999154));
#72343=CARTESIAN_POINT('',(35.,43.5225860117848,10.1166697508023));
#72344=CARTESIAN_POINT('Origin',(35.,52.,0.));
#72345=CARTESIAN_POINT('',(35.,33.3167260852698,26.8018655926851));
#72346=CARTESIAN_POINT('',(35.,32.689238504957,26.4474901710748));
#72347=CARTESIAN_POINT('',(35.,43.4909736336662,14.6766695249408));
#72348=CARTESIAN_POINT('Origin',(35.,52.,0.));
#72349=CARTESIAN_POINT('',(35.,28.156475035514,32.1800738014028));
#72350=CARTESIAN_POINT('',(35.,25.6202580076353,30.0926681235906));
#72351=CARTESIAN_POINT('',(35.,42.7365966237696,19.9458991541776));
#72352=CARTESIAN_POINT('Origin',(35.,52.,0.));
#72353=CARTESIAN_POINT('',(35.,22.1407037396679,36.580506751568));
#72354=CARTESIAN_POINT('',(35.,17.9422199667173,31.672400702755));
#72355=CARTESIAN_POINT('',(35.,40.875,25.764255762587));
#72356=CARTESIAN_POINT('Origin',(35.,52.,0.));
#72357=CARTESIAN_POINT('',(35.,15.4521983644287,39.8694595147163));
#72358=CARTESIAN_POINT('',(35.,10.2957205060146,31.1309491972475));
#72359=CARTESIAN_POINT('',(35.,37.5799388877191,31.8156206126726));
#72360=CARTESIAN_POINT('Origin',(35.,52.,0.));
#72361=CARTESIAN_POINT('',(35.,8.29418576107603,41.9469989254299));
#72362=CARTESIAN_POINT('',(35.,3.29848110862957,28.6167985098503));
#72363=CARTESIAN_POINT('',(35.,32.6394636654781,37.6542695780382));
#72364=CARTESIAN_POINT('Origin',(35.,52.,0.));
#72365=CARTESIAN_POINT('',(35.,0.884158520433538,42.75));
#72366=CARTESIAN_POINT('',(35.,-2.51990383326145,24.4622203695749));
#72367=CARTESIAN_POINT('',(35.,26.,42.75));
#72368=CARTESIAN_POINT('Origin',(35.,52.,0.));
#72369=CARTESIAN_POINT('',(35.,-6.55273342944652,42.2540639571139));
#72370=CARTESIAN_POINT('',(35.,-6.77229176400553,19.1423144546885));
#72371=CARTESIAN_POINT('',(35.,17.7925444749555,46.5467933045056));
#72372=CARTESIAN_POINT('Origin',(35.,52.,0.));
#72373=CARTESIAN_POINT('',(35.,-13.790523889916,40.4742595624789));
#72374=CARTESIAN_POINT('',(35.,-9.25112687675228,13.2184944708942));
#72375=CARTESIAN_POINT('',(35.,8.33721663337438,48.5280984645226));
#72376=CARTESIAN_POINT('Origin',(35.,52.,0.));
#72377=CARTESIAN_POINT('',(35.,-20.6092962603321,37.4646652720015));
#72378=CARTESIAN_POINT('',(35.,-9.94419665558418,7.27321159056857));
#72379=CARTESIAN_POINT('',(35.,-1.87499999999998,48.2809162609825));
#72380=CARTESIAN_POINT('Origin',(35.,52.,0.));
#72381=CARTESIAN_POINT('',(35.,-26.8018655926851,33.3167260852698));
#72382=CARTESIAN_POINT('',(35.,-9.02739147575637,1.84371448565053));
#72383=CARTESIAN_POINT('',(35.,-12.2217440044295,45.550900732495));
#72384=CARTESIAN_POINT('Origin',(35.,52.,0.));
#72385=CARTESIAN_POINT('',(35.,-32.1800738014028,28.156475035514));
#72386=CARTESIAN_POINT('',(35.,-6.8356053136496,-2.63728643807825));
#72387=CARTESIAN_POINT('',(35.,-22.0058262530064,40.2816711032583));
#72388=CARTESIAN_POINT('Origin',(35.,52.,0.));
#72389=CARTESIAN_POINT('',(35.,-36.580506751568,22.1407037396679));
#72390=CARTESIAN_POINT('',(35.,-3.8155269311951,-5.88705986787639));
#72391=CARTESIAN_POINT('',(35.,-30.5225860117848,32.6333302491977));
#72392=CARTESIAN_POINT('Origin',(35.,52.,0.));
#72393=CARTESIAN_POINT('',(35.,-39.8694595147163,15.4521983644287));
#72394=CARTESIAN_POINT('',(35.,-0.466222705023521,-7.79912374625847));
#72395=CARTESIAN_POINT('',(35.,-37.1304372991443,22.9776000530974));
#72396=CARTESIAN_POINT('Origin',(35.,52.,0.));
#72397=CARTESIAN_POINT('',(35.,-41.9469989254299,8.29418576107603));
#72398=CARTESIAN_POINT('',(35.,2.72515398447831,-8.44741415260574));
#72399=CARTESIAN_POINT('',(35.,-41.3165355114887,11.869721458495));
#72400=CARTESIAN_POINT('Origin',(35.,52.,0.));
#72401=CARTESIAN_POINT('',(35.,-42.75,0.884158520433541));
#72402=CARTESIAN_POINT('',(35.,5.34464795765368,-8.06811364356874));
#72403=CARTESIAN_POINT('',(35.,-42.75,8.41944674413805E-15));
#72404=CARTESIAN_POINT('Origin',(35.,52.,0.));
#72405=CARTESIAN_POINT('',(35.,-42.2540639571139,-6.55273342944651));
#72406=CARTESIAN_POINT('',(35.,7.10231334221714,-7.02161199697211));
#72407=CARTESIAN_POINT('',(35.,-41.3165355114887,-11.8697214584949));
#72408=CARTESIAN_POINT('Origin',(35.,52.,0.));
#72409=CARTESIAN_POINT('',(35.,-40.4742595624789,-13.790523889916));
#72410=CARTESIAN_POINT('',(35.,7.86639521349345,-5.73947769227399));
#72411=CARTESIAN_POINT('',(35.,-37.1304372991443,-22.9776000530973));
#72412=CARTESIAN_POINT('Origin',(35.,52.,0.));
#72413=CARTESIAN_POINT('',(35.,-37.4646652720015,-20.6092962603321));
#72414=CARTESIAN_POINT('',(35.,7.67678296510018,-4.66312663129778));
#72415=CARTESIAN_POINT('',(35.,-30.5225860117848,-32.6333302491977));
#72416=CARTESIAN_POINT('Origin',(35.,52.,0.));
#72417=CARTESIAN_POINT('',(35.,-33.3167260852698,-26.8018655926851));
#72418=CARTESIAN_POINT('',(35.,6.73618681903107,-4.18186745644989));
#72419=CARTESIAN_POINT('',(35.,-22.0058262530064,-40.2816711032583));
#72420=CARTESIAN_POINT('Origin',(35.,52.,0.));
#72421=CARTESIAN_POINT('',(35.,-28.156475035514,-32.1800738014028));
#72422=CARTESIAN_POINT('',(35.,5.38022362813726,-4.57806086793601));
#72423=CARTESIAN_POINT('',(35.,-12.2217440044295,-45.550900732495));
#72424=CARTESIAN_POINT('Origin',(35.,52.,0.));
#72425=CARTESIAN_POINT('',(35.,-22.1407037396679,-36.580506751568));
#72426=CARTESIAN_POINT('',(35.,4.03018609631655,-5.98624709660142));
#72427=CARTESIAN_POINT('',(35.,-1.87500000000003,-48.2809162609824));
#72428=CARTESIAN_POINT('Origin',(35.,52.,0.));
#72429=CARTESIAN_POINT('',(35.,-15.4521983644287,-39.8694595147163));
#72430=CARTESIAN_POINT('',(35.,3.13439725403449,-8.37137845275046));
#72431=CARTESIAN_POINT('',(35.,8.33721663337434,-48.5280984645226));
#72432=CARTESIAN_POINT('Origin',(35.,52.,0.));
#72433=CARTESIAN_POINT('',(35.,-8.29418576107602,-41.9469989254299));
#72434=CARTESIAN_POINT('',(35.,3.10546165827712,-11.5289507542864));
#72435=CARTESIAN_POINT('',(35.,17.7925444749555,-46.5467933045056));
#72436=CARTESIAN_POINT('Origin',(35.,52.,0.));
#72437=CARTESIAN_POINT('',(35.,-0.884158520433544,-42.75));
#72438=CARTESIAN_POINT('',(35.,4.26124531634016,-15.107142232039));
#72439=CARTESIAN_POINT('',(35.,26.,-42.75));
#72440=CARTESIAN_POINT('Origin',(35.,52.,0.));
#72441=CARTESIAN_POINT('',(35.,6.55273342944651,-42.2540639571139));
#72442=CARTESIAN_POINT('',(35.,6.7769842000665,-18.6483664248163));
#72443=CARTESIAN_POINT('',(35.,32.6394636654781,-37.6542695780382));
#72444=CARTESIAN_POINT('Origin',(35.,52.,0.));
#72445=CARTESIAN_POINT('',(35.,13.7905238899159,-40.4742595624789));
#72446=CARTESIAN_POINT('',(35.,10.6545880078863,-21.6452539709848));
#72447=CARTESIAN_POINT('',(35.,37.579938887719,-31.8156206126726));
#72448=CARTESIAN_POINT('Origin',(35.,52.,0.));
#72449=CARTESIAN_POINT('',(35.,20.6092962603321,-37.4646652720015));
#72450=CARTESIAN_POINT('',(35.,15.713132075629,-23.6042870591862));
#72451=CARTESIAN_POINT('',(35.,40.875,-25.764255762587));
#72452=CARTESIAN_POINT('Origin',(35.,52.,0.));
#72453=CARTESIAN_POINT('',(35.,26.8018655926851,-33.3167260852698));
#72454=CARTESIAN_POINT('',(35.,21.6019661517683,-24.1093372002754));
#72455=CARTESIAN_POINT('',(35.,42.7365966237696,-19.9458991541776));
#72456=CARTESIAN_POINT('Origin',(35.,52.,0.));
#72457=CARTESIAN_POINT('',(35.,32.1800738014028,-28.156475035514));
#72458=CARTESIAN_POINT('',(35.,27.835123677877,-22.8773208175763));
#72459=CARTESIAN_POINT('',(35.,43.4909736336662,-14.6766695249409));
#72460=CARTESIAN_POINT('Origin',(35.,52.,0.));
#72461=CARTESIAN_POINT('',(35.,36.580506751568,-22.1407037396679));
#72462=CARTESIAN_POINT('',(35.,33.8431208681613,-19.7990937382771));
#72463=CARTESIAN_POINT('',(35.,43.5225860117848,-10.1166697508023));
#72464=CARTESIAN_POINT('Origin',(35.,52.,0.));
#72465=CARTESIAN_POINT('',(35.,39.8694595147163,-15.4521983644287));
#72466=CARTESIAN_POINT('',(35.,39.0361049449744,-14.9604469982386));
#72467=CARTESIAN_POINT('',(35.,43.2132817780509,-6.26512220124734));
#72468=CARTESIAN_POINT('Origin',(35.,52.,0.));
#72469=CARTESIAN_POINT('',(35.,41.9469989254299,-8.29418576107602));
#72470=CARTESIAN_POINT('',(35.,42.870903248615,-8.64043360295818));
#72471=CARTESIAN_POINT('',(35.,42.8845273710551,-2.97719773202758));
#72472=CARTESIAN_POINT('Origin',(33.1,37.1361751213135,-8.2235635438135));
#72473=CARTESIAN_POINT('',(33.3226453080309,41.2086042970448,-9.54677599452213));
#72474=CARTESIAN_POINT('',(33.0964948753266,37.0720625104951,-8.20273209378168));
#72475=CARTESIAN_POINT('',(34.4,41.4083493394303,-8.63936369090333));
#72476=CARTESIAN_POINT('Origin',(26.8550245390365,0.,0.));
#72477=CARTESIAN_POINT('',(34.8617922858584,41.9261572390061,-8.41238483838185));
#72478=CARTESIAN_POINT('Ctrl Pts',(34.8617922858584,41.9261572390061,-8.41238483838185));
#72479=CARTESIAN_POINT('Ctrl Pts',(34.6297825291011,41.6665974739915,-8.52664381638108));
#72480=CARTESIAN_POINT('Ctrl Pts',(34.4,41.4083493394303,-8.63936369090333));
#72481=CARTESIAN_POINT('',(35.4377160618333,42.013006390788,-7.91983882283194));
#72482=CARTESIAN_POINT('Origin',(33.1,35.1439863533772,-14.5472582706722));
#72483=CARTESIAN_POINT('',(33.3226453080309,38.9247727484987,-16.5575380560557));
#72484=CARTESIAN_POINT('',(33.0964948753266,35.0844651005135,-14.5156102591403));
#72485=CARTESIAN_POINT('',(34.4,39.2790537077817,-15.6985967468815));
#72486=CARTESIAN_POINT('Origin',(26.8550245390365,0.,0.));
#72487=CARTESIAN_POINT('',(34.8617922858584,39.8284094059641,-15.5649826112914));
#72488=CARTESIAN_POINT('Ctrl Pts',(34.8617922858584,39.8284094059641,-15.5649826112914));
#72489=CARTESIAN_POINT('Ctrl Pts',(34.6297825291059,39.5529520737019,-15.6324336584845));
#72490=CARTESIAN_POINT('Ctrl Pts',(34.4,39.2790537077817,-15.6985967468815));
#72491=CARTESIAN_POINT('',(35.4377160618333,39.9994688419988,-15.0950006734014));
#72492=CARTESIAN_POINT('Origin',(33.1,32.0839653438087,-20.4289419162443));
#72493=CARTESIAN_POINT('',(33.3226453080309,35.4582316768749,-23.0652077022745));
#72494=CARTESIAN_POINT('',(33.0964948753266,32.0308439720488,-20.3874389520281));
#72495=CARTESIAN_POINT('',(34.4,35.9562839053824,-22.2808358845789));
#72496=CARTESIAN_POINT('Origin',(26.8550245390365,0.,0.));
#72497=CARTESIAN_POINT('',(34.8617922858584,36.5204955072696,-22.2446462638181));
#72498=CARTESIAN_POINT('Ctrl Pts',(34.8617922858584,36.5204955072696,-22.2446462638181));
#72499=CARTESIAN_POINT('Ctrl Pts',(34.6297825291007,36.2375102394006,-22.2632399142707));
#72500=CARTESIAN_POINT('Ctrl Pts',(34.4,35.9562839053824,-22.2808358845789));
#72501=CARTESIAN_POINT('',(35.4377160618333,36.7705676731535,-21.8115085669485));
#72502=CARTESIAN_POINT('Origin',(33.1,28.0490892825384,-25.6899024992348));
#72503=CARTESIAN_POINT('',(33.3226453080309,30.9143101784803,-28.872052684018));
#72504=CARTESIAN_POINT('',(33.0964948753266,28.0039818578826,-25.6398056289004));
#72505=CARTESIAN_POINT('',(34.4,31.5410006112756,-28.1860830985704));
#72506=CARTESIAN_POINT('Origin',(26.8550245390365,0.,0.));
#72507=CARTESIAN_POINT('',(34.8617922858584,32.1029248328491,-28.2484175959528));
#72508=CARTESIAN_POINT('Ctrl Pts',(34.8617922858584,32.1029248328491,-28.2484175959528));
#72509=CARTESIAN_POINT('Ctrl Pts',(34.629782529101,31.8210099935466,-28.2175888910033));
#72510=CARTESIAN_POINT('Ctrl Pts',(34.4,31.5410006112756,-28.1860830985704));
#72511=CARTESIAN_POINT('',(35.4377160618333,32.4244114123644,-27.8652848098447));
#72512=CARTESIAN_POINT('Origin',(33.1,23.1619558369422,-30.170288394504));
#72513=CARTESIAN_POINT('',(33.3226453080309,25.4310730087083,-33.8016349549212));
#72514=CARTESIAN_POINT('',(33.0964948753266,23.1262329256631,-30.1131197861062));
#72515=CARTESIAN_POINT('',(34.4,26.1673599741116,-33.234910440458));
#72516=CARTESIAN_POINT('Origin',(26.8550245390365,0.,0.));
#72517=CARTESIAN_POINT('',(34.8617922858584,26.7099230322463,-33.3938750538235));
#72518=CARTESIAN_POINT('Ctrl Pts',(34.8617922858584,26.7099230322463,-33.3938750538235));
#72519=CARTESIAN_POINT('Ctrl Pts',(34.6297825291025,26.4376444612481,-33.3145607080723));
#72520=CARTESIAN_POINT('Ctrl Pts',(34.4,26.1673599741116,-33.234910440458));
#72521=CARTESIAN_POINT('',(35.4377160618333,27.0930558183544,-33.0723884743082));
#72522=CARTESIAN_POINT('Origin',(33.1,17.5710580837557,-33.7339653438087));
#72523=CARTESIAN_POINT('',(33.3226453080309,19.1751255543105,-37.7041716521717));
#72524=CARTESIAN_POINT('',(33.0964948753266,17.5458051084359,-33.6714620365851));
#72525=CARTESIAN_POINT('',(34.4,19.9986373454573,-37.2739118462884));
#72526=CARTESIAN_POINT('Origin',(26.8550245390365,0.,0.));
#72527=CARTESIAN_POINT('',(34.8617922858584,20.505353736182,-37.5246765162999));
#72528=CARTESIAN_POINT('Ctrl Pts',(34.8617922858584,20.505353736182,-37.5246765162999));
#72529=CARTESIAN_POINT('Ctrl Pts',(34.6297825291059,20.25098448009,-37.3992864560092));
#72530=CARTESIAN_POINT('Ctrl Pts',(34.4,19.9986373454573,-37.2739118462884));
#72531=CARTESIAN_POINT('',(35.4377160618333,20.9384914330515,-37.274604350416));
#72532=CARTESIAN_POINT('Origin',(33.1,11.4462726220786,-36.2726528263519));
#72533=CARTESIAN_POINT('',(33.3226453080309,12.3365516130267,-40.4610861730024));
#72534=CARTESIAN_POINT('',(33.0964948753266,11.4322568815947,-36.2067139516643));
#72535=CARTESIAN_POINT('',(34.4,13.22226624086,-40.1803643021789));
#72536=CARTESIAN_POINT('Origin',(26.8550245390365,0.,0.));
#72537=CARTESIAN_POINT('',(34.8617922858584,13.6777396430533,-40.515309671231));
#72538=CARTESIAN_POINT('Ctrl Pts',(34.8617922858584,13.6777396430533,-40.515309671231));
#72539=CARTESIAN_POINT('Ctrl Pts',(34.6297825291018,13.449008582989,-40.3476538099283));
#72540=CARTESIAN_POINT('Ctrl Pts',(34.4,13.22226624086,-40.1803643021789));
#72541=CARTESIAN_POINT('',(35.4377160618333,14.1477215809433,-40.3442502351963));
#72542=CARTESIAN_POINT('Origin',(33.1,4.9736979588732,-37.7092141076143));
#72543=CARTESIAN_POINT('',(33.3226453080309,5.1231377935775,-41.9886110647639));
#72544=CARTESIAN_POINT('',(33.0964948753266,4.97134531440727,-37.6418431848034));
#72545=CARTESIAN_POINT('',(34.4,6.04414326732375,-41.8659567209931));
#72546=CARTESIAN_POINT('Origin',(26.8550245390365,0.,0.));
#72547=CARTESIAN_POINT('',(34.8617922858584,6.43453435214068,-42.2749056435377));
#72548=CARTESIAN_POINT('Ctrl Pts',(34.8617922858584,6.43453435214068,-42.2749056435377));
#72549=CARTESIAN_POINT('Ctrl Pts',(34.6297825291057,6.23839136562832,-42.0700781197363));
#72550=CARTESIAN_POINT('Ctrl Pts',(34.4,6.04414326732374,-41.8659567209931));
#72551=CARTESIAN_POINT('',(35.4377160618333,6.92708036769059,-42.1880564917558));
#72552=CARTESIAN_POINT('Origin',(33.1,-1.65000000000001,-38.));
#72553=CARTESIAN_POINT('',(33.3226453080309,-2.24593997529678,-42.240333256585));
#72554=CARTESIAN_POINT('',(33.0964948753266,-1.64061806453627,-37.933244060464));
#72555=CARTESIAN_POINT('',(34.4,-1.31762794090605,-42.2794732300362));
#72556=CARTESIAN_POINT('Origin',(26.8550245390365,0.,0.));
#72557=CARTESIAN_POINT('',(34.8617922858584,-1.00418100903022,-42.75));
#72558=CARTESIAN_POINT('Ctrl Pts',(34.8617922858584,-1.00418100903022,-42.75));
#72559=CARTESIAN_POINT('Ctrl Pts',(34.6297825291027,-1.16177621660441,-42.514224394357));
#72560=CARTESIAN_POINT('Ctrl Pts',(34.4,-1.31762794090605,-42.2794732300361));
#72561=CARTESIAN_POINT('',(35.4377160618333,-0.504036677262553,-42.75));
#72562=CARTESIAN_POINT('Origin',(33.1,-8.2235635438135,-37.1361751213135));
#72563=CARTESIAN_POINT('',(33.3226453080309,-9.54677599452213,-41.2086042970448));
#72564=CARTESIAN_POINT('',(33.0964948753266,-8.20273209378168,-37.0720625104951));
#72565=CARTESIAN_POINT('',(34.4,-8.63936369090332,-41.4083493394303));
#72566=CARTESIAN_POINT('Origin',(26.8550245390365,0.,0.));
#72567=CARTESIAN_POINT('',(34.8617922858584,-8.41238483838184,-41.9261572390061));
#72568=CARTESIAN_POINT('Ctrl Pts',(34.8617922858584,-8.41238483838184,-41.9261572390061));
#72569=CARTESIAN_POINT('Ctrl Pts',(34.6297825291012,-8.526643816381,-41.6665974739917));
#72570=CARTESIAN_POINT('Ctrl Pts',(34.4,-8.63936369090332,-41.4083493394303));
#72571=CARTESIAN_POINT('',(35.4377160618333,-7.91983882283194,-42.013006390788));
#72572=CARTESIAN_POINT('Origin',(33.1,-14.5472582706722,-35.1439863533772));
#72573=CARTESIAN_POINT('',(33.3226453080309,-16.5575380560557,-38.9247727484987));
#72574=CARTESIAN_POINT('',(33.0964948753266,-14.5156102591403,-35.0844651005135));
#72575=CARTESIAN_POINT('',(34.4,-15.6985967468815,-39.2790537077817));
#72576=CARTESIAN_POINT('Origin',(26.8550245390365,0.,0.));
#72577=CARTESIAN_POINT('',(34.8617922858584,-15.5649826112914,-39.8284094059641));
#72578=CARTESIAN_POINT('Ctrl Pts',(34.8617922858584,-15.5649826112914,-39.8284094059641));
#72579=CARTESIAN_POINT('Ctrl Pts',(34.6297825291,-15.6324336584862,-39.552952073695));
#72580=CARTESIAN_POINT('Ctrl Pts',(34.4,-15.6985967468815,-39.2790537077817));
#72581=CARTESIAN_POINT('',(35.4377160618333,-15.0950006734014,-39.9994688419988));
#72582=CARTESIAN_POINT('Origin',(33.1,-20.4289419162443,-32.0839653438087));
#72583=CARTESIAN_POINT('',(33.3226453080309,-23.0652077022745,-35.4582316768749));
#72584=CARTESIAN_POINT('',(33.0964948753266,-20.3874389520281,-32.0308439720488));
#72585=CARTESIAN_POINT('',(34.4,-22.2808358845789,-35.9562839053824));
#72586=CARTESIAN_POINT('Origin',(26.8550245390365,0.,0.));
#72587=CARTESIAN_POINT('',(34.8617922858584,-22.2446462638181,-36.5204955072696));
#72588=CARTESIAN_POINT('Ctrl Pts',(34.8617922858584,-22.2446462638181,-36.5204955072696));
#72589=CARTESIAN_POINT('Ctrl Pts',(34.629782529101,-22.2632399142707,-36.237510239401));
#72590=CARTESIAN_POINT('Ctrl Pts',(34.4,-22.2808358845789,-35.9562839053824));
#72591=CARTESIAN_POINT('',(35.4377160618333,-21.8115085669485,-36.7705676731535));
#72592=CARTESIAN_POINT('Origin',(33.1,-25.6899024992348,-28.0490892825384));
#72593=CARTESIAN_POINT('',(33.3226453080309,-28.872052684018,-30.9143101784803));
#72594=CARTESIAN_POINT('',(33.0964948753266,-25.6398056289004,-28.0039818578826));
#72595=CARTESIAN_POINT('',(34.4,-28.1860830985704,-31.5410006112756));
#72596=CARTESIAN_POINT('Origin',(26.8550245390365,0.,0.));
#72597=CARTESIAN_POINT('',(34.8617922858584,-28.2484175959528,-32.1029248328491));
#72598=CARTESIAN_POINT('Ctrl Pts',(34.8617922858584,-28.2484175959528,-32.1029248328491));
#72599=CARTESIAN_POINT('Ctrl Pts',(34.6297825291016,-28.2175888910034,-31.8210099935474));
#72600=CARTESIAN_POINT('Ctrl Pts',(34.4,-28.1860830985703,-31.5410006112756));
#72601=CARTESIAN_POINT('',(35.4377160618333,-27.8652848098447,-32.4244114123644));
#72602=CARTESIAN_POINT('Origin',(33.1,-30.170288394504,-23.1619558369422));
#72603=CARTESIAN_POINT('',(33.3226453080309,-33.8016349549212,-25.4310730087083));
#72604=CARTESIAN_POINT('',(33.0964948753266,-30.1131197861062,-23.1262329256631));
#72605=CARTESIAN_POINT('',(34.4,-33.234910440458,-26.1673599741116));
#72606=CARTESIAN_POINT('Origin',(26.8550245390365,0.,0.));
#72607=CARTESIAN_POINT('',(34.8617922858584,-33.3938750538235,-26.7099230322464));
#72608=CARTESIAN_POINT('Ctrl Pts',(34.8617922858584,-33.3938750538235,-26.7099230322464));
#72609=CARTESIAN_POINT('Ctrl Pts',(34.6297825291001,-33.3145607080714,-26.4376444612452));
#72610=CARTESIAN_POINT('Ctrl Pts',(34.4,-33.234910440458,-26.1673599741116));
#72611=CARTESIAN_POINT('',(35.4377160618333,-33.0723884743082,-27.0930558183544));
#72612=CARTESIAN_POINT('Origin',(33.1,-33.7339653438087,-17.5710580837557));
#72613=CARTESIAN_POINT('',(33.3226453080309,-37.7041716521717,-19.1751255543105));
#72614=CARTESIAN_POINT('',(33.0964948753266,-33.6714620365851,-17.5458051084359));
#72615=CARTESIAN_POINT('',(34.4,-37.2739118462885,-19.9986373454573));
#72616=CARTESIAN_POINT('Origin',(26.8550245390365,0.,0.));
#72617=CARTESIAN_POINT('',(34.8617922858584,-37.5246765162999,-20.5053537361819));
#72618=CARTESIAN_POINT('Ctrl Pts',(34.8617922858584,-37.5246765162999,-20.5053537361819));
#72619=CARTESIAN_POINT('Ctrl Pts',(34.6297825291016,-37.3992864560069,-20.2509844800853));
#72620=CARTESIAN_POINT('Ctrl Pts',(34.4,-37.2739118462884,-19.9986373454572));
#72621=CARTESIAN_POINT('',(35.4377160618333,-37.274604350416,-20.9384914330515));
#72622=CARTESIAN_POINT('Origin',(33.1,-36.2726528263519,-11.4462726220787));
#72623=CARTESIAN_POINT('',(33.3226453080309,-40.4610861730024,-12.3365516130268));
#72624=CARTESIAN_POINT('',(33.0964948753266,-36.2067139516643,-11.4322568815947));
#72625=CARTESIAN_POINT('',(34.4,-40.1803643021789,-13.22226624086));
#72626=CARTESIAN_POINT('Origin',(26.8550245390365,0.,0.));
#72627=CARTESIAN_POINT('',(34.8617922858584,-40.515309671231,-13.6777396430533));
#72628=CARTESIAN_POINT('Ctrl Pts',(34.8617922858584,-40.515309671231,-13.6777396430533));
#72629=CARTESIAN_POINT('Ctrl Pts',(34.6297825291007,-40.3476538099275,-13.4490085829879));
#72630=CARTESIAN_POINT('Ctrl Pts',(34.4,-40.1803643021789,-13.22226624086));
#72631=CARTESIAN_POINT('',(35.4377160618333,-40.3442502351963,-14.1477215809433));
#72632=CARTESIAN_POINT('Origin',(33.1,-37.7092141076143,-4.9736979588732));
#72633=CARTESIAN_POINT('',(33.3226453080309,-41.9886110647639,-5.12313779357751));
#72634=CARTESIAN_POINT('',(33.0964948753266,-37.6418431848034,-4.97134531440727));
#72635=CARTESIAN_POINT('',(34.4,-41.8659567209931,-6.04414326732375));
#72636=CARTESIAN_POINT('Origin',(26.8550245390365,0.,0.));
#72637=CARTESIAN_POINT('',(34.8617922858584,-42.2749056435377,-6.43453435214069));
#72638=CARTESIAN_POINT('Ctrl Pts',(34.8617922858584,-42.2749056435377,-6.43453435214069));
#72639=CARTESIAN_POINT('Ctrl Pts',(34.6297825291043,-42.0700781197351,-6.23839136562716));
#72640=CARTESIAN_POINT('Ctrl Pts',(34.4,-41.8659567209931,-6.04414326732375));
#72641=CARTESIAN_POINT('',(35.4377160618333,-42.1880564917558,-6.92708036769059));
#72642=CARTESIAN_POINT('Origin',(33.1,-38.,1.65));
#72643=CARTESIAN_POINT('',(33.3226453080309,-42.240333256585,2.24593997529678));
#72644=CARTESIAN_POINT('',(33.0964948753266,-37.933244060464,1.64061806453627));
#72645=CARTESIAN_POINT('',(34.4,-42.2794732300362,1.31762794090605));
#72646=CARTESIAN_POINT('Origin',(26.8550245390365,0.,0.));
#72647=CARTESIAN_POINT('',(34.8617922858584,-42.75,1.00418100903022));
#72648=CARTESIAN_POINT('Ctrl Pts',(34.8617922858584,-42.75,1.00418100903022));
#72649=CARTESIAN_POINT('Ctrl Pts',(34.629782529102,-42.5142243943562,1.16177621660493));
#72650=CARTESIAN_POINT('Ctrl Pts',(34.4,-42.2794732300361,1.31762794090605));
#72651=CARTESIAN_POINT('',(35.4377160618333,-42.75,0.50403667726255));
#72652=CARTESIAN_POINT('Origin',(33.1,-37.1361751213135,8.22356354381351));
#72653=CARTESIAN_POINT('',(33.3226453080309,-41.2086042970448,9.54677599452215));
#72654=CARTESIAN_POINT('',(33.0964948753266,-37.072062510495,8.20273209378169));
#72655=CARTESIAN_POINT('',(34.4,-41.4083493394303,8.63936369090334));
#72656=CARTESIAN_POINT('Origin',(26.8550245390365,0.,0.));
#72657=CARTESIAN_POINT('',(34.8617922858584,-41.926157239006,8.41238483838188));
#72658=CARTESIAN_POINT('Ctrl Pts',(34.8617922858584,-41.926157239006,8.41238483838188));
#72659=CARTESIAN_POINT('Ctrl Pts',(34.6297825290997,-41.66659747399,8.52664381638178));
#72660=CARTESIAN_POINT('Ctrl Pts',(34.4,-41.4083493394303,8.63936369090334));
#72661=CARTESIAN_POINT('',(35.4377160618333,-42.013006390788,7.91983882283195));
#72662=CARTESIAN_POINT('Origin',(33.1,-35.1439863533772,14.5472582706722));
#72663=CARTESIAN_POINT('',(33.3226453080309,-38.9247727484987,16.5575380560557));
#72664=CARTESIAN_POINT('',(33.0964948753266,-35.0844651005135,14.5156102591403));
#72665=CARTESIAN_POINT('',(34.4,-39.2790537077817,15.6985967468815));
#72666=CARTESIAN_POINT('Origin',(26.8550245390365,0.,0.));
#72667=CARTESIAN_POINT('',(34.8617922858584,-39.8284094059642,15.5649826112914));
#72668=CARTESIAN_POINT('Ctrl Pts',(34.8617922858584,-39.8284094059642,15.5649826112914));
#72669=CARTESIAN_POINT('Ctrl Pts',(34.6297825291024,-39.5529520736977,15.6324336584855));
#72670=CARTESIAN_POINT('Ctrl Pts',(34.4,-39.2790537077817,15.6985967468815));
#72671=CARTESIAN_POINT('',(35.4377160618333,-39.9994688419988,15.0950006734014));
#72672=CARTESIAN_POINT('Origin',(33.1,-32.0839653438087,20.4289419162443));
#72673=CARTESIAN_POINT('',(33.3226453080309,-35.4582316768749,23.0652077022745));
#72674=CARTESIAN_POINT('',(33.0964948753266,-32.0308439720488,20.387438952028));
#72675=CARTESIAN_POINT('',(34.4,-35.9562839053824,22.2808358845789));
#72676=CARTESIAN_POINT('Origin',(26.8550245390365,0.,0.));
#72677=CARTESIAN_POINT('',(34.8617922858584,-36.5204955072696,22.2446462638181));
#72678=CARTESIAN_POINT('Ctrl Pts',(34.8617922858584,-36.5204955072696,22.2446462638181));
#72679=CARTESIAN_POINT('Ctrl Pts',(34.6297825291014,-36.2375102394014,22.2632399142706));
#72680=CARTESIAN_POINT('Ctrl Pts',(34.4,-35.9562839053824,22.2808358845789));
#72681=CARTESIAN_POINT('',(35.4377160618333,-36.7705676731535,21.8115085669485));
#72682=CARTESIAN_POINT('Origin',(33.1,-28.0490892825384,25.6899024992348));
#72683=CARTESIAN_POINT('',(33.3226453080309,-30.9143101784803,28.872052684018));
#72684=CARTESIAN_POINT('',(33.0964948753266,-28.0039818578826,25.6398056289004));
#72685=CARTESIAN_POINT('',(34.4,-31.5410006112756,28.1860830985704));
#72686=CARTESIAN_POINT('Origin',(26.8550245390365,0.,0.));
#72687=CARTESIAN_POINT('',(34.8617922858584,-32.1029248328491,28.2484175959528));
#72688=CARTESIAN_POINT('Ctrl Pts',(34.8617922858584,-32.1029248328491,28.2484175959528));
#72689=CARTESIAN_POINT('Ctrl Pts',(34.6297825291016,-31.8210099935474,28.2175888910034));
#72690=CARTESIAN_POINT('Ctrl Pts',(34.4,-31.5410006112756,28.1860830985703));
#72691=CARTESIAN_POINT('',(35.4377160618333,-32.4244114123644,27.8652848098447));
#72692=CARTESIAN_POINT('Origin',(33.1,-23.1619558369422,30.170288394504));
#72693=CARTESIAN_POINT('',(33.3226453080309,-25.4310730087083,33.8016349549212));
#72694=CARTESIAN_POINT('',(33.0964948753266,-23.1262329256631,30.1131197861062));
#72695=CARTESIAN_POINT('',(34.4,-26.1673599741116,33.234910440458));
#72696=CARTESIAN_POINT('Origin',(26.8550245390365,0.,0.));
#72697=CARTESIAN_POINT('',(34.8617922858584,-26.7099230322463,33.3938750538235));
#72698=CARTESIAN_POINT('Ctrl Pts',(34.8617922858584,-26.7099230322463,33.3938750538235));
#72699=CARTESIAN_POINT('Ctrl Pts',(34.6297825290984,-26.4376444612432,33.3145607080708));
#72700=CARTESIAN_POINT('Ctrl Pts',(34.4,-26.1673599741116,33.234910440458));
#72701=CARTESIAN_POINT('',(35.4377160618333,-27.0930558183544,33.0723884743082));
#72702=CARTESIAN_POINT('Origin',(33.1,-17.5710580837557,33.7339653438087));
#72703=CARTESIAN_POINT('',(33.3226453080309,-19.1751255543105,37.7041716521717));
#72704=CARTESIAN_POINT('',(33.0964948753266,-17.5458051084359,33.6714620365851));
#72705=CARTESIAN_POINT('',(34.4,-19.9986373454573,37.2739118462884));
#72706=CARTESIAN_POINT('Origin',(26.8550245390365,0.,0.));
#72707=CARTESIAN_POINT('',(34.8617922858584,-20.5053537361819,37.5246765162999));
#72708=CARTESIAN_POINT('Ctrl Pts',(34.8617922858584,-20.5053537361819,37.5246765162999));
#72709=CARTESIAN_POINT('Ctrl Pts',(34.6297825291036,-20.2509844800875,37.3992864560079));
#72710=CARTESIAN_POINT('Ctrl Pts',(34.4,-19.9986373454573,37.2739118462884));
#72711=CARTESIAN_POINT('',(35.4377160618333,-20.9384914330515,37.274604350416));
#72712=CARTESIAN_POINT('Origin',(33.1,-11.4462726220787,36.2726528263519));
#72713=CARTESIAN_POINT('',(33.3226453080309,-12.3365516130268,40.4610861730024));
#72714=CARTESIAN_POINT('',(33.0964948753266,-11.4322568815947,36.2067139516643));
#72715=CARTESIAN_POINT('',(34.4,-13.22226624086,40.1803643021789));
#72716=CARTESIAN_POINT('Origin',(26.8550245390365,0.,0.));
#72717=CARTESIAN_POINT('',(34.8617922858584,-13.6777396430533,40.515309671231));
#72718=CARTESIAN_POINT('Ctrl Pts',(34.8617922858584,-13.6777396430533,40.515309671231));
#72719=CARTESIAN_POINT('Ctrl Pts',(34.6297825290975,-13.4490085829847,40.3476538099251));
#72720=CARTESIAN_POINT('Ctrl Pts',(34.4,-13.22226624086,40.1803643021789));
#72721=CARTESIAN_POINT('',(35.4377160618333,-14.1477215809433,40.3442502351963));
#72722=CARTESIAN_POINT('Origin',(33.1,-4.97369795887321,37.7092141076143));
#72723=CARTESIAN_POINT('',(33.3226453080309,-5.12313779357752,41.9886110647639));
#72724=CARTESIAN_POINT('',(33.0964948753266,-4.97134531440728,37.6418431848034));
#72725=CARTESIAN_POINT('',(34.4,-6.04414326732376,41.8659567209931));
#72726=CARTESIAN_POINT('Origin',(26.8550245390365,0.,0.));
#72727=CARTESIAN_POINT('',(34.8617922858584,-6.4345343521407,42.2749056435377));
#72728=CARTESIAN_POINT('Ctrl Pts',(34.8617922858584,-6.4345343521407,42.2749056435377));
#72729=CARTESIAN_POINT('Ctrl Pts',(34.629782529103,-6.23839136562604,42.0700781197339));
#72730=CARTESIAN_POINT('Ctrl Pts',(34.4,-6.04414326732376,41.8659567209931));
#72731=CARTESIAN_POINT('',(35.4377160618333,-6.9270803676906,42.1880564917558));
#72732=CARTESIAN_POINT('Origin',(33.1,1.65,38.));
#72733=CARTESIAN_POINT('',(33.3226453080309,2.24593997529677,42.240333256585));
#72734=CARTESIAN_POINT('',(33.0964948753266,1.64061806453627,37.933244060464));
#72735=CARTESIAN_POINT('',(34.4,1.31762794090604,42.2794732300362));
#72736=CARTESIAN_POINT('Origin',(26.8550245390365,0.,0.));
#72737=CARTESIAN_POINT('',(34.8617922858584,1.00418100903021,42.75));
#72738=CARTESIAN_POINT('Ctrl Pts',(34.8617922858584,1.00418100903021,42.75));
#72739=CARTESIAN_POINT('Ctrl Pts',(34.629782529099,1.16177621660694,42.5142243943532));
#72740=CARTESIAN_POINT('Ctrl Pts',(34.4,1.31762794090604,42.2794732300361));
#72741=CARTESIAN_POINT('',(35.4377160618333,0.504036677262548,42.75));
#72742=CARTESIAN_POINT('Origin',(33.1,8.2235635438135,37.1361751213135));
#72743=CARTESIAN_POINT('',(33.3226453080309,9.54677599452214,41.2086042970448));
#72744=CARTESIAN_POINT('',(33.0964948753266,8.20273209378168,37.0720625104951));
#72745=CARTESIAN_POINT('',(34.4,8.63936369090333,41.4083493394303));
#72746=CARTESIAN_POINT('Origin',(26.8550245390365,0.,0.));
#72747=CARTESIAN_POINT('',(34.8617922858584,8.41238483838185,41.9261572390061));
#72748=CARTESIAN_POINT('Ctrl Pts',(34.8617922858584,8.41238483838185,41.9261572390061));
#72749=CARTESIAN_POINT('Ctrl Pts',(34.6297825291019,8.52664381638067,41.6665974739925));
#72750=CARTESIAN_POINT('Ctrl Pts',(34.4,8.63936369090333,41.4083493394303));
#72751=CARTESIAN_POINT('',(35.4377160618333,7.91983882283194,42.013006390788));
#72752=CARTESIAN_POINT('Origin',(33.1,14.5472582706722,35.1439863533772));
#72753=CARTESIAN_POINT('',(33.3226453080309,16.5575380560557,38.9247727484987));
#72754=CARTESIAN_POINT('',(33.0964948753266,14.5156102591403,35.0844651005135));
#72755=CARTESIAN_POINT('',(34.4,15.6985967468815,39.2790537077817));
#72756=CARTESIAN_POINT('Origin',(26.8550245390365,0.,0.));
#72757=CARTESIAN_POINT('',(34.8617922858584,15.5649826112914,39.8284094059642));
#72758=CARTESIAN_POINT('Ctrl Pts',(34.8617922858584,15.5649826112914,39.8284094059641));
#72759=CARTESIAN_POINT('Ctrl Pts',(34.6297825291034,15.6324336584852,39.5529520736989));
#72760=CARTESIAN_POINT('Ctrl Pts',(34.4,15.6985967468815,39.2790537077817));
#72761=CARTESIAN_POINT('',(35.4377160618333,15.0950006734014,39.9994688419988));
#72762=CARTESIAN_POINT('Origin',(33.1,20.4289419162443,32.0839653438087));
#72763=CARTESIAN_POINT('',(33.3226453080309,23.0652077022745,35.4582316768749));
#72764=CARTESIAN_POINT('',(33.0964948753266,20.3874389520281,32.0308439720488));
#72765=CARTESIAN_POINT('',(34.4,22.2808358845789,35.9562839053824));
#72766=CARTESIAN_POINT('Origin',(26.8550245390365,0.,0.));
#72767=CARTESIAN_POINT('',(34.8617922858584,22.2446462638181,36.5204955072696));
#72768=CARTESIAN_POINT('Ctrl Pts',(34.8617922858584,22.2446462638181,36.5204955072696));
#72769=CARTESIAN_POINT('Ctrl Pts',(34.6297825291015,22.2632399142706,36.2375102394016));
#72770=CARTESIAN_POINT('Ctrl Pts',(34.4,22.2808358845789,35.9562839053824));
#72771=CARTESIAN_POINT('',(35.4377160618333,21.8115085669485,36.7705676731535));
#72772=CARTESIAN_POINT('Origin',(33.1,25.6899024992348,28.0490892825384));
#72773=CARTESIAN_POINT('',(33.3226453080309,28.872052684018,30.9143101784803));
#72774=CARTESIAN_POINT('',(33.0964948753266,25.6398056289004,28.0039818578826));
#72775=CARTESIAN_POINT('',(34.4,28.1860830985703,31.5410006112756));
#72776=CARTESIAN_POINT('Origin',(26.8550245390365,0.,0.));
#72777=CARTESIAN_POINT('',(34.8617922858584,28.2484175959528,32.1029248328492));
#72778=CARTESIAN_POINT('Ctrl Pts',(34.8617922858584,28.2484175959528,32.1029248328492));
#72779=CARTESIAN_POINT('Ctrl Pts',(34.6297825291063,28.217588891004,31.821009993553));
#72780=CARTESIAN_POINT('Ctrl Pts',(34.4,28.1860830985703,31.5410006112756));
#72781=CARTESIAN_POINT('',(35.4377160618333,27.8652848098447,32.4244114123644));
#72782=CARTESIAN_POINT('Origin',(33.1,30.170288394504,23.1619558369422));
#72783=CARTESIAN_POINT('',(33.3226453080309,33.8016349549212,25.4310730087083));
#72784=CARTESIAN_POINT('',(33.0964948753266,30.1131197861062,23.1262329256631));
#72785=CARTESIAN_POINT('',(34.4,33.234910440458,26.1673599741116));
#72786=CARTESIAN_POINT('Origin',(26.8550245390365,0.,0.));
#72787=CARTESIAN_POINT('',(34.8617922858584,33.3938750538235,26.7099230322464));
#72788=CARTESIAN_POINT('Ctrl Pts',(34.8617922858584,33.3938750538235,26.7099230322464));
#72789=CARTESIAN_POINT('Ctrl Pts',(34.6297825291001,33.3145607080714,26.4376444612452));
#72790=CARTESIAN_POINT('Ctrl Pts',(34.4,33.234910440458,26.1673599741116));
#72791=CARTESIAN_POINT('',(35.4377160618333,33.0723884743082,27.0930558183544));
#72792=CARTESIAN_POINT('Origin',(33.1,33.7339653438087,17.5710580837557));
#72793=CARTESIAN_POINT('',(33.3226453080309,37.7041716521717,19.1751255543105));
#72794=CARTESIAN_POINT('',(33.0964948753266,33.6714620365851,17.5458051084359));
#72795=CARTESIAN_POINT('',(34.4,37.2739118462884,19.9986373454573));
#72796=CARTESIAN_POINT('Origin',(26.8550245390365,0.,0.));
#72797=CARTESIAN_POINT('',(34.8617922858584,37.5246765162999,20.5053537361819));
#72798=CARTESIAN_POINT('Ctrl Pts',(34.8617922858584,37.5246765162999,20.5053537361819));
#72799=CARTESIAN_POINT('Ctrl Pts',(34.6297825291027,37.3992864560074,20.2509844800865));
#72800=CARTESIAN_POINT('Ctrl Pts',(34.4,37.2739118462884,19.9986373454573));
#72801=CARTESIAN_POINT('',(35.4377160618333,37.274604350416,20.9384914330515));
#72802=CARTESIAN_POINT('Origin',(33.1,36.2726528263519,11.4462726220787));
#72803=CARTESIAN_POINT('',(33.3226453080309,40.4610861730024,12.3365516130268));
#72804=CARTESIAN_POINT('',(33.0964948753266,36.2067139516643,11.4322568815947));
#72805=CARTESIAN_POINT('',(34.4,40.1803643021789,13.22226624086));
#72806=CARTESIAN_POINT('Origin',(26.8550245390365,0.,0.));
#72807=CARTESIAN_POINT('',(34.8617922858584,40.515309671231,13.6777396430533));
#72808=CARTESIAN_POINT('Ctrl Pts',(34.8617922858584,40.515309671231,13.6777396430533));
#72809=CARTESIAN_POINT('Ctrl Pts',(34.6297825290994,40.3476538099265,13.4490085829866));
#72810=CARTESIAN_POINT('Ctrl Pts',(34.4,40.1803643021789,13.22226624086));
#72811=CARTESIAN_POINT('',(35.4377160618333,40.3442502351963,14.1477215809433));
#72812=CARTESIAN_POINT('Origin',(33.1,37.7092141076143,4.97369795887321));
#72813=CARTESIAN_POINT('',(33.3226453080309,41.9886110647639,5.12313779357752));
#72814=CARTESIAN_POINT('',(33.0964948753266,37.6418431848034,4.97134531440728));
#72815=CARTESIAN_POINT('',(34.4,41.8659567209931,6.04414326732376));
#72816=CARTESIAN_POINT('Origin',(26.8550245390365,0.,0.));
#72817=CARTESIAN_POINT('',(34.8617922858584,42.2749056435377,6.4345343521407));
#72818=CARTESIAN_POINT('Ctrl Pts',(34.8617922858584,42.2749056435377,6.4345343521407));
#72819=CARTESIAN_POINT('Ctrl Pts',(34.629782529104,42.0700781197348,6.23839136562689));
#72820=CARTESIAN_POINT('Ctrl Pts',(34.4,41.8659567209931,6.04414326732376));
#72821=CARTESIAN_POINT('',(35.4377160618333,42.1880564917558,6.9270803676906));
#72822=CARTESIAN_POINT('Origin',(17.5,42.75,0.));
#72823=CARTESIAN_POINT('',(34.8617922858584,42.75,-1.00418100903021));
#72824=CARTESIAN_POINT('',(35.4377160618333,42.75,-0.504036677262545));
#72825=CARTESIAN_POINT('Ctrl Pts',(34.8617922858584,42.75,1.00418100903022));
#72826=CARTESIAN_POINT('Ctrl Pts',(34.8382109660634,42.75,1.80411241501588E-15));
#72827=CARTESIAN_POINT('Ctrl Pts',(34.8617922858584,42.75,-1.00418100903021));
#72828=CARTESIAN_POINT('Origin',(0.,37.,0.));
#72829=CARTESIAN_POINT('',(0.,42.75,0.884158520433536));
#72830=CARTESIAN_POINT('',(0.,37.6651655808655,-0.062325622023615));
#72831=CARTESIAN_POINT('',(0.,42.75,0.));
#72832=CARTESIAN_POINT('Origin',(0.,37.,0.));
#72833=CARTESIAN_POINT('',(0.,41.9469989254299,8.29418576107602));
#72834=CARTESIAN_POINT('',(0.,36.2945488399958,6.17584017667492));
#72835=CARTESIAN_POINT('',(0.,42.6583746990022,4.25977326949884));
#72836=CARTESIAN_POINT('Origin',(0.,37.,0.));
#72837=CARTESIAN_POINT('',(0.,39.8694595147163,15.4521983644287));
#72838=CARTESIAN_POINT('',(0.,33.4731411603662,11.6778166023976));
#72839=CARTESIAN_POINT('',(0.,42.335948439747,8.67557573757185));
#72840=CARTESIAN_POINT('Origin',(0.,37.,0.));
#72841=CARTESIAN_POINT('',(0.,36.580506751568,22.1407037396679));
#72842=CARTESIAN_POINT('',(0.,29.5122178964835,16.0943600450819));
#72843=CARTESIAN_POINT('',(0.,41.6475860117848,13.3642650149939));
#72844=CARTESIAN_POINT('Origin',(0.,37.,0.));
#72845=CARTESIAN_POINT('',(0.,32.1800738014028,28.156475035514));
#72846=CARTESIAN_POINT('',(0.,24.8063469907288,19.1973293864723));
#72847=CARTESIAN_POINT('',(0.,40.3921542999172,18.3696985987366));
#72848=CARTESIAN_POINT('Origin',(0.,37.,0.));
#72849=CARTESIAN_POINT('',(0.,26.8018655926851,33.3167260852698));
#72850=CARTESIAN_POINT('',(0.,19.7883255734973,20.897949308743));
#72851=CARTESIAN_POINT('',(0.,38.3354159575187,23.6389282279734));
#72852=CARTESIAN_POINT('Origin',(0.,37.,0.));
#72853=CARTESIAN_POINT('',(0.,20.6092962603321,37.4646652720015));
#72854=CARTESIAN_POINT('',(0.,14.8810740823533,21.2488434819817));
#72855=CARTESIAN_POINT('',(0.,35.25,29.0118510267787));
#72856=CARTESIAN_POINT('Origin',(0.,37.,0.));
#72857=CARTESIAN_POINT('',(0.,13.790523889916,40.4742595624789));
#72858=CARTESIAN_POINT('',(0.,10.4521657293574,20.4298559661641));
#72859=CARTESIAN_POINT('',(0.,30.9572722260229,34.2260741489971));
#72860=CARTESIAN_POINT('Origin',(0.,37.,0.));
#72861=CARTESIAN_POINT('',(0.,6.55273342944653,42.2540639571139));
#72862=CARTESIAN_POINT('',(0.,6.77630740640388,18.7196089291248));
#72863=CARTESIAN_POINT('',(0.,25.3656163375309,38.9368451155095));
#72864=CARTESIAN_POINT('Origin',(0.,37.,0.));
#72865=CARTESIAN_POINT('',(0.,-0.884158520433534,42.75));
#72866=CARTESIAN_POINT('',(0.,4.01009029474227,16.4564323480298));
#72867=CARTESIAN_POINT('',(0.,18.5,42.75));
#72868=CARTESIAN_POINT('Origin',(0.,37.,0.));
#72869=CARTESIAN_POINT('',(0.,-8.29418576107602,41.9469989254299));
#72870=CARTESIAN_POINT('',(0.,2.18181606689636,13.9935441805696));
#72871=CARTESIAN_POINT('',(0.,10.5186971470084,45.2642177670343));
#72872=CARTESIAN_POINT('Origin',(0.,37.,0.));
#72873=CARTESIAN_POINT('',(0.,-15.4521983644287,39.8694595147163));
#72874=CARTESIAN_POINT('',(0.,1.19736103864281,11.6540088485914));
#72875=CARTESIAN_POINT('',(0.,1.71454997167821,46.1176449281981));
#72876=CARTESIAN_POINT('Origin',(0.,37.,0.));
#72877=CARTESIAN_POINT('',(0.,-22.1407037396679,36.580506751568));
#72878=CARTESIAN_POINT('',(0.,0.861089067994371,9.69098078979665));
#72879=CARTESIAN_POINT('',(0.,-7.49999999999998,45.0333209967908));
#72880=CARTESIAN_POINT('Origin',(0.,37.,0.));
#72881=CARTESIAN_POINT('',(0.,-28.156475035514,32.1800738014028));
#72882=CARTESIAN_POINT('',(0.,0.909000315285454,8.25805229904004));
#72883=CARTESIAN_POINT('',(0.,-16.6229246706804,41.8578716586992));
#72884=CARTESIAN_POINT('Origin',(0.,37.,0.));
#72885=CARTESIAN_POINT('',(0.,-33.3167260852698,26.8018655926852));
#72886=CARTESIAN_POINT('',(0.,1.04982739730203,7.39325534798233));
#72887=CARTESIAN_POINT('',(0.,-25.1046455867554,36.5886420294625));
#72888=CARTESIAN_POINT('Origin',(0.,37.,0.));
#72889=CARTESIAN_POINT('',(0.,-37.4646652720015,20.6092962603321));
#72890=CARTESIAN_POINT('',(0.,1.00884095837589,7.01857020850226));
#72891=CARTESIAN_POINT('',(0.,-32.3975860117848,29.3857349850061));
#72892=CARTESIAN_POINT('Origin',(0.,37.,0.));
#72893=CARTESIAN_POINT('',(0.,-40.4742595624789,13.790523889916));
#72894=CARTESIAN_POINT('',(0.,0.568817492022398,6.95487569709476));
#72895=CARTESIAN_POINT('',(0.,-38.0077706374481,20.5671465167728));
#72896=CARTESIAN_POINT('Origin',(0.,37.,0.));
#72897=CARTESIAN_POINT('',(0.,-42.2540639571139,6.55273342944654));
#72898=CARTESIAN_POINT('',(0.,-0.39700986412022,6.95036949266363));
#72899=CARTESIAN_POINT('',(0.,-41.5426881835415,10.5871459210237));
#72900=CARTESIAN_POINT('Origin',(0.,37.,0.));
#72901=CARTESIAN_POINT('',(0.,-42.75,-0.884158520433531));
#72902=CARTESIAN_POINT('',(0.,-1.90419702074843,6.718823527578));
#72903=CARTESIAN_POINT('',(0.,-42.75,7.50096164477754E-15));
#72904=CARTESIAN_POINT('Origin',(0.,37.,0.));
#72905=CARTESIAN_POINT('',(0.,-41.9469989254299,-8.29418576107601));
#72906=CARTESIAN_POINT('',(0.,-3.85120042414092,5.98282072632249));
#72907=CARTESIAN_POINT('',(0.,-41.5426881835416,-10.5871459210237));
#72908=CARTESIAN_POINT('Origin',(0.,37.,0.));
#72909=CARTESIAN_POINT('',(0.,-39.8694595147163,-15.4521983644287));
#72910=CARTESIAN_POINT('',(0.,-6.02918648963184,4.51649335041757));
#72911=CARTESIAN_POINT('',(0.,-38.0077706374481,-20.5671465167728));
#72912=CARTESIAN_POINT('Origin',(0.,37.,0.));
#72913=CARTESIAN_POINT('',(0.,-36.580506751568,-22.1407037396679));
#72914=CARTESIAN_POINT('',(0.,-8.14642990287292,2.18232617468118));
#72915=CARTESIAN_POINT('',(0.,-32.3975860117848,-29.385734985006));
#72916=CARTESIAN_POINT('Origin',(0.,37.,0.));
#72917=CARTESIAN_POINT('',(0.,-32.1800738014028,-28.156475035514));
#72918=CARTESIAN_POINT('',(0.,-9.86438200079779,-1.04270499302577));
#72919=CARTESIAN_POINT('',(0.,-25.1046455867554,-36.5886420294625));
#72920=CARTESIAN_POINT('Origin',(0.,37.,0.));
#72921=CARTESIAN_POINT('',(0.,-26.8018655926852,-33.3167260852698));
#72922=CARTESIAN_POINT('',(0.,-10.8410320540273,-5.05510237718296));
#72923=CARTESIAN_POINT('',(0.,-16.6229246706805,-41.8578716586992));
#72924=CARTESIAN_POINT('Origin',(0.,37.,0.));
#72925=CARTESIAN_POINT('',(0.,-20.6092962603321,-37.4646652720015));
#72926=CARTESIAN_POINT('',(0.,-10.7762546488599,-9.62865516777302));
#72927=CARTESIAN_POINT('',(0.,-7.50000000000002,-45.0333209967908));
#72928=CARTESIAN_POINT('Origin',(0.,37.,0.));
#72929=CARTESIAN_POINT('',(0.,-13.790523889916,-40.4742595624789));
#72930=CARTESIAN_POINT('',(0.,-9.45354915528123,-14.4338924757149));
#72931=CARTESIAN_POINT('',(0.,1.71454997167818,-46.1176449281981));
#72932=CARTESIAN_POINT('Origin',(0.,37.,0.));
#72933=CARTESIAN_POINT('',(0.,-6.55273342944652,-42.2540639571139));
#72934=CARTESIAN_POINT('',(0.,-6.77296855766818,-19.07107195038));
#72935=CARTESIAN_POINT('',(0.,10.5186971470084,-45.2642177670343));
#72936=CARTESIAN_POINT('Origin',(0.,37.,0.));
#72937=CARTESIAN_POINT('',(0.,0.884158520433529,-42.75));
#72938=CARTESIAN_POINT('',(0.,-2.77105885485935,-23.1129302535842));
#72939=CARTESIAN_POINT('',(0.,18.5,-42.75));
#72940=CARTESIAN_POINT('Origin',(0.,37.,0.));
#72941=CARTESIAN_POINT('',(0.,8.294185761076,-41.9469989254299));
#72942=CARTESIAN_POINT('',(0.,2.37483551724878,-26.1522050835671));
#72943=CARTESIAN_POINT('',(0.,25.3656163375309,-38.9368451155095));
#72944=CARTESIAN_POINT('Origin',(0.,37.,0.));
#72945=CARTESIAN_POINT('',(0.,15.4521983644287,-39.8694595147163));
#72946=CARTESIAN_POINT('',(0.,8.35868429062286,-27.8483188014066));
#72947=CARTESIAN_POINT('',(0.,30.9572722260229,-34.2260741489971));
#72948=CARTESIAN_POINT('Origin',(0.,37.,0.));
#72949=CARTESIAN_POINT('',(0.,22.1407037396679,-36.580506751568));
#72950=CARTESIAN_POINT('',(0.,14.7731229383951,-27.9676670095597));
#72951=CARTESIAN_POINT('',(0.,35.25,-29.0118510267787));
#72952=CARTESIAN_POINT('Origin',(0.,37.,0.));
#72953=CARTESIAN_POINT('',(0.,28.156475035514,-32.1800738014028));
#72954=CARTESIAN_POINT('',(0.,21.1490346947835,-26.4126766924866));
#72955=CARTESIAN_POINT('',(0.,38.3354159575187,-23.6389282279734));
#72956=CARTESIAN_POINT('Origin',(0.,37.,0.));
#72957=CARTESIAN_POINT('',(0.,33.3167260852698,-26.8018655926852));
#72958=CARTESIAN_POINT('',(0.,27.002879083228,-23.2361022795424));
#72959=CARTESIAN_POINT('',(0.,40.3921542999172,-18.3696985987366));
#72960=CARTESIAN_POINT('Origin',(0.,37.,0.));
#72961=CARTESIAN_POINT('',(0.,37.4646652720015,-20.6092962603321));
#72962=CARTESIAN_POINT('',(0.,31.8863396081306,-18.638758522711));
#72963=CARTESIAN_POINT('',(0.,41.6475860117848,-13.364265014994));
#72964=CARTESIAN_POINT('Origin',(0.,37.,0.));
#72965=CARTESIAN_POINT('',(0.,40.4742595624789,-13.790523889916));
#72966=CARTESIAN_POINT('',(0.,35.4325659339014,-12.9508391875439));
#72967=CARTESIAN_POINT('',(0.,42.335948439747,-8.67557573757187));
#72968=CARTESIAN_POINT('Origin',(0.,37.,0.));
#72969=CARTESIAN_POINT('',(0.,42.2540639571139,-6.55273342944652));
#72970=CARTESIAN_POINT('',(0.,37.3936710153845,-6.59890647140843));
#72971=CARTESIAN_POINT('',(0.,42.6583746990022,-4.25977326949884));
#72972=CARTESIAN_POINT('Origin',(17.5,42.1005314412719,-7.42345959526127));
#72973=CARTESIAN_POINT('',(0.138207714141615,42.2749056435377,-6.43453435214071));
#72974=CARTESIAN_POINT('',(-0.437716061833263,42.1880564917558,-6.92708036769061));
#72975=CARTESIAN_POINT('Ctrl Pts',(0.138207714141624,41.9261572390061,-8.41238483838185));
#72976=CARTESIAN_POINT('Ctrl Pts',(0.16178903393654,42.1005314412719,-7.42345959526128));
#72977=CARTESIAN_POINT('Ctrl Pts',(0.138207714141615,42.2749056435377,-6.43453435214071));
#72978=CARTESIAN_POINT('Origin',(17.5,40.1718595385976,-14.6213611271724));
#72979=CARTESIAN_POINT('',(0.13820771414162,40.515309671231,-13.6777396430533));
#72980=CARTESIAN_POINT('',(-0.437716061833263,40.3442502351963,-14.1477215809433));
#72981=CARTESIAN_POINT('Ctrl Pts',(0.138207714141623,39.8284094059641,-15.5649826112914));
#72982=CARTESIAN_POINT('Ctrl Pts',(0.161789033936545,40.1718595385976,-14.6213611271724));
#72983=CARTESIAN_POINT('Ctrl Pts',(0.13820771414162,40.515309671231,-13.6777396430533));
#72984=CARTESIAN_POINT('Origin',(17.5,37.0225860117847,-21.375));
#72985=CARTESIAN_POINT('',(0.138207714141623,37.5246765162998,-20.505353736182));
#72986=CARTESIAN_POINT('',(-0.437716061833263,37.274604350416,-20.9384914330516));
#72987=CARTESIAN_POINT('Ctrl Pts',(0.138207714141626,36.5204955072696,-22.2446462638181));
#72988=CARTESIAN_POINT('Ctrl Pts',(0.161789033936547,37.0225860117847,-21.375));
#72989=CARTESIAN_POINT('Ctrl Pts',(0.138207714141623,37.5246765162998,-20.505353736182));
#72990=CARTESIAN_POINT('Origin',(17.5,32.7483999433363,-27.4791703140996));
#72991=CARTESIAN_POINT('',(0.138207714141626,33.3938750538235,-26.7099230322464));
#72992=CARTESIAN_POINT('',(-0.437716061833263,33.0723884743082,-27.0930558183544));
#72993=CARTESIAN_POINT('Ctrl Pts',(0.13820771414163,32.1029248328491,-28.2484175959528));
#72994=CARTESIAN_POINT('Ctrl Pts',(0.16178903393655,32.7483999433363,-27.4791703140996));
#72995=CARTESIAN_POINT('Ctrl Pts',(0.138207714141626,33.3938750538235,-26.7099230322464));
#72996=CARTESIAN_POINT('Origin',(17.5,27.4791703140995,-32.7483999433363));
#72997=CARTESIAN_POINT('',(0.138207714141627,28.2484175959528,-32.1029248328492));
#72998=CARTESIAN_POINT('',(-0.437716061833263,27.8652848098447,-32.4244114123644));
#72999=CARTESIAN_POINT('Ctrl Pts',(0.138207714141623,26.7099230322463,-33.3938750538235));
#73000=CARTESIAN_POINT('Ctrl Pts',(0.161789033936551,27.4791703140995,-32.7483999433363));
#73001=CARTESIAN_POINT('Ctrl Pts',(0.138207714141627,28.2484175959528,-32.1029248328492));
#73002=CARTESIAN_POINT('Origin',(17.5,21.375,-37.0225860117847));
#73003=CARTESIAN_POINT('',(0.138207714141627,22.2446462638181,-36.5204955072696));
#73004=CARTESIAN_POINT('',(-0.437716061833263,21.8115085669485,-36.7705676731535));
#73005=CARTESIAN_POINT('Ctrl Pts',(0.138207714141623,20.505353736182,-37.5246765162999));
#73006=CARTESIAN_POINT('Ctrl Pts',(0.16178903393655,21.375,-37.0225860117847));
#73007=CARTESIAN_POINT('Ctrl Pts',(0.138207714141627,22.2446462638181,-36.5204955072696));
#73008=CARTESIAN_POINT('Origin',(17.5,14.6213611271723,-40.1718595385976));
#73009=CARTESIAN_POINT('',(0.138207714141622,15.5649826112913,-39.8284094059642));
#73010=CARTESIAN_POINT('',(-0.437716061833263,15.0950006734014,-39.9994688419989));
#73011=CARTESIAN_POINT('Ctrl Pts',(0.138207714141626,13.6777396430533,-40.515309671231));
#73012=CARTESIAN_POINT('Ctrl Pts',(0.161789033936545,14.6213611271723,-40.1718595385976));
#73013=CARTESIAN_POINT('Ctrl Pts',(0.138207714141622,15.5649826112913,-39.8284094059642));
#73014=CARTESIAN_POINT('Origin',(17.5,7.42345959526125,-42.1005314412719));
#73015=CARTESIAN_POINT('',(0.138207714141623,8.41238483838183,-41.9261572390061));
#73016=CARTESIAN_POINT('',(-0.437716061833263,7.91983882283192,-42.013006390788));
#73017=CARTESIAN_POINT('Ctrl Pts',(0.138207714141623,6.43453435214068,-42.2749056435377));
#73018=CARTESIAN_POINT('Ctrl Pts',(0.161789033936546,7.42345959526126,-42.1005314412719));
#73019=CARTESIAN_POINT('Ctrl Pts',(0.138207714141623,8.41238483838183,-41.9261572390061));
#73020=CARTESIAN_POINT('Origin',(17.5,-7.8530475995324E-15,-42.75));
#73021=CARTESIAN_POINT('',(0.138207714141622,1.0041810090302,-42.75));
#73022=CARTESIAN_POINT('',(-0.437716061833263,0.504036677262537,-42.75));
#73023=CARTESIAN_POINT('Ctrl Pts',(0.138207714141621,-1.00418100903022,
-42.75));
#73024=CARTESIAN_POINT('Ctrl Pts',(0.161789033936545,-7.49400541621981E-15,
-42.75));
#73025=CARTESIAN_POINT('Ctrl Pts',(0.138207714141622,1.0041810090302,-42.75));
#73026=CARTESIAN_POINT('Origin',(17.5,-7.42345959526127,-42.1005314412719));
#73027=CARTESIAN_POINT('',(0.138207714141622,-6.4345343521407,-42.2749056435377));
#73028=CARTESIAN_POINT('',(-0.437716061833263,-6.9270803676906,-42.1880564917558));
#73029=CARTESIAN_POINT('Ctrl Pts',(0.138207714141623,-8.41238483838184,
-41.9261572390061));
#73030=CARTESIAN_POINT('Ctrl Pts',(0.161789033936548,-7.42345959526127,
-42.1005314412719));
#73031=CARTESIAN_POINT('Ctrl Pts',(0.138207714141622,-6.4345343521407,-42.2749056435377));
#73032=CARTESIAN_POINT('Origin',(17.5,-14.6213611271724,-40.1718595385976));
#73033=CARTESIAN_POINT('',(0.138207714141628,-13.6777396430533,-40.515309671231));
#73034=CARTESIAN_POINT('',(-0.437716061833263,-14.1477215809433,-40.3442502351963));
#73035=CARTESIAN_POINT('Ctrl Pts',(0.138207714141625,-15.5649826112914,
-39.8284094059641));
#73036=CARTESIAN_POINT('Ctrl Pts',(0.161789033936553,-14.6213611271724,
-40.1718595385976));
#73037=CARTESIAN_POINT('Ctrl Pts',(0.138207714141628,-13.6777396430533,
-40.515309671231));
#73038=CARTESIAN_POINT('Origin',(17.5,-21.375,-37.0225860117847));
#73039=CARTESIAN_POINT('',(0.138207714141623,-20.505353736182,-37.5246765162998));
#73040=CARTESIAN_POINT('',(-0.437716061833263,-20.9384914330516,-37.274604350416));
#73041=CARTESIAN_POINT('Ctrl Pts',(0.138207714141625,-22.2446462638181,
-36.5204955072696));
#73042=CARTESIAN_POINT('Ctrl Pts',(0.161789033936547,-21.375,-37.0225860117847));
#73043=CARTESIAN_POINT('Ctrl Pts',(0.138207714141623,-20.505353736182,-37.5246765162998));
#73044=CARTESIAN_POINT('Origin',(17.5,-27.4791703140996,-32.7483999433363));
#73045=CARTESIAN_POINT('',(0.138207714141625,-26.7099230322463,-33.3938750538235));
#73046=CARTESIAN_POINT('',(-0.437716061833263,-27.0930558183544,-33.0723884743082));
#73047=CARTESIAN_POINT('Ctrl Pts',(0.138207714141625,-28.2484175959528,
-32.1029248328492));
#73048=CARTESIAN_POINT('Ctrl Pts',(0.161789033936547,-27.4791703140996,
-32.7483999433363));
#73049=CARTESIAN_POINT('Ctrl Pts',(0.138207714141625,-26.7099230322464,
-33.3938750538235));
#73050=CARTESIAN_POINT('Origin',(17.5,-32.7483999433363,-27.4791703140996));
#73051=CARTESIAN_POINT('',(0.138207714141624,-32.1029248328492,-28.2484175959528));
#73052=CARTESIAN_POINT('',(-0.437716061833263,-32.4244114123644,-27.8652848098447));
#73053=CARTESIAN_POINT('Ctrl Pts',(0.138207714141623,-33.3938750538235,
-26.7099230322464));
#73054=CARTESIAN_POINT('Ctrl Pts',(0.161789033936548,-32.7483999433363,
-27.4791703140996));
#73055=CARTESIAN_POINT('Ctrl Pts',(0.138207714141624,-32.1029248328492,
-28.2484175959527));
#73056=CARTESIAN_POINT('Origin',(17.5,-37.0225860117848,-21.375));
#73057=CARTESIAN_POINT('',(0.138207714141622,-36.5204955072697,-22.244646263818));
#73058=CARTESIAN_POINT('',(-0.437716061833263,-36.7705676731535,-21.8115085669484));
#73059=CARTESIAN_POINT('Ctrl Pts',(0.138207714141633,-37.5246765162999,
-20.5053537361819));
#73060=CARTESIAN_POINT('Ctrl Pts',(0.161789033936547,-37.0225860117848,
-21.375));
#73061=CARTESIAN_POINT('Ctrl Pts',(0.138207714141622,-36.5204955072697,
-22.244646263818));
#73062=CARTESIAN_POINT('Origin',(17.5,-40.1718595385976,-14.6213611271723));
#73063=CARTESIAN_POINT('',(0.138207714141633,-39.8284094059642,-15.5649826112914));
#73064=CARTESIAN_POINT('',(-0.437716061833263,-39.9994688419988,-15.0950006734014));
#73065=CARTESIAN_POINT('Ctrl Pts',(0.138207714141626,-40.515309671231,-13.6777396430533));
#73066=CARTESIAN_POINT('Ctrl Pts',(0.161789033936555,-40.1718595385976,
-14.6213611271723));
#73067=CARTESIAN_POINT('Ctrl Pts',(0.138207714141633,-39.8284094059642,
-15.5649826112914));
#73068=CARTESIAN_POINT('Origin',(17.5,-42.1005314412719,-7.42345959526126));
#73069=CARTESIAN_POINT('',(0.138207714141624,-41.9261572390061,-8.41238483838183));
#73070=CARTESIAN_POINT('',(-0.437716061833263,-42.013006390788,-7.91983882283192));
#73071=CARTESIAN_POINT('Ctrl Pts',(0.138207714141624,-42.2749056435377,
-6.43453435214068));
#73072=CARTESIAN_POINT('Ctrl Pts',(0.161789033936547,-42.1005314412719,
-7.42345959526126));
#73073=CARTESIAN_POINT('Ctrl Pts',(0.138207714141624,-41.9261572390061,
-8.41238483838183));
#73074=CARTESIAN_POINT('Origin',(17.5,-42.75,5.23536506635493E-15));
#73075=CARTESIAN_POINT('',(0.138207714141623,-42.75,-1.00418100903021));
#73076=CARTESIAN_POINT('',(-0.437716061833263,-42.75,-0.50403667726254));
#73077=CARTESIAN_POINT('',(0.149999999999998,-42.75,-5.05935899139558E-15));
#73078=CARTESIAN_POINT('Ctrl Pts',(0.149999999999998,-42.75,-4.88335291643624E-15));
#73079=CARTESIAN_POINT('Ctrl Pts',(0.149999999999999,-42.75,-0.502021265003248));
#73080=CARTESIAN_POINT('Ctrl Pts',(0.138207714141623,-42.75,-1.00418100903021));
#73081=CARTESIAN_POINT('Ctrl Pts',(0.13820771414162,-42.75,1.00418100903021));
#73082=CARTESIAN_POINT('Ctrl Pts',(0.149999999999998,-42.75,0.502021265003246));
#73083=CARTESIAN_POINT('Ctrl Pts',(0.149999999999998,-42.75,-4.88335291643624E-15));
#73084=CARTESIAN_POINT('Origin',(17.5,-42.1005314412719,7.42345959526129));
#73085=CARTESIAN_POINT('',(0.138207714141624,-42.2749056435377,6.43453435214071));
#73086=CARTESIAN_POINT('',(-0.437716061833263,-42.1880564917558,6.92708036769062));
#73087=CARTESIAN_POINT('Ctrl Pts',(0.138207714141622,-41.926157239006,8.41238483838185));
#73088=CARTESIAN_POINT('Ctrl Pts',(0.161789033936547,-42.1005314412719,
7.42345959526129));
#73089=CARTESIAN_POINT('Ctrl Pts',(0.138207714141624,-42.2749056435377,
6.43453435214071));
#73090=CARTESIAN_POINT('Origin',(17.5,-40.1718595385976,14.6213611271723));
#73091=CARTESIAN_POINT('',(0.138207714141621,-40.515309671231,13.6777396430533));
#73092=CARTESIAN_POINT('',(-0.437716061833263,-40.3442502351963,14.1477215809433));
#73093=CARTESIAN_POINT('Ctrl Pts',(0.138207714141621,-39.8284094059642,
15.5649826112914));
#73094=CARTESIAN_POINT('Ctrl Pts',(0.161789033936546,-40.1718595385976,
14.6213611271723));
#73095=CARTESIAN_POINT('Ctrl Pts',(0.138207714141621,-40.515309671231,13.6777396430533));
#73096=CARTESIAN_POINT('Origin',(17.5,-37.0225860117848,21.375));
#73097=CARTESIAN_POINT('',(0.138207714141623,-37.5246765162999,20.5053537361819));
#73098=CARTESIAN_POINT('',(-0.437716061833263,-37.274604350416,20.9384914330515));
#73099=CARTESIAN_POINT('Ctrl Pts',(0.138207714141621,-36.5204955072697,
22.244646263818));
#73100=CARTESIAN_POINT('Ctrl Pts',(0.161789033936545,-37.0225860117848,
21.375));
#73101=CARTESIAN_POINT('Ctrl Pts',(0.138207714141623,-37.5246765162999,
20.5053537361819));
#73102=CARTESIAN_POINT('Origin',(17.5,-32.7483999433363,27.4791703140996));
#73103=CARTESIAN_POINT('',(0.138207714141626,-33.3938750538235,26.7099230322464));
#73104=CARTESIAN_POINT('',(-0.437716061833263,-33.0723884743082,27.0930558183544));
#73105=CARTESIAN_POINT('Ctrl Pts',(0.138207714141625,-32.1029248328492,
28.2484175959528));
#73106=CARTESIAN_POINT('Ctrl Pts',(0.161789033936548,-32.7483999433363,
27.4791703140996));
#73107=CARTESIAN_POINT('Ctrl Pts',(0.138207714141626,-33.3938750538235,
26.7099230322464));
#73108=CARTESIAN_POINT('Origin',(17.5,-27.4791703140996,32.7483999433363));
#73109=CARTESIAN_POINT('',(0.13820771414163,-28.2484175959528,32.1029248328492));
#73110=CARTESIAN_POINT('',(-0.437716061833263,-27.8652848098447,32.4244114123644));
#73111=CARTESIAN_POINT('Ctrl Pts',(0.138207714141626,-26.7099230322463,
33.3938750538235));
#73112=CARTESIAN_POINT('Ctrl Pts',(0.161789033936555,-27.4791703140996,
32.7483999433363));
#73113=CARTESIAN_POINT('Ctrl Pts',(0.13820771414163,-28.2484175959528,32.1029248328492));
#73114=CARTESIAN_POINT('Origin',(17.5,-21.375,37.0225860117848));
#73115=CARTESIAN_POINT('',(0.138207714141625,-22.244646263818,36.5204955072697));
#73116=CARTESIAN_POINT('',(-0.437716061833263,-21.8115085669485,36.7705676731535));
#73117=CARTESIAN_POINT('Ctrl Pts',(0.138207714141623,-20.5053537361819,
37.5246765162999));
#73118=CARTESIAN_POINT('Ctrl Pts',(0.161789033936548,-21.375,37.0225860117848));
#73119=CARTESIAN_POINT('Ctrl Pts',(0.138207714141625,-22.244646263818,36.5204955072697));
#73120=CARTESIAN_POINT('Origin',(17.5,-14.6213611271723,40.1718595385976));
#73121=CARTESIAN_POINT('',(0.138207714141622,-15.5649826112914,39.8284094059642));
#73122=CARTESIAN_POINT('',(-0.437716061833263,-15.0950006734014,39.9994688419988));
#73123=CARTESIAN_POINT('Ctrl Pts',(0.138207714141626,-13.6777396430533,
40.515309671231));
#73124=CARTESIAN_POINT('Ctrl Pts',(0.161789033936544,-14.6213611271723,
40.1718595385976));
#73125=CARTESIAN_POINT('Ctrl Pts',(0.138207714141622,-15.5649826112914,
39.8284094059642));
#73126=CARTESIAN_POINT('Origin',(17.5,-7.42345959526127,42.1005314412719));
#73127=CARTESIAN_POINT('',(0.138207714141624,-8.41238483838185,41.9261572390061));
#73128=CARTESIAN_POINT('',(-0.437716061833263,-7.91983882283194,42.013006390788));
#73129=CARTESIAN_POINT('Ctrl Pts',(0.138207714141616,-6.4345343521407,42.2749056435377));
#73130=CARTESIAN_POINT('Ctrl Pts',(0.161789033936548,-7.42345959526127,
42.1005314412719));
#73131=CARTESIAN_POINT('Ctrl Pts',(0.138207714141624,-8.41238483838185,
41.9261572390061));
#73132=CARTESIAN_POINT('Origin',(17.5,2.61768253317747E-15,42.75));
#73133=CARTESIAN_POINT('',(0.13820771414162,-1.0041810090302,42.75));
#73134=CARTESIAN_POINT('',(-0.437716061833263,-0.504036677262543,42.75));
#73135=CARTESIAN_POINT('Ctrl Pts',(0.138207714141629,1.00418100903022,42.75));
#73136=CARTESIAN_POINT('Ctrl Pts',(0.161789033936545,7.49400541621981E-15,
42.75));
#73137=CARTESIAN_POINT('Ctrl Pts',(0.13820771414162,-1.0041810090302,42.75));
#73138=CARTESIAN_POINT('Origin',(17.5,7.42345959526128,42.1005314412719));
#73139=CARTESIAN_POINT('',(0.138207714141615,6.43453435214071,42.2749056435377));
#73140=CARTESIAN_POINT('',(-0.437716061833263,6.92708036769061,42.1880564917558));
#73141=CARTESIAN_POINT('Ctrl Pts',(0.138207714141621,8.41238483838185,41.9261572390061));
#73142=CARTESIAN_POINT('Ctrl Pts',(0.161789033936541,7.42345959526128,42.1005314412719));
#73143=CARTESIAN_POINT('Ctrl Pts',(0.138207714141615,6.43453435214071,42.2749056435377));
#73144=CARTESIAN_POINT('Origin',(17.5,14.6213611271723,40.1718595385976));
#73145=CARTESIAN_POINT('',(0.138207714141621,13.6777396430533,40.515309671231));
#73146=CARTESIAN_POINT('',(-0.437716061833263,14.1477215809433,40.3442502351963));
#73147=CARTESIAN_POINT('Ctrl Pts',(0.138207714141624,15.5649826112914,39.8284094059642));
#73148=CARTESIAN_POINT('Ctrl Pts',(0.161789033936547,14.6213611271723,40.1718595385976));
#73149=CARTESIAN_POINT('Ctrl Pts',(0.138207714141621,13.6777396430533,40.515309671231));
#73150=CARTESIAN_POINT('Origin',(17.5,21.375,37.0225860117847));
#73151=CARTESIAN_POINT('',(0.138207714141623,20.505353736182,37.5246765162999));
#73152=CARTESIAN_POINT('',(-0.437716061833263,20.9384914330515,37.274604350416));
#73153=CARTESIAN_POINT('Ctrl Pts',(0.138207714141622,22.2446462638181,36.5204955072696));
#73154=CARTESIAN_POINT('Ctrl Pts',(0.161789033936545,21.375,37.0225860117847));
#73155=CARTESIAN_POINT('Ctrl Pts',(0.138207714141623,20.505353736182,37.5246765162999));
#73156=CARTESIAN_POINT('Origin',(17.5,27.4791703140996,32.7483999433363));
#73157=CARTESIAN_POINT('',(0.138207714141625,26.7099230322463,33.3938750538235));
#73158=CARTESIAN_POINT('',(-0.437716061833263,27.0930558183544,33.0723884743082));
#73159=CARTESIAN_POINT('Ctrl Pts',(0.138207714141625,28.2484175959528,32.1029248328492));
#73160=CARTESIAN_POINT('Ctrl Pts',(0.16178903393655,27.4791703140995,32.7483999433363));
#73161=CARTESIAN_POINT('Ctrl Pts',(0.138207714141625,26.7099230322463,33.3938750538235));
#73162=CARTESIAN_POINT('Origin',(17.5,32.7483999433363,27.4791703140996));
#73163=CARTESIAN_POINT('',(0.138207714141624,32.1029248328492,28.2484175959528));
#73164=CARTESIAN_POINT('',(-0.437716061833263,32.4244114123644,27.8652848098447));
#73165=CARTESIAN_POINT('Ctrl Pts',(0.138207714141623,33.3938750538235,26.7099230322464));
#73166=CARTESIAN_POINT('Ctrl Pts',(0.161789033936548,32.7483999433363,27.4791703140996));
#73167=CARTESIAN_POINT('Ctrl Pts',(0.138207714141624,32.1029248328492,28.2484175959527));
#73168=CARTESIAN_POINT('Origin',(17.5,37.0225860117848,21.375));
#73169=CARTESIAN_POINT('',(0.138207714141628,36.5204955072696,22.244646263818));
#73170=CARTESIAN_POINT('',(-0.437716061833263,36.7705676731535,21.8115085669485));
#73171=CARTESIAN_POINT('Ctrl Pts',(0.138207714141626,37.5246765162999,20.5053537361819));
#73172=CARTESIAN_POINT('Ctrl Pts',(0.161789033936552,37.0225860117848,21.375));
#73173=CARTESIAN_POINT('Ctrl Pts',(0.138207714141628,36.5204955072696,22.2446462638181));
#73174=CARTESIAN_POINT('Origin',(17.5,40.1718595385976,14.6213611271723));
#73175=CARTESIAN_POINT('',(0.138207714141622,39.8284094059642,15.5649826112914));
#73176=CARTESIAN_POINT('',(-0.437716061833263,39.9994688419988,15.0950006734014));
#73177=CARTESIAN_POINT('Ctrl Pts',(0.138207714141626,40.515309671231,13.6777396430533));
#73178=CARTESIAN_POINT('Ctrl Pts',(0.161789033936544,40.1718595385976,14.6213611271723));
#73179=CARTESIAN_POINT('Ctrl Pts',(0.138207714141622,39.8284094059642,15.5649826112914));
#73180=CARTESIAN_POINT('Origin',(17.5,42.1005314412719,7.42345959526127));
#73181=CARTESIAN_POINT('',(0.138207714141622,41.9261572390061,8.41238483838184));
#73182=CARTESIAN_POINT('',(-0.437716061833263,42.013006390788,7.91983882283194));
#73183=CARTESIAN_POINT('Ctrl Pts',(0.138207714141617,42.2749056435377,6.4345343521407));
#73184=CARTESIAN_POINT('Ctrl Pts',(0.161789033936546,42.1005314412719,7.42345959526127));
#73185=CARTESIAN_POINT('Ctrl Pts',(0.138207714141622,41.9261572390061,8.41238483838184));
#73186=CARTESIAN_POINT('Origin',(17.5,42.75,0.));
#73187=CARTESIAN_POINT('',(0.138207714141622,42.75,1.00418100903021));
#73188=CARTESIAN_POINT('',(-0.437716061833263,42.75,0.504036677262545));
#73189=CARTESIAN_POINT('Ctrl Pts',(0.13820771414163,42.75,-1.00418100903022));
#73190=CARTESIAN_POINT('Ctrl Pts',(0.161789033936547,42.75,-1.80411241501588E-15));
#73191=CARTESIAN_POINT('Ctrl Pts',(0.138207714141622,42.75,1.00418100903021));
#73192=CARTESIAN_POINT('Origin',(33.1,37.7092141076143,-4.97369795887321));
#73193=CARTESIAN_POINT('',(29.9040600247032,41.9886110647639,-5.12313779357752));
#73194=CARTESIAN_POINT('',(17.5,41.9886110647639,-5.12313779357752));
#73195=CARTESIAN_POINT('',(30.5247014514712,37.5318349744051,-4.96750374304977));
#73196=CARTESIAN_POINT('Origin',(30.5,37.7092141076143,-4.97369795887321));
#73197=CARTESIAN_POINT('',(29.9005519666592,41.9206753505941,-5.65216579287046));
#73198=CARTESIAN_POINT('Origin',(35.8405517186909,0.,0.));
#73199=CARTESIAN_POINT('',(30.4955273645547,37.6544606275072,-5.46749010626366));
#73200=CARTESIAN_POINT('Origin',(30.5,37.6223900187809,-5.46610183537932));
#73201=CARTESIAN_POINT('',(24.1697957402248,41.8715390397407,-6.00534915250319));
#73202=CARTESIAN_POINT('Origin',(97.7155570771054,0.,0.));
#73203=CARTESIAN_POINT('',(24.1012882089558,37.6326386190063,-5.86270716268919));
#73204=CARTESIAN_POINT('Origin',(24.1,37.5529307477141,-5.8600249365842));
#73205=CARTESIAN_POINT('',(23.3381365738089,41.9060788618227,-5.75938837262207));
#73206=CARTESIAN_POINT('Origin',(8.01433437672608,0.,0.));
#73207=CARTESIAN_POINT('',(23.1004586919557,37.6133097693334,-5.56495784004782));
#73208=CARTESIAN_POINT('Origin',(23.1,37.6050252010142,-5.56458261068054));
#73209=CARTESIAN_POINT('',(22.6451513366954,41.9578594516632,-5.3691740737731));
#73210=CARTESIAN_POINT('Origin',(14.1732738814488,0.,0.));
#73211=CARTESIAN_POINT('',(22.399682944576,37.6689447622493,-5.17040276961776));
#73212=CARTESIAN_POINT('Origin',(22.4,37.674484472081,-5.17065950947565));
#73213=CARTESIAN_POINT('',(21.896707744792,41.9886110647639,-5.12313779357752));
#73214=CARTESIAN_POINT('Origin',(9.86169260701005,0.,0.));
#73215=CARTESIAN_POINT('',(21.7998387845652,37.7020801925101,-4.97344883706828));
#73216=CARTESIAN_POINT('Origin',(21.8,37.7092141076143,-4.97369795887321));
#73217=CARTESIAN_POINT('',(13.103292255208,41.9886110647639,-5.12313779357752));
#73218=CARTESIAN_POINT('',(17.5,41.9886110647639,-5.12313779357752));
#73219=CARTESIAN_POINT('',(13.2021921742626,37.6122086000507,-4.97031045190415));
#73220=CARTESIAN_POINT('Origin',(13.2,37.7092141076143,-4.97369795887321));
#73221=CARTESIAN_POINT('',(12.3548486633046,41.9578594516632,-5.3691740737731));
#73222=CARTESIAN_POINT('Origin',(25.13830739299,0.,0.));
#73223=CARTESIAN_POINT('',(12.6002487187375,37.6701387661531,-5.17045810616099));
#73224=CARTESIAN_POINT('Origin',(12.6,37.674484472081,-5.17065950947565));
#73225=CARTESIAN_POINT('',(11.6618634261911,41.9060788618227,-5.75938837262207));
#73226=CARTESIAN_POINT('Origin',(20.8267261185512,0.,0.));
#73227=CARTESIAN_POINT('',(11.8996457869536,37.6114227454796,-5.56487237189312));
#73228=CARTESIAN_POINT('Origin',(11.9,37.6050252010142,-5.56458261068054));
#73229=CARTESIAN_POINT('',(10.8302042597752,41.8715390397407,-6.00534915250319));
#73230=CARTESIAN_POINT('Origin',(26.9856656232739,0.,0.));
#73231=CARTESIAN_POINT('',(10.899790263986,37.565908154163,-5.86046163546711));
#73232=CARTESIAN_POINT('Origin',(10.9,37.5529307477141,-5.8600249365842));
#73233=CARTESIAN_POINT('',(5.09944803334083,41.9206753505941,-5.65216579287046));
#73234=CARTESIAN_POINT('Origin',(-62.7155570771055,0.,0.));
#73235=CARTESIAN_POINT('',(4.55736144060343,38.0336947942479,-5.48390637564378));
#73236=CARTESIAN_POINT('Origin',(4.5,37.6223900187809,-5.46610183537932));
#73237=CARTESIAN_POINT('',(5.09593997529677,41.9886110647639,-5.12313779357752));
#73238=CARTESIAN_POINT('Origin',(-0.840551718690872,0.,0.));
#73239=CARTESIAN_POINT('',(4.49524972087093,37.6751027358433,-4.97250676352255));
#73240=CARTESIAN_POINT('Origin',(4.5,37.7092141076143,-4.97369795887321));
#73241=CARTESIAN_POINT('',(1.67735469196905,41.9886110647639,-5.12313779357752));
#73242=CARTESIAN_POINT('',(17.5,41.9886110647639,-5.12313779357752));
#73243=CARTESIAN_POINT('',(1.90350512467335,37.6418431848034,-4.97134531440729));
#73244=CARTESIAN_POINT('Origin',(1.9,37.7092141076143,-4.97369795887321));
#73245=CARTESIAN_POINT('',(0.600000000000001,41.8659567209931,-6.04414326732376));
#73246=CARTESIAN_POINT('Origin',(8.14497546096349,0.,0.));
#73247=CARTESIAN_POINT('Ctrl Pts',(0.138207714141615,42.2749056435377,-6.43453435214071));
#73248=CARTESIAN_POINT('Ctrl Pts',(0.370217470893695,42.0700781197368,-6.23839136562887));
#73249=CARTESIAN_POINT('Ctrl Pts',(0.600000000000008,41.8659567209931,-6.04414326732376));
#73250=CARTESIAN_POINT('Origin',(1.9,37.1361751213135,-8.2235635438135));
#73251=CARTESIAN_POINT('',(5.09593997529677,41.2086042970448,-9.54677599452213));
#73252=CARTESIAN_POINT('',(17.5,41.2086042970448,-9.54677599452213));
#73253=CARTESIAN_POINT('',(4.47529854852883,36.9673747121716,-8.16871696615113));
#73254=CARTESIAN_POINT('Origin',(4.5,37.1361751213135,-8.2235635438135));
#73255=CARTESIAN_POINT('',(5.09944803334083,41.325703839893,-9.02641690470011));
#73256=CARTESIAN_POINT('Origin',(-0.840551718690874,0.,0.));
#73257=CARTESIAN_POINT('',(4.50447263544529,37.253610541118,-7.74082391359485));
#73258=CARTESIAN_POINT('Origin',(4.5,37.2229992101469,-7.7311596673074));
#73259=CARTESIAN_POINT('',(10.8302042597752,41.4003266344532,-8.6777274997883));
#73260=CARTESIAN_POINT('Origin',(-62.7155570771054,0.,0.));
#73261=CARTESIAN_POINT('',(10.8987117910442,37.3682767550424,-7.36197779558791));
#73262=CARTESIAN_POINT('Origin',(10.9,37.2924584812137,-7.33723656610251));
#73263=CARTESIAN_POINT('',(11.6618634261911,41.3486599091995,-8.92066834454427));
#73264=CARTESIAN_POINT('Origin',(26.9856656232739,0.,0.));
#73265=CARTESIAN_POINT('',(11.8995413080444,37.2482773116316,-7.63515978098257));
#73266=CARTESIAN_POINT('Origin',(11.9,37.2403640279136,-7.63267889200617));
#73267=CARTESIAN_POINT('',(12.3548486633046,41.2638565969525,-9.30505984645652));
#73268=CARTESIAN_POINT('Origin',(20.8267261185512,0.,0.));
#73269=CARTESIAN_POINT('',(12.600317055424,37.1656113221937,-8.02494855741037));
#73270=CARTESIAN_POINT('Origin',(12.6,37.1709047568469,-8.02660199321106));
#73271=CARTESIAN_POINT('',(13.103292255208,41.2086042970448,-9.54677599452213));
#73272=CARTESIAN_POINT('Origin',(25.13830739299,0.,0.));
#73273=CARTESIAN_POINT('',(13.2001612154348,37.1293862292573,-8.22135769906884));
#73274=CARTESIAN_POINT('Origin',(13.2,37.1361751213135,-8.2235635438135));
#73275=CARTESIAN_POINT('',(21.896707744792,41.2086042970448,-9.54677599452213));
#73276=CARTESIAN_POINT('',(17.5,41.2086042970448,-9.54677599452213));
#73277=CARTESIAN_POINT('',(21.7978078257374,37.0438611660612,-8.19356892151487));
#73278=CARTESIAN_POINT('Origin',(21.8,37.1361751213135,-8.2235635438135));
#73279=CARTESIAN_POINT('',(22.6451513366954,41.2638565969525,-9.30505984645652));
#73280=CARTESIAN_POINT('Origin',(9.86169260701005,0.,0.));
#73281=CARTESIAN_POINT('',(22.3997512812625,37.1667522450638,-8.02530493145534));
#73282=CARTESIAN_POINT('Origin',(22.4,37.1709047568469,-8.02660199321106));
#73283=CARTESIAN_POINT('',(23.3381365738089,41.3486599091995,-8.92066834454427));
#73284=CARTESIAN_POINT('Origin',(14.1732738814488,0.,0.));
#73285=CARTESIAN_POINT('',(23.1003542130464,37.2464748574103,-7.6345946946079));
#73286=CARTESIAN_POINT('Origin',(23.1,37.2403640279136,-7.63267889200617));
#73287=CARTESIAN_POINT('',(24.1697957402248,41.4003266344532,-8.6777274997883));
#73288=CARTESIAN_POINT('Origin',(8.01433437672608,0.,0.));
#73289=CARTESIAN_POINT('',(24.100209736014,37.3048026141052,-7.34126473779837));
#73290=CARTESIAN_POINT('Origin',(24.1,37.2924584812137,-7.33723656610251));
#73291=CARTESIAN_POINT('',(29.9005519666592,41.325703839893,-9.02641690470011));
#73292=CARTESIAN_POINT('Origin',(97.7155570771055,0.,0.));
#73293=CARTESIAN_POINT('',(30.4426385593966,37.6155887839604,-7.85510339046017));
#73294=CARTESIAN_POINT('Origin',(30.5,37.2229992101469,-7.7311596673074));
#73295=CARTESIAN_POINT('',(29.9040600247032,41.2086042970448,-9.54677599452213));
#73296=CARTESIAN_POINT('Origin',(35.8405517186909,0.,0.));
#73297=CARTESIAN_POINT('',(30.5047502791291,37.1037135041708,-8.21301612503228));
#73298=CARTESIAN_POINT('Origin',(30.5,37.1361751213135,-8.2235635438135));
#73299=CARTESIAN_POINT('',(17.5,41.2086042970448,-9.54677599452213));
#73300=CARTESIAN_POINT('Origin',(17.5,42.1005314412719,-7.42345959526127));
#73301=CARTESIAN_POINT('Ctrl Pts',(34.8617922858584,42.2749056435377,-6.4345343521407));
#73302=CARTESIAN_POINT('Ctrl Pts',(34.8382109660635,42.1005314412719,-7.42345959526127));
#73303=CARTESIAN_POINT('Ctrl Pts',(34.8617922858584,41.9261572390061,-8.41238483838185));
#73304=CARTESIAN_POINT('Origin',(34.7,0.,0.));
#73305=CARTESIAN_POINT('',(35.,-42.9,-5.25373476834215E-15));
#73306=CARTESIAN_POINT('Origin',(35.,0.,0.));
#73307=CARTESIAN_POINT('',(34.85,-42.75,-5.28447809747245E-15));
#73308=CARTESIAN_POINT('',(34.7,-42.6,-5.21699536436772E-15));
#73309=CARTESIAN_POINT('Ctrl Pts',(34.85,-42.75,-5.33359112858996E-15));
#73310=CARTESIAN_POINT('Ctrl Pts',(34.85,-42.75,0.50202126500325));
#73311=CARTESIAN_POINT('Ctrl Pts',(34.8617922858584,-42.75,1.00418100903022));
#73312=CARTESIAN_POINT('Origin',(34.4,0.,0.));
#73313=CARTESIAN_POINT('Ctrl Pts',(34.8617922858584,-42.2749056435377,6.43453435214071));
#73314=CARTESIAN_POINT('Ctrl Pts',(34.8382109660634,-42.1005314412719,7.42345959526129));
#73315=CARTESIAN_POINT('Ctrl Pts',(34.8617922858584,-41.926157239006,8.41238483838188));
#73316=CARTESIAN_POINT('Origin',(34.4,0.,0.));
#73317=CARTESIAN_POINT('Ctrl Pts',(34.8617922858584,-40.515309671231,13.6777396430533));
#73318=CARTESIAN_POINT('Ctrl Pts',(34.8382109660634,-40.1718595385976,14.6213611271723));
#73319=CARTESIAN_POINT('Ctrl Pts',(34.8617922858584,-39.8284094059642,15.5649826112914));
#73320=CARTESIAN_POINT('Origin',(34.4,0.,0.));
#73321=CARTESIAN_POINT('Ctrl Pts',(34.8617922858584,-37.5246765162999,20.5053537361819));
#73322=CARTESIAN_POINT('Ctrl Pts',(34.8382109660634,-37.0225860117847,21.375));
#73323=CARTESIAN_POINT('Ctrl Pts',(34.8617922858584,-36.5204955072696,22.2446462638181));
#73324=CARTESIAN_POINT('Origin',(34.4,0.,0.));
#73325=CARTESIAN_POINT('Ctrl Pts',(34.8617922858584,-33.3938750538235,26.7099230322464));
#73326=CARTESIAN_POINT('Ctrl Pts',(34.8382109660634,-32.7483999433363,27.4791703140996));
#73327=CARTESIAN_POINT('Ctrl Pts',(34.8617922858584,-32.1029248328491,28.2484175959528));
#73328=CARTESIAN_POINT('Origin',(34.4,0.,0.));
#73329=CARTESIAN_POINT('Ctrl Pts',(34.8617922858584,-28.2484175959528,32.1029248328492));
#73330=CARTESIAN_POINT('Ctrl Pts',(34.8382109660634,-27.4791703140996,32.7483999433363));
#73331=CARTESIAN_POINT('Ctrl Pts',(34.8617922858584,-26.7099230322463,33.3938750538235));
#73332=CARTESIAN_POINT('Origin',(34.4,0.,0.));
#73333=CARTESIAN_POINT('Ctrl Pts',(34.8617922858584,-22.244646263818,36.5204955072697));
#73334=CARTESIAN_POINT('Ctrl Pts',(34.8382109660635,-21.375,37.0225860117848));
#73335=CARTESIAN_POINT('Ctrl Pts',(34.8617922858584,-20.5053537361819,37.5246765162999));
#73336=CARTESIAN_POINT('Origin',(34.4,0.,0.));
#73337=CARTESIAN_POINT('Ctrl Pts',(34.8617922858584,-15.5649826112914,39.8284094059642));
#73338=CARTESIAN_POINT('Ctrl Pts',(34.8382109660635,-14.6213611271723,40.1718595385976));
#73339=CARTESIAN_POINT('Ctrl Pts',(34.8617922858584,-13.6777396430533,40.515309671231));
#73340=CARTESIAN_POINT('Origin',(34.4,0.,0.));
#73341=CARTESIAN_POINT('Ctrl Pts',(34.8617922858584,-8.41238483838184,41.9261572390061));
#73342=CARTESIAN_POINT('Ctrl Pts',(34.8382109660634,-7.42345959526127,42.1005314412719));
#73343=CARTESIAN_POINT('Ctrl Pts',(34.8617922858584,-6.4345343521407,42.2749056435377));
#73344=CARTESIAN_POINT('Origin',(34.4,0.,0.));
#73345=CARTESIAN_POINT('Ctrl Pts',(34.8617922858584,-1.0041810090302,42.75));
#73346=CARTESIAN_POINT('Ctrl Pts',(34.8382109660635,4.30211422042248E-15,
42.75));
#73347=CARTESIAN_POINT('Ctrl Pts',(34.8617922858584,1.00418100903021,42.75));
#73348=CARTESIAN_POINT('Origin',(34.4,0.,0.));
#73349=CARTESIAN_POINT('Ctrl Pts',(34.8617922858584,6.4345343521407,42.2749056435377));
#73350=CARTESIAN_POINT('Ctrl Pts',(34.8382109660634,7.42345959526127,42.1005314412719));
#73351=CARTESIAN_POINT('Ctrl Pts',(34.8617922858584,8.41238483838185,41.9261572390061));
#73352=CARTESIAN_POINT('Origin',(34.4,0.,0.));
#73353=CARTESIAN_POINT('Ctrl Pts',(34.8617922858584,13.6777396430533,40.515309671231));
#73354=CARTESIAN_POINT('Ctrl Pts',(34.8382109660634,14.6213611271723,40.1718595385976));
#73355=CARTESIAN_POINT('Ctrl Pts',(34.8617922858584,15.5649826112914,39.8284094059642));
#73356=CARTESIAN_POINT('Origin',(34.4,0.,0.));
#73357=CARTESIAN_POINT('Ctrl Pts',(34.8617922858584,20.5053537361819,37.5246765162999));
#73358=CARTESIAN_POINT('Ctrl Pts',(34.8382109660634,21.375,37.0225860117847));
#73359=CARTESIAN_POINT('Ctrl Pts',(34.8617922858584,22.2446462638181,36.5204955072696));
#73360=CARTESIAN_POINT('Origin',(34.4,0.,0.));
#73361=CARTESIAN_POINT('Ctrl Pts',(34.8617922858584,26.7099230322463,33.3938750538235));
#73362=CARTESIAN_POINT('Ctrl Pts',(34.8382109660634,27.4791703140995,32.7483999433363));
#73363=CARTESIAN_POINT('Ctrl Pts',(34.8617922858584,28.2484175959528,32.1029248328492));
#73364=CARTESIAN_POINT('Origin',(34.4,0.,0.));
#73365=CARTESIAN_POINT('Ctrl Pts',(34.8617922858584,32.1029248328492,28.2484175959528));
#73366=CARTESIAN_POINT('Ctrl Pts',(34.8382109660634,32.7483999433363,27.4791703140995));
#73367=CARTESIAN_POINT('Ctrl Pts',(34.8617922858584,33.3938750538235,26.7099230322464));
#73368=CARTESIAN_POINT('Origin',(34.4,0.,0.));
#73369=CARTESIAN_POINT('Ctrl Pts',(34.8617922858584,36.5204955072696,22.244646263818));
#73370=CARTESIAN_POINT('Ctrl Pts',(34.8382109660634,37.0225860117847,21.375));
#73371=CARTESIAN_POINT('Ctrl Pts',(34.8617922858584,37.5246765162998,20.5053537361819));
#73372=CARTESIAN_POINT('Origin',(34.4,0.,0.));
#73373=CARTESIAN_POINT('Ctrl Pts',(34.8617922858584,39.8284094059642,15.5649826112914));
#73374=CARTESIAN_POINT('Ctrl Pts',(34.8382109660635,40.1718595385976,14.6213611271723));
#73375=CARTESIAN_POINT('Ctrl Pts',(34.8617922858584,40.515309671231,13.6777396430533));
#73376=CARTESIAN_POINT('Origin',(34.4,0.,0.));
#73377=CARTESIAN_POINT('Ctrl Pts',(34.8617922858584,41.9261572390061,8.41238483838185));
#73378=CARTESIAN_POINT('Ctrl Pts',(34.8382109660634,42.1005314412719,7.42345959526127));
#73379=CARTESIAN_POINT('Ctrl Pts',(34.8617922858584,42.2749056435377,6.4345343521407));
#73380=CARTESIAN_POINT('Origin',(34.4,0.,0.));
#73381=CARTESIAN_POINT('',(34.4,42.2794732300362,-1.31762794090604));
#73382=CARTESIAN_POINT('Ctrl Pts',(34.8617922858584,42.75,-1.00418100903021));
#73383=CARTESIAN_POINT('Ctrl Pts',(34.6297825290987,42.5142243943529,-1.16177621660715));
#73384=CARTESIAN_POINT('Ctrl Pts',(34.4,42.2794732300361,-1.31762794090604));
#73385=CARTESIAN_POINT('Origin',(34.4,0.,0.));
#73386=CARTESIAN_POINT('Origin',(34.4,0.,0.));
#73387=CARTESIAN_POINT('Ctrl Pts',(34.8617922858584,40.515309671231,-13.6777396430533));
#73388=CARTESIAN_POINT('Ctrl Pts',(34.8382109660634,40.1718595385976,-14.6213611271724));
#73389=CARTESIAN_POINT('Ctrl Pts',(34.8617922858584,39.8284094059641,-15.5649826112914));
#73390=CARTESIAN_POINT('Origin',(34.4,0.,0.));
#73391=CARTESIAN_POINT('Ctrl Pts',(34.8617922858584,37.5246765162999,-20.505353736182));
#73392=CARTESIAN_POINT('Ctrl Pts',(34.8382109660634,37.0225860117847,-21.375));
#73393=CARTESIAN_POINT('Ctrl Pts',(34.8617922858584,36.5204955072696,-22.2446462638181));
#73394=CARTESIAN_POINT('Origin',(34.4,0.,0.));
#73395=CARTESIAN_POINT('Ctrl Pts',(34.8617922858584,33.3938750538235,-26.7099230322464));
#73396=CARTESIAN_POINT('Ctrl Pts',(34.8382109660635,32.7483999433363,-27.4791703140996));
#73397=CARTESIAN_POINT('Ctrl Pts',(34.8617922858584,32.1029248328491,-28.2484175959528));
#73398=CARTESIAN_POINT('Origin',(34.4,0.,0.));
#73399=CARTESIAN_POINT('Ctrl Pts',(34.8617922858584,28.2484175959528,-32.1029248328492));
#73400=CARTESIAN_POINT('Ctrl Pts',(34.8382109660634,27.4791703140995,-32.7483999433363));
#73401=CARTESIAN_POINT('Ctrl Pts',(34.8617922858584,26.7099230322463,-33.3938750538235));
#73402=CARTESIAN_POINT('Origin',(34.4,0.,0.));
#73403=CARTESIAN_POINT('Ctrl Pts',(34.8617922858584,22.2446462638181,-36.5204955072696));
#73404=CARTESIAN_POINT('Ctrl Pts',(34.8382109660635,21.375,-37.0225860117847));
#73405=CARTESIAN_POINT('Ctrl Pts',(34.8617922858584,20.505353736182,-37.5246765162999));
#73406=CARTESIAN_POINT('Origin',(34.4,0.,0.));
#73407=CARTESIAN_POINT('Ctrl Pts',(34.8617922858584,15.5649826112914,-39.8284094059642));
#73408=CARTESIAN_POINT('Ctrl Pts',(34.8382109660634,14.6213611271723,-40.1718595385976));
#73409=CARTESIAN_POINT('Ctrl Pts',(34.8617922858584,13.6777396430533,-40.515309671231));
#73410=CARTESIAN_POINT('Origin',(34.4,0.,0.));
#73411=CARTESIAN_POINT('Ctrl Pts',(34.8617922858584,8.41238483838183,-41.9261572390061));
#73412=CARTESIAN_POINT('Ctrl Pts',(34.8382109660635,7.42345959526126,-42.1005314412719));
#73413=CARTESIAN_POINT('Ctrl Pts',(34.8617922858584,6.43453435214068,-42.2749056435377));
#73414=CARTESIAN_POINT('Origin',(34.4,0.,0.));
#73415=CARTESIAN_POINT('Ctrl Pts',(34.8617922858584,1.0041810090302,-42.75));
#73416=CARTESIAN_POINT('Ctrl Pts',(34.8382109660634,-8.74300631892311E-15,
-42.75));
#73417=CARTESIAN_POINT('Ctrl Pts',(34.8617922858584,-1.00418100903022,-42.75));
#73418=CARTESIAN_POINT('Origin',(34.4,0.,0.));
#73419=CARTESIAN_POINT('Ctrl Pts',(34.8617922858584,-6.4345343521407,-42.2749056435377));
#73420=CARTESIAN_POINT('Ctrl Pts',(34.8382109660634,-7.42345959526127,-42.1005314412719));
#73421=CARTESIAN_POINT('Ctrl Pts',(34.8617922858584,-8.41238483838184,-41.9261572390061));
#73422=CARTESIAN_POINT('Origin',(34.4,0.,0.));
#73423=CARTESIAN_POINT('Ctrl Pts',(34.8617922858584,-13.6777396430533,-40.515309671231));
#73424=CARTESIAN_POINT('Ctrl Pts',(34.8382109660634,-14.6213611271724,-40.1718595385976));
#73425=CARTESIAN_POINT('Ctrl Pts',(34.8617922858584,-15.5649826112914,-39.8284094059641));
#73426=CARTESIAN_POINT('Origin',(34.4,0.,0.));
#73427=CARTESIAN_POINT('Ctrl Pts',(34.8617922858584,-20.505353736182,-37.5246765162999));
#73428=CARTESIAN_POINT('Ctrl Pts',(34.8382109660634,-21.375,-37.0225860117847));
#73429=CARTESIAN_POINT('Ctrl Pts',(34.8617922858584,-22.2446462638181,-36.5204955072696));
#73430=CARTESIAN_POINT('Origin',(34.4,0.,0.));
#73431=CARTESIAN_POINT('Ctrl Pts',(34.8617922858584,-26.7099230322464,-33.3938750538235));
#73432=CARTESIAN_POINT('Ctrl Pts',(34.8382109660634,-27.4791703140996,-32.7483999433363));
#73433=CARTESIAN_POINT('Ctrl Pts',(34.8617922858584,-28.2484175959528,-32.1029248328491));
#73434=CARTESIAN_POINT('Origin',(34.4,0.,0.));
#73435=CARTESIAN_POINT('Ctrl Pts',(34.8617922858584,-32.1029248328492,-28.2484175959528));
#73436=CARTESIAN_POINT('Ctrl Pts',(34.8382109660634,-32.7483999433363,-27.4791703140995));
#73437=CARTESIAN_POINT('Ctrl Pts',(34.8617922858584,-33.3938750538235,-26.7099230322464));
#73438=CARTESIAN_POINT('Origin',(34.4,0.,0.));
#73439=CARTESIAN_POINT('Ctrl Pts',(34.8617922858584,-36.5204955072697,-22.244646263818));
#73440=CARTESIAN_POINT('Ctrl Pts',(34.8382109660634,-37.0225860117848,-21.375));
#73441=CARTESIAN_POINT('Ctrl Pts',(34.8617922858584,-37.5246765162999,-20.5053537361819));
#73442=CARTESIAN_POINT('Origin',(34.4,0.,0.));
#73443=CARTESIAN_POINT('Ctrl Pts',(34.8617922858584,-39.8284094059642,-15.5649826112914));
#73444=CARTESIAN_POINT('Ctrl Pts',(34.8382109660635,-40.1718595385976,-14.6213611271723));
#73445=CARTESIAN_POINT('Ctrl Pts',(34.8617922858584,-40.515309671231,-13.6777396430533));
#73446=CARTESIAN_POINT('Origin',(34.4,0.,0.));
#73447=CARTESIAN_POINT('Ctrl Pts',(34.8617922858584,-41.9261572390061,-8.41238483838183));
#73448=CARTESIAN_POINT('Ctrl Pts',(34.8382109660635,-42.1005314412719,-7.42345959526126));
#73449=CARTESIAN_POINT('Ctrl Pts',(34.8617922858584,-42.2749056435377,-6.43453435214069));
#73450=CARTESIAN_POINT('Origin',(34.4,0.,0.));
#73451=CARTESIAN_POINT('Ctrl Pts',(34.8617922858584,-42.75,-1.0041810090302));
#73452=CARTESIAN_POINT('Ctrl Pts',(34.85,-42.75,-0.502021265003246));
#73453=CARTESIAN_POINT('Ctrl Pts',(34.85,-42.75,-5.33359112858996E-15));
#73454=CARTESIAN_POINT('Origin',(17.5,0.,0.));
#73455=CARTESIAN_POINT('',(0.600000000000001,40.1803643021789,-13.22226624086));
#73456=CARTESIAN_POINT('Origin',(0.600000000000001,0.,0.));
#73457=CARTESIAN_POINT('',(1.67735469196905,40.4610861730024,-12.3365516130268));
#73458=CARTESIAN_POINT('Origin',(8.14497546096349,0.,0.));
#73459=CARTESIAN_POINT('',(5.09593997529677,40.4610861730024,-12.3365516130268));
#73460=CARTESIAN_POINT('',(17.5,40.4610861730024,-12.3365516130268));
#73461=CARTESIAN_POINT('',(5.09944803334083,40.3023178069695,-12.8457455753269));
#73462=CARTESIAN_POINT('Origin',(-0.840551718690872,0.,0.));
#73463=CARTESIAN_POINT('',(10.8302042597752,40.1925983403041,-13.1850308552912));
#73464=CARTESIAN_POINT('Origin',(-62.7155570771055,0.,0.));
#73465=CARTESIAN_POINT('',(11.6618634261911,40.2693240660821,-12.9488045494888));
#73466=CARTESIAN_POINT('Origin',(26.9856656232739,0.,0.));
#73467=CARTESIAN_POINT('',(12.3548486633046,40.3880779943072,-12.5735100877104));
#73468=CARTESIAN_POINT('Origin',(20.8267261185512,0.,0.));
#73469=CARTESIAN_POINT('',(13.103292255208,40.4610861730024,-12.3365516130268));
#73470=CARTESIAN_POINT('Origin',(25.13830739299,0.,0.));
#73471=CARTESIAN_POINT('',(21.896707744792,40.4610861730024,-12.3365516130268));
#73472=CARTESIAN_POINT('',(17.5,40.4610861730024,-12.3365516130268));
#73473=CARTESIAN_POINT('',(22.6451513366954,40.3880779943072,-12.5735100877104));
#73474=CARTESIAN_POINT('Origin',(9.86169260701006,0.,0.));
#73475=CARTESIAN_POINT('',(23.3381365738089,40.2693240660821,-12.9488045494888));
#73476=CARTESIAN_POINT('Origin',(14.1732738814488,0.,0.));
#73477=CARTESIAN_POINT('',(24.1697957402248,40.1925983403041,-13.1850308552912));
#73478=CARTESIAN_POINT('Origin',(8.01433437672608,0.,0.));
#73479=CARTESIAN_POINT('',(29.9005519666592,40.3023178069695,-12.8457455753269));
#73480=CARTESIAN_POINT('Origin',(97.7155570771054,0.,0.));
#73481=CARTESIAN_POINT('',(29.9040600247032,40.4610861730024,-12.3365516130268));
#73482=CARTESIAN_POINT('Origin',(35.8405517186909,0.,0.));
#73483=CARTESIAN_POINT('',(17.5,40.4610861730024,-12.3365516130268));
#73484=CARTESIAN_POINT('Origin',(33.1,36.2726528263519,-11.4462726220787));
#73485=CARTESIAN_POINT('',(30.5247014514712,36.0990440950346,-11.409370947074));
#73486=CARTESIAN_POINT('Origin',(30.5,36.2726528263519,-11.4462726220787));
#73487=CARTESIAN_POINT('',(30.4955273645547,36.1329850680974,-11.9230551151638));
#73488=CARTESIAN_POINT('Origin',(30.5,36.101642754689,-11.9161189324716));
#73489=CARTESIAN_POINT('',(24.1012882089558,36.0428658633082,-12.3084785844451));
#73490=CARTESIAN_POINT('Origin',(24.1,35.9648346973588,-12.291995980786));
#73491=CARTESIAN_POINT('',(23.1004586919557,36.0755342895717,-12.0118963235317));
#73492=CARTESIAN_POINT('Origin',(23.1,36.0674407403565,-12.0100881945502));
#73493=CARTESIAN_POINT('',(22.399682944576,36.1988378309035,-11.6329963463162));
#73494=CARTESIAN_POINT('Origin',(22.4,36.2042487976867,-11.6342111462359));
#73495=CARTESIAN_POINT('',(21.7998387845652,36.2656705509953,-11.4447884936363));
#73496=CARTESIAN_POINT('Origin',(21.8,36.2726528263519,-11.4462726220787));
#73497=CARTESIAN_POINT('',(13.2021921742626,36.1777092848303,-11.4260917493401));
#73498=CARTESIAN_POINT('Origin',(13.2,36.2726528263519,-11.4462726220787));
#73499=CARTESIAN_POINT('',(12.6002487187375,36.2000040861152,-11.633258178775));
#73500=CARTESIAN_POINT('Origin',(12.6,36.2042487976867,-11.6342111462359));
#73501=CARTESIAN_POINT('',(11.8996457869536,36.0736907752397,-12.0114844755769));
#73502=CARTESIAN_POINT('Origin',(11.9,36.0674407403565,-12.0100881945502));
#73503=CARTESIAN_POINT('',(10.899790263986,35.9775391158784,-12.2946795482123));
#73504=CARTESIAN_POINT('Origin',(10.9,35.9648346973588,-12.291995980786));
#73505=CARTESIAN_POINT('',(4.55736144060343,36.5036071604488,-12.0050753064885));
#73506=CARTESIAN_POINT('Origin',(4.5,36.101642754689,-11.9161189324716));
#73507=CARTESIAN_POINT('',(4.49524972087093,36.2392665318678,-11.4391761461162));
#73508=CARTESIAN_POINT('Origin',(4.5,36.2726528263519,-11.4462726220787));
#73509=CARTESIAN_POINT('',(1.90350512467335,36.2067139516643,-11.4322568815947));
#73510=CARTESIAN_POINT('Origin',(1.9,36.2726528263519,-11.4462726220787));
#73511=CARTESIAN_POINT('Ctrl Pts',(0.13820771414162,40.515309671231,-13.6777396430533));
#73512=CARTESIAN_POINT('Ctrl Pts',(0.370217470898406,40.3476538099281,-13.4490085829888));
#73513=CARTESIAN_POINT('Ctrl Pts',(0.600000000000009,40.1803643021789,-13.22226624086));
#73514=CARTESIAN_POINT('Origin',(1.9,35.1439863533772,-14.5472582706722));
#73515=CARTESIAN_POINT('',(5.09593997529677,38.9247727484987,-16.5575380560557));
#73516=CARTESIAN_POINT('',(17.5,38.9247727484987,-16.5575380560557));
#73517=CARTESIAN_POINT('',(4.47529854852883,34.987274410005,-14.4639330523272));
#73518=CARTESIAN_POINT('Origin',(4.5,35.1439863533772,-14.5472582706722));
#73519=CARTESIAN_POINT('',(5.09944803334083,39.1304526938498,-16.0654185122698));
#73520=CARTESIAN_POINT('Origin',(-0.840551718690874,0.,0.));
#73521=CARTESIAN_POINT('',(4.50447263544529,35.343464522354,-14.0922449867892));
#73522=CARTESIAN_POINT('Origin',(4.5,35.31499642504,-14.0774119602792));
#73523=CARTESIAN_POINT('',(10.8302042597752,39.2644910802189,-15.7349845952073));
#73524=CARTESIAN_POINT('Origin',(-62.7155570771055,0.,0.));
#73525=CARTESIAN_POINT('',(10.8987117910442,35.5221746368434,-13.7390659716653));
#73526=CARTESIAN_POINT('Origin',(10.9,35.4518044823703,-13.7015349119649));
#73527=CARTESIAN_POINT('',(11.6618634261911,39.1714230536436,-15.96526278996));
#73528=CARTESIAN_POINT('Origin',(26.9856656232739,0.,0.));
#73529=CARTESIAN_POINT('',(11.8995413080444,35.35656070068,-13.9872600241959));
#73530=CARTESIAN_POINT('Origin',(11.9,35.3491984393726,-13.9834426982006));
#73531=CARTESIAN_POINT('',(12.3548486633046,39.0211592104439,-16.3290885806033));
#73532=CARTESIAN_POINT('Origin',(20.8267261185512,0.,0.));
#73533=CARTESIAN_POINT('',(12.600317055424,35.2074644826695,-14.3567722348383));
#73534=CARTESIAN_POINT('Origin',(12.6,35.2123903820423,-14.359319746515));
#73535=CARTESIAN_POINT('',(13.103292255208,38.9247727484987,-16.5575380560557));
#73536=CARTESIAN_POINT('Origin',(25.13830739299,0.,0.));
#73537=CARTESIAN_POINT('',(13.2001612154348,35.137683640766,-14.5439070589318));
#73538=CARTESIAN_POINT('Origin',(13.2,35.1439863533772,-14.5472582706722));
#73539=CARTESIAN_POINT('',(21.896707744792,38.9247727484987,-16.5575380560557));
#73540=CARTESIAN_POINT('',(17.5,38.9247727484987,-16.5575380560557));
#73541=CARTESIAN_POINT('',(21.7978078257374,35.0582833660355,-14.501689183981));
#73542=CARTESIAN_POINT('Origin',(21.8,35.1439863533772,-14.5472582706722));
#73543=CARTESIAN_POINT('',(22.6451513366954,39.0211592104439,-16.3290885806033));
#73544=CARTESIAN_POINT('Origin',(9.86169260701006,0.,0.));
#73545=CARTESIAN_POINT('',(22.3997512812625,35.208526188654,-14.357321313938));
#73546=CARTESIAN_POINT('Origin',(22.4,35.2123903820423,-14.359319746515));
#73547=CARTESIAN_POINT('',(23.3381365738089,39.1714230536436,-15.96526278996));
#73548=CARTESIAN_POINT('Origin',(14.1732738814488,0.,0.));
#73549=CARTESIAN_POINT('',(23.1003542130464,35.3548837560077,-13.9863905298622));
#73550=CARTESIAN_POINT('Origin',(23.1,35.3491984393726,-13.9834426982006));
#73551=CARTESIAN_POINT('',(24.1697957402248,39.2644910802189,-15.7349845952073));
#73552=CARTESIAN_POINT('Origin',(8.01433437672606,0.,0.));
#73553=CARTESIAN_POINT('',(24.100209736014,35.4632615954716,-13.7076454228629));
#73554=CARTESIAN_POINT('Origin',(24.1,35.4518044823703,-13.7015349119649));
#73555=CARTESIAN_POINT('',(29.9005519666592,39.1304526938498,-16.0654185122698));
#73556=CARTESIAN_POINT('Origin',(97.7155570771054,0.,0.));
#73557=CARTESIAN_POINT('',(30.4426385593966,35.6800990794245,-14.267645163841));
#73558=CARTESIAN_POINT('Origin',(30.5,35.31499642504,-14.0774119602792));
#73559=CARTESIAN_POINT('',(29.9040600247032,38.9247727484987,-16.5575380560557));
#73560=CARTESIAN_POINT('Origin',(35.8405517186909,0.,0.));
#73561=CARTESIAN_POINT('',(30.5047502791291,35.1138494411902,-14.5312341902212));
#73562=CARTESIAN_POINT('Origin',(30.5,35.1439863533772,-14.5472582706722));
#73563=CARTESIAN_POINT('',(17.5,38.9247727484987,-16.5575380560557));
#73564=CARTESIAN_POINT('Origin',(17.5,40.1718595385976,-14.6213611271724));
#73565=CARTESIAN_POINT('Origin',(17.5,0.,0.));
#73566=CARTESIAN_POINT('',(0.600000000000001,37.2739118462884,-19.9986373454573));
#73567=CARTESIAN_POINT('Origin',(0.600000000000001,0.,0.));
#73568=CARTESIAN_POINT('',(1.67735469196905,37.7041716521717,-19.1751255543105));
#73569=CARTESIAN_POINT('Origin',(8.14497546096349,0.,0.));
#73570=CARTESIAN_POINT('',(5.09593997529677,37.7041716521717,-19.1751255543105));
#73571=CARTESIAN_POINT('',(17.5,37.7041716521717,-19.1751255543105));
#73572=CARTESIAN_POINT('',(5.09944803334083,37.459394730737,-19.6490138787379));
#73573=CARTESIAN_POINT('Origin',(-0.840551718690872,0.,0.));
#73574=CARTESIAN_POINT('',(10.8302042597752,37.2924258787336,-19.9640920674886));
#73575=CARTESIAN_POINT('Origin',(-62.7155570771055,0.,0.));
#73576=CARTESIAN_POINT('',(11.6618634261911,37.4090062358548,-19.7447778525305));
#73577=CARTESIAN_POINT('Origin',(26.9856656232739,0.,0.));
#73578=CARTESIAN_POINT('',(12.3548486633046,37.5911252244478,-19.3958063601357));
#73579=CARTESIAN_POINT('Origin',(20.8267261185512,0.,0.));
#73580=CARTESIAN_POINT('',(13.103292255208,37.7041716521717,-19.1751255543105));
#73581=CARTESIAN_POINT('Origin',(25.13830739299,0.,0.));
#73582=CARTESIAN_POINT('',(21.896707744792,37.7041716521717,-19.1751255543105));
#73583=CARTESIAN_POINT('',(17.5,37.7041716521717,-19.1751255543105));
#73584=CARTESIAN_POINT('',(22.6451513366954,37.5911252244478,-19.3958063601357));
#73585=CARTESIAN_POINT('Origin',(9.86169260701006,0.,0.));
#73586=CARTESIAN_POINT('',(23.3381365738089,37.4090062358548,-19.7447778525305));
#73587=CARTESIAN_POINT('Origin',(14.1732738814488,0.,0.));
#73588=CARTESIAN_POINT('',(24.1697957402248,37.2924258787336,-19.9640920674886));
#73589=CARTESIAN_POINT('Origin',(8.01433437672609,0.,0.));
#73590=CARTESIAN_POINT('',(29.9005519666592,37.459394730737,-19.6490138787379));
#73591=CARTESIAN_POINT('Origin',(97.7155570771054,0.,0.));
#73592=CARTESIAN_POINT('',(29.9040600247032,37.7041716521717,-19.1751255543105));
#73593=CARTESIAN_POINT('Origin',(35.8405517186909,0.,0.));
#73594=CARTESIAN_POINT('',(17.5,37.7041716521717,-19.1751255543105));
#73595=CARTESIAN_POINT('Origin',(33.1,33.7339653438087,-17.5710580837557));
#73596=CARTESIAN_POINT('',(30.5247014514712,33.5694020278342,-17.5045701882916));
#73597=CARTESIAN_POINT('Origin',(30.5,33.7339653438087,-17.5710580837557));
#73598=CARTESIAN_POINT('',(30.4955273645547,33.5136270415661,-18.0163441277467));
#73599=CARTESIAN_POINT('Origin',(30.5,33.4839653438087,-18.0040707856479));
#73600=CARTESIAN_POINT('',(24.1012882089558,33.3579488669236,-18.3802631128034));
#73601=CARTESIAN_POINT('Origin',(24.1,33.2839653438087,-18.3504809471617));
#73602=CARTESIAN_POINT('',(23.1004586919557,33.4416219555226,-18.0938594155378));
#73603=CARTESIAN_POINT('Origin',(23.1,33.4339653438087,-18.0906733260264));
#73604=CARTESIAN_POINT('',(22.399682944576,33.6288475295615,-17.742127215612));
#73605=CARTESIAN_POINT('Origin',(22.4,33.6339653438087,-17.7442631645126));
#73606=CARTESIAN_POINT('',(21.7998387845652,33.7273468611033,-17.5683840431675));
#73607=CARTESIAN_POINT('Origin',(21.8,33.7339653438087,-17.5710580837557));
#73608=CARTESIAN_POINT('',(13.2021921742626,33.6439685797945,-17.5346970308537));
#73609=CARTESIAN_POINT('Origin',(13.2,33.7339653438087,-17.5710580837557));
#73610=CARTESIAN_POINT('',(12.6002487187375,33.6299506000067,-17.7425875883397));
#73611=CARTESIAN_POINT('Origin',(12.6,33.6339653438087,-17.7442631645126));
#73612=CARTESIAN_POINT('',(11.8996457869536,33.4398779649625,-18.0931337015746));
#73613=CARTESIAN_POINT('Origin',(11.9,33.4339653438087,-18.0906733260264));
#73614=CARTESIAN_POINT('',(10.899790263986,33.2960107570711,-18.3553298442931));
#73615=CARTESIAN_POINT('Origin',(10.9,33.2839653438087,-18.3504809471617));
#73616=CARTESIAN_POINT('',(4.55736144060343,33.8643758947959,-18.1614760990067));
#73617=CARTESIAN_POINT('Origin',(4.5,33.4839653438087,-18.0040707856479));
#73618=CARTESIAN_POINT('',(4.49524972087093,33.7023185522751,-17.5582719500126));
#73619=CARTESIAN_POINT('Origin',(4.5,33.7339653438087,-17.5710580837557));
#73620=CARTESIAN_POINT('',(1.90350512467335,33.6714620365851,-17.5458051084359));
#73621=CARTESIAN_POINT('Origin',(1.9,33.7339653438087,-17.5710580837557));
#73622=CARTESIAN_POINT('Ctrl Pts',(0.138207714141623,37.5246765162998,-20.505353736182));
#73623=CARTESIAN_POINT('Ctrl Pts',(0.370217470896568,37.3992864560078,-20.2509844800873));
#73624=CARTESIAN_POINT('Ctrl Pts',(0.600000000000009,37.2739118462884,-19.9986373454573));
#73625=CARTESIAN_POINT('Origin',(1.9,32.0839653438087,-20.4289419162443));
#73626=CARTESIAN_POINT('',(5.09593997529677,35.4582316768749,-23.0652077022745));
#73627=CARTESIAN_POINT('',(17.5,35.4582316768749,-23.0652077022745));
#73628=CARTESIAN_POINT('',(4.47529854852883,31.9441034793054,-20.3196698518115));
#73629=CARTESIAN_POINT('Origin',(4.5,32.0839653438087,-20.4289419162443));
#73630=CARTESIAN_POINT('',(5.09944803334083,35.7462425436685,-22.6162805078382));
#73631=CARTESIAN_POINT('Origin',(-0.840551718690874,0.,0.));
#73632=CARTESIAN_POINT('',(4.50447263544529,32.3594252187343,-20.01548032708));
#73633=CARTESIAN_POINT('Origin',(4.5,32.3339653438087,-19.9959292143521));
#73634=CARTESIAN_POINT('',(10.8302042597752,35.9356238333033,-22.3141421459872));
#73635=CARTESIAN_POINT('Origin',(-62.7155570771054,0.,0.));
#73636=CARTESIAN_POINT('',(10.8987117910442,32.5967492173915,-19.6986995804965));
#73637=CARTESIAN_POINT('Origin',(10.9,32.5339653438087,-19.6495190528383));
#73638=CARTESIAN_POINT('',(11.6618634261911,35.8039823302991,-22.5247608043155));
#73639=CARTESIAN_POINT('Origin',(26.9856656232739,0.,0.));
#73640=CARTESIAN_POINT('',(11.8995413080444,32.3905528841213,-19.9143644494692));
#73641=CARTESIAN_POINT('Origin',(11.9,32.3839653438087,-19.9093266739737));
#73642=CARTESIAN_POINT('',(12.3548486633046,35.5928236469852,-22.856966221146));
#73643=CARTESIAN_POINT('Origin',(20.8267261185512,0.,0.));
#73644=CARTESIAN_POINT('',(12.600317055424,32.179556650676,-20.2523726527879));
#73645=CARTESIAN_POINT('Origin',(12.6,32.1839653438087,-20.2557368354875));
#73646=CARTESIAN_POINT('',(13.103292255208,35.4582316768749,-23.0652077022745));
#73647=CARTESIAN_POINT('Origin',(25.13830739299,0.,0.));
#73648=CARTESIAN_POINT('',(13.2001612154348,32.0783403153759,-20.4245471623811));
#73649=CARTESIAN_POINT('Origin',(13.2,32.0839653438087,-20.4289419162443));
#73650=CARTESIAN_POINT('',(21.896707744792,35.4582316768749,-23.0652077022745));
#73651=CARTESIAN_POINT('',(17.5,35.4582316768749,-23.0652077022745));
#73652=CARTESIAN_POINT('',(21.7978078257374,32.0074773662801,-20.3691829588007));
#73653=CARTESIAN_POINT('Origin',(21.8,32.0839653438087,-20.4289419162443));
#73654=CARTESIAN_POINT('',(22.6451513366954,35.5928236469852,-22.856966221146));
#73655=CARTESIAN_POINT('Origin',(9.86169260701005,0.,0.));
#73656=CARTESIAN_POINT('',(22.3997512812625,32.180506880376,-20.2530977534517));
#73657=CARTESIAN_POINT('Origin',(22.4,32.1839653438087,-20.2557368354875));
#73658=CARTESIAN_POINT('',(23.3381365738089,35.8039823302991,-22.5247608043155));
#73659=CARTESIAN_POINT('Origin',(14.1732738814488,0.,0.));
#73660=CARTESIAN_POINT('',(23.1003542130464,32.3890524021132,-19.9132169663217));
#73661=CARTESIAN_POINT('Origin',(23.1,32.3839653438087,-19.9093266739737));
#73662=CARTESIAN_POINT('',(24.1697957402248,35.9356238333033,-22.3141421459872));
#73663=CARTESIAN_POINT('Origin',(8.01433437672607,0.,0.));
#73664=CARTESIAN_POINT('',(24.100209736014,32.544187318536,-19.657526238157));
#73665=CARTESIAN_POINT('Origin',(24.1,32.5339653438087,-19.6495190528383));
#73666=CARTESIAN_POINT('',(29.9005519666592,35.7462425436685,-22.6162805078382));
#73667=CARTESIAN_POINT('Origin',(97.7155570771054,0.,0.));
#73668=CARTESIAN_POINT('',(30.4426385593966,32.6604876193616,-20.2466717586954));
#73669=CARTESIAN_POINT('Origin',(30.5,32.3339653438087,-19.9959292143521));
#73670=CARTESIAN_POINT('',(29.9040600247032,35.4582316768749,-23.0652077022745));
#73671=CARTESIAN_POINT('Origin',(35.8405517186909,0.,0.));
#73672=CARTESIAN_POINT('',(30.5047502791291,32.0570688314042,-20.4079280576996));
#73673=CARTESIAN_POINT('Origin',(30.5,32.0839653438087,-20.4289419162443));
#73674=CARTESIAN_POINT('',(17.5,35.4582316768749,-23.0652077022745));
#73675=CARTESIAN_POINT('Origin',(17.5,37.0225860117847,-21.375));
#73676=CARTESIAN_POINT('Origin',(17.5,0.,0.));
#73677=CARTESIAN_POINT('',(0.600000000000001,33.234910440458,-26.1673599741116));
#73678=CARTESIAN_POINT('Origin',(0.600000000000001,0.,0.));
#73679=CARTESIAN_POINT('',(1.67735469196904,33.8016349549212,-25.4310730087083));
#73680=CARTESIAN_POINT('Origin',(8.14497546096349,0.,0.));
#73681=CARTESIAN_POINT('',(5.09593997529677,33.8016349549212,-25.4310730087083));
#73682=CARTESIAN_POINT('',(17.5,33.8016349549212,-25.4310730087083));
#73683=CARTESIAN_POINT('',(5.09944803334083,33.4782869009793,-25.8552568383243));
#73684=CARTESIAN_POINT('Origin',(-0.840551718690872,0.,0.));
#73685=CARTESIAN_POINT('',(10.8302042597752,33.2591419277157,-26.1365544445335));
#73686=CARTESIAN_POINT('Origin',(-62.7155570771055,0.,0.));
#73687=CARTESIAN_POINT('',(11.6618634261911,33.4120346810215,-25.9408160718628));
#73688=CARTESIAN_POINT('Origin',(26.9856656232739,0.,0.));
#73689=CARTESIAN_POINT('',(12.3548486633046,33.6519851366708,-25.6287708710599));
#73690=CARTESIAN_POINT('Origin',(20.8267261185512,0.,0.));
#73691=CARTESIAN_POINT('',(13.103292255208,33.8016349549212,-25.4310730087083));
#73692=CARTESIAN_POINT('Origin',(25.13830739299,0.,0.));
#73693=CARTESIAN_POINT('',(21.896707744792,33.8016349549212,-25.4310730087083));
#73694=CARTESIAN_POINT('',(17.5,33.8016349549212,-25.4310730087083));
#73695=CARTESIAN_POINT('',(22.6451513366954,33.6519851366708,-25.6287708710599));
#73696=CARTESIAN_POINT('Origin',(9.86169260701004,0.,0.));
#73697=CARTESIAN_POINT('',(23.3381365738089,33.4120346810215,-25.9408160718628));
#73698=CARTESIAN_POINT('Origin',(14.1732738814488,0.,0.));
#73699=CARTESIAN_POINT('',(24.1697957402248,33.2591419277157,-26.1365544445335));
#73700=CARTESIAN_POINT('Origin',(8.01433437672609,0.,0.));
#73701=CARTESIAN_POINT('',(29.9005519666592,33.4782869009793,-25.8552568383243));
#73702=CARTESIAN_POINT('Origin',(97.7155570771054,0.,0.));
#73703=CARTESIAN_POINT('',(29.9040600247032,33.8016349549212,-25.4310730087083));
#73704=CARTESIAN_POINT('Origin',(35.8405517186909,0.,0.));
#73705=CARTESIAN_POINT('',(17.5,33.8016349549212,-25.4310730087083));
#73706=CARTESIAN_POINT('Origin',(33.1,30.1702883945039,-23.1619558369422));
#73707=CARTESIAN_POINT('',(30.5247014514712,30.0197706669552,-23.0679019220779));
#73708=CARTESIAN_POINT('Origin',(30.5,30.1702883945039,-23.1619558369422));
#73709=CARTESIAN_POINT('',(30.4955273645547,29.8759744160903,-23.562215640718));
#73710=CARTESIAN_POINT('Origin',(30.5,29.8488945896607,-23.5449780585017));
#73711=CARTESIAN_POINT('',(24.1012882089558,29.6594674741542,-23.893572647341));
#73712=CARTESIAN_POINT('Origin',(24.1,29.5917795457861,-23.8513958357493));
#73713=CARTESIAN_POINT('',(23.1004586919557,29.7916028606322,-23.6260497451375));
#73714=CARTESIAN_POINT('Origin',(23.1,29.784615828692,-23.6215825028136));
#73715=CARTESIAN_POINT('',(22.399682944576,30.0370617130518,-23.3121725274111));
#73716=CARTESIAN_POINT('Origin',(22.4,30.0417308725666,-23.315164725566));
#73717=CARTESIAN_POINT('',(21.7998387845652,30.1642348036977,-23.1581731335784));
#73718=CARTESIAN_POINT('Origin',(21.8,30.1702883945039,-23.1619558369422));
#73719=CARTESIAN_POINT('',(13.2021921742626,30.0879729141313,-23.1105194160696));
#73720=CARTESIAN_POINT('Origin',(13.2,30.1702883945039,-23.1619558369422));
#73721=CARTESIAN_POINT('',(12.6002487187375,30.038068082493,-23.3128174522151));
#73722=CARTESIAN_POINT('Origin',(12.6,30.0417308725666,-23.315164725566));
#73723=CARTESIAN_POINT('',(11.8996457869536,29.7900113841146,-23.6250322156174));
#73724=CARTESIAN_POINT('Origin',(11.9,29.784615828692,-23.6215825028136));
#73725=CARTESIAN_POINT('',(10.899790263986,29.6027999600046,-23.8582627313001));
#73726=CARTESIAN_POINT('Origin',(10.9,29.5917795457861,-23.8513958357493));
#73727=CARTESIAN_POINT('',(4.55736144060343,30.1961927037808,-23.7660496304069));
#73728=CARTESIAN_POINT('Origin',(4.5,29.8488945896607,-23.5449780585017));
#73729=CARTESIAN_POINT('',(4.49524972087093,30.1413426776676,-23.1438685456221));
#73730=CARTESIAN_POINT('Origin',(4.5,30.1702883945039,-23.1619558369422));
#73731=CARTESIAN_POINT('',(1.90350512467335,30.1131197861062,-23.1262329256631));
#73732=CARTESIAN_POINT('Origin',(1.9,30.1702883945039,-23.1619558369422));
#73733=CARTESIAN_POINT('Ctrl Pts',(0.138207714141626,33.3938750538235,-26.7099230322464));
#73734=CARTESIAN_POINT('Ctrl Pts',(0.370217470894619,33.3145607080732,-26.4376444612514));
#73735=CARTESIAN_POINT('Ctrl Pts',(0.600000000000007,33.234910440458,-26.1673599741116));
#73736=CARTESIAN_POINT('Origin',(1.9,28.0490892825384,-25.6899024992348));
#73737=CARTESIAN_POINT('',(5.09593997529677,30.9143101784803,-28.872052684018));
#73738=CARTESIAN_POINT('',(17.5,30.9143101784803,-28.872052684018));
#73739=CARTESIAN_POINT('',(4.47529854852883,27.9303271288835,-25.5580037650976));
#73740=CARTESIAN_POINT('Origin',(4.5,28.0490892825384,-25.6899024992348));
#73741=CARTESIAN_POINT('',(5.09944803334083,31.2759009022694,-28.4799582645661));
#73742=CARTESIAN_POINT('Origin',(-0.840551718690874,0.,0.));
#73743=CARTESIAN_POINT('',(4.50447263544529,28.3921611545025,-25.3305554259542));
#73744=CARTESIAN_POINT('Origin',(4.5,28.3704830873816,-25.3068802776753));
#73745=CARTESIAN_POINT('',(10.8302042597752,31.5148708405159,-28.2152957791621));
#73746=CARTESIAN_POINT('Origin',(-62.7155570771054,0.,0.));
#73747=CARTESIAN_POINT('',(10.8987117910442,28.6808880677203,-25.0597981705973));
#73748=CARTESIAN_POINT('Origin',(10.9,28.6275981312562,-25.0004625004277));
#73749=CARTESIAN_POINT('',(11.6618634261911,31.3486557215378,-28.3998553597108));
#73750=CARTESIAN_POINT('Origin',(26.9856656232739,0.,0.));
#73751=CARTESIAN_POINT('',(11.8995413080444,28.4403745085892,-25.2363809880999));
#73752=CARTESIAN_POINT('Origin',(11.9,28.4347618483503,-25.2302758333634));
#73753=CARTESIAN_POINT('',(12.3548486633046,31.0830181478507,-28.6903465092421));
#73754=CARTESIAN_POINT('Origin',(20.8267261185512,0.,0.));
#73755=CARTESIAN_POINT('',(12.600317055424,28.1738892734931,-25.5326149758776));
#73756=CARTESIAN_POINT('Origin',(12.6,28.1776468044757,-25.536693610611));
#73757=CARTESIAN_POINT('',(13.103292255208,30.9143101784803,-28.872052684018));
#73758=CARTESIAN_POINT('Origin',(25.13830739299,0.,0.));
#73759=CARTESIAN_POINT('',(13.2001612154348,28.0443128519265,-25.684597735621));
#73760=CARTESIAN_POINT('Origin',(13.2,28.0490892825384,-25.6899024992348));
#73761=CARTESIAN_POINT('',(21.896707744792,30.9143101784803,-28.872052684018));
#73762=CARTESIAN_POINT('',(17.5,30.9143101784803,-28.872052684018));
#73763=CARTESIAN_POINT('',(21.7978078257374,27.9841403633154,-25.6177694167212));
#73764=CARTESIAN_POINT('Origin',(21.8,28.0490892825384,-25.6899024992348));
#73765=CARTESIAN_POINT('',(22.6451513366954,31.0830181478507,-28.6903465092421));
#73766=CARTESIAN_POINT('Origin',(9.86169260701004,0.,0.));
#73767=CARTESIAN_POINT('',(22.3997512812625,28.1746991546599,-25.5334940662887));
#73768=CARTESIAN_POINT('Origin',(22.4,28.1776468044757,-25.536693610611));
#73769=CARTESIAN_POINT('',(23.3381365738089,31.3486557215378,-28.3998553597108));
#73770=CARTESIAN_POINT('Origin',(14.1732738814488,0.,0.));
#73771=CARTESIAN_POINT('',(23.1003542130464,28.4390960806318,-25.2349903818335));
#73772=CARTESIAN_POINT('Origin',(23.1,28.4347618483503,-25.2302758333634));
#73773=CARTESIAN_POINT('',(24.1697957402248,31.5148708405159,-28.2152957791621));
#73774=CARTESIAN_POINT('Origin',(8.01433437672607,0.,0.));
#73775=CARTESIAN_POINT('',(24.100209736014,28.63627437808,-25.0101230658929));
#73776=CARTESIAN_POINT('Origin',(24.1,28.6275981312562,-25.0004625004277));
#73777=CARTESIAN_POINT('',(29.9005519666592,31.2759009022694,-28.4799582645661));
#73778=CARTESIAN_POINT('Origin',(97.7155570771054,0.,0.));
#73779=CARTESIAN_POINT('',(30.4426385593966,28.6485037699886,-25.610513477472));
#73780=CARTESIAN_POINT('Origin',(30.5,28.3704830873816,-25.3068802776753));
#73781=CARTESIAN_POINT('',(29.9040600247032,30.9143101784803,-28.872052684018));
#73782=CARTESIAN_POINT('Origin',(35.8405517186909,0.,0.));
#73783=CARTESIAN_POINT('',(30.5047502791291,28.0262504068355,-25.6645373580546));
#73784=CARTESIAN_POINT('Origin',(30.5,28.0490892825384,-25.6899024992348));
#73785=CARTESIAN_POINT('',(17.5,30.9143101784803,-28.872052684018));
#73786=CARTESIAN_POINT('Origin',(17.5,32.7483999433363,-27.4791703140996));
#73787=CARTESIAN_POINT('Origin',(17.5,0.,0.));
#73788=CARTESIAN_POINT('',(0.600000000000001,28.1860830985703,-31.5410006112756));
#73789=CARTESIAN_POINT('Origin',(0.600000000000001,0.,0.));
#73790=CARTESIAN_POINT('',(1.67735469196904,28.872052684018,-30.9143101784803));
#73791=CARTESIAN_POINT('Origin',(8.14497546096349,0.,0.));
#73792=CARTESIAN_POINT('',(5.09593997529677,28.872052684018,-30.9143101784803));
#73793=CARTESIAN_POINT('',(17.5,28.872052684018,-30.9143101784803));
#73794=CARTESIAN_POINT('',(5.09944803334083,28.4799582645661,-31.2759009022694));
#73795=CARTESIAN_POINT('Origin',(-0.840551718690872,0.,0.));
#73796=CARTESIAN_POINT('',(10.8302042597752,28.2152957791621,-31.5148708405159));
#73797=CARTESIAN_POINT('Origin',(-62.7155570771055,0.,0.));
#73798=CARTESIAN_POINT('',(11.6618634261911,28.3998553597108,-31.3486557215378));
#73799=CARTESIAN_POINT('Origin',(26.9856656232739,0.,0.));
#73800=CARTESIAN_POINT('',(12.3548486633046,28.6903465092421,-31.0830181478507));
#73801=CARTESIAN_POINT('Origin',(20.8267261185512,0.,0.));
#73802=CARTESIAN_POINT('',(13.103292255208,28.872052684018,-30.9143101784803));
#73803=CARTESIAN_POINT('Origin',(25.13830739299,0.,0.));
#73804=CARTESIAN_POINT('',(21.896707744792,28.872052684018,-30.9143101784803));
#73805=CARTESIAN_POINT('',(17.5,28.872052684018,-30.9143101784803));
#73806=CARTESIAN_POINT('',(22.6451513366954,28.6903465092421,-31.0830181478507));
#73807=CARTESIAN_POINT('Origin',(9.86169260701007,0.,0.));
#73808=CARTESIAN_POINT('',(23.3381365738089,28.3998553597108,-31.3486557215378));
#73809=CARTESIAN_POINT('Origin',(14.1732738814488,0.,0.));
#73810=CARTESIAN_POINT('',(24.1697957402248,28.2152957791621,-31.5148708405159));
#73811=CARTESIAN_POINT('Origin',(8.01433437672609,0.,0.));
#73812=CARTESIAN_POINT('',(29.9005519666592,28.4799582645661,-31.2759009022694));
#73813=CARTESIAN_POINT('Origin',(97.7155570771054,0.,0.));
#73814=CARTESIAN_POINT('',(29.9040600247032,28.872052684018,-30.9143101784803));
#73815=CARTESIAN_POINT('Origin',(35.8405517186909,0.,0.));
#73816=CARTESIAN_POINT('',(17.5,28.872052684018,-30.9143101784803));
#73817=CARTESIAN_POINT('Origin',(33.1,25.6899024992348,-28.0490892825384));
#73818=CARTESIAN_POINT('',(30.5247014514712,25.5580037650976,-27.9303271288835));
#73819=CARTESIAN_POINT('Origin',(30.5,25.6899024992348,-28.0490892825384));
#73820=CARTESIAN_POINT('',(30.4955273645547,25.3305554259542,-28.3921611545025));
#73821=CARTESIAN_POINT('Origin',(30.5,25.3068802776753,-28.3704830873817));
#73822=CARTESIAN_POINT('',(24.1012882089558,25.0597981705973,-28.6808880677203));
#73823=CARTESIAN_POINT('Origin',(24.1,25.0004625004277,-28.6275981312563));
#73824=CARTESIAN_POINT('',(23.1004586919557,25.2363809880999,-28.4403745085892));
#73825=CARTESIAN_POINT('Origin',(23.1,25.2302758333634,-28.4347618483503));
#73826=CARTESIAN_POINT('',(22.399682944576,25.5326149758775,-28.1738892734932));
#73827=CARTESIAN_POINT('Origin',(22.4,25.536693610611,-28.1776468044757));
#73828=CARTESIAN_POINT('',(21.7998387845652,25.684597735621,-28.0443128519265));
#73829=CARTESIAN_POINT('Origin',(21.8,25.6899024992348,-28.0490892825384));
#73830=CARTESIAN_POINT('',(13.2021921742626,25.6177694167211,-27.9841403633154));
#73831=CARTESIAN_POINT('Origin',(13.2,25.6899024992348,-28.0490892825384));
#73832=CARTESIAN_POINT('',(12.6002487187375,25.5334940662887,-28.1746991546599));
#73833=CARTESIAN_POINT('Origin',(12.6,25.536693610611,-28.1776468044757));
#73834=CARTESIAN_POINT('',(11.8996457869536,25.2349903818335,-28.4390960806318));
#73835=CARTESIAN_POINT('Origin',(11.9,25.2302758333634,-28.4347618483503));
#73836=CARTESIAN_POINT('',(10.899790263986,25.0101230658929,-28.63627437808));
#73837=CARTESIAN_POINT('Origin',(10.9,25.0004625004277,-28.6275981312563));
#73838=CARTESIAN_POINT('',(4.55736144060343,25.610513477472,-28.6485037699886));
#73839=CARTESIAN_POINT('Origin',(4.5,25.3068802776753,-28.3704830873817));
#73840=CARTESIAN_POINT('',(4.49524972087093,25.6645373580546,-28.0262504068355));
#73841=CARTESIAN_POINT('Origin',(4.5,25.6899024992348,-28.0490892825384));
#73842=CARTESIAN_POINT('',(1.90350512467335,25.6398056289004,-28.0039818578826));
#73843=CARTESIAN_POINT('Origin',(1.9,25.6899024992348,-28.0490892825384));
#73844=CARTESIAN_POINT('Ctrl Pts',(0.138207714141627,28.2484175959528,-32.1029248328492));
#73845=CARTESIAN_POINT('Ctrl Pts',(0.370217470896185,28.2175888910037,-31.82100999355));
#73846=CARTESIAN_POINT('Ctrl Pts',(0.600000000000008,28.1860830985703,-31.5410006112756));
#73847=CARTESIAN_POINT('Origin',(1.9,23.1619558369422,-30.170288394504));
#73848=CARTESIAN_POINT('',(5.09593997529677,25.4310730087083,-33.8016349549212));
#73849=CARTESIAN_POINT('',(17.5,25.4310730087083,-33.8016349549212));
#73850=CARTESIAN_POINT('',(4.47529854852883,23.0679019220779,-30.0197706669552));
#73851=CARTESIAN_POINT('Origin',(4.5,23.1619558369422,-30.170288394504));
#73852=CARTESIAN_POINT('',(5.09944803334083,25.8552568383243,-33.4782869009794));
#73853=CARTESIAN_POINT('Origin',(-0.840551718690874,0.,0.));
#73854=CARTESIAN_POINT('',(4.50447263544529,23.562215640718,-29.8759744160904));
#73855=CARTESIAN_POINT('Origin',(4.5,23.5449780585017,-29.8488945896607));
#73856=CARTESIAN_POINT('',(10.8302042597752,26.1365544445334,-33.2591419277157));
#73857=CARTESIAN_POINT('Origin',(-62.7155570771056,0.,0.));
#73858=CARTESIAN_POINT('',(10.8987117910442,23.893572647341,-29.6594674741542));
#73859=CARTESIAN_POINT('Origin',(10.9,23.8513958357493,-29.5917795457861));
#73860=CARTESIAN_POINT('',(11.6618634261911,25.9408160718628,-33.4120346810215));
#73861=CARTESIAN_POINT('Origin',(26.9856656232739,0.,0.));
#73862=CARTESIAN_POINT('',(11.8995413080444,23.6260497451375,-29.7916028606322));
#73863=CARTESIAN_POINT('Origin',(11.9,23.6215825028136,-29.784615828692));
#73864=CARTESIAN_POINT('',(12.3548486633046,25.6287708710599,-33.6519851366708));
#73865=CARTESIAN_POINT('Origin',(20.8267261185512,0.,0.));
#73866=CARTESIAN_POINT('',(12.600317055424,23.312172527411,-30.0370617130518));
#73867=CARTESIAN_POINT('Origin',(12.6,23.315164725566,-30.0417308725667));
#73868=CARTESIAN_POINT('',(13.103292255208,25.4310730087083,-33.8016349549212));
#73869=CARTESIAN_POINT('Origin',(25.13830739299,0.,0.));
#73870=CARTESIAN_POINT('',(13.2001612154348,23.1581731335784,-30.1642348036977));
#73871=CARTESIAN_POINT('Origin',(13.2,23.1619558369422,-30.170288394504));
#73872=CARTESIAN_POINT('',(21.896707744792,25.4310730087083,-33.8016349549212));
#73873=CARTESIAN_POINT('',(17.5,25.4310730087083,-33.8016349549212));
#73874=CARTESIAN_POINT('',(21.7978078257374,23.1105194160696,-30.0879729141313));
#73875=CARTESIAN_POINT('Origin',(21.8,23.1619558369422,-30.170288394504));
#73876=CARTESIAN_POINT('',(22.6451513366954,25.6287708710599,-33.6519851366708));
#73877=CARTESIAN_POINT('Origin',(9.86169260701005,0.,0.));
#73878=CARTESIAN_POINT('',(22.3997512812625,23.3128174522151,-30.0380680824931));
#73879=CARTESIAN_POINT('Origin',(22.4,23.315164725566,-30.0417308725667));
#73880=CARTESIAN_POINT('',(23.3381365738089,25.9408160718628,-33.4120346810215));
#73881=CARTESIAN_POINT('Origin',(14.1732738814488,0.,0.));
#73882=CARTESIAN_POINT('',(23.1003542130464,23.6250322156174,-29.7900113841146));
#73883=CARTESIAN_POINT('Origin',(23.1,23.6215825028136,-29.784615828692));
#73884=CARTESIAN_POINT('',(24.1697957402248,26.1365544445334,-33.2591419277157));
#73885=CARTESIAN_POINT('Origin',(8.01433437672607,0.,0.));
#73886=CARTESIAN_POINT('',(24.100209736014,23.8582627313001,-29.6027999600046));
#73887=CARTESIAN_POINT('Origin',(24.1,23.8513958357493,-29.5917795457861));
#73888=CARTESIAN_POINT('',(29.9005519666592,25.8552568383243,-33.4782869009794));
#73889=CARTESIAN_POINT('Origin',(97.7155570771055,0.,0.));
#73890=CARTESIAN_POINT('',(30.4426385593966,23.7660496304069,-30.1961927037808));
#73891=CARTESIAN_POINT('Origin',(30.5,23.5449780585017,-29.8488945896607));
#73892=CARTESIAN_POINT('',(29.9040600247032,25.4310730087083,-33.8016349549212));
#73893=CARTESIAN_POINT('Origin',(35.8405517186909,0.,0.));
#73894=CARTESIAN_POINT('',(30.5047502791291,23.1438685456221,-30.1413426776677));
#73895=CARTESIAN_POINT('Origin',(30.5,23.1619558369422,-30.170288394504));
#73896=CARTESIAN_POINT('',(17.5,25.4310730087083,-33.8016349549212));
#73897=CARTESIAN_POINT('Origin',(17.5,27.4791703140995,-32.7483999433363));
#73898=CARTESIAN_POINT('Origin',(17.5,0.,0.));
#73899=CARTESIAN_POINT('',(0.600000000000001,22.2808358845789,-35.9562839053824));
#73900=CARTESIAN_POINT('Origin',(0.600000000000001,0.,0.));
#73901=CARTESIAN_POINT('',(1.67735469196904,23.0652077022745,-35.4582316768749));
#73902=CARTESIAN_POINT('Origin',(8.14497546096349,0.,0.));
#73903=CARTESIAN_POINT('',(5.09593997529677,23.0652077022745,-35.4582316768749));
#73904=CARTESIAN_POINT('',(17.5,23.0652077022745,-35.4582316768749));
#73905=CARTESIAN_POINT('',(5.09944803334083,22.6162805078382,-35.7462425436685));
#73906=CARTESIAN_POINT('Origin',(-0.840551718690872,0.,0.));
#73907=CARTESIAN_POINT('',(10.8302042597752,22.3141421459872,-35.9356238333033));
#73908=CARTESIAN_POINT('Origin',(-62.7155570771055,0.,0.));
#73909=CARTESIAN_POINT('',(11.6618634261911,22.5247608043155,-35.8039823302991));
#73910=CARTESIAN_POINT('Origin',(26.9856656232739,0.,0.));
#73911=CARTESIAN_POINT('',(12.3548486633046,22.856966221146,-35.5928236469852));
#73912=CARTESIAN_POINT('Origin',(20.8267261185512,0.,0.));
#73913=CARTESIAN_POINT('',(13.103292255208,23.0652077022745,-35.4582316768749));
#73914=CARTESIAN_POINT('Origin',(25.13830739299,0.,0.));
#73915=CARTESIAN_POINT('',(21.896707744792,23.0652077022745,-35.4582316768749));
#73916=CARTESIAN_POINT('',(17.5,23.0652077022745,-35.4582316768749));
#73917=CARTESIAN_POINT('',(22.6451513366954,22.856966221146,-35.5928236469852));
#73918=CARTESIAN_POINT('Origin',(9.86169260701005,0.,0.));
#73919=CARTESIAN_POINT('',(23.3381365738089,22.5247608043155,-35.8039823302992));
#73920=CARTESIAN_POINT('Origin',(14.1732738814488,0.,0.));
#73921=CARTESIAN_POINT('',(24.1697957402248,22.3141421459872,-35.9356238333033));
#73922=CARTESIAN_POINT('Origin',(8.01433437672609,0.,0.));
#73923=CARTESIAN_POINT('',(29.9005519666592,22.6162805078382,-35.7462425436685));
#73924=CARTESIAN_POINT('Origin',(97.7155570771054,0.,0.));
#73925=CARTESIAN_POINT('',(29.9040600247032,23.0652077022745,-35.4582316768749));
#73926=CARTESIAN_POINT('Origin',(35.8405517186909,0.,0.));
#73927=CARTESIAN_POINT('',(17.5,23.0652077022745,-35.4582316768749));
#73928=CARTESIAN_POINT('Origin',(33.1,20.4289419162443,-32.0839653438087));
#73929=CARTESIAN_POINT('',(30.5247014514712,20.3196698518115,-31.9441034793054));
#73930=CARTESIAN_POINT('Origin',(30.5,20.4289419162443,-32.0839653438087));
#73931=CARTESIAN_POINT('',(30.4955273645547,20.01548032708,-32.3594252187343));
#73932=CARTESIAN_POINT('Origin',(30.5,19.9959292143521,-32.3339653438087));
#73933=CARTESIAN_POINT('',(24.1012882089558,19.6986995804965,-32.5967492173916));
#73934=CARTESIAN_POINT('Origin',(24.1,19.6495190528383,-32.5339653438087));
#73935=CARTESIAN_POINT('',(23.1004586919557,19.9143644494692,-32.3905528841213));
#73936=CARTESIAN_POINT('Origin',(23.1,19.9093266739737,-32.3839653438087));
#73937=CARTESIAN_POINT('',(22.399682944576,20.2523726527879,-32.1795566506761));
#73938=CARTESIAN_POINT('Origin',(22.4,20.2557368354874,-32.1839653438087));
#73939=CARTESIAN_POINT('',(21.7998387845652,20.4245471623811,-32.0783403153759));
#73940=CARTESIAN_POINT('Origin',(21.8,20.4289419162443,-32.0839653438087));
#73941=CARTESIAN_POINT('',(13.2021921742626,20.3691829588007,-32.0074773662801));
#73942=CARTESIAN_POINT('Origin',(13.2,20.4289419162443,-32.0839653438087));
#73943=CARTESIAN_POINT('',(12.6002487187375,20.2530977534517,-32.180506880376));
#73944=CARTESIAN_POINT('Origin',(12.6,20.2557368354874,-32.1839653438087));
#73945=CARTESIAN_POINT('',(11.8996457869536,19.9132169663217,-32.3890524021132));
#73946=CARTESIAN_POINT('Origin',(11.9,19.9093266739737,-32.3839653438087));
#73947=CARTESIAN_POINT('',(10.899790263986,19.657526238157,-32.544187318536));
#73948=CARTESIAN_POINT('Origin',(10.9,19.6495190528383,-32.5339653438087));
#73949=CARTESIAN_POINT('',(4.55736144060343,20.2466717586954,-32.6604876193617));
#73950=CARTESIAN_POINT('Origin',(4.5,19.9959292143521,-32.3339653438087));
#73951=CARTESIAN_POINT('',(4.49524972087093,20.4079280576996,-32.0570688314042));
#73952=CARTESIAN_POINT('Origin',(4.5,20.4289419162443,-32.0839653438087));
#73953=CARTESIAN_POINT('',(1.90350512467335,20.3874389520281,-32.0308439720488));
#73954=CARTESIAN_POINT('Origin',(1.9,20.4289419162443,-32.0839653438087));
#73955=CARTESIAN_POINT('Ctrl Pts',(0.138207714141627,22.2446462638181,-36.5204955072696));
#73956=CARTESIAN_POINT('Ctrl Pts',(0.370217470898034,22.2632399142706,-36.2375102394021));
#73957=CARTESIAN_POINT('Ctrl Pts',(0.600000000000007,22.2808358845789,-35.9562839053824));
#73958=CARTESIAN_POINT('Origin',(1.9,17.5710580837557,-33.7339653438087));
#73959=CARTESIAN_POINT('',(5.09593997529677,19.1751255543105,-37.7041716521717));
#73960=CARTESIAN_POINT('',(17.5,19.1751255543105,-37.7041716521717));
#73961=CARTESIAN_POINT('',(4.47529854852883,17.5045701882916,-33.5694020278343));
#73962=CARTESIAN_POINT('Origin',(4.5,17.5710580837557,-33.7339653438087));
#73963=CARTESIAN_POINT('',(5.09944803334083,19.6490138787379,-37.459394730737));
#73964=CARTESIAN_POINT('Origin',(-0.840551718690874,0.,0.));
#73965=CARTESIAN_POINT('',(4.50447263544529,18.0163441277467,-33.5136270415661));
#73966=CARTESIAN_POINT('Origin',(4.5,18.0040707856479,-33.4839653438087));
#73967=CARTESIAN_POINT('',(10.8302042597752,19.9640920674886,-37.2924258787336));
#73968=CARTESIAN_POINT('Origin',(-62.7155570771054,0.,0.));
#73969=CARTESIAN_POINT('',(10.8987117910442,18.3802631128034,-33.3579488669236));
#73970=CARTESIAN_POINT('Origin',(10.9,18.3504809471617,-33.2839653438087));
#73971=CARTESIAN_POINT('',(11.6618634261911,19.7447778525305,-37.4090062358548));
#73972=CARTESIAN_POINT('Origin',(26.9856656232739,0.,0.));
#73973=CARTESIAN_POINT('',(11.8995413080444,18.0938594155378,-33.4416219555226));
#73974=CARTESIAN_POINT('Origin',(11.9,18.0906733260263,-33.4339653438087));
#73975=CARTESIAN_POINT('',(12.3548486633046,19.3958063601357,-37.5911252244478));
#73976=CARTESIAN_POINT('Origin',(20.8267261185512,0.,0.));
#73977=CARTESIAN_POINT('',(12.600317055424,17.742127215612,-33.6288475295615));
#73978=CARTESIAN_POINT('Origin',(12.6,17.7442631645126,-33.6339653438087));
#73979=CARTESIAN_POINT('',(13.103292255208,19.1751255543105,-37.7041716521717));
#73980=CARTESIAN_POINT('Origin',(25.13830739299,0.,0.));
#73981=CARTESIAN_POINT('',(13.2001612154348,17.5683840431675,-33.7273468611033));
#73982=CARTESIAN_POINT('Origin',(13.2,17.5710580837557,-33.7339653438087));
#73983=CARTESIAN_POINT('',(21.896707744792,19.1751255543105,-37.7041716521717));
#73984=CARTESIAN_POINT('',(17.5,19.1751255543105,-37.7041716521717));
#73985=CARTESIAN_POINT('',(21.7978078257374,17.5346970308537,-33.6439685797945));
#73986=CARTESIAN_POINT('Origin',(21.8,17.5710580837557,-33.7339653438087));
#73987=CARTESIAN_POINT('',(22.6451513366954,19.3958063601357,-37.5911252244478));
#73988=CARTESIAN_POINT('Origin',(9.86169260701005,0.,0.));
#73989=CARTESIAN_POINT('',(22.3997512812625,17.7425875883397,-33.6299506000067));
#73990=CARTESIAN_POINT('Origin',(22.4,17.7442631645126,-33.6339653438087));
#73991=CARTESIAN_POINT('',(23.3381365738089,19.7447778525305,-37.4090062358548));
#73992=CARTESIAN_POINT('Origin',(14.1732738814488,0.,0.));
#73993=CARTESIAN_POINT('',(23.1003542130464,18.0931337015746,-33.4398779649625));
#73994=CARTESIAN_POINT('Origin',(23.1,18.0906733260263,-33.4339653438087));
#73995=CARTESIAN_POINT('',(24.1697957402248,19.9640920674886,-37.2924258787336));
#73996=CARTESIAN_POINT('Origin',(8.01433437672608,0.,0.));
#73997=CARTESIAN_POINT('',(24.100209736014,18.3553298442931,-33.2960107570711));
#73998=CARTESIAN_POINT('Origin',(24.1,18.3504809471617,-33.2839653438087));
#73999=CARTESIAN_POINT('',(29.9005519666592,19.6490138787379,-37.459394730737));
#74000=CARTESIAN_POINT('Origin',(97.7155570771054,0.,0.));
#74001=CARTESIAN_POINT('',(30.4426385593966,18.1614760990067,-33.864375894796));
#74002=CARTESIAN_POINT('Origin',(30.5,18.0040707856479,-33.4839653438087));
#74003=CARTESIAN_POINT('',(29.9040600247032,19.1751255543105,-37.7041716521717));
#74004=CARTESIAN_POINT('Origin',(35.8405517186909,0.,0.));
#74005=CARTESIAN_POINT('',(30.5047502791291,17.5582719500126,-33.7023185522751));
#74006=CARTESIAN_POINT('Origin',(30.5,17.5710580837557,-33.7339653438087));
#74007=CARTESIAN_POINT('',(17.5,19.1751255543105,-37.7041716521717));
#74008=CARTESIAN_POINT('Origin',(17.5,21.375,-37.0225860117847));
#74009=CARTESIAN_POINT('Origin',(17.5,0.,0.));
#74010=CARTESIAN_POINT('',(0.600000000000001,15.6985967468814,-39.2790537077817));
#74011=CARTESIAN_POINT('Origin',(0.600000000000001,0.,0.));
#74012=CARTESIAN_POINT('',(1.67735469196904,16.5575380560557,-38.9247727484987));
#74013=CARTESIAN_POINT('Origin',(8.14497546096349,0.,0.));
#74014=CARTESIAN_POINT('',(5.09593997529677,16.5575380560557,-38.9247727484987));
#74015=CARTESIAN_POINT('',(17.5,16.5575380560557,-38.9247727484987));
#74016=CARTESIAN_POINT('',(5.09944803334083,16.0654185122698,-39.1304526938498));
#74017=CARTESIAN_POINT('Origin',(-0.840551718690872,0.,0.));
#74018=CARTESIAN_POINT('',(10.8302042597752,15.7349845952072,-39.2644910802189));
#74019=CARTESIAN_POINT('Origin',(-62.7155570771055,0.,0.));
#74020=CARTESIAN_POINT('',(11.6618634261911,15.9652627899599,-39.1714230536436));
#74021=CARTESIAN_POINT('Origin',(26.9856656232739,0.,0.));
#74022=CARTESIAN_POINT('',(12.3548486633046,16.3290885806033,-39.0211592104439));
#74023=CARTESIAN_POINT('Origin',(20.8267261185512,0.,0.));
#74024=CARTESIAN_POINT('',(13.103292255208,16.5575380560557,-38.9247727484987));
#74025=CARTESIAN_POINT('Origin',(25.13830739299,0.,0.));
#74026=CARTESIAN_POINT('',(21.896707744792,16.5575380560557,-38.9247727484987));
#74027=CARTESIAN_POINT('',(17.5,16.5575380560557,-38.9247727484987));
#74028=CARTESIAN_POINT('',(22.6451513366954,16.3290885806033,-39.0211592104439));
#74029=CARTESIAN_POINT('Origin',(9.86169260701006,0.,0.));
#74030=CARTESIAN_POINT('',(23.3381365738089,15.9652627899599,-39.1714230536436));
#74031=CARTESIAN_POINT('Origin',(14.1732738814488,0.,0.));
#74032=CARTESIAN_POINT('',(24.1697957402248,15.7349845952072,-39.2644910802189));
#74033=CARTESIAN_POINT('Origin',(8.01433437672609,0.,0.));
#74034=CARTESIAN_POINT('',(29.9005519666592,16.0654185122698,-39.1304526938498));
#74035=CARTESIAN_POINT('Origin',(97.7155570771054,0.,0.));
#74036=CARTESIAN_POINT('',(29.9040600247032,16.5575380560557,-38.9247727484987));
#74037=CARTESIAN_POINT('Origin',(35.8405517186909,0.,0.));
#74038=CARTESIAN_POINT('',(17.5,16.5575380560557,-38.9247727484987));
#74039=CARTESIAN_POINT('Origin',(33.1,14.5472582706721,-35.1439863533772));
#74040=CARTESIAN_POINT('',(30.5247014514712,14.4639330523271,-34.987274410005));
#74041=CARTESIAN_POINT('Origin',(30.5,14.5472582706721,-35.1439863533772));
#74042=CARTESIAN_POINT('',(30.4955273645547,14.0922449867892,-35.343464522354));
#74043=CARTESIAN_POINT('Origin',(30.5,14.0774119602792,-35.31499642504));
#74044=CARTESIAN_POINT('',(24.1012882089558,13.7390659716653,-35.5221746368434));
#74045=CARTESIAN_POINT('Origin',(24.1,13.7015349119648,-35.4518044823703));
#74046=CARTESIAN_POINT('',(23.1004586919557,13.9872600241959,-35.35656070068));
#74047=CARTESIAN_POINT('Origin',(23.1,13.9834426982006,-35.3491984393726));
#74048=CARTESIAN_POINT('',(22.399682944576,14.3567722348382,-35.2074644826695));
#74049=CARTESIAN_POINT('Origin',(22.4,14.359319746515,-35.2123903820423));
#74050=CARTESIAN_POINT('',(21.7998387845652,14.5439070589317,-35.137683640766));
#74051=CARTESIAN_POINT('Origin',(21.8,14.5472582706721,-35.1439863533772));
#74052=CARTESIAN_POINT('',(13.2021921742626,14.501689183981,-35.0582833660355));
#74053=CARTESIAN_POINT('Origin',(13.2,14.5472582706721,-35.1439863533772));
#74054=CARTESIAN_POINT('',(12.6002487187375,14.3573213139379,-35.208526188654));
#74055=CARTESIAN_POINT('Origin',(12.6,14.359319746515,-35.2123903820423));
#74056=CARTESIAN_POINT('',(11.8996457869536,13.9863905298622,-35.3548837560077));
#74057=CARTESIAN_POINT('Origin',(11.9,13.9834426982006,-35.3491984393726));
#74058=CARTESIAN_POINT('',(10.899790263986,13.7076454228628,-35.4632615954717));
#74059=CARTESIAN_POINT('Origin',(10.9,13.7015349119648,-35.4518044823703));
#74060=CARTESIAN_POINT('',(4.55736144060343,14.267645163841,-35.6800990794246));
#74061=CARTESIAN_POINT('Origin',(4.5,14.0774119602792,-35.31499642504));
#74062=CARTESIAN_POINT('',(4.49524972087093,14.5312341902212,-35.1138494411902));
#74063=CARTESIAN_POINT('Origin',(4.5,14.5472582706721,-35.1439863533772));
#74064=CARTESIAN_POINT('',(1.90350512467335,14.5156102591402,-35.0844651005135));
#74065=CARTESIAN_POINT('Origin',(1.9,14.5472582706721,-35.1439863533772));
#74066=CARTESIAN_POINT('Ctrl Pts',(0.138207714141622,15.5649826112913,-39.8284094059642));
#74067=CARTESIAN_POINT('Ctrl Pts',(0.370217470896767,15.6324336584852,-39.5529520736987));
#74068=CARTESIAN_POINT('Ctrl Pts',(0.600000000000007,15.6985967468815,-39.2790537077817));
#74069=CARTESIAN_POINT('Origin',(1.9,11.4462726220786,-36.2726528263519));
#74070=CARTESIAN_POINT('',(5.09593997529677,12.3365516130267,-40.4610861730024));
#74071=CARTESIAN_POINT('',(17.5,12.3365516130267,-40.4610861730024));
#74072=CARTESIAN_POINT('',(4.47529854852883,11.409370947074,-36.0990440950346));
#74073=CARTESIAN_POINT('Origin',(4.5,11.4462726220786,-36.2726528263519));
#74074=CARTESIAN_POINT('',(5.09944803334083,12.8457455753269,-40.3023178069695));
#74075=CARTESIAN_POINT('Origin',(-0.840551718690874,0.,0.));
#74076=CARTESIAN_POINT('',(4.50447263544529,11.9230551151638,-36.1329850680974));
#74077=CARTESIAN_POINT('Origin',(4.5,11.9161189324716,-36.101642754689));
#74078=CARTESIAN_POINT('',(10.8302042597752,13.1850308552911,-40.1925983403042));
#74079=CARTESIAN_POINT('Origin',(-62.7155570771054,0.,0.));
#74080=CARTESIAN_POINT('',(10.8987117910442,12.3084785844451,-36.0428658633082));
#74081=CARTESIAN_POINT('Origin',(10.9,12.291995980786,-35.9648346973588));
#74082=CARTESIAN_POINT('',(11.6618634261911,12.9488045494887,-40.2693240660821));
#74083=CARTESIAN_POINT('Origin',(26.9856656232739,0.,0.));
#74084=CARTESIAN_POINT('',(11.8995413080444,12.0118963235316,-36.0755342895718));
#74085=CARTESIAN_POINT('Origin',(11.9,12.0100881945502,-36.0674407403565));
#74086=CARTESIAN_POINT('',(12.3548486633046,12.5735100877104,-40.3880779943072));
#74087=CARTESIAN_POINT('Origin',(20.8267261185512,0.,0.));
#74088=CARTESIAN_POINT('',(12.600317055424,11.6329963463162,-36.1988378309035));
#74089=CARTESIAN_POINT('Origin',(12.6,11.6342111462358,-36.2042487976867));
#74090=CARTESIAN_POINT('',(13.103292255208,12.3365516130267,-40.4610861730024));
#74091=CARTESIAN_POINT('Origin',(25.13830739299,0.,0.));
#74092=CARTESIAN_POINT('',(13.2001612154348,11.4447884936362,-36.2656705509953));
#74093=CARTESIAN_POINT('Origin',(13.2,11.4462726220786,-36.2726528263519));
#74094=CARTESIAN_POINT('',(21.896707744792,12.3365516130267,-40.4610861730024));
#74095=CARTESIAN_POINT('',(17.5,12.3365516130267,-40.4610861730024));
#74096=CARTESIAN_POINT('',(21.7978078257374,11.42609174934,-36.1777092848303));
#74097=CARTESIAN_POINT('Origin',(21.8,11.4462726220786,-36.2726528263519));
#74098=CARTESIAN_POINT('',(22.6451513366954,12.5735100877104,-40.3880779943072));
#74099=CARTESIAN_POINT('Origin',(9.86169260701006,0.,0.));
#74100=CARTESIAN_POINT('',(22.3997512812625,11.633258178775,-36.2000040861152));
#74101=CARTESIAN_POINT('Origin',(22.4,11.6342111462358,-36.2042487976867));
#74102=CARTESIAN_POINT('',(23.3381365738089,12.9488045494887,-40.2693240660821));
#74103=CARTESIAN_POINT('Origin',(14.1732738814488,0.,0.));
#74104=CARTESIAN_POINT('',(23.1003542130464,12.0114844755768,-36.0736907752397));
#74105=CARTESIAN_POINT('Origin',(23.1,12.0100881945502,-36.0674407403565));
#74106=CARTESIAN_POINT('',(24.1697957402248,13.1850308552911,-40.1925983403042));
#74107=CARTESIAN_POINT('Origin',(8.01433437672607,0.,0.));
#74108=CARTESIAN_POINT('',(24.100209736014,12.2946795482123,-35.9775391158784));
#74109=CARTESIAN_POINT('Origin',(24.1,12.291995980786,-35.9648346973588));
#74110=CARTESIAN_POINT('',(29.9005519666592,12.8457455753269,-40.3023178069695));
#74111=CARTESIAN_POINT('Origin',(97.7155570771054,0.,0.));
#74112=CARTESIAN_POINT('',(30.4426385593966,12.0050753064884,-36.5036071604488));
#74113=CARTESIAN_POINT('Origin',(30.5,11.9161189324716,-36.101642754689));
#74114=CARTESIAN_POINT('',(29.9040600247032,12.3365516130267,-40.4610861730024));
#74115=CARTESIAN_POINT('Origin',(35.8405517186909,0.,0.));
#74116=CARTESIAN_POINT('',(30.5047502791291,11.4391761461162,-36.2392665318678));
#74117=CARTESIAN_POINT('Origin',(30.5,11.4462726220786,-36.2726528263519));
#74118=CARTESIAN_POINT('',(17.5,12.3365516130267,-40.4610861730024));
#74119=CARTESIAN_POINT('Origin',(17.5,14.6213611271723,-40.1718595385976));
#74120=CARTESIAN_POINT('Origin',(17.5,0.,0.));
#74121=CARTESIAN_POINT('',(0.600000000000001,8.63936369090331,-41.4083493394303));
#74122=CARTESIAN_POINT('Origin',(0.600000000000001,0.,0.));
#74123=CARTESIAN_POINT('',(1.67735469196904,9.54677599452212,-41.2086042970448));
#74124=CARTESIAN_POINT('Origin',(8.14497546096349,0.,0.));
#74125=CARTESIAN_POINT('',(5.09593997529677,9.54677599452211,-41.2086042970448));
#74126=CARTESIAN_POINT('',(17.5,9.54677599452211,-41.2086042970448));
#74127=CARTESIAN_POINT('',(5.09944803334083,9.02641690470009,-41.325703839893));
#74128=CARTESIAN_POINT('Origin',(-0.840551718690872,0.,0.));
#74129=CARTESIAN_POINT('',(10.8302042597752,8.67772749978828,-41.4003266344532));
#74130=CARTESIAN_POINT('Origin',(-62.7155570771055,0.,0.));
#74131=CARTESIAN_POINT('',(11.6618634261911,8.92066834454425,-41.3486599091996));
#74132=CARTESIAN_POINT('Origin',(26.9856656232739,0.,0.));
#74133=CARTESIAN_POINT('',(12.3548486633046,9.3050598464565,-41.2638565969525));
#74134=CARTESIAN_POINT('Origin',(20.8267261185512,0.,0.));
#74135=CARTESIAN_POINT('',(13.103292255208,9.54677599452212,-41.2086042970448));
#74136=CARTESIAN_POINT('Origin',(25.13830739299,0.,0.));
#74137=CARTESIAN_POINT('',(21.896707744792,9.54677599452211,-41.2086042970448));
#74138=CARTESIAN_POINT('',(17.5,9.54677599452211,-41.2086042970448));
#74139=CARTESIAN_POINT('',(22.6451513366954,9.3050598464565,-41.2638565969525));
#74140=CARTESIAN_POINT('Origin',(9.86169260701005,0.,0.));
#74141=CARTESIAN_POINT('',(23.3381365738089,8.92066834454425,-41.3486599091996));
#74142=CARTESIAN_POINT('Origin',(14.1732738814488,0.,0.));
#74143=CARTESIAN_POINT('',(24.1697957402248,8.67772749978828,-41.4003266344532));
#74144=CARTESIAN_POINT('Origin',(8.01433437672608,0.,0.));
#74145=CARTESIAN_POINT('',(29.9005519666592,9.02641690470009,-41.325703839893));
#74146=CARTESIAN_POINT('Origin',(97.7155570771054,0.,0.));
#74147=CARTESIAN_POINT('',(29.9040600247032,9.54677599452211,-41.2086042970448));
#74148=CARTESIAN_POINT('Origin',(35.8405517186909,0.,0.));
#74149=CARTESIAN_POINT('',(17.5,9.54677599452211,-41.2086042970448));
#74150=CARTESIAN_POINT('Origin',(33.1,8.22356354381348,-37.1361751213135));
#74151=CARTESIAN_POINT('',(30.5247014514712,8.16871696615112,-36.9673747121716));
#74152=CARTESIAN_POINT('Origin',(30.5,8.22356354381348,-37.1361751213135));
#74153=CARTESIAN_POINT('',(30.4955273645547,7.74082391359483,-37.253610541118));
#74154=CARTESIAN_POINT('Origin',(30.5,7.73115966730738,-37.2229992101469));
#74155=CARTESIAN_POINT('',(24.1012882089558,7.36197779558789,-37.3682767550424));
#74156=CARTESIAN_POINT('Origin',(24.1,7.33723656610249,-37.2924584812137));
#74157=CARTESIAN_POINT('',(23.1004586919557,7.63515978098255,-37.2482773116316));
#74158=CARTESIAN_POINT('Origin',(23.1,7.63267889200616,-37.2403640279136));
#74159=CARTESIAN_POINT('',(22.399682944576,8.02494855741035,-37.1656113221937));
#74160=CARTESIAN_POINT('Origin',(22.4,8.02660199321104,-37.1709047568469));
#74161=CARTESIAN_POINT('',(21.7998387845652,8.22135769906883,-37.1293862292573));
#74162=CARTESIAN_POINT('Origin',(21.8,8.22356354381348,-37.1361751213135));
#74163=CARTESIAN_POINT('',(13.2021921742626,8.19356892151486,-37.0438611660612));
#74164=CARTESIAN_POINT('Origin',(13.2,8.22356354381348,-37.1361751213135));
#74165=CARTESIAN_POINT('',(12.6002487187375,8.02530493145532,-37.1667522450638));
#74166=CARTESIAN_POINT('Origin',(12.6,8.02660199321104,-37.1709047568469));
#74167=CARTESIAN_POINT('',(11.8996457869536,7.63459469460788,-37.2464748574103));
#74168=CARTESIAN_POINT('Origin',(11.9,7.63267889200616,-37.2403640279136));
#74169=CARTESIAN_POINT('',(10.899790263986,7.34126473779835,-37.3048026141052));
#74170=CARTESIAN_POINT('Origin',(10.9,7.33723656610249,-37.2924584812137));
#74171=CARTESIAN_POINT('',(4.55736144060343,7.85510339046015,-37.6155887839604));
#74172=CARTESIAN_POINT('Origin',(4.5,7.73115966730738,-37.2229992101469));
#74173=CARTESIAN_POINT('',(4.49524972087093,8.21301612503226,-37.1037135041708));
#74174=CARTESIAN_POINT('Origin',(4.5,8.22356354381348,-37.1361751213135));
#74175=CARTESIAN_POINT('',(1.90350512467335,8.20273209378166,-37.0720625104951));
#74176=CARTESIAN_POINT('Origin',(1.9,8.22356354381348,-37.1361751213135));
#74177=CARTESIAN_POINT('Ctrl Pts',(0.138207714141623,8.41238483838183,-41.9261572390061));
#74178=CARTESIAN_POINT('Ctrl Pts',(0.370217470900092,8.52664381638163,-41.6665974739903));
#74179=CARTESIAN_POINT('Ctrl Pts',(0.600000000000007,8.63936369090331,-41.4083493394303));
#74180=CARTESIAN_POINT('Origin',(1.9,4.9736979588732,-37.7092141076143));
#74181=CARTESIAN_POINT('',(5.09593997529677,5.1231377935775,-41.9886110647639));
#74182=CARTESIAN_POINT('',(17.5,5.1231377935775,-41.9886110647639));
#74183=CARTESIAN_POINT('',(4.47529854852883,4.96750374304975,-37.5318349744051));
#74184=CARTESIAN_POINT('Origin',(4.5,4.9736979588732,-37.7092141076143));
#74185=CARTESIAN_POINT('',(5.09944803334083,5.65216579287044,-41.9206753505941));
#74186=CARTESIAN_POINT('Origin',(-0.840551718690874,0.,0.));
#74187=CARTESIAN_POINT('',(4.50447263544529,5.46749010626365,-37.6544606275072));
#74188=CARTESIAN_POINT('Origin',(4.5,5.4661018353793,-37.6223900187809));
#74189=CARTESIAN_POINT('',(10.8302042597752,6.00534915250317,-41.8715390397407));
#74190=CARTESIAN_POINT('Origin',(-62.7155570771055,0.,0.));
#74191=CARTESIAN_POINT('',(10.8987117910442,5.86270716268917,-37.6326386190063));
#74192=CARTESIAN_POINT('Origin',(10.9,5.86002493658418,-37.5529307477141));
#74193=CARTESIAN_POINT('',(11.6618634261911,5.75938837262205,-41.9060788618227));
#74194=CARTESIAN_POINT('Origin',(26.9856656232739,0.,0.));
#74195=CARTESIAN_POINT('',(11.8995413080444,5.5649578400478,-37.6133097693334));
#74196=CARTESIAN_POINT('Origin',(11.9,5.56458261068052,-37.6050252010142));
#74197=CARTESIAN_POINT('',(12.3548486633046,5.36917407377308,-41.9578594516632));
#74198=CARTESIAN_POINT('Origin',(20.8267261185512,0.,0.));
#74199=CARTESIAN_POINT('',(12.600317055424,5.17040276961774,-37.6689447622493));
#74200=CARTESIAN_POINT('Origin',(12.6,5.17065950947564,-37.674484472081));
#74201=CARTESIAN_POINT('',(13.103292255208,5.1231377935775,-41.9886110647639));
#74202=CARTESIAN_POINT('Origin',(25.13830739299,0.,0.));
#74203=CARTESIAN_POINT('',(13.2001612154348,4.97344883706827,-37.7020801925101));
#74204=CARTESIAN_POINT('Origin',(13.2,4.9736979588732,-37.7092141076143));
#74205=CARTESIAN_POINT('',(21.896707744792,5.1231377935775,-41.9886110647639));
#74206=CARTESIAN_POINT('',(17.5,5.1231377935775,-41.9886110647639));
#74207=CARTESIAN_POINT('',(21.7978078257374,4.97031045190413,-37.6122086000506));
#74208=CARTESIAN_POINT('Origin',(21.8,4.9736979588732,-37.7092141076143));
#74209=CARTESIAN_POINT('',(22.6451513366954,5.36917407377308,-41.9578594516632));
#74210=CARTESIAN_POINT('Origin',(9.86169260701005,0.,0.));
#74211=CARTESIAN_POINT('',(22.3997512812625,5.17045810616097,-37.6701387661531));
#74212=CARTESIAN_POINT('Origin',(22.4,5.17065950947564,-37.674484472081));
#74213=CARTESIAN_POINT('',(23.3381365738089,5.75938837262205,-41.9060788618227));
#74214=CARTESIAN_POINT('Origin',(14.1732738814488,0.,0.));
#74215=CARTESIAN_POINT('',(23.1003542130464,5.5648723718931,-37.6114227454796));
#74216=CARTESIAN_POINT('Origin',(23.1,5.56458261068052,-37.6050252010142));
#74217=CARTESIAN_POINT('',(24.1697957402248,6.00534915250317,-41.8715390397407));
#74218=CARTESIAN_POINT('Origin',(8.01433437672608,0.,0.));
#74219=CARTESIAN_POINT('',(24.100209736014,5.86046163546709,-37.565908154163));
#74220=CARTESIAN_POINT('Origin',(24.1,5.86002493658418,-37.5529307477141));
#74221=CARTESIAN_POINT('',(29.9005519666592,5.65216579287044,-41.9206753505941));
#74222=CARTESIAN_POINT('Origin',(97.7155570771054,0.,0.));
#74223=CARTESIAN_POINT('',(30.4426385593966,5.48390637564376,-38.0336947942479));
#74224=CARTESIAN_POINT('Origin',(30.5,5.4661018353793,-37.6223900187809));
#74225=CARTESIAN_POINT('',(29.9040600247032,5.1231377935775,-41.9886110647639));
#74226=CARTESIAN_POINT('Origin',(35.8405517186909,0.,0.));
#74227=CARTESIAN_POINT('',(30.5047502791291,4.97250676352253,-37.6751027358433));
#74228=CARTESIAN_POINT('Origin',(30.5,4.9736979588732,-37.7092141076143));
#74229=CARTESIAN_POINT('',(17.5,5.1231377935775,-41.9886110647639));
#74230=CARTESIAN_POINT('Origin',(17.5,7.42345959526125,-42.1005314412719));
#74231=CARTESIAN_POINT('Origin',(17.5,0.,0.));
#74232=CARTESIAN_POINT('',(0.600000000000001,1.31762794090603,-42.2794732300362));
#74233=CARTESIAN_POINT('Origin',(0.600000000000001,0.,0.));
#74234=CARTESIAN_POINT('',(1.67735469196904,2.24593997529676,-42.240333256585));
#74235=CARTESIAN_POINT('Origin',(8.14497546096349,0.,0.));
#74236=CARTESIAN_POINT('',(5.09593997529677,2.24593997529676,-42.240333256585));
#74237=CARTESIAN_POINT('',(17.5,2.24593997529676,-42.240333256585));
#74238=CARTESIAN_POINT('',(5.09944803334083,1.71315218706844,-42.2652943865761));
#74239=CARTESIAN_POINT('Origin',(-0.840551718690872,0.,0.));
#74240=CARTESIAN_POINT('',(10.8302042597752,1.35680204543027,-42.2782342134758));
#74241=CARTESIAN_POINT('Origin',(-62.7155570771055,0.,0.));
#74242=CARTESIAN_POINT('',(11.6618634261911,1.6050239055556,-42.269538656846));
#74243=CARTESIAN_POINT('Origin',(26.9856656232739,0.,0.));
#74244=CARTESIAN_POINT('',(12.3548486633046,1.99830157746261,-42.2527725812817));
#74245=CARTESIAN_POINT('Origin',(20.8267261185512,0.,0.));
#74246=CARTESIAN_POINT('',(13.103292255208,2.24593997529676,-42.240333256585));
#74247=CARTESIAN_POINT('Origin',(25.13830739299,0.,0.));
#74248=CARTESIAN_POINT('',(21.896707744792,2.24593997529676,-42.240333256585));
#74249=CARTESIAN_POINT('',(17.5,2.24593997529676,-42.240333256585));
#74250=CARTESIAN_POINT('',(22.6451513366954,1.99830157746261,-42.2527725812817));
#74251=CARTESIAN_POINT('Origin',(9.86169260701006,0.,0.));
#74252=CARTESIAN_POINT('',(23.3381365738089,1.6050239055556,-42.269538656846));
#74253=CARTESIAN_POINT('Origin',(14.1732738814488,0.,0.));
#74254=CARTESIAN_POINT('',(24.1697957402248,1.35680204543027,-42.2782342134758));
#74255=CARTESIAN_POINT('Origin',(8.01433437672608,0.,0.));
#74256=CARTESIAN_POINT('',(29.9005519666592,1.71315218706844,-42.2652943865761));
#74257=CARTESIAN_POINT('Origin',(97.7155570771054,0.,0.));
#74258=CARTESIAN_POINT('',(29.9040600247032,2.24593997529676,-42.240333256585));
#74259=CARTESIAN_POINT('Origin',(35.8405517186909,0.,0.));
#74260=CARTESIAN_POINT('',(17.5,2.24593997529676,-42.240333256585));
#74261=CARTESIAN_POINT('Origin',(33.1,1.64999999999999,-38.));
#74262=CARTESIAN_POINT('',(30.5247014514712,1.62529854852883,-37.8242400401031));
#74263=CARTESIAN_POINT('Origin',(30.5,1.64999999999999,-38.));
#74264=CARTESIAN_POINT('',(30.4955273645547,1.15420182283181,-38.0318244548267));
#74265=CARTESIAN_POINT('Origin',(30.5,1.14999999999999,-38.));
#74266=CARTESIAN_POINT('',(24.1012882089558,0.761199649532065,-38.0789626932999));
#74267=CARTESIAN_POINT('Origin',(24.1,0.749999999999993,-38.));
#74268=CARTESIAN_POINT('',(23.1004586919557,1.05106907140132,-38.0082238650069));
#74269=CARTESIAN_POINT('Origin',(23.1,1.04999999999999,-38.));
#74270=CARTESIAN_POINT('',(22.399682944576,1.44929087888548,-37.9944998683999));
#74271=CARTESIAN_POINT('Origin',(22.4,1.44999999999999,-38.));
#74272=CARTESIAN_POINT('',(21.7998387845652,1.64900654572745,-37.9929312055486));
#74273=CARTESIAN_POINT('Origin',(21.8,1.64999999999999,-38.));
#74274=CARTESIAN_POINT('',(13.2021921742626,1.63649121351442,-37.9038799896544));
#74275=CARTESIAN_POINT('Origin',(13.2,1.64999999999999,-38.));
#74276=CARTESIAN_POINT('',(12.6002487187375,1.4494437196307,-37.9956853417913));
#74277=CARTESIAN_POINT('Origin',(12.6,1.44999999999999,-38.));
#74278=CARTESIAN_POINT('',(11.8996457869536,1.05082556284928,-38.0063506678963));
#74279=CARTESIAN_POINT('Origin',(11.9,1.04999999999999,-38.));
#74280=CARTESIAN_POINT('',(10.899790263986,0.751823438535061,-38.01285608245));
#74281=CARTESIAN_POINT('Origin',(10.9,0.749999999999993,-38.));
#74282=CARTESIAN_POINT('',(4.55736144060343,1.20388827543429,-38.408147857702));
#74283=CARTESIAN_POINT('Origin',(4.5,1.14999999999999,-38.));
#74284=CARTESIAN_POINT('',(4.49524972087093,1.64524972087092,-37.9662000077121));
#74285=CARTESIAN_POINT('Origin',(4.5,1.64999999999999,-38.));
#74286=CARTESIAN_POINT('',(1.90350512467335,1.64061806453626,-37.933244060464));
#74287=CARTESIAN_POINT('Origin',(1.9,1.64999999999999,-38.));
#74288=CARTESIAN_POINT('Ctrl Pts',(0.138207714141622,1.0041810090302,-42.75));
#74289=CARTESIAN_POINT('Ctrl Pts',(0.370217470898645,1.16177621660533,-42.5142243943556));
#74290=CARTESIAN_POINT('Ctrl Pts',(0.600000000000007,1.31762794090604,-42.2794732300361));
#74291=CARTESIAN_POINT('Origin',(1.9,-1.65000000000001,-38.));
#74292=CARTESIAN_POINT('',(5.09593997529677,-2.24593997529678,-42.240333256585));
#74293=CARTESIAN_POINT('',(17.5,-2.24593997529678,-42.240333256585));
#74294=CARTESIAN_POINT('',(4.47529854852883,-1.62529854852884,-37.8242400401031));
#74295=CARTESIAN_POINT('Origin',(4.5,-1.65000000000001,-38.));
#74296=CARTESIAN_POINT('',(5.09944803334083,-1.71315218706845,-42.2652943865761));
#74297=CARTESIAN_POINT('Origin',(-0.840551718690874,0.,0.));
#74298=CARTESIAN_POINT('',(4.50447263544529,-1.15420182283182,-38.0318244548267));
#74299=CARTESIAN_POINT('Origin',(4.5,-1.15000000000001,-38.));
#74300=CARTESIAN_POINT('',(10.8302042597752,-1.35680204543028,-42.2782342134758));
#74301=CARTESIAN_POINT('Origin',(-62.7155570771055,0.,0.));
#74302=CARTESIAN_POINT('',(10.8987117910442,-0.761199649532079,-38.0789626932999));
#74303=CARTESIAN_POINT('Origin',(10.9,-0.750000000000007,-38.));
#74304=CARTESIAN_POINT('',(11.6618634261911,-1.60502390555562,-42.269538656846));
#74305=CARTESIAN_POINT('Origin',(26.9856656232739,0.,0.));
#74306=CARTESIAN_POINT('',(11.8995413080444,-1.05106907140134,-38.0082238650069));
#74307=CARTESIAN_POINT('Origin',(11.9,-1.05000000000001,-38.));
#74308=CARTESIAN_POINT('',(12.3548486633046,-1.99830157746262,-42.2527725812817));
#74309=CARTESIAN_POINT('Origin',(20.8267261185512,0.,0.));
#74310=CARTESIAN_POINT('',(12.600317055424,-1.4492908788855,-37.9944998683999));
#74311=CARTESIAN_POINT('Origin',(12.6,-1.45000000000001,-38.));
#74312=CARTESIAN_POINT('',(13.103292255208,-2.24593997529678,-42.240333256585));
#74313=CARTESIAN_POINT('Origin',(25.13830739299,0.,0.));
#74314=CARTESIAN_POINT('',(13.2001612154348,-1.64900654572746,-37.9929312055486));
#74315=CARTESIAN_POINT('Origin',(13.2,-1.65000000000001,-38.));
#74316=CARTESIAN_POINT('',(21.896707744792,-2.24593997529678,-42.240333256585));
#74317=CARTESIAN_POINT('',(17.5,-2.24593997529678,-42.240333256585));
#74318=CARTESIAN_POINT('',(21.7978078257374,-1.63649121351443,-37.9038799896544));
#74319=CARTESIAN_POINT('Origin',(21.8,-1.65000000000001,-38.));
#74320=CARTESIAN_POINT('',(22.6451513366954,-1.99830157746262,-42.2527725812817));
#74321=CARTESIAN_POINT('Origin',(9.86169260701005,0.,0.));
#74322=CARTESIAN_POINT('',(22.3997512812625,-1.44944371963072,-37.9956853417913));
#74323=CARTESIAN_POINT('Origin',(22.4,-1.45000000000001,-38.));
#74324=CARTESIAN_POINT('',(23.3381365738089,-1.60502390555562,-42.269538656846));
#74325=CARTESIAN_POINT('Origin',(14.1732738814488,0.,0.));
#74326=CARTESIAN_POINT('',(23.1003542130464,-1.05082556284929,-38.0063506678963));
#74327=CARTESIAN_POINT('Origin',(23.1,-1.05000000000001,-38.));
#74328=CARTESIAN_POINT('',(24.1697957402248,-1.35680204543028,-42.2782342134758));
#74329=CARTESIAN_POINT('Origin',(8.01433437672608,0.,0.));
#74330=CARTESIAN_POINT('',(24.100209736014,-0.751823438535075,-38.01285608245));
#74331=CARTESIAN_POINT('Origin',(24.1,-0.750000000000007,-38.));
#74332=CARTESIAN_POINT('',(29.9005519666592,-1.71315218706845,-42.2652943865761));
#74333=CARTESIAN_POINT('Origin',(97.7155570771054,0.,0.));
#74334=CARTESIAN_POINT('',(30.4426385593966,-1.20388827543431,-38.408147857702));
#74335=CARTESIAN_POINT('Origin',(30.5,-1.15000000000001,-38.));
#74336=CARTESIAN_POINT('',(29.9040600247032,-2.24593997529678,-42.240333256585));
#74337=CARTESIAN_POINT('Origin',(35.8405517186909,0.,0.));
#74338=CARTESIAN_POINT('',(30.5047502791291,-1.64524972087094,-37.9662000077121));
#74339=CARTESIAN_POINT('Origin',(30.5,-1.65000000000001,-38.));
#74340=CARTESIAN_POINT('',(17.5,-2.24593997529678,-42.240333256585));
#74341=CARTESIAN_POINT('Origin',(17.5,-7.8530475995324E-15,-42.75));
#74342=CARTESIAN_POINT('Origin',(17.5,0.,0.));
#74343=CARTESIAN_POINT('',(0.600000000000001,-6.04414326732376,-41.8659567209931));
#74344=CARTESIAN_POINT('Origin',(0.600000000000001,0.,0.));
#74345=CARTESIAN_POINT('',(1.67735469196905,-5.12313779357752,-41.9886110647639));
#74346=CARTESIAN_POINT('Origin',(8.14497546096349,0.,0.));
#74347=CARTESIAN_POINT('',(5.09593997529677,-5.12313779357752,-41.9886110647639));
#74348=CARTESIAN_POINT('',(17.5,-5.12313779357752,-41.9886110647639));
#74349=CARTESIAN_POINT('',(5.09944803334083,-5.65216579287046,-41.9206753505941));
#74350=CARTESIAN_POINT('Origin',(-0.840551718690872,0.,0.));
#74351=CARTESIAN_POINT('',(10.8302042597752,-6.00534915250318,-41.8715390397407));
#74352=CARTESIAN_POINT('Origin',(-62.7155570771055,0.,0.));
#74353=CARTESIAN_POINT('',(11.6618634261911,-5.75938837262207,-41.9060788618227));
#74354=CARTESIAN_POINT('Origin',(26.9856656232739,0.,0.));
#74355=CARTESIAN_POINT('',(12.3548486633046,-5.3691740737731,-41.9578594516632));
#74356=CARTESIAN_POINT('Origin',(20.8267261185512,0.,0.));
#74357=CARTESIAN_POINT('',(13.103292255208,-5.12313779357752,-41.9886110647639));
#74358=CARTESIAN_POINT('Origin',(25.13830739299,0.,0.));
#74359=CARTESIAN_POINT('',(21.896707744792,-5.12313779357752,-41.9886110647639));
#74360=CARTESIAN_POINT('',(17.5,-5.12313779357752,-41.9886110647639));
#74361=CARTESIAN_POINT('',(22.6451513366954,-5.3691740737731,-41.9578594516632));
#74362=CARTESIAN_POINT('Origin',(9.86169260701005,0.,0.));
#74363=CARTESIAN_POINT('',(23.3381365738089,-5.75938837262207,-41.9060788618227));
#74364=CARTESIAN_POINT('Origin',(14.1732738814488,0.,0.));
#74365=CARTESIAN_POINT('',(24.1697957402248,-6.00534915250318,-41.8715390397407));
#74366=CARTESIAN_POINT('Origin',(8.01433437672608,0.,0.));
#74367=CARTESIAN_POINT('',(29.9005519666592,-5.65216579287046,-41.9206753505941));
#74368=CARTESIAN_POINT('Origin',(97.7155570771054,0.,0.));
#74369=CARTESIAN_POINT('',(29.9040600247032,-5.12313779357752,-41.9886110647639));
#74370=CARTESIAN_POINT('Origin',(35.8405517186909,0.,0.));
#74371=CARTESIAN_POINT('',(17.5,-5.12313779357752,-41.9886110647639));
#74372=CARTESIAN_POINT('Origin',(33.1,-4.97369795887321,-37.7092141076143));
#74373=CARTESIAN_POINT('',(30.5247014514712,-4.96750374304976,-37.5318349744051));
#74374=CARTESIAN_POINT('Origin',(30.5,-4.97369795887321,-37.7092141076143));
#74375=CARTESIAN_POINT('',(30.4955273645547,-5.46749010626366,-37.6544606275072));
#74376=CARTESIAN_POINT('Origin',(30.5,-5.46610183537931,-37.6223900187809));
#74377=CARTESIAN_POINT('',(24.1012882089558,-5.86270716268919,-37.6326386190063));
#74378=CARTESIAN_POINT('Origin',(24.1,-5.8600249365842,-37.5529307477141));
#74379=CARTESIAN_POINT('',(23.1004586919557,-5.56495784004782,-37.6133097693334));
#74380=CARTESIAN_POINT('Origin',(23.1,-5.56458261068053,-37.6050252010142));
#74381=CARTESIAN_POINT('',(22.399682944576,-5.17040276961776,-37.6689447622493));
#74382=CARTESIAN_POINT('Origin',(22.4,-5.17065950947565,-37.674484472081));
#74383=CARTESIAN_POINT('',(21.7998387845652,-4.97344883706828,-37.7020801925101));
#74384=CARTESIAN_POINT('Origin',(21.8,-4.97369795887321,-37.7092141076143));
#74385=CARTESIAN_POINT('',(13.2021921742626,-4.97031045190415,-37.6122086000507));
#74386=CARTESIAN_POINT('Origin',(13.2,-4.97369795887321,-37.7092141076143));
#74387=CARTESIAN_POINT('',(12.6002487187375,-5.17045810616098,-37.6701387661531));
#74388=CARTESIAN_POINT('Origin',(12.6,-5.17065950947565,-37.674484472081));
#74389=CARTESIAN_POINT('',(11.8996457869536,-5.56487237189311,-37.6114227454796));
#74390=CARTESIAN_POINT('Origin',(11.9,-5.56458261068053,-37.6050252010142));
#74391=CARTESIAN_POINT('',(10.899790263986,-5.8604616354671,-37.565908154163));
#74392=CARTESIAN_POINT('Origin',(10.9,-5.8600249365842,-37.5529307477141));
#74393=CARTESIAN_POINT('',(4.55736144060343,-5.48390637564377,-38.0336947942479));
#74394=CARTESIAN_POINT('Origin',(4.5,-5.46610183537931,-37.6223900187809));
#74395=CARTESIAN_POINT('',(4.49524972087093,-4.97250676352255,-37.6751027358433));
#74396=CARTESIAN_POINT('Origin',(4.5,-4.97369795887321,-37.7092141076143));
#74397=CARTESIAN_POINT('',(1.90350512467335,-4.97134531440728,-37.6418431848034));
#74398=CARTESIAN_POINT('Origin',(1.9,-4.97369795887321,-37.7092141076143));
#74399=CARTESIAN_POINT('Ctrl Pts',(0.138207714141622,-6.4345343521407,-42.2749056435377));
#74400=CARTESIAN_POINT('Ctrl Pts',(0.370217470893856,-6.23839136562873,
-42.0700781197367));
#74401=CARTESIAN_POINT('Ctrl Pts',(0.600000000000006,-6.04414326732376,
-41.8659567209931));
#74402=CARTESIAN_POINT('Origin',(1.9,-8.2235635438135,-37.1361751213135));
#74403=CARTESIAN_POINT('',(5.09593997529677,-9.54677599452213,-41.2086042970448));
#74404=CARTESIAN_POINT('',(17.5,-9.54677599452213,-41.2086042970448));
#74405=CARTESIAN_POINT('',(4.47529854852883,-8.16871696615113,-36.9673747121716));
#74406=CARTESIAN_POINT('Origin',(4.5,-8.2235635438135,-37.1361751213135));
#74407=CARTESIAN_POINT('',(5.09944803334083,-9.02641690470011,-41.325703839893));
#74408=CARTESIAN_POINT('Origin',(-0.840551718690874,0.,0.));
#74409=CARTESIAN_POINT('',(4.50447263544529,-7.74082391359484,-37.253610541118));
#74410=CARTESIAN_POINT('Origin',(4.5,-7.73115966730739,-37.2229992101469));
#74411=CARTESIAN_POINT('',(10.8302042597752,-8.6777274997883,-41.4003266344532));
#74412=CARTESIAN_POINT('Origin',(-62.7155570771055,0.,0.));
#74413=CARTESIAN_POINT('',(10.8987117910442,-7.36197779558791,-37.3682767550424));
#74414=CARTESIAN_POINT('Origin',(10.9,-7.33723656610251,-37.2924584812137));
#74415=CARTESIAN_POINT('',(11.6618634261911,-8.92066834454427,-41.3486599091995));
#74416=CARTESIAN_POINT('Origin',(26.9856656232739,0.,0.));
#74417=CARTESIAN_POINT('',(11.8995413080444,-7.63515978098256,-37.2482773116316));
#74418=CARTESIAN_POINT('Origin',(11.9,-7.63267889200617,-37.2403640279136));
#74419=CARTESIAN_POINT('',(12.3548486633046,-9.30505984645652,-41.2638565969525));
#74420=CARTESIAN_POINT('Origin',(20.8267261185512,0.,0.));
#74421=CARTESIAN_POINT('',(12.600317055424,-8.02494855741037,-37.1656113221937));
#74422=CARTESIAN_POINT('Origin',(12.6,-8.02660199321105,-37.1709047568469));
#74423=CARTESIAN_POINT('',(13.103292255208,-9.54677599452213,-41.2086042970448));
#74424=CARTESIAN_POINT('Origin',(25.13830739299,0.,0.));
#74425=CARTESIAN_POINT('',(13.2001612154348,-8.22135769906884,-37.1293862292573));
#74426=CARTESIAN_POINT('Origin',(13.2,-8.2235635438135,-37.1361751213135));
#74427=CARTESIAN_POINT('',(21.896707744792,-9.54677599452213,-41.2086042970448));
#74428=CARTESIAN_POINT('',(17.5,-9.54677599452213,-41.2086042970448));
#74429=CARTESIAN_POINT('',(21.7978078257374,-8.19356892151487,-37.0438611660612));
#74430=CARTESIAN_POINT('Origin',(21.8,-8.2235635438135,-37.1361751213135));
#74431=CARTESIAN_POINT('',(22.6451513366954,-9.30505984645652,-41.2638565969525));
#74432=CARTESIAN_POINT('Origin',(9.86169260701004,0.,0.));
#74433=CARTESIAN_POINT('',(22.3997512812625,-8.02530493145534,-37.1667522450638));
#74434=CARTESIAN_POINT('Origin',(22.4,-8.02660199321105,-37.1709047568469));
#74435=CARTESIAN_POINT('',(23.3381365738089,-8.92066834454426,-41.3486599091995));
#74436=CARTESIAN_POINT('Origin',(14.1732738814488,0.,0.));
#74437=CARTESIAN_POINT('',(23.1003542130464,-7.6345946946079,-37.2464748574103));
#74438=CARTESIAN_POINT('Origin',(23.1,-7.63267889200617,-37.2403640279136));
#74439=CARTESIAN_POINT('',(24.1697957402248,-8.6777274997883,-41.4003266344532));
#74440=CARTESIAN_POINT('Origin',(8.01433437672608,0.,0.));
#74441=CARTESIAN_POINT('',(24.100209736014,-7.34126473779837,-37.3048026141052));
#74442=CARTESIAN_POINT('Origin',(24.1,-7.33723656610251,-37.2924584812137));
#74443=CARTESIAN_POINT('',(29.9005519666592,-9.02641690470011,-41.325703839893));
#74444=CARTESIAN_POINT('Origin',(97.7155570771055,0.,0.));
#74445=CARTESIAN_POINT('',(30.4426385593966,-7.85510339046017,-37.6155887839604));
#74446=CARTESIAN_POINT('Origin',(30.5,-7.73115966730739,-37.2229992101469));
#74447=CARTESIAN_POINT('',(29.9040600247032,-9.54677599452213,-41.2086042970448));
#74448=CARTESIAN_POINT('Origin',(35.8405517186909,0.,0.));
#74449=CARTESIAN_POINT('',(30.5047502791291,-8.21301612503227,-37.1037135041708));
#74450=CARTESIAN_POINT('Origin',(30.5,-8.2235635438135,-37.1361751213135));
#74451=CARTESIAN_POINT('',(17.5,-9.54677599452213,-41.2086042970448));
#74452=CARTESIAN_POINT('Origin',(17.5,-7.42345959526127,-42.1005314412719));
#74453=CARTESIAN_POINT('Origin',(17.5,0.,0.));
#74454=CARTESIAN_POINT('',(0.600000000000001,-13.22226624086,-40.1803643021789));
#74455=CARTESIAN_POINT('Origin',(0.600000000000001,0.,0.));
#74456=CARTESIAN_POINT('',(1.67735469196905,-12.3365516130268,-40.4610861730024));
#74457=CARTESIAN_POINT('Origin',(8.14497546096349,0.,0.));
#74458=CARTESIAN_POINT('',(5.09593997529677,-12.3365516130268,-40.4610861730024));
#74459=CARTESIAN_POINT('',(17.5,-12.3365516130268,-40.4610861730024));
#74460=CARTESIAN_POINT('',(5.09944803334083,-12.8457455753269,-40.3023178069695));
#74461=CARTESIAN_POINT('Origin',(-0.840551718690874,0.,0.));
#74462=CARTESIAN_POINT('',(10.8302042597752,-13.1850308552912,-40.1925983403041));
#74463=CARTESIAN_POINT('Origin',(-62.7155570771055,0.,0.));
#74464=CARTESIAN_POINT('',(11.6618634261911,-12.9488045494888,-40.2693240660821));
#74465=CARTESIAN_POINT('Origin',(26.9856656232739,0.,0.));
#74466=CARTESIAN_POINT('',(12.3548486633046,-12.5735100877104,-40.3880779943072));
#74467=CARTESIAN_POINT('Origin',(20.8267261185512,0.,0.));
#74468=CARTESIAN_POINT('',(13.103292255208,-12.3365516130268,-40.4610861730024));
#74469=CARTESIAN_POINT('Origin',(25.13830739299,0.,0.));
#74470=CARTESIAN_POINT('',(21.896707744792,-12.3365516130268,-40.4610861730024));
#74471=CARTESIAN_POINT('',(17.5,-12.3365516130268,-40.4610861730024));
#74472=CARTESIAN_POINT('',(22.6451513366954,-12.5735100877104,-40.3880779943072));
#74473=CARTESIAN_POINT('Origin',(9.86169260701005,0.,0.));
#74474=CARTESIAN_POINT('',(23.3381365738089,-12.9488045494888,-40.2693240660821));
#74475=CARTESIAN_POINT('Origin',(14.1732738814488,0.,0.));
#74476=CARTESIAN_POINT('',(24.1697957402248,-13.1850308552912,-40.1925983403042));
#74477=CARTESIAN_POINT('Origin',(8.01433437672608,0.,0.));
#74478=CARTESIAN_POINT('',(29.9005519666592,-12.8457455753269,-40.3023178069695));
#74479=CARTESIAN_POINT('Origin',(97.7155570771054,0.,0.));
#74480=CARTESIAN_POINT('',(29.9040600247032,-12.3365516130268,-40.4610861730024));
#74481=CARTESIAN_POINT('Origin',(35.8405517186909,0.,0.));
#74482=CARTESIAN_POINT('',(17.5,-12.3365516130268,-40.4610861730024));
#74483=CARTESIAN_POINT('Origin',(33.1,-11.4462726220787,-36.2726528263519));
#74484=CARTESIAN_POINT('',(30.5247014514712,-11.409370947074,-36.0990440950346));
#74485=CARTESIAN_POINT('Origin',(30.5,-11.4462726220787,-36.2726528263519));
#74486=CARTESIAN_POINT('',(30.4955273645547,-11.9230551151638,-36.1329850680974));
#74487=CARTESIAN_POINT('Origin',(30.5,-11.9161189324716,-36.101642754689));
#74488=CARTESIAN_POINT('',(24.1012882089558,-12.3084785844451,-36.0428658633082));
#74489=CARTESIAN_POINT('Origin',(24.1,-12.291995980786,-35.9648346973588));
#74490=CARTESIAN_POINT('',(23.1004586919557,-12.0118963235317,-36.0755342895717));
#74491=CARTESIAN_POINT('Origin',(23.1,-12.0100881945502,-36.0674407403565));
#74492=CARTESIAN_POINT('',(22.399682944576,-11.6329963463162,-36.1988378309035));
#74493=CARTESIAN_POINT('Origin',(22.4,-11.6342111462359,-36.2042487976867));
#74494=CARTESIAN_POINT('',(21.7998387845652,-11.4447884936363,-36.2656705509953));
#74495=CARTESIAN_POINT('Origin',(21.8,-11.4462726220787,-36.2726528263519));
#74496=CARTESIAN_POINT('',(13.2021921742626,-11.4260917493401,-36.1777092848303));
#74497=CARTESIAN_POINT('Origin',(13.2,-11.4462726220787,-36.2726528263519));
#74498=CARTESIAN_POINT('',(12.6002487187375,-11.633258178775,-36.2000040861152));
#74499=CARTESIAN_POINT('Origin',(12.6,-11.6342111462359,-36.2042487976867));
#74500=CARTESIAN_POINT('',(11.8996457869536,-12.0114844755769,-36.0736907752397));
#74501=CARTESIAN_POINT('Origin',(11.9,-12.0100881945502,-36.0674407403565));
#74502=CARTESIAN_POINT('',(10.899790263986,-12.2946795482123,-35.9775391158784));
#74503=CARTESIAN_POINT('Origin',(10.9,-12.291995980786,-35.9648346973588));
#74504=CARTESIAN_POINT('',(4.55736144060343,-12.0050753064885,-36.5036071604488));
#74505=CARTESIAN_POINT('Origin',(4.5,-11.9161189324716,-36.101642754689));
#74506=CARTESIAN_POINT('',(4.49524972087093,-11.4391761461162,-36.2392665318678));
#74507=CARTESIAN_POINT('Origin',(4.5,-11.4462726220787,-36.2726528263519));
#74508=CARTESIAN_POINT('',(1.90350512467335,-11.4322568815947,-36.2067139516643));
#74509=CARTESIAN_POINT('Origin',(1.9,-11.4462726220787,-36.2726528263519));
#74510=CARTESIAN_POINT('Ctrl Pts',(0.138207714141628,-13.6777396430533,
-40.515309671231));
#74511=CARTESIAN_POINT('Ctrl Pts',(0.370217470898111,-13.4490085829891,
-40.3476538099283));
#74512=CARTESIAN_POINT('Ctrl Pts',(0.600000000000007,-13.22226624086,-40.1803643021789));
#74513=CARTESIAN_POINT('Origin',(1.9,-14.5472582706722,-35.1439863533772));
#74514=CARTESIAN_POINT('',(5.09593997529677,-16.5575380560557,-38.9247727484987));
#74515=CARTESIAN_POINT('',(17.5,-16.5575380560557,-38.9247727484987));
#74516=CARTESIAN_POINT('',(4.47529854852883,-14.4639330523272,-34.987274410005));
#74517=CARTESIAN_POINT('Origin',(4.5,-14.5472582706722,-35.1439863533772));
#74518=CARTESIAN_POINT('',(5.09944803334084,-16.0654185122698,-39.1304526938498));
#74519=CARTESIAN_POINT('Origin',(-0.840551718690874,0.,0.));
#74520=CARTESIAN_POINT('',(4.50447263544529,-14.0922449867892,-35.343464522354));
#74521=CARTESIAN_POINT('Origin',(4.5,-14.0774119602792,-35.31499642504));
#74522=CARTESIAN_POINT('',(10.8302042597752,-15.7349845952073,-39.2644910802189));
#74523=CARTESIAN_POINT('Origin',(-62.7155570771055,0.,0.));
#74524=CARTESIAN_POINT('',(10.8987117910442,-13.7390659716653,-35.5221746368434));
#74525=CARTESIAN_POINT('Origin',(10.9,-13.7015349119649,-35.4518044823703));
#74526=CARTESIAN_POINT('',(11.6618634261911,-15.96526278996,-39.1714230536436));
#74527=CARTESIAN_POINT('Origin',(26.9856656232739,0.,0.));
#74528=CARTESIAN_POINT('',(11.8995413080444,-13.9872600241959,-35.35656070068));
#74529=CARTESIAN_POINT('Origin',(11.9,-13.9834426982006,-35.3491984393726));
#74530=CARTESIAN_POINT('',(12.3548486633046,-16.3290885806033,-39.0211592104439));
#74531=CARTESIAN_POINT('Origin',(20.8267261185512,0.,0.));
#74532=CARTESIAN_POINT('',(12.600317055424,-14.3567722348383,-35.2074644826695));
#74533=CARTESIAN_POINT('Origin',(12.6,-14.359319746515,-35.2123903820423));
#74534=CARTESIAN_POINT('',(13.103292255208,-16.5575380560557,-38.9247727484987));
#74535=CARTESIAN_POINT('Origin',(25.13830739299,0.,0.));
#74536=CARTESIAN_POINT('',(13.2001612154348,-14.5439070589318,-35.137683640766));
#74537=CARTESIAN_POINT('Origin',(13.2,-14.5472582706722,-35.1439863533772));
#74538=CARTESIAN_POINT('',(21.896707744792,-16.5575380560557,-38.9247727484987));
#74539=CARTESIAN_POINT('',(17.5,-16.5575380560557,-38.9247727484987));
#74540=CARTESIAN_POINT('',(21.7978078257374,-14.501689183981,-35.0582833660355));
#74541=CARTESIAN_POINT('Origin',(21.8,-14.5472582706722,-35.1439863533772));
#74542=CARTESIAN_POINT('',(22.6451513366954,-16.3290885806033,-39.0211592104439));
#74543=CARTESIAN_POINT('Origin',(9.86169260701004,0.,0.));
#74544=CARTESIAN_POINT('',(22.3997512812625,-14.357321313938,-35.208526188654));
#74545=CARTESIAN_POINT('Origin',(22.4,-14.359319746515,-35.2123903820423));
#74546=CARTESIAN_POINT('',(23.3381365738089,-15.96526278996,-39.1714230536436));
#74547=CARTESIAN_POINT('Origin',(14.1732738814488,0.,0.));
#74548=CARTESIAN_POINT('',(23.1003542130464,-13.9863905298622,-35.3548837560077));
#74549=CARTESIAN_POINT('Origin',(23.1,-13.9834426982006,-35.3491984393726));
#74550=CARTESIAN_POINT('',(24.1697957402248,-15.7349845952073,-39.2644910802189));
#74551=CARTESIAN_POINT('Origin',(8.01433437672606,0.,0.));
#74552=CARTESIAN_POINT('',(24.100209736014,-13.7076454228629,-35.4632615954717));
#74553=CARTESIAN_POINT('Origin',(24.1,-13.7015349119649,-35.4518044823703));
#74554=CARTESIAN_POINT('',(29.9005519666592,-16.0654185122698,-39.1304526938498));
#74555=CARTESIAN_POINT('Origin',(97.7155570771054,0.,0.));
#74556=CARTESIAN_POINT('',(30.4426385593966,-14.267645163841,-35.6800990794245));
#74557=CARTESIAN_POINT('Origin',(30.5,-14.0774119602792,-35.31499642504));
#74558=CARTESIAN_POINT('',(29.9040600247032,-16.5575380560557,-38.9247727484987));
#74559=CARTESIAN_POINT('Origin',(35.8405517186909,0.,0.));
#74560=CARTESIAN_POINT('',(30.5047502791291,-14.5312341902212,-35.1138494411902));
#74561=CARTESIAN_POINT('Origin',(30.5,-14.5472582706722,-35.1439863533772));
#74562=CARTESIAN_POINT('',(17.5,-16.5575380560557,-38.9247727484987));
#74563=CARTESIAN_POINT('Origin',(17.5,-14.6213611271724,-40.1718595385976));
#74564=CARTESIAN_POINT('Origin',(17.5,0.,0.));
#74565=CARTESIAN_POINT('',(0.600000000000001,-19.9986373454573,-37.2739118462884));
#74566=CARTESIAN_POINT('Origin',(0.600000000000001,0.,0.));
#74567=CARTESIAN_POINT('',(1.67735469196905,-19.1751255543105,-37.7041716521717));
#74568=CARTESIAN_POINT('Origin',(8.14497546096349,0.,0.));
#74569=CARTESIAN_POINT('',(5.09593997529677,-19.1751255543105,-37.7041716521717));
#74570=CARTESIAN_POINT('',(17.5,-19.1751255543105,-37.7041716521717));
#74571=CARTESIAN_POINT('',(5.09944803334083,-19.6490138787379,-37.459394730737));
#74572=CARTESIAN_POINT('Origin',(-0.840551718690872,0.,0.));
#74573=CARTESIAN_POINT('',(10.8302042597752,-19.9640920674886,-37.2924258787336));
#74574=CARTESIAN_POINT('Origin',(-62.7155570771055,0.,0.));
#74575=CARTESIAN_POINT('',(11.6618634261911,-19.7447778525305,-37.4090062358548));
#74576=CARTESIAN_POINT('Origin',(26.9856656232739,0.,0.));
#74577=CARTESIAN_POINT('',(12.3548486633046,-19.3958063601357,-37.5911252244478));
#74578=CARTESIAN_POINT('Origin',(20.8267261185512,0.,0.));
#74579=CARTESIAN_POINT('',(13.103292255208,-19.1751255543105,-37.7041716521717));
#74580=CARTESIAN_POINT('Origin',(25.13830739299,0.,0.));
#74581=CARTESIAN_POINT('',(21.896707744792,-19.1751255543105,-37.7041716521717));
#74582=CARTESIAN_POINT('',(17.5,-19.1751255543105,-37.7041716521717));
#74583=CARTESIAN_POINT('',(22.6451513366954,-19.3958063601357,-37.5911252244478));
#74584=CARTESIAN_POINT('Origin',(9.86169260701006,0.,0.));
#74585=CARTESIAN_POINT('',(23.3381365738089,-19.7447778525305,-37.4090062358548));
#74586=CARTESIAN_POINT('Origin',(14.1732738814488,0.,0.));
#74587=CARTESIAN_POINT('',(24.1697957402248,-19.9640920674886,-37.2924258787336));
#74588=CARTESIAN_POINT('Origin',(8.01433437672609,0.,0.));
#74589=CARTESIAN_POINT('',(29.9005519666592,-19.6490138787379,-37.459394730737));
#74590=CARTESIAN_POINT('Origin',(97.7155570771054,0.,0.));
#74591=CARTESIAN_POINT('',(29.9040600247032,-19.1751255543105,-37.7041716521717));
#74592=CARTESIAN_POINT('Origin',(35.8405517186909,0.,0.));
#74593=CARTESIAN_POINT('',(17.5,-19.1751255543105,-37.7041716521717));
#74594=CARTESIAN_POINT('Origin',(33.1,-17.5710580837557,-33.7339653438087));
#74595=CARTESIAN_POINT('',(30.5247014514712,-17.5045701882916,-33.5694020278342));
#74596=CARTESIAN_POINT('Origin',(30.5,-17.5710580837557,-33.7339653438087));
#74597=CARTESIAN_POINT('',(30.4955273645547,-18.0163441277467,-33.5136270415661));
#74598=CARTESIAN_POINT('Origin',(30.5,-18.0040707856479,-33.4839653438087));
#74599=CARTESIAN_POINT('',(24.1012882089558,-18.3802631128034,-33.3579488669236));
#74600=CARTESIAN_POINT('Origin',(24.1,-18.3504809471617,-33.2839653438087));
#74601=CARTESIAN_POINT('',(23.1004586919557,-18.0938594155378,-33.4416219555226));
#74602=CARTESIAN_POINT('Origin',(23.1,-18.0906733260264,-33.4339653438087));
#74603=CARTESIAN_POINT('',(22.399682944576,-17.742127215612,-33.6288475295615));
#74604=CARTESIAN_POINT('Origin',(22.4,-17.7442631645126,-33.6339653438087));
#74605=CARTESIAN_POINT('',(21.7998387845652,-17.5683840431675,-33.7273468611033));
#74606=CARTESIAN_POINT('Origin',(21.8,-17.5710580837557,-33.7339653438087));
#74607=CARTESIAN_POINT('',(13.2021921742626,-17.5346970308537,-33.6439685797945));
#74608=CARTESIAN_POINT('Origin',(13.2,-17.5710580837557,-33.7339653438087));
#74609=CARTESIAN_POINT('',(12.6002487187375,-17.7425875883397,-33.6299506000067));
#74610=CARTESIAN_POINT('Origin',(12.6,-17.7442631645126,-33.6339653438087));
#74611=CARTESIAN_POINT('',(11.8996457869536,-18.0931337015746,-33.4398779649625));
#74612=CARTESIAN_POINT('Origin',(11.9,-18.0906733260264,-33.4339653438087));
#74613=CARTESIAN_POINT('',(10.899790263986,-18.3553298442931,-33.2960107570711));
#74614=CARTESIAN_POINT('Origin',(10.9,-18.3504809471617,-33.2839653438087));
#74615=CARTESIAN_POINT('',(4.55736144060343,-18.1614760990067,-33.8643758947959));
#74616=CARTESIAN_POINT('Origin',(4.5,-18.0040707856479,-33.4839653438087));
#74617=CARTESIAN_POINT('',(4.49524972087093,-17.5582719500126,-33.7023185522751));
#74618=CARTESIAN_POINT('Origin',(4.5,-17.5710580837557,-33.7339653438087));
#74619=CARTESIAN_POINT('',(1.90350512467335,-17.5458051084359,-33.6714620365851));
#74620=CARTESIAN_POINT('Origin',(1.9,-17.5710580837557,-33.7339653438087));
#74621=CARTESIAN_POINT('Ctrl Pts',(0.138207714141623,-20.505353736182,-37.5246765162998));
#74622=CARTESIAN_POINT('Ctrl Pts',(0.370217470901057,-20.2509844800824,
-37.3992864560054));
#74623=CARTESIAN_POINT('Ctrl Pts',(0.600000000000006,-19.9986373454573,
-37.2739118462884));
#74624=CARTESIAN_POINT('Origin',(1.9,-20.4289419162443,-32.0839653438087));
#74625=CARTESIAN_POINT('',(5.09593997529677,-23.0652077022745,-35.4582316768749));
#74626=CARTESIAN_POINT('',(17.5,-23.0652077022745,-35.4582316768749));
#74627=CARTESIAN_POINT('',(4.47529854852883,-20.3196698518115,-31.9441034793054));
#74628=CARTESIAN_POINT('Origin',(4.5,-20.4289419162443,-32.0839653438087));
#74629=CARTESIAN_POINT('',(5.09944803334083,-22.6162805078382,-35.7462425436685));
#74630=CARTESIAN_POINT('Origin',(-0.840551718690874,0.,0.));
#74631=CARTESIAN_POINT('',(4.50447263544529,-20.01548032708,-32.3594252187343));
#74632=CARTESIAN_POINT('Origin',(4.5,-19.9959292143521,-32.3339653438087));
#74633=CARTESIAN_POINT('',(10.8302042597752,-22.3141421459872,-35.9356238333033));
#74634=CARTESIAN_POINT('Origin',(-62.7155570771054,0.,0.));
#74635=CARTESIAN_POINT('',(10.8987117910442,-19.6986995804965,-32.5967492173915));
#74636=CARTESIAN_POINT('Origin',(10.9,-19.6495190528383,-32.5339653438087));
#74637=CARTESIAN_POINT('',(11.6618634261911,-22.5247608043155,-35.8039823302991));
#74638=CARTESIAN_POINT('Origin',(26.9856656232739,0.,0.));
#74639=CARTESIAN_POINT('',(11.8995413080444,-19.9143644494692,-32.3905528841213));
#74640=CARTESIAN_POINT('Origin',(11.9,-19.9093266739737,-32.3839653438087));
#74641=CARTESIAN_POINT('',(12.3548486633046,-22.856966221146,-35.5928236469852));
#74642=CARTESIAN_POINT('Origin',(20.8267261185512,0.,0.));
#74643=CARTESIAN_POINT('',(12.600317055424,-20.2523726527879,-32.179556650676));
#74644=CARTESIAN_POINT('Origin',(12.6,-20.2557368354875,-32.1839653438087));
#74645=CARTESIAN_POINT('',(13.103292255208,-23.0652077022745,-35.4582316768749));
#74646=CARTESIAN_POINT('Origin',(25.13830739299,0.,0.));
#74647=CARTESIAN_POINT('',(13.2001612154348,-20.4245471623811,-32.0783403153759));
#74648=CARTESIAN_POINT('Origin',(13.2,-20.4289419162443,-32.0839653438087));
#74649=CARTESIAN_POINT('',(21.896707744792,-23.0652077022745,-35.4582316768749));
#74650=CARTESIAN_POINT('',(17.5,-23.0652077022745,-35.4582316768749));
#74651=CARTESIAN_POINT('',(21.7978078257374,-20.3691829588007,-32.0074773662801));
#74652=CARTESIAN_POINT('Origin',(21.8,-20.4289419162443,-32.0839653438087));
#74653=CARTESIAN_POINT('',(22.6451513366954,-22.856966221146,-35.5928236469852));
#74654=CARTESIAN_POINT('Origin',(9.86169260701005,0.,0.));
#74655=CARTESIAN_POINT('',(22.3997512812625,-20.2530977534517,-32.180506880376));
#74656=CARTESIAN_POINT('Origin',(22.4,-20.2557368354875,-32.1839653438087));
#74657=CARTESIAN_POINT('',(23.3381365738089,-22.5247608043155,-35.8039823302991));
#74658=CARTESIAN_POINT('Origin',(14.1732738814488,0.,0.));
#74659=CARTESIAN_POINT('',(23.1003542130464,-19.9132169663217,-32.3890524021132));
#74660=CARTESIAN_POINT('Origin',(23.1,-19.9093266739737,-32.3839653438087));
#74661=CARTESIAN_POINT('',(24.1697957402248,-22.3141421459872,-35.9356238333033));
#74662=CARTESIAN_POINT('Origin',(8.01433437672607,0.,0.));
#74663=CARTESIAN_POINT('',(24.100209736014,-19.657526238157,-32.544187318536));
#74664=CARTESIAN_POINT('Origin',(24.1,-19.6495190528383,-32.5339653438087));
#74665=CARTESIAN_POINT('',(29.9005519666592,-22.6162805078382,-35.7462425436685));
#74666=CARTESIAN_POINT('Origin',(97.7155570771054,0.,0.));
#74667=CARTESIAN_POINT('',(30.4426385593966,-20.2466717586954,-32.6604876193616));
#74668=CARTESIAN_POINT('Origin',(30.5,-19.9959292143521,-32.3339653438087));
#74669=CARTESIAN_POINT('',(29.9040600247032,-23.0652077022745,-35.4582316768749));
#74670=CARTESIAN_POINT('Origin',(35.8405517186909,0.,0.));
#74671=CARTESIAN_POINT('',(30.5047502791291,-20.4079280576996,-32.0570688314042));
#74672=CARTESIAN_POINT('Origin',(30.5,-20.4289419162443,-32.0839653438087));
#74673=CARTESIAN_POINT('',(17.5,-23.0652077022745,-35.4582316768749));
#74674=CARTESIAN_POINT('Origin',(17.5,-21.375,-37.0225860117847));
#74675=CARTESIAN_POINT('Origin',(17.5,0.,0.));
#74676=CARTESIAN_POINT('',(0.600000000000001,-26.1673599741116,-33.234910440458));
#74677=CARTESIAN_POINT('Origin',(0.600000000000001,0.,0.));
#74678=CARTESIAN_POINT('',(1.67735469196904,-25.4310730087083,-33.8016349549212));
#74679=CARTESIAN_POINT('Origin',(8.14497546096349,0.,0.));
#74680=CARTESIAN_POINT('',(5.09593997529677,-25.4310730087083,-33.8016349549212));
#74681=CARTESIAN_POINT('',(17.5,-25.4310730087083,-33.8016349549212));
#74682=CARTESIAN_POINT('',(5.09944803334083,-25.8552568383243,-33.4782869009794));
#74683=CARTESIAN_POINT('Origin',(-0.840551718690872,0.,0.));
#74684=CARTESIAN_POINT('',(10.8302042597752,-26.1365544445335,-33.2591419277157));
#74685=CARTESIAN_POINT('Origin',(-62.7155570771055,0.,0.));
#74686=CARTESIAN_POINT('',(11.6618634261911,-25.9408160718628,-33.4120346810215));
#74687=CARTESIAN_POINT('Origin',(26.9856656232739,0.,0.));
#74688=CARTESIAN_POINT('',(12.3548486633046,-25.6287708710599,-33.6519851366708));
#74689=CARTESIAN_POINT('Origin',(20.8267261185512,0.,0.));
#74690=CARTESIAN_POINT('',(13.103292255208,-25.4310730087083,-33.8016349549212));
#74691=CARTESIAN_POINT('Origin',(25.13830739299,0.,0.));
#74692=CARTESIAN_POINT('',(21.896707744792,-25.4310730087083,-33.8016349549212));
#74693=CARTESIAN_POINT('',(17.5,-25.4310730087083,-33.8016349549212));
#74694=CARTESIAN_POINT('',(22.6451513366954,-25.6287708710599,-33.6519851366708));
#74695=CARTESIAN_POINT('Origin',(9.86169260701005,0.,0.));
#74696=CARTESIAN_POINT('',(23.3381365738089,-25.9408160718628,-33.4120346810215));
#74697=CARTESIAN_POINT('Origin',(14.1732738814488,0.,0.));
#74698=CARTESIAN_POINT('',(24.1697957402248,-26.1365544445335,-33.2591419277157));
#74699=CARTESIAN_POINT('Origin',(8.01433437672609,0.,0.));
#74700=CARTESIAN_POINT('',(29.9005519666592,-25.8552568383243,-33.4782869009794));
#74701=CARTESIAN_POINT('Origin',(97.7155570771054,0.,0.));
#74702=CARTESIAN_POINT('',(29.9040600247032,-25.4310730087083,-33.8016349549212));
#74703=CARTESIAN_POINT('Origin',(35.8405517186909,0.,0.));
#74704=CARTESIAN_POINT('',(17.5,-25.4310730087083,-33.8016349549212));
#74705=CARTESIAN_POINT('Origin',(33.1,-23.1619558369422,-30.1702883945039));
#74706=CARTESIAN_POINT('',(30.5247014514712,-23.0679019220779,-30.0197706669552));
#74707=CARTESIAN_POINT('Origin',(30.5,-23.1619558369422,-30.1702883945039));
#74708=CARTESIAN_POINT('',(30.4955273645547,-23.562215640718,-29.8759744160904));
#74709=CARTESIAN_POINT('Origin',(30.5,-23.5449780585017,-29.8488945896607));
#74710=CARTESIAN_POINT('',(24.1012882089558,-23.893572647341,-29.6594674741542));
#74711=CARTESIAN_POINT('Origin',(24.1,-23.8513958357493,-29.5917795457861));
#74712=CARTESIAN_POINT('',(23.1004586919557,-23.6260497451375,-29.7916028606322));
#74713=CARTESIAN_POINT('Origin',(23.1,-23.6215825028136,-29.784615828692));
#74714=CARTESIAN_POINT('',(22.399682944576,-23.312172527411,-30.0370617130518));
#74715=CARTESIAN_POINT('Origin',(22.4,-23.315164725566,-30.0417308725666));
#74716=CARTESIAN_POINT('',(21.7998387845652,-23.1581731335784,-30.1642348036977));
#74717=CARTESIAN_POINT('Origin',(21.8,-23.1619558369422,-30.1702883945039));
#74718=CARTESIAN_POINT('',(13.2021921742626,-23.1105194160696,-30.0879729141313));
#74719=CARTESIAN_POINT('Origin',(13.2,-23.1619558369422,-30.1702883945039));
#74720=CARTESIAN_POINT('',(12.6002487187375,-23.3128174522151,-30.038068082493));
#74721=CARTESIAN_POINT('Origin',(12.6,-23.315164725566,-30.0417308725666));
#74722=CARTESIAN_POINT('',(11.8996457869536,-23.6250322156174,-29.7900113841146));
#74723=CARTESIAN_POINT('Origin',(11.9,-23.6215825028136,-29.784615828692));
#74724=CARTESIAN_POINT('',(10.899790263986,-23.8582627313001,-29.6027999600046));
#74725=CARTESIAN_POINT('Origin',(10.9,-23.8513958357493,-29.5917795457861));
#74726=CARTESIAN_POINT('',(4.55736144060343,-23.7660496304069,-30.1961927037808));
#74727=CARTESIAN_POINT('Origin',(4.5,-23.5449780585017,-29.8488945896607));
#74728=CARTESIAN_POINT('',(4.49524972087093,-23.1438685456221,-30.1413426776676));
#74729=CARTESIAN_POINT('Origin',(4.5,-23.1619558369422,-30.1702883945039));
#74730=CARTESIAN_POINT('',(1.90350512467335,-23.1262329256631,-30.1131197861062));
#74731=CARTESIAN_POINT('Origin',(1.9,-23.1619558369422,-30.1702883945039));
#74732=CARTESIAN_POINT('Ctrl Pts',(0.138207714141625,-26.7099230322463,
-33.3938750538235));
#74733=CARTESIAN_POINT('Ctrl Pts',(0.370217470898728,-26.4376444612466,
-33.3145607080718));
#74734=CARTESIAN_POINT('Ctrl Pts',(0.600000000000006,-26.1673599741116,
-33.234910440458));
#74735=CARTESIAN_POINT('Origin',(1.9,-25.6899024992348,-28.0490892825384));
#74736=CARTESIAN_POINT('',(5.09593997529677,-28.872052684018,-30.9143101784803));
#74737=CARTESIAN_POINT('',(17.5,-28.872052684018,-30.9143101784803));
#74738=CARTESIAN_POINT('',(4.47529854852883,-25.5580037650976,-27.9303271288835));
#74739=CARTESIAN_POINT('Origin',(4.5,-25.6899024992348,-28.0490892825384));
#74740=CARTESIAN_POINT('',(5.09944803334083,-28.4799582645661,-31.2759009022694));
#74741=CARTESIAN_POINT('Origin',(-0.840551718690874,0.,0.));
#74742=CARTESIAN_POINT('',(4.50447263544529,-25.3305554259542,-28.3921611545025));
#74743=CARTESIAN_POINT('Origin',(4.5,-25.3068802776753,-28.3704830873816));
#74744=CARTESIAN_POINT('',(10.8302042597752,-28.2152957791621,-31.5148708405159));
#74745=CARTESIAN_POINT('Origin',(-62.7155570771053,0.,0.));
#74746=CARTESIAN_POINT('',(10.8987117910442,-25.0597981705973,-28.6808880677203));
#74747=CARTESIAN_POINT('Origin',(10.9,-25.0004625004277,-28.6275981312563));
#74748=CARTESIAN_POINT('',(11.6618634261911,-28.3998553597108,-31.3486557215378));
#74749=CARTESIAN_POINT('Origin',(26.9856656232739,0.,0.));
#74750=CARTESIAN_POINT('',(11.8995413080444,-25.2363809880999,-28.4403745085892));
#74751=CARTESIAN_POINT('Origin',(11.9,-25.2302758333634,-28.4347618483503));
#74752=CARTESIAN_POINT('',(12.3548486633046,-28.6903465092421,-31.0830181478507));
#74753=CARTESIAN_POINT('Origin',(20.8267261185512,0.,0.));
#74754=CARTESIAN_POINT('',(12.600317055424,-25.5326149758775,-28.1738892734932));
#74755=CARTESIAN_POINT('Origin',(12.6,-25.536693610611,-28.1776468044757));
#74756=CARTESIAN_POINT('',(13.103292255208,-28.872052684018,-30.9143101784803));
#74757=CARTESIAN_POINT('Origin',(25.13830739299,0.,0.));
#74758=CARTESIAN_POINT('',(13.2001612154348,-25.684597735621,-28.0443128519265));
#74759=CARTESIAN_POINT('Origin',(13.2,-25.6899024992348,-28.0490892825384));
#74760=CARTESIAN_POINT('',(21.896707744792,-28.872052684018,-30.9143101784803));
#74761=CARTESIAN_POINT('',(17.5,-28.872052684018,-30.9143101784803));
#74762=CARTESIAN_POINT('',(21.7978078257374,-25.6177694167211,-27.9841403633154));
#74763=CARTESIAN_POINT('Origin',(21.8,-25.6899024992348,-28.0490892825384));
#74764=CARTESIAN_POINT('',(22.6451513366954,-28.6903465092421,-31.0830181478507));
#74765=CARTESIAN_POINT('Origin',(9.86169260701004,0.,0.));
#74766=CARTESIAN_POINT('',(22.3997512812625,-25.5334940662887,-28.1746991546599));
#74767=CARTESIAN_POINT('Origin',(22.4,-25.536693610611,-28.1776468044757));
#74768=CARTESIAN_POINT('',(23.3381365738089,-28.3998553597108,-31.3486557215378));
#74769=CARTESIAN_POINT('Origin',(14.1732738814488,0.,0.));
#74770=CARTESIAN_POINT('',(23.1003542130464,-25.2349903818335,-28.4390960806318));
#74771=CARTESIAN_POINT('Origin',(23.1,-25.2302758333634,-28.4347618483503));
#74772=CARTESIAN_POINT('',(24.1697957402248,-28.2152957791621,-31.5148708405159));
#74773=CARTESIAN_POINT('Origin',(8.01433437672607,0.,0.));
#74774=CARTESIAN_POINT('',(24.100209736014,-25.0101230658929,-28.63627437808));
#74775=CARTESIAN_POINT('Origin',(24.1,-25.0004625004277,-28.6275981312563));
#74776=CARTESIAN_POINT('',(29.9005519666592,-28.4799582645661,-31.2759009022694));
#74777=CARTESIAN_POINT('Origin',(97.7155570771054,0.,0.));
#74778=CARTESIAN_POINT('',(30.4426385593966,-25.610513477472,-28.6485037699886));
#74779=CARTESIAN_POINT('Origin',(30.5,-25.3068802776753,-28.3704830873816));
#74780=CARTESIAN_POINT('',(29.9040600247032,-28.872052684018,-30.9143101784803));
#74781=CARTESIAN_POINT('Origin',(35.8405517186909,0.,0.));
#74782=CARTESIAN_POINT('',(30.5047502791291,-25.6645373580546,-28.0262504068355));
#74783=CARTESIAN_POINT('Origin',(30.5,-25.6899024992348,-28.0490892825384));
#74784=CARTESIAN_POINT('',(17.5,-28.872052684018,-30.9143101784803));
#74785=CARTESIAN_POINT('Origin',(17.5,-27.4791703140996,-32.7483999433363));
#74786=CARTESIAN_POINT('Origin',(17.5,0.,0.));
#74787=CARTESIAN_POINT('',(0.600000000000001,-31.5410006112756,-28.1860830985703));
#74788=CARTESIAN_POINT('Origin',(0.600000000000001,0.,0.));
#74789=CARTESIAN_POINT('',(1.67735469196904,-30.9143101784803,-28.872052684018));
#74790=CARTESIAN_POINT('Origin',(8.14497546096349,0.,0.));
#74791=CARTESIAN_POINT('',(5.09593997529677,-30.9143101784803,-28.872052684018));
#74792=CARTESIAN_POINT('',(17.5,-30.9143101784803,-28.872052684018));
#74793=CARTESIAN_POINT('',(5.09944803334083,-31.2759009022694,-28.4799582645661));
#74794=CARTESIAN_POINT('Origin',(-0.840551718690872,0.,0.));
#74795=CARTESIAN_POINT('',(10.8302042597752,-31.5148708405159,-28.2152957791621));
#74796=CARTESIAN_POINT('Origin',(-62.7155570771055,0.,0.));
#74797=CARTESIAN_POINT('',(11.6618634261911,-31.3486557215378,-28.3998553597108));
#74798=CARTESIAN_POINT('Origin',(26.9856656232739,0.,0.));
#74799=CARTESIAN_POINT('',(12.3548486633046,-31.0830181478507,-28.6903465092421));
#74800=CARTESIAN_POINT('Origin',(20.8267261185512,0.,0.));
#74801=CARTESIAN_POINT('',(13.103292255208,-30.9143101784803,-28.872052684018));
#74802=CARTESIAN_POINT('Origin',(25.13830739299,0.,0.));
#74803=CARTESIAN_POINT('',(21.896707744792,-30.9143101784803,-28.872052684018));
#74804=CARTESIAN_POINT('',(17.5,-30.9143101784803,-28.872052684018));
#74805=CARTESIAN_POINT('',(22.6451513366954,-31.0830181478507,-28.6903465092421));
#74806=CARTESIAN_POINT('Origin',(9.86169260701006,0.,0.));
#74807=CARTESIAN_POINT('',(23.3381365738089,-31.3486557215378,-28.3998553597108));
#74808=CARTESIAN_POINT('Origin',(14.1732738814488,0.,0.));
#74809=CARTESIAN_POINT('',(24.1697957402248,-31.5148708405159,-28.2152957791621));
#74810=CARTESIAN_POINT('Origin',(8.01433437672608,0.,0.));
#74811=CARTESIAN_POINT('',(29.9005519666592,-31.2759009022694,-28.4799582645661));
#74812=CARTESIAN_POINT('Origin',(97.7155570771054,0.,0.));
#74813=CARTESIAN_POINT('',(29.9040600247032,-30.9143101784803,-28.872052684018));
#74814=CARTESIAN_POINT('Origin',(35.8405517186909,0.,0.));
#74815=CARTESIAN_POINT('',(17.5,-30.9143101784803,-28.872052684018));
#74816=CARTESIAN_POINT('Origin',(33.1,-28.0490892825384,-25.6899024992348));
#74817=CARTESIAN_POINT('',(30.5247014514712,-27.9303271288835,-25.5580037650976));
#74818=CARTESIAN_POINT('Origin',(30.5,-28.0490892825384,-25.6899024992348));
#74819=CARTESIAN_POINT('',(30.4955273645547,-28.3921611545025,-25.3305554259542));
#74820=CARTESIAN_POINT('Origin',(30.5,-28.3704830873816,-25.3068802776753));
#74821=CARTESIAN_POINT('',(24.1012882089558,-28.6808880677203,-25.0597981705973));
#74822=CARTESIAN_POINT('Origin',(24.1,-28.6275981312563,-25.0004625004277));
#74823=CARTESIAN_POINT('',(23.1004586919557,-28.4403745085892,-25.2363809880999));
#74824=CARTESIAN_POINT('Origin',(23.1,-28.4347618483503,-25.2302758333634));
#74825=CARTESIAN_POINT('',(22.399682944576,-28.1738892734932,-25.5326149758775));
#74826=CARTESIAN_POINT('Origin',(22.4,-28.1776468044757,-25.536693610611));
#74827=CARTESIAN_POINT('',(21.7998387845652,-28.0443128519265,-25.684597735621));
#74828=CARTESIAN_POINT('Origin',(21.8,-28.0490892825384,-25.6899024992348));
#74829=CARTESIAN_POINT('',(13.2021921742626,-27.9841403633154,-25.6177694167211));
#74830=CARTESIAN_POINT('Origin',(13.2,-28.0490892825384,-25.6899024992348));
#74831=CARTESIAN_POINT('',(12.6002487187375,-28.1746991546599,-25.5334940662887));
#74832=CARTESIAN_POINT('Origin',(12.6,-28.1776468044757,-25.536693610611));
#74833=CARTESIAN_POINT('',(11.8996457869536,-28.4390960806318,-25.2349903818335));
#74834=CARTESIAN_POINT('Origin',(11.9,-28.4347618483503,-25.2302758333634));
#74835=CARTESIAN_POINT('',(10.899790263986,-28.63627437808,-25.0101230658929));
#74836=CARTESIAN_POINT('Origin',(10.9,-28.6275981312563,-25.0004625004277));
#74837=CARTESIAN_POINT('',(4.55736144060343,-28.6485037699886,-25.610513477472));
#74838=CARTESIAN_POINT('Origin',(4.5,-28.3704830873816,-25.3068802776753));
#74839=CARTESIAN_POINT('',(4.49524972087093,-28.0262504068355,-25.6645373580546));
#74840=CARTESIAN_POINT('Origin',(4.5,-28.0490892825384,-25.6899024992348));
#74841=CARTESIAN_POINT('',(1.90350512467335,-28.0039818578826,-25.6398056289004));
#74842=CARTESIAN_POINT('Origin',(1.9,-28.0490892825384,-25.6899024992348));
#74843=CARTESIAN_POINT('Ctrl Pts',(0.138207714141624,-32.1029248328492,
-28.2484175959527));
#74844=CARTESIAN_POINT('Ctrl Pts',(0.370217470897375,-31.8210099935485,
-28.2175888910035));
#74845=CARTESIAN_POINT('Ctrl Pts',(0.600000000000006,-31.5410006112756,
-28.1860830985703));
#74846=CARTESIAN_POINT('Origin',(1.9,-30.170288394504,-23.1619558369422));
#74847=CARTESIAN_POINT('',(5.09593997529677,-33.8016349549212,-25.4310730087083));
#74848=CARTESIAN_POINT('',(17.5,-33.8016349549212,-25.4310730087083));
#74849=CARTESIAN_POINT('',(4.47529854852883,-30.0197706669552,-23.0679019220779));
#74850=CARTESIAN_POINT('Origin',(4.5,-30.170288394504,-23.1619558369422));
#74851=CARTESIAN_POINT('',(5.09944803334083,-33.4782869009794,-25.8552568383243));
#74852=CARTESIAN_POINT('Origin',(-0.840551718690874,0.,0.));
#74853=CARTESIAN_POINT('',(4.50447263544529,-29.8759744160904,-23.562215640718));
#74854=CARTESIAN_POINT('Origin',(4.5,-29.8488945896607,-23.5449780585017));
#74855=CARTESIAN_POINT('',(10.8302042597752,-33.2591419277157,-26.1365544445334));
#74856=CARTESIAN_POINT('Origin',(-62.7155570771055,0.,0.));
#74857=CARTESIAN_POINT('',(10.8987117910442,-29.6594674741542,-23.893572647341));
#74858=CARTESIAN_POINT('Origin',(10.9,-29.5917795457861,-23.8513958357493));
#74859=CARTESIAN_POINT('',(11.6618634261911,-33.4120346810215,-25.9408160718628));
#74860=CARTESIAN_POINT('Origin',(26.9856656232739,0.,0.));
#74861=CARTESIAN_POINT('',(11.8995413080444,-29.7916028606322,-23.6260497451375));
#74862=CARTESIAN_POINT('Origin',(11.9,-29.784615828692,-23.6215825028136));
#74863=CARTESIAN_POINT('',(12.3548486633046,-33.6519851366708,-25.6287708710599));
#74864=CARTESIAN_POINT('Origin',(20.8267261185512,0.,0.));
#74865=CARTESIAN_POINT('',(12.600317055424,-30.0370617130518,-23.312172527411));
#74866=CARTESIAN_POINT('Origin',(12.6,-30.0417308725667,-23.315164725566));
#74867=CARTESIAN_POINT('',(13.103292255208,-33.8016349549212,-25.4310730087083));
#74868=CARTESIAN_POINT('Origin',(25.13830739299,0.,0.));
#74869=CARTESIAN_POINT('',(13.2001612154348,-30.1642348036977,-23.1581731335784));
#74870=CARTESIAN_POINT('Origin',(13.2,-30.170288394504,-23.1619558369422));
#74871=CARTESIAN_POINT('',(21.896707744792,-33.8016349549212,-25.4310730087083));
#74872=CARTESIAN_POINT('',(17.5,-33.8016349549212,-25.4310730087083));
#74873=CARTESIAN_POINT('',(21.7978078257374,-30.0879729141313,-23.1105194160696));
#74874=CARTESIAN_POINT('Origin',(21.8,-30.170288394504,-23.1619558369422));
#74875=CARTESIAN_POINT('',(22.6451513366954,-33.6519851366708,-25.6287708710599));
#74876=CARTESIAN_POINT('Origin',(9.86169260701005,0.,0.));
#74877=CARTESIAN_POINT('',(22.3997512812625,-30.0380680824931,-23.3128174522151));
#74878=CARTESIAN_POINT('Origin',(22.4,-30.0417308725667,-23.315164725566));
#74879=CARTESIAN_POINT('',(23.3381365738089,-33.4120346810215,-25.9408160718628));
#74880=CARTESIAN_POINT('Origin',(14.1732738814488,0.,0.));
#74881=CARTESIAN_POINT('',(23.1003542130464,-29.7900113841146,-23.6250322156174));
#74882=CARTESIAN_POINT('Origin',(23.1,-29.784615828692,-23.6215825028136));
#74883=CARTESIAN_POINT('',(24.1697957402248,-33.2591419277157,-26.1365544445335));
#74884=CARTESIAN_POINT('Origin',(8.01433437672607,0.,0.));
#74885=CARTESIAN_POINT('',(24.100209736014,-29.6027999600046,-23.8582627313001));
#74886=CARTESIAN_POINT('Origin',(24.1,-29.5917795457861,-23.8513958357493));
#74887=CARTESIAN_POINT('',(29.9005519666592,-33.4782869009794,-25.8552568383243));
#74888=CARTESIAN_POINT('Origin',(97.7155570771054,0.,0.));
#74889=CARTESIAN_POINT('',(30.4426385593966,-30.1961927037808,-23.7660496304069));
#74890=CARTESIAN_POINT('Origin',(30.5,-29.8488945896607,-23.5449780585017));
#74891=CARTESIAN_POINT('',(29.9040600247032,-33.8016349549212,-25.4310730087083));
#74892=CARTESIAN_POINT('Origin',(35.8405517186909,0.,0.));
#74893=CARTESIAN_POINT('',(30.5047502791291,-30.1413426776677,-23.1438685456221));
#74894=CARTESIAN_POINT('Origin',(30.5,-30.170288394504,-23.1619558369422));
#74895=CARTESIAN_POINT('',(17.5,-33.8016349549212,-25.4310730087083));
#74896=CARTESIAN_POINT('Origin',(17.5,-32.7483999433363,-27.4791703140996));
#74897=CARTESIAN_POINT('Origin',(17.5,0.,0.));
#74898=CARTESIAN_POINT('',(0.600000000000001,-35.9562839053824,-22.2808358845789));
#74899=CARTESIAN_POINT('Origin',(0.600000000000001,0.,0.));
#74900=CARTESIAN_POINT('',(1.67735469196904,-35.4582316768749,-23.0652077022745));
#74901=CARTESIAN_POINT('Origin',(8.14497546096349,0.,0.));
#74902=CARTESIAN_POINT('',(5.09593997529677,-35.4582316768749,-23.0652077022745));
#74903=CARTESIAN_POINT('',(17.5,-35.4582316768749,-23.0652077022745));
#74904=CARTESIAN_POINT('',(5.09944803334083,-35.7462425436685,-22.6162805078382));
#74905=CARTESIAN_POINT('Origin',(-0.840551718690872,0.,0.));
#74906=CARTESIAN_POINT('',(10.8302042597752,-35.9356238333033,-22.3141421459872));
#74907=CARTESIAN_POINT('Origin',(-62.7155570771054,0.,0.));
#74908=CARTESIAN_POINT('',(11.6618634261911,-35.8039823302992,-22.5247608043154));
#74909=CARTESIAN_POINT('Origin',(26.9856656232739,0.,0.));
#74910=CARTESIAN_POINT('',(12.3548486633046,-35.5928236469852,-22.856966221146));
#74911=CARTESIAN_POINT('Origin',(20.8267261185512,0.,0.));
#74912=CARTESIAN_POINT('',(13.103292255208,-35.4582316768749,-23.0652077022745));
#74913=CARTESIAN_POINT('Origin',(25.13830739299,0.,0.));
#74914=CARTESIAN_POINT('',(21.896707744792,-35.4582316768749,-23.0652077022745));
#74915=CARTESIAN_POINT('',(17.5,-35.4582316768749,-23.0652077022745));
#74916=CARTESIAN_POINT('',(22.6451513366954,-35.5928236469852,-22.856966221146));
#74917=CARTESIAN_POINT('Origin',(9.86169260701006,0.,0.));
#74918=CARTESIAN_POINT('',(23.3381365738089,-35.8039823302992,-22.5247608043154));
#74919=CARTESIAN_POINT('Origin',(14.1732738814488,0.,0.));
#74920=CARTESIAN_POINT('',(24.1697957402248,-35.9356238333033,-22.3141421459872));
#74921=CARTESIAN_POINT('Origin',(8.0143343767261,0.,0.));
#74922=CARTESIAN_POINT('',(29.9005519666592,-35.7462425436685,-22.6162805078382));
#74923=CARTESIAN_POINT('Origin',(97.7155570771053,0.,0.));
#74924=CARTESIAN_POINT('',(29.9040600247032,-35.4582316768749,-23.0652077022745));
#74925=CARTESIAN_POINT('Origin',(35.8405517186909,0.,0.));
#74926=CARTESIAN_POINT('',(17.5,-35.4582316768749,-23.0652077022745));
#74927=CARTESIAN_POINT('Origin',(33.1,-32.0839653438087,-20.4289419162443));
#74928=CARTESIAN_POINT('',(30.5247014514712,-31.9441034793054,-20.3196698518115));
#74929=CARTESIAN_POINT('Origin',(30.5,-32.0839653438087,-20.4289419162443));
#74930=CARTESIAN_POINT('',(30.4955273645547,-32.3594252187343,-20.01548032708));
#74931=CARTESIAN_POINT('Origin',(30.5,-32.3339653438087,-19.9959292143521));
#74932=CARTESIAN_POINT('',(24.1012882089558,-32.5967492173916,-19.6986995804965));
#74933=CARTESIAN_POINT('Origin',(24.1,-32.5339653438087,-19.6495190528383));
#74934=CARTESIAN_POINT('',(23.1004586919557,-32.3905528841213,-19.9143644494691));
#74935=CARTESIAN_POINT('Origin',(23.1,-32.3839653438087,-19.9093266739736));
#74936=CARTESIAN_POINT('',(22.399682944576,-32.1795566506761,-20.2523726527878));
#74937=CARTESIAN_POINT('Origin',(22.4,-32.1839653438087,-20.2557368354874));
#74938=CARTESIAN_POINT('',(21.7998387845652,-32.0783403153759,-20.4245471623811));
#74939=CARTESIAN_POINT('Origin',(21.8,-32.0839653438087,-20.4289419162443));
#74940=CARTESIAN_POINT('',(13.2021921742626,-32.0074773662801,-20.3691829588007));
#74941=CARTESIAN_POINT('Origin',(13.2,-32.0839653438087,-20.4289419162443));
#74942=CARTESIAN_POINT('',(12.6002487187375,-32.180506880376,-20.2530977534517));
#74943=CARTESIAN_POINT('Origin',(12.6,-32.1839653438087,-20.2557368354874));
#74944=CARTESIAN_POINT('',(11.8996457869536,-32.3890524021132,-19.9132169663217));
#74945=CARTESIAN_POINT('Origin',(11.9,-32.3839653438087,-19.9093266739736));
#74946=CARTESIAN_POINT('',(10.899790263986,-32.544187318536,-19.6575262381569));
#74947=CARTESIAN_POINT('Origin',(10.9,-32.5339653438087,-19.6495190528383));
#74948=CARTESIAN_POINT('',(4.55736144060343,-32.6604876193617,-20.2466717586953));
#74949=CARTESIAN_POINT('Origin',(4.5,-32.3339653438087,-19.9959292143521));
#74950=CARTESIAN_POINT('',(4.49524972087093,-32.0570688314042,-20.4079280576995));
#74951=CARTESIAN_POINT('Origin',(4.5,-32.0839653438087,-20.4289419162443));
#74952=CARTESIAN_POINT('',(1.90350512467335,-32.0308439720488,-20.387438952028));
#74953=CARTESIAN_POINT('Origin',(1.9,-32.0839653438087,-20.4289419162443));
#74954=CARTESIAN_POINT('Ctrl Pts',(0.138207714141622,-36.5204955072697,
-22.244646263818));
#74955=CARTESIAN_POINT('Ctrl Pts',(0.37021747089714,-36.2375102394032,-22.2632399142705));
#74956=CARTESIAN_POINT('Ctrl Pts',(0.600000000000006,-35.9562839053824,
-22.2808358845789));
#74957=CARTESIAN_POINT('Origin',(1.9,-33.7339653438087,-17.5710580837557));
#74958=CARTESIAN_POINT('',(5.09593997529677,-37.7041716521717,-19.1751255543105));
#74959=CARTESIAN_POINT('',(17.5,-37.7041716521717,-19.1751255543105));
#74960=CARTESIAN_POINT('',(4.47529854852883,-33.5694020278343,-17.5045701882916));
#74961=CARTESIAN_POINT('Origin',(4.5,-33.7339653438087,-17.5710580837557));
#74962=CARTESIAN_POINT('',(5.09944803334084,-37.459394730737,-19.6490138787379));
#74963=CARTESIAN_POINT('Origin',(-0.840551718690874,0.,0.));
#74964=CARTESIAN_POINT('',(4.50447263544529,-33.5136270415661,-18.0163441277467));
#74965=CARTESIAN_POINT('Origin',(4.5,-33.4839653438087,-18.0040707856479));
#74966=CARTESIAN_POINT('',(10.8302042597752,-37.2924258787336,-19.9640920674886));
#74967=CARTESIAN_POINT('Origin',(-62.7155570771054,0.,0.));
#74968=CARTESIAN_POINT('',(10.8987117910442,-33.3579488669236,-18.3802631128033));
#74969=CARTESIAN_POINT('Origin',(10.9,-33.2839653438087,-18.3504809471617));
#74970=CARTESIAN_POINT('',(11.6618634261911,-37.4090062358548,-19.7447778525305));
#74971=CARTESIAN_POINT('Origin',(26.9856656232739,0.,0.));
#74972=CARTESIAN_POINT('',(11.8995413080444,-33.4416219555226,-18.0938594155378));
#74973=CARTESIAN_POINT('Origin',(11.9,-33.4339653438087,-18.0906733260263));
#74974=CARTESIAN_POINT('',(12.3548486633046,-37.5911252244479,-19.3958063601357));
#74975=CARTESIAN_POINT('Origin',(20.8267261185512,0.,0.));
#74976=CARTESIAN_POINT('',(12.600317055424,-33.6288475295616,-17.742127215612));
#74977=CARTESIAN_POINT('Origin',(12.6,-33.6339653438087,-17.7442631645126));
#74978=CARTESIAN_POINT('',(13.103292255208,-37.7041716521717,-19.1751255543105));
#74979=CARTESIAN_POINT('Origin',(25.13830739299,0.,0.));
#74980=CARTESIAN_POINT('',(13.2001612154348,-33.7273468611033,-17.5683840431675));
#74981=CARTESIAN_POINT('Origin',(13.2,-33.7339653438087,-17.5710580837557));
#74982=CARTESIAN_POINT('',(21.896707744792,-37.7041716521717,-19.1751255543105));
#74983=CARTESIAN_POINT('',(17.5,-37.7041716521717,-19.1751255543105));
#74984=CARTESIAN_POINT('',(21.7978078257374,-33.6439685797946,-17.5346970308537));
#74985=CARTESIAN_POINT('Origin',(21.8,-33.7339653438087,-17.5710580837557));
#74986=CARTESIAN_POINT('',(22.6451513366954,-37.5911252244479,-19.3958063601357));
#74987=CARTESIAN_POINT('Origin',(9.86169260701005,0.,0.));
#74988=CARTESIAN_POINT('',(22.3997512812625,-33.6299506000067,-17.7425875883397));
#74989=CARTESIAN_POINT('Origin',(22.4,-33.6339653438087,-17.7442631645126));
#74990=CARTESIAN_POINT('',(23.3381365738089,-37.4090062358548,-19.7447778525305));
#74991=CARTESIAN_POINT('Origin',(14.1732738814488,0.,0.));
#74992=CARTESIAN_POINT('',(23.1003542130464,-33.4398779649625,-18.0931337015746));
#74993=CARTESIAN_POINT('Origin',(23.1,-33.4339653438087,-18.0906733260263));
#74994=CARTESIAN_POINT('',(24.1697957402248,-37.2924258787336,-19.9640920674886));
#74995=CARTESIAN_POINT('Origin',(8.01433437672607,0.,0.));
#74996=CARTESIAN_POINT('',(24.100209736014,-33.2960107570711,-18.3553298442931));
#74997=CARTESIAN_POINT('Origin',(24.1,-33.2839653438087,-18.3504809471617));
#74998=CARTESIAN_POINT('',(29.9005519666592,-37.459394730737,-19.6490138787379));
#74999=CARTESIAN_POINT('Origin',(97.7155570771054,0.,0.));
#75000=CARTESIAN_POINT('',(30.4426385593966,-33.864375894796,-18.1614760990067));
#75001=CARTESIAN_POINT('Origin',(30.5,-33.4839653438087,-18.0040707856479));
#75002=CARTESIAN_POINT('',(29.9040600247032,-37.7041716521717,-19.1751255543105));
#75003=CARTESIAN_POINT('Origin',(35.8405517186909,0.,0.));
#75004=CARTESIAN_POINT('',(30.5047502791291,-33.7023185522751,-17.5582719500126));
#75005=CARTESIAN_POINT('Origin',(30.5,-33.7339653438087,-17.5710580837557));
#75006=CARTESIAN_POINT('',(17.5,-37.7041716521717,-19.1751255543105));
#75007=CARTESIAN_POINT('Origin',(17.5,-37.0225860117848,-21.375));
#75008=CARTESIAN_POINT('Origin',(17.5,0.,0.));
#75009=CARTESIAN_POINT('',(0.600000000000001,-39.2790537077817,-15.6985967468815));
#75010=CARTESIAN_POINT('Origin',(0.600000000000001,0.,0.));
#75011=CARTESIAN_POINT('',(1.67735469196904,-38.9247727484987,-16.5575380560557));
#75012=CARTESIAN_POINT('Origin',(8.14497546096349,0.,0.));
#75013=CARTESIAN_POINT('',(5.09593997529677,-38.9247727484987,-16.5575380560557));
#75014=CARTESIAN_POINT('',(17.5,-38.9247727484987,-16.5575380560557));
#75015=CARTESIAN_POINT('',(5.09944803334083,-39.1304526938498,-16.0654185122698));
#75016=CARTESIAN_POINT('Origin',(-0.840551718690872,0.,0.));
#75017=CARTESIAN_POINT('',(10.8302042597752,-39.2644910802189,-15.7349845952072));
#75018=CARTESIAN_POINT('Origin',(-62.7155570771054,0.,0.));
#75019=CARTESIAN_POINT('',(11.6618634261911,-39.1714230536436,-15.9652627899599));
#75020=CARTESIAN_POINT('Origin',(26.9856656232739,0.,0.));
#75021=CARTESIAN_POINT('',(12.3548486633046,-39.0211592104439,-16.3290885806033));
#75022=CARTESIAN_POINT('Origin',(20.8267261185512,0.,0.));
#75023=CARTESIAN_POINT('',(13.103292255208,-38.9247727484987,-16.5575380560557));
#75024=CARTESIAN_POINT('Origin',(25.13830739299,0.,0.));
#75025=CARTESIAN_POINT('',(21.896707744792,-38.9247727484987,-16.5575380560557));
#75026=CARTESIAN_POINT('',(17.5,-38.9247727484987,-16.5575380560557));
#75027=CARTESIAN_POINT('',(22.6451513366954,-39.0211592104439,-16.3290885806033));
#75028=CARTESIAN_POINT('Origin',(9.86169260701007,0.,0.));
#75029=CARTESIAN_POINT('',(23.3381365738089,-39.1714230536436,-15.9652627899599));
#75030=CARTESIAN_POINT('Origin',(14.1732738814488,0.,0.));
#75031=CARTESIAN_POINT('',(24.1697957402248,-39.2644910802189,-15.7349845952072));
#75032=CARTESIAN_POINT('Origin',(8.01433437672609,0.,0.));
#75033=CARTESIAN_POINT('',(29.9005519666592,-39.1304526938498,-16.0654185122698));
#75034=CARTESIAN_POINT('Origin',(97.7155570771054,0.,0.));
#75035=CARTESIAN_POINT('',(29.9040600247032,-38.9247727484987,-16.5575380560557));
#75036=CARTESIAN_POINT('Origin',(35.8405517186909,0.,0.));
#75037=CARTESIAN_POINT('',(17.5,-38.9247727484987,-16.5575380560557));
#75038=CARTESIAN_POINT('Origin',(33.1,-35.1439863533772,-14.5472582706722));
#75039=CARTESIAN_POINT('',(30.5247014514712,-34.987274410005,-14.4639330523272));
#75040=CARTESIAN_POINT('Origin',(30.5,-35.1439863533772,-14.5472582706722));
#75041=CARTESIAN_POINT('',(30.4955273645547,-35.343464522354,-14.0922449867892));
#75042=CARTESIAN_POINT('Origin',(30.5,-35.31499642504,-14.0774119602792));
#75043=CARTESIAN_POINT('',(24.1012882089558,-35.5221746368434,-13.7390659716653));
#75044=CARTESIAN_POINT('Origin',(24.1,-35.4518044823703,-13.7015349119648));
#75045=CARTESIAN_POINT('',(23.1004586919557,-35.35656070068,-13.9872600241959));
#75046=CARTESIAN_POINT('Origin',(23.1,-35.3491984393726,-13.9834426982006));
#75047=CARTESIAN_POINT('',(22.399682944576,-35.2074644826695,-14.3567722348382));
#75048=CARTESIAN_POINT('Origin',(22.4,-35.2123903820423,-14.359319746515));
#75049=CARTESIAN_POINT('',(21.7998387845652,-35.137683640766,-14.5439070589317));
#75050=CARTESIAN_POINT('Origin',(21.8,-35.1439863533772,-14.5472582706722));
#75051=CARTESIAN_POINT('',(13.2021921742626,-35.0582833660355,-14.501689183981));
#75052=CARTESIAN_POINT('Origin',(13.2,-35.1439863533772,-14.5472582706722));
#75053=CARTESIAN_POINT('',(12.6002487187375,-35.208526188654,-14.3573213139379));
#75054=CARTESIAN_POINT('Origin',(12.6,-35.2123903820423,-14.359319746515));
#75055=CARTESIAN_POINT('',(11.8996457869536,-35.3548837560077,-13.9863905298622));
#75056=CARTESIAN_POINT('Origin',(11.9,-35.3491984393726,-13.9834426982006));
#75057=CARTESIAN_POINT('',(10.899790263986,-35.4632615954717,-13.7076454228629));
#75058=CARTESIAN_POINT('Origin',(10.9,-35.4518044823703,-13.7015349119648));
#75059=CARTESIAN_POINT('',(4.55736144060343,-35.6800990794245,-14.267645163841));
#75060=CARTESIAN_POINT('Origin',(4.5,-35.31499642504,-14.0774119602792));
#75061=CARTESIAN_POINT('',(4.49524972087093,-35.1138494411902,-14.5312341902212));
#75062=CARTESIAN_POINT('Origin',(4.5,-35.1439863533772,-14.5472582706722));
#75063=CARTESIAN_POINT('',(1.90350512467335,-35.0844651005135,-14.5156102591402));
#75064=CARTESIAN_POINT('Origin',(1.9,-35.1439863533772,-14.5472582706722));
#75065=CARTESIAN_POINT('Ctrl Pts',(0.138207714141633,-39.8284094059642,
-15.5649826112914));
#75066=CARTESIAN_POINT('Ctrl Pts',(0.370217470894376,-39.5529520737016,
-15.6324336584845));
#75067=CARTESIAN_POINT('Ctrl Pts',(0.600000000000006,-39.2790537077817,
-15.6985967468815));
#75068=CARTESIAN_POINT('Origin',(1.9,-36.2726528263519,-11.4462726220787));
#75069=CARTESIAN_POINT('',(5.09593997529677,-40.4610861730024,-12.3365516130268));
#75070=CARTESIAN_POINT('',(17.5,-40.4610861730024,-12.3365516130268));
#75071=CARTESIAN_POINT('',(4.47529854852883,-36.0990440950346,-11.409370947074));
#75072=CARTESIAN_POINT('Origin',(4.5,-36.2726528263519,-11.4462726220787));
#75073=CARTESIAN_POINT('',(5.09944803334083,-40.3023178069695,-12.8457455753269));
#75074=CARTESIAN_POINT('Origin',(-0.840551718690874,0.,0.));
#75075=CARTESIAN_POINT('',(4.50447263544529,-36.1329850680974,-11.9230551151638));
#75076=CARTESIAN_POINT('Origin',(4.5,-36.101642754689,-11.9161189324716));
#75077=CARTESIAN_POINT('',(10.8302042597752,-40.1925983403042,-13.1850308552911));
#75078=CARTESIAN_POINT('Origin',(-62.7155570771055,0.,0.));
#75079=CARTESIAN_POINT('',(10.8987117910442,-36.0428658633082,-12.3084785844451));
#75080=CARTESIAN_POINT('Origin',(10.9,-35.9648346973588,-12.291995980786));
#75081=CARTESIAN_POINT('',(11.6618634261911,-40.2693240660821,-12.9488045494888));
#75082=CARTESIAN_POINT('Origin',(26.9856656232739,0.,0.));
#75083=CARTESIAN_POINT('',(11.8995413080444,-36.0755342895717,-12.0118963235316));
#75084=CARTESIAN_POINT('Origin',(11.9,-36.0674407403565,-12.0100881945502));
#75085=CARTESIAN_POINT('',(12.3548486633046,-40.3880779943072,-12.5735100877104));
#75086=CARTESIAN_POINT('Origin',(20.8267261185512,0.,0.));
#75087=CARTESIAN_POINT('',(12.600317055424,-36.1988378309035,-11.6329963463162));
#75088=CARTESIAN_POINT('Origin',(12.6,-36.2042487976867,-11.6342111462358));
#75089=CARTESIAN_POINT('',(13.103292255208,-40.4610861730024,-12.3365516130268));
#75090=CARTESIAN_POINT('Origin',(25.13830739299,0.,0.));
#75091=CARTESIAN_POINT('',(13.2001612154348,-36.2656705509953,-11.4447884936362));
#75092=CARTESIAN_POINT('Origin',(13.2,-36.2726528263519,-11.4462726220787));
#75093=CARTESIAN_POINT('',(21.896707744792,-40.4610861730024,-12.3365516130268));
#75094=CARTESIAN_POINT('',(17.5,-40.4610861730024,-12.3365516130268));
#75095=CARTESIAN_POINT('',(21.7978078257374,-36.1777092848303,-11.4260917493401));
#75096=CARTESIAN_POINT('Origin',(21.8,-36.2726528263519,-11.4462726220787));
#75097=CARTESIAN_POINT('',(22.6451513366954,-40.3880779943072,-12.5735100877104));
#75098=CARTESIAN_POINT('Origin',(9.86169260701005,0.,0.));
#75099=CARTESIAN_POINT('',(22.3997512812625,-36.2000040861152,-11.633258178775));
#75100=CARTESIAN_POINT('Origin',(22.4,-36.2042487976867,-11.6342111462358));
#75101=CARTESIAN_POINT('',(23.3381365738089,-40.2693240660821,-12.9488045494888));
#75102=CARTESIAN_POINT('Origin',(14.1732738814488,0.,0.));
#75103=CARTESIAN_POINT('',(23.1003542130464,-36.0736907752397,-12.0114844755768));
#75104=CARTESIAN_POINT('Origin',(23.1,-36.0674407403565,-12.0100881945502));
#75105=CARTESIAN_POINT('',(24.1697957402248,-40.1925983403042,-13.1850308552911));
#75106=CARTESIAN_POINT('Origin',(8.01433437672608,0.,0.));
#75107=CARTESIAN_POINT('',(24.100209736014,-35.9775391158784,-12.2946795482123));
#75108=CARTESIAN_POINT('Origin',(24.1,-35.9648346973588,-12.291995980786));
#75109=CARTESIAN_POINT('',(29.9005519666592,-40.3023178069695,-12.8457455753269));
#75110=CARTESIAN_POINT('Origin',(97.7155570771054,0.,0.));
#75111=CARTESIAN_POINT('',(30.4426385593966,-36.5036071604488,-12.0050753064884));
#75112=CARTESIAN_POINT('Origin',(30.5,-36.101642754689,-11.9161189324716));
#75113=CARTESIAN_POINT('',(29.9040600247032,-40.4610861730024,-12.3365516130268));
#75114=CARTESIAN_POINT('Origin',(35.8405517186909,0.,0.));
#75115=CARTESIAN_POINT('',(30.5047502791291,-36.2392665318678,-11.4391761461162));
#75116=CARTESIAN_POINT('Origin',(30.5,-36.2726528263519,-11.4462726220787));
#75117=CARTESIAN_POINT('',(17.5,-40.4610861730024,-12.3365516130268));
#75118=CARTESIAN_POINT('Origin',(17.5,-40.1718595385976,-14.6213611271723));
#75119=CARTESIAN_POINT('Origin',(17.5,0.,0.));
#75120=CARTESIAN_POINT('',(0.600000000000001,-41.4083493394303,-8.63936369090331));
#75121=CARTESIAN_POINT('Origin',(0.600000000000001,0.,0.));
#75122=CARTESIAN_POINT('',(1.67735469196904,-41.2086042970448,-9.54677599452212));
#75123=CARTESIAN_POINT('Origin',(8.14497546096349,0.,0.));
#75124=CARTESIAN_POINT('',(5.09593997529677,-41.2086042970448,-9.54677599452212));
#75125=CARTESIAN_POINT('',(17.5,-41.2086042970448,-9.54677599452212));
#75126=CARTESIAN_POINT('',(5.09944803334083,-41.325703839893,-9.02641690470009));
#75127=CARTESIAN_POINT('Origin',(-0.840551718690872,0.,0.));
#75128=CARTESIAN_POINT('',(10.8302042597752,-41.4003266344532,-8.67772749978829));
#75129=CARTESIAN_POINT('Origin',(-62.7155570771055,0.,0.));
#75130=CARTESIAN_POINT('',(11.6618634261911,-41.3486599091995,-8.92066834454425));
#75131=CARTESIAN_POINT('Origin',(26.9856656232739,0.,0.));
#75132=CARTESIAN_POINT('',(12.3548486633046,-41.2638565969525,-9.3050598464565));
#75133=CARTESIAN_POINT('Origin',(20.8267261185512,0.,0.));
#75134=CARTESIAN_POINT('',(13.103292255208,-41.2086042970448,-9.54677599452212));
#75135=CARTESIAN_POINT('Origin',(25.13830739299,0.,0.));
#75136=CARTESIAN_POINT('',(21.896707744792,-41.2086042970448,-9.54677599452212));
#75137=CARTESIAN_POINT('',(17.5,-41.2086042970448,-9.54677599452212));
#75138=CARTESIAN_POINT('',(22.6451513366954,-41.2638565969525,-9.3050598464565));
#75139=CARTESIAN_POINT('Origin',(9.86169260701005,0.,0.));
#75140=CARTESIAN_POINT('',(23.3381365738089,-41.3486599091995,-8.92066834454425));
#75141=CARTESIAN_POINT('Origin',(14.1732738814488,0.,0.));
#75142=CARTESIAN_POINT('',(24.1697957402248,-41.4003266344532,-8.67772749978828));
#75143=CARTESIAN_POINT('Origin',(8.01433437672607,0.,0.));
#75144=CARTESIAN_POINT('',(29.9005519666592,-41.325703839893,-9.02641690470009));
#75145=CARTESIAN_POINT('Origin',(97.7155570771054,0.,0.));
#75146=CARTESIAN_POINT('',(29.9040600247032,-41.2086042970448,-9.54677599452212));
#75147=CARTESIAN_POINT('Origin',(35.8405517186909,0.,0.));
#75148=CARTESIAN_POINT('',(17.5,-41.2086042970448,-9.54677599452212));
#75149=CARTESIAN_POINT('Origin',(33.1,-37.1361751213135,-8.22356354381348));
#75150=CARTESIAN_POINT('',(30.5247014514712,-36.9673747121716,-8.16871696615112));
#75151=CARTESIAN_POINT('Origin',(30.5,-37.1361751213135,-8.22356354381348));
#75152=CARTESIAN_POINT('',(30.4955273645547,-37.253610541118,-7.74082391359483));
#75153=CARTESIAN_POINT('Origin',(30.5,-37.2229992101469,-7.73115966730738));
#75154=CARTESIAN_POINT('',(24.1012882089558,-37.3682767550424,-7.3619777955879));
#75155=CARTESIAN_POINT('Origin',(24.1,-37.2924584812137,-7.3372365661025));
#75156=CARTESIAN_POINT('',(23.1004586919557,-37.2482773116316,-7.63515978098255));
#75157=CARTESIAN_POINT('Origin',(23.1,-37.2403640279136,-7.63267889200616));
#75158=CARTESIAN_POINT('',(22.399682944576,-37.1656113221937,-8.02494855741036));
#75159=CARTESIAN_POINT('Origin',(22.4,-37.1709047568469,-8.02660199321104));
#75160=CARTESIAN_POINT('',(21.7998387845652,-37.1293862292573,-8.22135769906883));
#75161=CARTESIAN_POINT('Origin',(21.8,-37.1361751213135,-8.22356354381348));
#75162=CARTESIAN_POINT('',(13.2021921742626,-37.0438611660612,-8.19356892151486));
#75163=CARTESIAN_POINT('Origin',(13.2,-37.1361751213135,-8.22356354381348));
#75164=CARTESIAN_POINT('',(12.6002487187375,-37.1667522450638,-8.02530493145533));
#75165=CARTESIAN_POINT('Origin',(12.6,-37.1709047568469,-8.02660199321104));
#75166=CARTESIAN_POINT('',(11.8996457869536,-37.2464748574103,-7.63459469460788));
#75167=CARTESIAN_POINT('Origin',(11.9,-37.2403640279136,-7.63267889200616));
#75168=CARTESIAN_POINT('',(10.899790263986,-37.3048026141052,-7.34126473779836));
#75169=CARTESIAN_POINT('Origin',(10.9,-37.2924584812137,-7.3372365661025));
#75170=CARTESIAN_POINT('',(4.55736144060343,-37.6155887839604,-7.85510339046015));
#75171=CARTESIAN_POINT('Origin',(4.5,-37.2229992101469,-7.73115966730738));
#75172=CARTESIAN_POINT('',(4.49524972087093,-37.1037135041708,-8.21301612503226));
#75173=CARTESIAN_POINT('Origin',(4.5,-37.1361751213135,-8.22356354381348));
#75174=CARTESIAN_POINT('',(1.90350512467335,-37.0720625104951,-8.20273209378166));
#75175=CARTESIAN_POINT('Origin',(1.9,-37.1361751213135,-8.22356354381348));
#75176=CARTESIAN_POINT('Ctrl Pts',(0.138207714141624,-41.9261572390061,
-8.41238483838183));
#75177=CARTESIAN_POINT('Ctrl Pts',(0.370217470898825,-41.6665974739917,
-8.52664381638101));
#75178=CARTESIAN_POINT('Ctrl Pts',(0.600000000000005,-41.4083493394303,
-8.63936369090331));
#75179=CARTESIAN_POINT('Origin',(1.9,-37.7092141076143,-4.9736979588732));
#75180=CARTESIAN_POINT('',(5.09593997529677,-41.9886110647639,-5.1231377935775));
#75181=CARTESIAN_POINT('',(17.5,-41.9886110647639,-5.1231377935775));
#75182=CARTESIAN_POINT('',(4.47529854852883,-37.5318349744051,-4.96750374304975));
#75183=CARTESIAN_POINT('Origin',(4.5,-37.7092141076143,-4.9736979588732));
#75184=CARTESIAN_POINT('',(5.09944803334083,-41.9206753505941,-5.65216579287045));
#75185=CARTESIAN_POINT('Origin',(-0.840551718690874,0.,0.));
#75186=CARTESIAN_POINT('',(4.50447263544529,-37.6544606275072,-5.46749010626365));
#75187=CARTESIAN_POINT('Origin',(4.5,-37.6223900187809,-5.4661018353793));
#75188=CARTESIAN_POINT('',(10.8302042597752,-41.8715390397407,-6.00534915250317));
#75189=CARTESIAN_POINT('Origin',(-62.7155570771055,0.,0.));
#75190=CARTESIAN_POINT('',(10.8987117910442,-37.6326386190063,-5.86270716268918));
#75191=CARTESIAN_POINT('Origin',(10.9,-37.5529307477141,-5.86002493658419));
#75192=CARTESIAN_POINT('',(11.6618634261911,-41.9060788618227,-5.75938837262205));
#75193=CARTESIAN_POINT('Origin',(26.9856656232739,0.,0.));
#75194=CARTESIAN_POINT('',(11.8995413080444,-37.6133097693334,-5.5649578400478));
#75195=CARTESIAN_POINT('Origin',(11.9,-37.6050252010142,-5.56458261068052));
#75196=CARTESIAN_POINT('',(12.3548486633046,-41.9578594516632,-5.36917407377309));
#75197=CARTESIAN_POINT('Origin',(20.8267261185512,0.,0.));
#75198=CARTESIAN_POINT('',(12.600317055424,-37.6689447622493,-5.17040276961774));
#75199=CARTESIAN_POINT('Origin',(12.6,-37.674484472081,-5.17065950947564));
#75200=CARTESIAN_POINT('',(13.103292255208,-41.9886110647639,-5.1231377935775));
#75201=CARTESIAN_POINT('Origin',(25.13830739299,0.,0.));
#75202=CARTESIAN_POINT('',(13.2001612154348,-37.7020801925101,-4.97344883706827));
#75203=CARTESIAN_POINT('Origin',(13.2,-37.7092141076143,-4.9736979588732));
#75204=CARTESIAN_POINT('',(21.896707744792,-41.9886110647639,-5.1231377935775));
#75205=CARTESIAN_POINT('',(17.5,-41.9886110647639,-5.1231377935775));
#75206=CARTESIAN_POINT('',(21.7978078257374,-37.6122086000506,-4.97031045190414));
#75207=CARTESIAN_POINT('Origin',(21.8,-37.7092141076143,-4.9736979588732));
#75208=CARTESIAN_POINT('',(22.6451513366954,-41.9578594516632,-5.36917407377309));
#75209=CARTESIAN_POINT('Origin',(9.86169260701005,0.,0.));
#75210=CARTESIAN_POINT('',(22.3997512812625,-37.6701387661531,-5.17045810616097));
#75211=CARTESIAN_POINT('Origin',(22.4,-37.674484472081,-5.17065950947564));
#75212=CARTESIAN_POINT('',(23.3381365738089,-41.9060788618227,-5.75938837262206));
#75213=CARTESIAN_POINT('Origin',(14.1732738814488,0.,0.));
#75214=CARTESIAN_POINT('',(23.1003542130464,-37.6114227454796,-5.5648723718931));
#75215=CARTESIAN_POINT('Origin',(23.1,-37.6050252010142,-5.56458261068052));
#75216=CARTESIAN_POINT('',(24.1697957402248,-41.8715390397407,-6.00534915250317));
#75217=CARTESIAN_POINT('Origin',(8.01433437672608,0.,0.));
#75218=CARTESIAN_POINT('',(24.100209736014,-37.565908154163,-5.86046163546709));
#75219=CARTESIAN_POINT('Origin',(24.1,-37.5529307477141,-5.86002493658419));
#75220=CARTESIAN_POINT('',(29.9005519666592,-41.9206753505941,-5.65216579287045));
#75221=CARTESIAN_POINT('Origin',(97.7155570771054,0.,0.));
#75222=CARTESIAN_POINT('',(30.4426385593966,-38.0336947942479,-5.48390637564376));
#75223=CARTESIAN_POINT('Origin',(30.5,-37.6223900187809,-5.4661018353793));
#75224=CARTESIAN_POINT('',(29.9040600247032,-41.9886110647639,-5.1231377935775));
#75225=CARTESIAN_POINT('Origin',(35.8405517186909,0.,0.));
#75226=CARTESIAN_POINT('',(30.5047502791291,-37.6751027358433,-4.97250676352253));
#75227=CARTESIAN_POINT('Origin',(30.5,-37.7092141076143,-4.9736979588732));
#75228=CARTESIAN_POINT('',(17.5,-41.9886110647639,-5.1231377935775));
#75229=CARTESIAN_POINT('Origin',(17.5,-42.1005314412719,-7.42345959526126));
#75230=CARTESIAN_POINT('Origin',(17.5,0.,0.));
#75231=CARTESIAN_POINT('',(0.600000000000001,-42.2794732300362,-1.31762794090604));
#75232=CARTESIAN_POINT('Origin',(0.600000000000001,0.,0.));
#75233=CARTESIAN_POINT('',(1.67735469196904,-42.240333256585,-2.24593997529677));
#75234=CARTESIAN_POINT('Origin',(8.14497546096349,0.,0.));
#75235=CARTESIAN_POINT('',(5.09593997529677,-42.240333256585,-2.24593997529676));
#75236=CARTESIAN_POINT('',(17.5,-42.240333256585,-2.24593997529677));
#75237=CARTESIAN_POINT('',(5.09944803334083,-42.2652943865761,-1.71315218706844));
#75238=CARTESIAN_POINT('Origin',(-0.840551718690872,0.,0.));
#75239=CARTESIAN_POINT('',(10.8302042597752,-42.2782342134758,-1.35680204543027));
#75240=CARTESIAN_POINT('Origin',(-62.7155570771055,0.,0.));
#75241=CARTESIAN_POINT('',(11.6618634261911,-42.269538656846,-1.60502390555561));
#75242=CARTESIAN_POINT('Origin',(26.9856656232739,0.,0.));
#75243=CARTESIAN_POINT('',(12.3548486633046,-42.2527725812817,-1.99830157746261));
#75244=CARTESIAN_POINT('Origin',(20.8267261185512,0.,0.));
#75245=CARTESIAN_POINT('',(13.103292255208,-42.240333256585,-2.24593997529677));
#75246=CARTESIAN_POINT('Origin',(25.13830739299,0.,0.));
#75247=CARTESIAN_POINT('',(21.896707744792,-42.240333256585,-2.24593997529677));
#75248=CARTESIAN_POINT('',(17.5,-42.240333256585,-2.24593997529677));
#75249=CARTESIAN_POINT('',(22.6451513366954,-42.2527725812817,-1.99830157746261));
#75250=CARTESIAN_POINT('Origin',(9.86169260701005,0.,0.));
#75251=CARTESIAN_POINT('',(23.3381365738089,-42.269538656846,-1.6050239055556));
#75252=CARTESIAN_POINT('Origin',(14.1732738814488,0.,0.));
#75253=CARTESIAN_POINT('',(24.1697957402248,-42.2782342134758,-1.35680204543027));
#75254=CARTESIAN_POINT('Origin',(8.01433437672608,0.,0.));
#75255=CARTESIAN_POINT('',(29.9005519666592,-42.2652943865761,-1.71315218706844));
#75256=CARTESIAN_POINT('Origin',(97.7155570771054,0.,0.));
#75257=CARTESIAN_POINT('',(29.9040600247032,-42.240333256585,-2.24593997529677));
#75258=CARTESIAN_POINT('Origin',(35.8405517186909,0.,0.));
#75259=CARTESIAN_POINT('',(17.5,-42.240333256585,-2.24593997529677));
#75260=CARTESIAN_POINT('Origin',(33.1,-38.,-1.65));
#75261=CARTESIAN_POINT('',(30.5247014514712,-37.8242400401031,-1.62529854852883));
#75262=CARTESIAN_POINT('Origin',(30.5,-38.,-1.65));
#75263=CARTESIAN_POINT('',(30.4955273645547,-38.0318244548267,-1.15420182283181));
#75264=CARTESIAN_POINT('Origin',(30.5,-38.,-1.15));
#75265=CARTESIAN_POINT('',(24.1012882089558,-38.0789626932999,-0.761199649532067));
#75266=CARTESIAN_POINT('Origin',(24.1,-38.,-0.749999999999995));
#75267=CARTESIAN_POINT('',(23.1004586919557,-38.0082238650069,-1.05106907140133));
#75268=CARTESIAN_POINT('Origin',(23.1,-38.,-1.05));
#75269=CARTESIAN_POINT('',(22.399682944576,-37.9944998683999,-1.44929087888548));
#75270=CARTESIAN_POINT('Origin',(22.4,-38.,-1.45));
#75271=CARTESIAN_POINT('',(21.7998387845652,-37.9929312055486,-1.64900654572745));
#75272=CARTESIAN_POINT('Origin',(21.8,-38.,-1.65));
#75273=CARTESIAN_POINT('',(13.2021921742626,-37.9038799896544,-1.63649121351442));
#75274=CARTESIAN_POINT('Origin',(13.2,-38.,-1.65));
#75275=CARTESIAN_POINT('',(12.6002487187375,-37.9956853417913,-1.44944371963071));
#75276=CARTESIAN_POINT('Origin',(12.6,-38.,-1.45));
#75277=CARTESIAN_POINT('',(11.8996457869536,-38.0063506678963,-1.05082556284928));
#75278=CARTESIAN_POINT('Origin',(11.9,-38.,-1.05));
#75279=CARTESIAN_POINT('',(10.899790263986,-38.01285608245,-0.751823438535063));
#75280=CARTESIAN_POINT('Origin',(10.9,-38.,-0.749999999999995));
#75281=CARTESIAN_POINT('',(4.55736144060343,-38.408147857702,-1.2038882754343));
#75282=CARTESIAN_POINT('Origin',(4.5,-38.,-1.15));
#75283=CARTESIAN_POINT('',(4.49524972087093,-37.9662000077121,-1.64524972087092));
#75284=CARTESIAN_POINT('Origin',(4.5,-38.,-1.65));
#75285=CARTESIAN_POINT('',(1.90350512467335,-37.933244060464,-1.64061806453626));
#75286=CARTESIAN_POINT('Origin',(1.9,-38.,-1.65));
#75287=CARTESIAN_POINT('Ctrl Pts',(0.138207714141623,-42.75,-1.00418100903021));
#75288=CARTESIAN_POINT('Ctrl Pts',(0.370217470896624,-42.5142243943577,
-1.16177621660397));
#75289=CARTESIAN_POINT('Ctrl Pts',(0.600000000000005,-42.2794732300361,
-1.31762794090604));
#75290=CARTESIAN_POINT('Origin',(1.9,-38.,1.65));
#75291=CARTESIAN_POINT('',(5.09593997529677,-42.240333256585,2.24593997529678));
#75292=CARTESIAN_POINT('',(17.5,-42.240333256585,2.24593997529678));
#75293=CARTESIAN_POINT('',(4.47529854852883,-37.8242400401031,1.62529854852884));
#75294=CARTESIAN_POINT('Origin',(4.5,-38.,1.65));
#75295=CARTESIAN_POINT('',(5.09944803334083,-42.2652943865761,1.71315218706845));
#75296=CARTESIAN_POINT('Origin',(-0.840551718690874,0.,0.));
#75297=CARTESIAN_POINT('',(4.50447263544529,-38.0318244548267,1.15420182283182));
#75298=CARTESIAN_POINT('Origin',(4.5,-38.,1.15));
#75299=CARTESIAN_POINT('',(10.8302042597752,-42.2782342134758,1.35680204543028));
#75300=CARTESIAN_POINT('Origin',(-62.7155570771055,0.,0.));
#75301=CARTESIAN_POINT('',(10.8987117910442,-38.0789626932999,0.761199649532077));
#75302=CARTESIAN_POINT('Origin',(10.9,-38.,0.750000000000005));
#75303=CARTESIAN_POINT('',(11.6618634261911,-42.269538656846,1.60502390555562));
#75304=CARTESIAN_POINT('Origin',(26.9856656232739,0.,0.));
#75305=CARTESIAN_POINT('',(11.8995413080444,-38.0082238650069,1.05106907140134));
#75306=CARTESIAN_POINT('Origin',(11.9,-38.,1.05));
#75307=CARTESIAN_POINT('',(12.3548486633046,-42.2527725812817,1.99830157746262));
#75308=CARTESIAN_POINT('Origin',(20.8267261185512,0.,0.));
#75309=CARTESIAN_POINT('',(12.600317055424,-37.9944998683999,1.44929087888549));
#75310=CARTESIAN_POINT('Origin',(12.6,-38.,1.45));
#75311=CARTESIAN_POINT('',(13.103292255208,-42.240333256585,2.24593997529678));
#75312=CARTESIAN_POINT('Origin',(25.13830739299,0.,0.));
#75313=CARTESIAN_POINT('',(13.2001612154348,-37.9929312055486,1.64900654572746));
#75314=CARTESIAN_POINT('Origin',(13.2,-38.,1.65));
#75315=CARTESIAN_POINT('',(21.896707744792,-42.240333256585,2.24593997529678));
#75316=CARTESIAN_POINT('',(17.5,-42.240333256585,2.24593997529678));
#75317=CARTESIAN_POINT('',(21.7978078257374,-37.9038799896544,1.63649121351443));
#75318=CARTESIAN_POINT('Origin',(21.8,-38.,1.65));
#75319=CARTESIAN_POINT('',(22.6451513366954,-42.2527725812817,1.99830157746262));
#75320=CARTESIAN_POINT('Origin',(9.86169260701005,0.,0.));
#75321=CARTESIAN_POINT('',(22.3997512812625,-37.9956853417913,1.44944371963072));
#75322=CARTESIAN_POINT('Origin',(22.4,-38.,1.45));
#75323=CARTESIAN_POINT('',(23.3381365738089,-42.269538656846,1.60502390555561));
#75324=CARTESIAN_POINT('Origin',(14.1732738814488,0.,0.));
#75325=CARTESIAN_POINT('',(23.1003542130464,-38.0063506678963,1.05082556284929));
#75326=CARTESIAN_POINT('Origin',(23.1,-38.,1.05));
#75327=CARTESIAN_POINT('',(24.1697957402248,-42.2782342134758,1.35680204543028));
#75328=CARTESIAN_POINT('Origin',(8.01433437672608,0.,0.));
#75329=CARTESIAN_POINT('',(24.100209736014,-38.01285608245,0.751823438535072));
#75330=CARTESIAN_POINT('Origin',(24.1,-38.,0.750000000000005));
#75331=CARTESIAN_POINT('',(29.9005519666592,-42.2652943865761,1.71315218706845));
#75332=CARTESIAN_POINT('Origin',(97.7155570771054,0.,0.));
#75333=CARTESIAN_POINT('',(30.4426385593966,-38.408147857702,1.20388827543431));
#75334=CARTESIAN_POINT('Origin',(30.5,-38.,1.15));
#75335=CARTESIAN_POINT('',(29.9040600247032,-42.240333256585,2.24593997529678));
#75336=CARTESIAN_POINT('Origin',(35.8405517186909,0.,0.));
#75337=CARTESIAN_POINT('',(30.5047502791291,-37.9662000077121,1.64524972087093));
#75338=CARTESIAN_POINT('Origin',(30.5,-38.,1.65));
#75339=CARTESIAN_POINT('',(17.5,-42.240333256585,2.24593997529678));
#75340=CARTESIAN_POINT('Origin',(17.5,-42.75,5.23536506635493E-15));
#75341=CARTESIAN_POINT('Origin',(17.5,0.,0.));
#75342=CARTESIAN_POINT('',(0.600000000000001,-41.8659567209931,6.04414326732378));
#75343=CARTESIAN_POINT('Origin',(0.600000000000001,0.,0.));
#75344=CARTESIAN_POINT('',(1.67735469196905,-41.9886110647639,5.12313779357753));
#75345=CARTESIAN_POINT('Origin',(8.14497546096349,0.,0.));
#75346=CARTESIAN_POINT('',(5.09593997529677,-41.9886110647639,5.12313779357753));
#75347=CARTESIAN_POINT('',(17.5,-41.9886110647639,5.12313779357753));
#75348=CARTESIAN_POINT('',(5.09944803334083,-41.9206753505941,5.65216579287047));
#75349=CARTESIAN_POINT('Origin',(-0.840551718690872,0.,0.));
#75350=CARTESIAN_POINT('',(10.8302042597752,-41.8715390397407,6.0053491525032));
#75351=CARTESIAN_POINT('Origin',(-62.7155570771055,0.,0.));
#75352=CARTESIAN_POINT('',(11.6618634261911,-41.9060788618227,5.75938837262208));
#75353=CARTESIAN_POINT('Origin',(26.9856656232739,0.,0.));
#75354=CARTESIAN_POINT('',(12.3548486633046,-41.9578594516632,5.36917407377311));
#75355=CARTESIAN_POINT('Origin',(20.8267261185512,0.,0.));
#75356=CARTESIAN_POINT('',(13.103292255208,-41.9886110647639,5.12313779357753));
#75357=CARTESIAN_POINT('Origin',(25.13830739299,0.,0.));
#75358=CARTESIAN_POINT('',(21.896707744792,-41.9886110647639,5.12313779357753));
#75359=CARTESIAN_POINT('',(17.5,-41.9886110647639,5.12313779357753));
#75360=CARTESIAN_POINT('',(22.6451513366954,-41.9578594516632,5.36917407377311));
#75361=CARTESIAN_POINT('Origin',(9.86169260701006,0.,0.));
#75362=CARTESIAN_POINT('',(23.3381365738089,-41.9060788618227,5.75938837262209));
#75363=CARTESIAN_POINT('Origin',(14.1732738814488,0.,0.));
#75364=CARTESIAN_POINT('',(24.1697957402248,-41.8715390397407,6.0053491525032));
#75365=CARTESIAN_POINT('Origin',(8.01433437672608,0.,0.));
#75366=CARTESIAN_POINT('',(29.9005519666592,-41.9206753505941,5.65216579287048));
#75367=CARTESIAN_POINT('Origin',(97.7155570771054,0.,0.));
#75368=CARTESIAN_POINT('',(29.9040600247032,-41.9886110647639,5.12313779357753));
#75369=CARTESIAN_POINT('Origin',(35.8405517186909,0.,0.));
#75370=CARTESIAN_POINT('',(17.5,-41.9886110647639,5.12313779357753));
#75371=CARTESIAN_POINT('Origin',(33.1,-37.7092141076143,4.97369795887322));
#75372=CARTESIAN_POINT('',(30.5247014514712,-37.5318349744051,4.96750374304978));
#75373=CARTESIAN_POINT('Origin',(30.5,-37.7092141076143,4.97369795887322));
#75374=CARTESIAN_POINT('',(30.4955273645547,-37.6544606275072,5.46749010626367));
#75375=CARTESIAN_POINT('Origin',(30.5,-37.6223900187809,5.46610183537933));
#75376=CARTESIAN_POINT('',(24.1012882089558,-37.6326386190063,5.8627071626892));
#75377=CARTESIAN_POINT('Origin',(24.1,-37.5529307477141,5.86002493658421));
#75378=CARTESIAN_POINT('',(23.1004586919557,-37.6133097693334,5.56495784004783));
#75379=CARTESIAN_POINT('Origin',(23.1,-37.6050252010142,5.56458261068055));
#75380=CARTESIAN_POINT('',(22.399682944576,-37.6689447622493,5.17040276961777));
#75381=CARTESIAN_POINT('Origin',(22.4,-37.674484472081,5.17065950947566));
#75382=CARTESIAN_POINT('',(21.7998387845652,-37.7020801925101,4.97344883706829));
#75383=CARTESIAN_POINT('Origin',(21.8,-37.7092141076143,4.97369795887322));
#75384=CARTESIAN_POINT('',(13.2021921742626,-37.6122086000506,4.97031045190416));
#75385=CARTESIAN_POINT('Origin',(13.2,-37.7092141076143,4.97369795887322));
#75386=CARTESIAN_POINT('',(12.6002487187375,-37.6701387661531,5.170458106161));
#75387=CARTESIAN_POINT('Origin',(12.6,-37.674484472081,5.17065950947566));
#75388=CARTESIAN_POINT('',(11.8996457869536,-37.6114227454796,5.56487237189313));
#75389=CARTESIAN_POINT('Origin',(11.9,-37.6050252010142,5.56458261068055));
#75390=CARTESIAN_POINT('',(10.899790263986,-37.565908154163,5.86046163546712));
#75391=CARTESIAN_POINT('Origin',(10.9,-37.5529307477141,5.86002493658421));
#75392=CARTESIAN_POINT('',(4.55736144060343,-38.0336947942479,5.48390637564379));
#75393=CARTESIAN_POINT('Origin',(4.5,-37.6223900187809,5.46610183537933));
#75394=CARTESIAN_POINT('',(4.49524972087093,-37.6751027358433,4.97250676352256));
#75395=CARTESIAN_POINT('Origin',(4.5,-37.7092141076143,4.97369795887322));
#75396=CARTESIAN_POINT('',(1.90350512467335,-37.6418431848034,4.9713453144073));
#75397=CARTESIAN_POINT('Origin',(1.9,-37.7092141076143,4.97369795887322));
#75398=CARTESIAN_POINT('Ctrl Pts',(0.138207714141624,-42.2749056435377,
6.43453435214071));
#75399=CARTESIAN_POINT('Ctrl Pts',(0.370217470893479,-42.070078119737,6.23839136562906));
#75400=CARTESIAN_POINT('Ctrl Pts',(0.600000000000005,-41.8659567209931,
6.04414326732377));
#75401=CARTESIAN_POINT('Origin',(1.9,-37.1361751213135,8.22356354381351));
#75402=CARTESIAN_POINT('',(5.09593997529677,-41.2086042970448,9.54677599452214));
#75403=CARTESIAN_POINT('',(17.5,-41.2086042970448,9.54677599452214));
#75404=CARTESIAN_POINT('',(4.47529854852883,-36.9673747121716,8.16871696615114));
#75405=CARTESIAN_POINT('Origin',(4.5,-37.1361751213135,8.22356354381351));
#75406=CARTESIAN_POINT('',(5.09944803334083,-41.325703839893,9.02641690470012));
#75407=CARTESIAN_POINT('Origin',(-0.840551718690874,0.,0.));
#75408=CARTESIAN_POINT('',(4.50447263544529,-37.253610541118,7.74082391359486));
#75409=CARTESIAN_POINT('Origin',(4.5,-37.2229992101469,7.73115966730741));
#75410=CARTESIAN_POINT('',(10.8302042597752,-41.4003266344532,8.67772749978831));
#75411=CARTESIAN_POINT('Origin',(-62.7155570771054,0.,0.));
#75412=CARTESIAN_POINT('',(10.8987117910442,-37.3682767550424,7.36197779558792));
#75413=CARTESIAN_POINT('Origin',(10.9,-37.2924584812137,7.33723656610252));
#75414=CARTESIAN_POINT('',(11.6618634261911,-41.3486599091995,8.92066834454429));
#75415=CARTESIAN_POINT('Origin',(26.9856656232739,0.,0.));
#75416=CARTESIAN_POINT('',(11.8995413080444,-37.2482773116316,7.63515978098258));
#75417=CARTESIAN_POINT('Origin',(11.9,-37.2403640279136,7.63267889200618));
#75418=CARTESIAN_POINT('',(12.3548486633046,-41.2638565969525,9.30505984645653));
#75419=CARTESIAN_POINT('Origin',(20.8267261185512,0.,0.));
#75420=CARTESIAN_POINT('',(12.600317055424,-37.1656113221937,8.02494855741038));
#75421=CARTESIAN_POINT('Origin',(12.6,-37.1709047568469,8.02660199321107));
#75422=CARTESIAN_POINT('',(13.103292255208,-41.2086042970448,9.54677599452214));
#75423=CARTESIAN_POINT('Origin',(25.13830739299,0.,0.));
#75424=CARTESIAN_POINT('',(13.2001612154348,-37.1293862292573,8.22135769906885));
#75425=CARTESIAN_POINT('Origin',(13.2,-37.1361751213135,8.22356354381351));
#75426=CARTESIAN_POINT('',(21.896707744792,-41.2086042970448,9.54677599452214));
#75427=CARTESIAN_POINT('',(17.5,-41.2086042970448,9.54677599452214));
#75428=CARTESIAN_POINT('',(21.7978078257374,-37.0438611660612,8.19356892151488));
#75429=CARTESIAN_POINT('Origin',(21.8,-37.1361751213135,8.22356354381351));
#75430=CARTESIAN_POINT('',(22.6451513366954,-41.2638565969525,9.30505984645653));
#75431=CARTESIAN_POINT('Origin',(9.86169260701005,0.,0.));
#75432=CARTESIAN_POINT('',(22.3997512812625,-37.1667522450638,8.02530493145535));
#75433=CARTESIAN_POINT('Origin',(22.4,-37.1709047568469,8.02660199321107));
#75434=CARTESIAN_POINT('',(23.3381365738089,-41.3486599091995,8.92066834454428));
#75435=CARTESIAN_POINT('Origin',(14.1732738814488,0.,0.));
#75436=CARTESIAN_POINT('',(23.1003542130464,-37.2464748574103,7.63459469460791));
#75437=CARTESIAN_POINT('Origin',(23.1,-37.2403640279136,7.63267889200618));
#75438=CARTESIAN_POINT('',(24.1697957402248,-41.4003266344532,8.67772749978831));
#75439=CARTESIAN_POINT('Origin',(8.01433437672608,0.,0.));
#75440=CARTESIAN_POINT('',(24.100209736014,-37.3048026141052,7.34126473779838));
#75441=CARTESIAN_POINT('Origin',(24.1,-37.2924584812137,7.33723656610252));
#75442=CARTESIAN_POINT('',(29.9005519666592,-41.325703839893,9.02641690470012));
#75443=CARTESIAN_POINT('Origin',(97.7155570771055,0.,0.));
#75444=CARTESIAN_POINT('',(30.4426385593966,-37.6155887839604,7.85510339046018));
#75445=CARTESIAN_POINT('Origin',(30.5,-37.2229992101469,7.73115966730741));
#75446=CARTESIAN_POINT('',(29.9040600247032,-41.2086042970448,9.54677599452215));
#75447=CARTESIAN_POINT('Origin',(35.8405517186909,0.,0.));
#75448=CARTESIAN_POINT('',(30.5047502791291,-37.1037135041708,8.21301612503228));
#75449=CARTESIAN_POINT('Origin',(30.5,-37.1361751213135,8.22356354381351));
#75450=CARTESIAN_POINT('',(17.5,-41.2086042970448,9.54677599452214));
#75451=CARTESIAN_POINT('Origin',(17.5,-42.1005314412719,7.42345959526129));
#75452=CARTESIAN_POINT('Origin',(17.5,0.,0.));
#75453=CARTESIAN_POINT('',(0.600000000000001,-40.1803643021789,13.22226624086));
#75454=CARTESIAN_POINT('Origin',(0.600000000000001,0.,0.));
#75455=CARTESIAN_POINT('',(1.67735469196905,-40.4610861730024,12.3365516130268));
#75456=CARTESIAN_POINT('Origin',(8.14497546096349,0.,0.));
#75457=CARTESIAN_POINT('',(5.09593997529677,-40.4610861730024,12.3365516130268));
#75458=CARTESIAN_POINT('',(17.5,-40.4610861730024,12.3365516130268));
#75459=CARTESIAN_POINT('',(5.09944803334083,-40.3023178069695,12.8457455753269));
#75460=CARTESIAN_POINT('Origin',(-0.840551718690872,0.,0.));
#75461=CARTESIAN_POINT('',(10.8302042597752,-40.1925983403042,13.1850308552911));
#75462=CARTESIAN_POINT('Origin',(-62.7155570771054,0.,0.));
#75463=CARTESIAN_POINT('',(11.6618634261911,-40.2693240660821,12.9488045494888));
#75464=CARTESIAN_POINT('Origin',(26.9856656232739,0.,0.));
#75465=CARTESIAN_POINT('',(12.3548486633046,-40.3880779943072,12.5735100877104));
#75466=CARTESIAN_POINT('Origin',(20.8267261185512,0.,0.));
#75467=CARTESIAN_POINT('',(13.103292255208,-40.4610861730024,12.3365516130268));
#75468=CARTESIAN_POINT('Origin',(25.13830739299,0.,0.));
#75469=CARTESIAN_POINT('',(21.896707744792,-40.4610861730024,12.3365516130268));
#75470=CARTESIAN_POINT('',(17.5,-40.4610861730024,12.3365516130268));
#75471=CARTESIAN_POINT('',(22.6451513366954,-40.3880779943072,12.5735100877104));
#75472=CARTESIAN_POINT('Origin',(9.86169260701006,0.,0.));
#75473=CARTESIAN_POINT('',(23.3381365738089,-40.2693240660821,12.9488045494888));
#75474=CARTESIAN_POINT('Origin',(14.1732738814488,0.,0.));
#75475=CARTESIAN_POINT('',(24.1697957402248,-40.1925983403042,13.1850308552911));
#75476=CARTESIAN_POINT('Origin',(8.01433437672608,0.,0.));
#75477=CARTESIAN_POINT('',(29.9005519666592,-40.3023178069695,12.8457455753269));
#75478=CARTESIAN_POINT('Origin',(97.7155570771054,0.,0.));
#75479=CARTESIAN_POINT('',(29.9040600247032,-40.4610861730024,12.3365516130268));
#75480=CARTESIAN_POINT('Origin',(35.8405517186909,0.,0.));
#75481=CARTESIAN_POINT('',(17.5,-40.4610861730024,12.3365516130268));
#75482=CARTESIAN_POINT('Origin',(33.1,-36.2726528263519,11.4462726220787));
#75483=CARTESIAN_POINT('',(30.5247014514712,-36.0990440950346,11.409370947074));
#75484=CARTESIAN_POINT('Origin',(30.5,-36.2726528263519,11.4462726220787));
#75485=CARTESIAN_POINT('',(30.4955273645547,-36.1329850680974,11.9230551151638));
#75486=CARTESIAN_POINT('Origin',(30.5,-36.101642754689,11.9161189324716));
#75487=CARTESIAN_POINT('',(24.1012882089558,-36.0428658633082,12.3084785844451));
#75488=CARTESIAN_POINT('Origin',(24.1,-35.9648346973588,12.291995980786));
#75489=CARTESIAN_POINT('',(23.1004586919557,-36.0755342895717,12.0118963235317));
#75490=CARTESIAN_POINT('Origin',(23.1,-36.0674407403565,12.0100881945502));
#75491=CARTESIAN_POINT('',(22.399682944576,-36.1988378309035,11.6329963463162));
#75492=CARTESIAN_POINT('Origin',(22.4,-36.2042487976867,11.6342111462359));
#75493=CARTESIAN_POINT('',(21.7998387845652,-36.2656705509953,11.4447884936363));
#75494=CARTESIAN_POINT('Origin',(21.8,-36.2726528263519,11.4462726220787));
#75495=CARTESIAN_POINT('',(13.2021921742626,-36.1777092848303,11.4260917493401));
#75496=CARTESIAN_POINT('Origin',(13.2,-36.2726528263519,11.4462726220787));
#75497=CARTESIAN_POINT('',(12.6002487187375,-36.2000040861152,11.633258178775));
#75498=CARTESIAN_POINT('Origin',(12.6,-36.2042487976867,11.6342111462359));
#75499=CARTESIAN_POINT('',(11.8996457869536,-36.0736907752397,12.0114844755768));
#75500=CARTESIAN_POINT('Origin',(11.9,-36.0674407403565,12.0100881945502));
#75501=CARTESIAN_POINT('',(10.899790263986,-35.9775391158784,12.2946795482123));
#75502=CARTESIAN_POINT('Origin',(10.9,-35.9648346973588,12.291995980786));
#75503=CARTESIAN_POINT('',(4.55736144060343,-36.5036071604488,12.0050753064884));
#75504=CARTESIAN_POINT('Origin',(4.5,-36.101642754689,11.9161189324716));
#75505=CARTESIAN_POINT('',(4.49524972087093,-36.2392665318678,11.4391761461162));
#75506=CARTESIAN_POINT('Origin',(4.5,-36.2726528263519,11.4462726220787));
#75507=CARTESIAN_POINT('',(1.90350512467335,-36.2067139516643,11.4322568815947));
#75508=CARTESIAN_POINT('Origin',(1.9,-36.2726528263519,11.4462726220787));
#75509=CARTESIAN_POINT('Ctrl Pts',(0.138207714141621,-40.515309671231,13.6777396430533));
#75510=CARTESIAN_POINT('Ctrl Pts',(0.370217470899141,-40.3476538099276,
13.4490085829881));
#75511=CARTESIAN_POINT('Ctrl Pts',(0.600000000000005,-40.1803643021789,
13.22226624086));
#75512=CARTESIAN_POINT('Origin',(1.9,-35.1439863533772,14.5472582706722));
#75513=CARTESIAN_POINT('',(5.09593997529677,-38.9247727484987,16.5575380560557));
#75514=CARTESIAN_POINT('',(17.5,-38.9247727484987,16.5575380560557));
#75515=CARTESIAN_POINT('',(4.47529854852883,-34.987274410005,14.4639330523272));
#75516=CARTESIAN_POINT('Origin',(4.5,-35.1439863533772,14.5472582706722));
#75517=CARTESIAN_POINT('',(5.09944803334083,-39.1304526938498,16.0654185122698));
#75518=CARTESIAN_POINT('Origin',(-0.840551718690874,0.,0.));
#75519=CARTESIAN_POINT('',(4.50447263544529,-35.343464522354,14.0922449867892));
#75520=CARTESIAN_POINT('Origin',(4.5,-35.31499642504,14.0774119602792));
#75521=CARTESIAN_POINT('',(10.8302042597752,-39.2644910802189,15.7349845952072));
#75522=CARTESIAN_POINT('Origin',(-62.7155570771055,0.,0.));
#75523=CARTESIAN_POINT('',(10.8987117910442,-35.5221746368434,13.7390659716653));
#75524=CARTESIAN_POINT('Origin',(10.9,-35.4518044823703,13.7015349119648));
#75525=CARTESIAN_POINT('',(11.6618634261911,-39.1714230536436,15.9652627899599));
#75526=CARTESIAN_POINT('Origin',(26.9856656232739,0.,0.));
#75527=CARTESIAN_POINT('',(11.8995413080444,-35.35656070068,13.9872600241959));
#75528=CARTESIAN_POINT('Origin',(11.9,-35.3491984393726,13.9834426982006));
#75529=CARTESIAN_POINT('',(12.3548486633046,-39.0211592104439,16.3290885806033));
#75530=CARTESIAN_POINT('Origin',(20.8267261185512,0.,0.));
#75531=CARTESIAN_POINT('',(12.600317055424,-35.2074644826695,14.3567722348383));
#75532=CARTESIAN_POINT('Origin',(12.6,-35.2123903820423,14.359319746515));
#75533=CARTESIAN_POINT('',(13.103292255208,-38.9247727484987,16.5575380560557));
#75534=CARTESIAN_POINT('Origin',(25.13830739299,0.,0.));
#75535=CARTESIAN_POINT('',(13.2001612154348,-35.137683640766,14.5439070589318));
#75536=CARTESIAN_POINT('Origin',(13.2,-35.1439863533772,14.5472582706722));
#75537=CARTESIAN_POINT('',(21.896707744792,-38.9247727484987,16.5575380560557));
#75538=CARTESIAN_POINT('',(17.5,-38.9247727484987,16.5575380560557));
#75539=CARTESIAN_POINT('',(21.7978078257374,-35.0582833660355,14.501689183981));
#75540=CARTESIAN_POINT('Origin',(21.8,-35.1439863533772,14.5472582706722));
#75541=CARTESIAN_POINT('',(22.6451513366954,-39.0211592104439,16.3290885806033));
#75542=CARTESIAN_POINT('Origin',(9.86169260701005,0.,0.));
#75543=CARTESIAN_POINT('',(22.3997512812625,-35.208526188654,14.3573213139379));
#75544=CARTESIAN_POINT('Origin',(22.4,-35.2123903820423,14.359319746515));
#75545=CARTESIAN_POINT('',(23.3381365738089,-39.1714230536436,15.9652627899599));
#75546=CARTESIAN_POINT('Origin',(14.1732738814488,0.,0.));
#75547=CARTESIAN_POINT('',(23.1003542130464,-35.3548837560077,13.9863905298622));
#75548=CARTESIAN_POINT('Origin',(23.1,-35.3491984393726,13.9834426982006));
#75549=CARTESIAN_POINT('',(24.1697957402248,-39.2644910802189,15.7349845952072));
#75550=CARTESIAN_POINT('Origin',(8.01433437672607,0.,0.));
#75551=CARTESIAN_POINT('',(24.100209736014,-35.4632615954717,13.7076454228629));
#75552=CARTESIAN_POINT('Origin',(24.1,-35.4518044823703,13.7015349119648));
#75553=CARTESIAN_POINT('',(29.9005519666592,-39.1304526938498,16.0654185122698));
#75554=CARTESIAN_POINT('Origin',(97.7155570771054,0.,0.));
#75555=CARTESIAN_POINT('',(30.4426385593966,-35.6800990794245,14.267645163841));
#75556=CARTESIAN_POINT('Origin',(30.5,-35.31499642504,14.0774119602792));
#75557=CARTESIAN_POINT('',(29.9040600247032,-38.9247727484987,16.5575380560557));
#75558=CARTESIAN_POINT('Origin',(35.8405517186909,0.,0.));
#75559=CARTESIAN_POINT('',(30.5047502791291,-35.1138494411902,14.5312341902212));
#75560=CARTESIAN_POINT('Origin',(30.5,-35.1439863533772,14.5472582706722));
#75561=CARTESIAN_POINT('',(17.5,-38.9247727484987,16.5575380560557));
#75562=CARTESIAN_POINT('Origin',(17.5,-40.1718595385976,14.6213611271723));
#75563=CARTESIAN_POINT('Origin',(17.5,0.,0.));
#75564=CARTESIAN_POINT('',(0.600000000000001,-37.2739118462884,19.9986373454573));
#75565=CARTESIAN_POINT('Origin',(0.600000000000001,0.,0.));
#75566=CARTESIAN_POINT('',(1.67735469196905,-37.7041716521717,19.1751255543105));
#75567=CARTESIAN_POINT('Origin',(8.14497546096349,0.,0.));
#75568=CARTESIAN_POINT('',(5.09593997529677,-37.7041716521717,19.1751255543105));
#75569=CARTESIAN_POINT('',(17.5,-37.7041716521717,19.1751255543105));
#75570=CARTESIAN_POINT('',(5.09944803334083,-37.459394730737,19.6490138787379));
#75571=CARTESIAN_POINT('Origin',(-0.840551718690874,0.,0.));
#75572=CARTESIAN_POINT('',(10.8302042597752,-37.2924258787336,19.9640920674886));
#75573=CARTESIAN_POINT('Origin',(-62.7155570771055,0.,0.));
#75574=CARTESIAN_POINT('',(11.6618634261911,-37.4090062358548,19.7447778525305));
#75575=CARTESIAN_POINT('Origin',(26.9856656232739,0.,0.));
#75576=CARTESIAN_POINT('',(12.3548486633046,-37.5911252244478,19.3958063601357));
#75577=CARTESIAN_POINT('Origin',(20.8267261185512,0.,0.));
#75578=CARTESIAN_POINT('',(13.103292255208,-37.7041716521717,19.1751255543105));
#75579=CARTESIAN_POINT('Origin',(25.13830739299,0.,0.));
#75580=CARTESIAN_POINT('',(21.896707744792,-37.7041716521717,19.1751255543105));
#75581=CARTESIAN_POINT('',(17.5,-37.7041716521717,19.1751255543105));
#75582=CARTESIAN_POINT('',(22.6451513366954,-37.5911252244478,19.3958063601357));
#75583=CARTESIAN_POINT('Origin',(9.86169260701006,0.,0.));
#75584=CARTESIAN_POINT('',(23.3381365738089,-37.4090062358548,19.7447778525305));
#75585=CARTESIAN_POINT('Origin',(14.1732738814488,0.,0.));
#75586=CARTESIAN_POINT('',(24.1697957402248,-37.2924258787336,19.9640920674886));
#75587=CARTESIAN_POINT('Origin',(8.01433437672608,0.,0.));
#75588=CARTESIAN_POINT('',(29.9005519666592,-37.459394730737,19.6490138787379));
#75589=CARTESIAN_POINT('Origin',(97.7155570771054,0.,0.));
#75590=CARTESIAN_POINT('',(29.9040600247032,-37.7041716521717,19.1751255543105));
#75591=CARTESIAN_POINT('Origin',(35.8405517186909,0.,0.));
#75592=CARTESIAN_POINT('',(17.5,-37.7041716521717,19.1751255543105));
#75593=CARTESIAN_POINT('Origin',(33.1,-33.7339653438087,17.5710580837557));
#75594=CARTESIAN_POINT('',(30.5247014514712,-33.5694020278343,17.5045701882916));
#75595=CARTESIAN_POINT('Origin',(30.5,-33.7339653438087,17.5710580837557));
#75596=CARTESIAN_POINT('',(30.4955273645547,-33.5136270415661,18.0163441277467));
#75597=CARTESIAN_POINT('Origin',(30.5,-33.4839653438087,18.0040707856479));
#75598=CARTESIAN_POINT('',(24.1012882089558,-33.3579488669236,18.3802631128033));
#75599=CARTESIAN_POINT('Origin',(24.1,-33.2839653438087,18.3504809471617));
#75600=CARTESIAN_POINT('',(23.1004586919557,-33.4416219555226,18.0938594155378));
#75601=CARTESIAN_POINT('Origin',(23.1,-33.4339653438087,18.0906733260263));
#75602=CARTESIAN_POINT('',(22.399682944576,-33.6288475295615,17.742127215612));
#75603=CARTESIAN_POINT('Origin',(22.4,-33.6339653438087,17.7442631645126));
#75604=CARTESIAN_POINT('',(21.7998387845652,-33.7273468611033,17.5683840431675));
#75605=CARTESIAN_POINT('Origin',(21.8,-33.7339653438087,17.5710580837557));
#75606=CARTESIAN_POINT('',(13.2021921742626,-33.6439685797946,17.5346970308537));
#75607=CARTESIAN_POINT('Origin',(13.2,-33.7339653438087,17.5710580837557));
#75608=CARTESIAN_POINT('',(12.6002487187375,-33.6299506000067,17.7425875883397));
#75609=CARTESIAN_POINT('Origin',(12.6,-33.6339653438087,17.7442631645126));
#75610=CARTESIAN_POINT('',(11.8996457869536,-33.4398779649625,18.0931337015746));
#75611=CARTESIAN_POINT('Origin',(11.9,-33.4339653438087,18.0906733260263));
#75612=CARTESIAN_POINT('',(10.899790263986,-33.2960107570711,18.3553298442931));
#75613=CARTESIAN_POINT('Origin',(10.9,-33.2839653438087,18.3504809471617));
#75614=CARTESIAN_POINT('',(4.55736144060343,-33.864375894796,18.1614760990067));
#75615=CARTESIAN_POINT('Origin',(4.5,-33.4839653438087,18.0040707856479));
#75616=CARTESIAN_POINT('',(4.49524972087093,-33.7023185522751,17.5582719500126));
#75617=CARTESIAN_POINT('Origin',(4.5,-33.7339653438087,17.5710580837557));
#75618=CARTESIAN_POINT('',(1.90350512467335,-33.6714620365851,17.5458051084359));
#75619=CARTESIAN_POINT('Origin',(1.9,-33.7339653438087,17.5710580837557));
#75620=CARTESIAN_POINT('Ctrl Pts',(0.138207714141623,-37.5246765162999,
20.5053537361819));
#75621=CARTESIAN_POINT('Ctrl Pts',(0.370217470897676,-37.3992864560072,
20.2509844800861));
#75622=CARTESIAN_POINT('Ctrl Pts',(0.600000000000005,-37.2739118462884,
19.9986373454573));
#75623=CARTESIAN_POINT('Origin',(1.9,-32.0839653438087,20.4289419162443));
#75624=CARTESIAN_POINT('',(5.09593997529677,-35.4582316768749,23.0652077022745));
#75625=CARTESIAN_POINT('',(17.5,-35.4582316768749,23.0652077022745));
#75626=CARTESIAN_POINT('',(4.47529854852883,-31.9441034793054,20.3196698518115));
#75627=CARTESIAN_POINT('Origin',(4.5,-32.0839653438087,20.4289419162443));
#75628=CARTESIAN_POINT('',(5.09944803334083,-35.7462425436685,22.6162805078382));
#75629=CARTESIAN_POINT('Origin',(-0.840551718690874,0.,0.));
#75630=CARTESIAN_POINT('',(4.50447263544529,-32.3594252187343,20.01548032708));
#75631=CARTESIAN_POINT('Origin',(4.5,-32.3339653438087,19.9959292143521));
#75632=CARTESIAN_POINT('',(10.8302042597752,-35.9356238333033,22.3141421459872));
#75633=CARTESIAN_POINT('Origin',(-62.7155570771055,0.,0.));
#75634=CARTESIAN_POINT('',(10.8987117910442,-32.5967492173916,19.6986995804965));
#75635=CARTESIAN_POINT('Origin',(10.9,-32.5339653438087,19.6495190528383));
#75636=CARTESIAN_POINT('',(11.6618634261911,-35.8039823302991,22.5247608043155));
#75637=CARTESIAN_POINT('Origin',(26.9856656232739,0.,0.));
#75638=CARTESIAN_POINT('',(11.8995413080444,-32.3905528841213,19.9143644494691));
#75639=CARTESIAN_POINT('Origin',(11.9,-32.3839653438087,19.9093266739737));
#75640=CARTESIAN_POINT('',(12.3548486633046,-35.5928236469852,22.856966221146));
#75641=CARTESIAN_POINT('Origin',(20.8267261185512,0.,0.));
#75642=CARTESIAN_POINT('',(12.600317055424,-32.1795566506761,20.2523726527878));
#75643=CARTESIAN_POINT('Origin',(12.6,-32.1839653438087,20.2557368354874));
#75644=CARTESIAN_POINT('',(13.103292255208,-35.4582316768749,23.0652077022745));
#75645=CARTESIAN_POINT('Origin',(25.13830739299,0.,0.));
#75646=CARTESIAN_POINT('',(13.2001612154348,-32.0783403153759,20.4245471623811));
#75647=CARTESIAN_POINT('Origin',(13.2,-32.0839653438087,20.4289419162443));
#75648=CARTESIAN_POINT('',(21.896707744792,-35.4582316768749,23.0652077022745));
#75649=CARTESIAN_POINT('',(17.5,-35.4582316768749,23.0652077022745));
#75650=CARTESIAN_POINT('',(21.7978078257374,-32.0074773662801,20.3691829588007));
#75651=CARTESIAN_POINT('Origin',(21.8,-32.0839653438087,20.4289419162443));
#75652=CARTESIAN_POINT('',(22.6451513366954,-35.5928236469852,22.856966221146));
#75653=CARTESIAN_POINT('Origin',(9.86169260701004,0.,0.));
#75654=CARTESIAN_POINT('',(22.3997512812625,-32.180506880376,20.2530977534517));
#75655=CARTESIAN_POINT('Origin',(22.4,-32.1839653438087,20.2557368354874));
#75656=CARTESIAN_POINT('',(23.3381365738089,-35.8039823302992,22.5247608043155));
#75657=CARTESIAN_POINT('Origin',(14.1732738814488,0.,0.));
#75658=CARTESIAN_POINT('',(23.1003542130464,-32.3890524021132,19.9132169663217));
#75659=CARTESIAN_POINT('Origin',(23.1,-32.3839653438087,19.9093266739737));
#75660=CARTESIAN_POINT('',(24.1697957402248,-35.9356238333033,22.3141421459872));
#75661=CARTESIAN_POINT('Origin',(8.01433437672607,0.,0.));
#75662=CARTESIAN_POINT('',(24.100209736014,-32.544187318536,19.6575262381569));
#75663=CARTESIAN_POINT('Origin',(24.1,-32.5339653438087,19.6495190528383));
#75664=CARTESIAN_POINT('',(29.9005519666592,-35.7462425436685,22.6162805078382));
#75665=CARTESIAN_POINT('Origin',(97.7155570771054,0.,0.));
#75666=CARTESIAN_POINT('',(30.4426385593966,-32.6604876193617,20.2466717586953));
#75667=CARTESIAN_POINT('Origin',(30.5,-32.3339653438087,19.9959292143521));
#75668=CARTESIAN_POINT('',(29.9040600247032,-35.4582316768749,23.0652077022745));
#75669=CARTESIAN_POINT('Origin',(35.8405517186909,0.,0.));
#75670=CARTESIAN_POINT('',(30.5047502791291,-32.0570688314042,20.4079280576996));
#75671=CARTESIAN_POINT('Origin',(30.5,-32.0839653438087,20.4289419162443));
#75672=CARTESIAN_POINT('',(17.5,-35.4582316768749,23.0652077022745));
#75673=CARTESIAN_POINT('Origin',(17.5,-37.0225860117848,21.375));
#75674=CARTESIAN_POINT('Origin',(17.5,0.,0.));
#75675=CARTESIAN_POINT('',(0.600000000000001,-33.234910440458,26.1673599741116));
#75676=CARTESIAN_POINT('Origin',(0.600000000000001,0.,0.));
#75677=CARTESIAN_POINT('',(1.67735469196904,-33.8016349549212,25.4310730087083));
#75678=CARTESIAN_POINT('Origin',(8.14497546096349,0.,0.));
#75679=CARTESIAN_POINT('',(5.09593997529677,-33.8016349549212,25.4310730087083));
#75680=CARTESIAN_POINT('',(17.5,-33.8016349549212,25.4310730087083));
#75681=CARTESIAN_POINT('',(5.09944803334083,-33.4782869009794,25.8552568383243));
#75682=CARTESIAN_POINT('Origin',(-0.840551718690872,0.,0.));
#75683=CARTESIAN_POINT('',(10.8302042597752,-33.2591419277157,26.1365544445335));
#75684=CARTESIAN_POINT('Origin',(-62.7155570771055,0.,0.));
#75685=CARTESIAN_POINT('',(11.6618634261911,-33.4120346810215,25.9408160718628));
#75686=CARTESIAN_POINT('Origin',(26.9856656232739,0.,0.));
#75687=CARTESIAN_POINT('',(12.3548486633046,-33.6519851366708,25.6287708710599));
#75688=CARTESIAN_POINT('Origin',(20.8267261185512,0.,0.));
#75689=CARTESIAN_POINT('',(13.103292255208,-33.8016349549212,25.4310730087083));
#75690=CARTESIAN_POINT('Origin',(25.13830739299,0.,0.));
#75691=CARTESIAN_POINT('',(21.896707744792,-33.8016349549212,25.4310730087083));
#75692=CARTESIAN_POINT('',(17.5,-33.8016349549212,25.4310730087083));
#75693=CARTESIAN_POINT('',(22.6451513366954,-33.6519851366708,25.6287708710599));
#75694=CARTESIAN_POINT('Origin',(9.86169260701005,0.,0.));
#75695=CARTESIAN_POINT('',(23.3381365738089,-33.4120346810215,25.9408160718628));
#75696=CARTESIAN_POINT('Origin',(14.1732738814488,0.,0.));
#75697=CARTESIAN_POINT('',(24.1697957402248,-33.2591419277157,26.1365544445335));
#75698=CARTESIAN_POINT('Origin',(8.01433437672609,0.,0.));
#75699=CARTESIAN_POINT('',(29.9005519666592,-33.4782869009794,25.8552568383243));
#75700=CARTESIAN_POINT('Origin',(97.7155570771054,0.,0.));
#75701=CARTESIAN_POINT('',(29.9040600247032,-33.8016349549212,25.4310730087083));
#75702=CARTESIAN_POINT('Origin',(35.8405517186909,0.,0.));
#75703=CARTESIAN_POINT('',(17.5,-33.8016349549212,25.4310730087083));
#75704=CARTESIAN_POINT('Origin',(33.1,-30.1702883945039,23.1619558369422));
#75705=CARTESIAN_POINT('',(30.5247014514712,-30.0197706669552,23.0679019220779));
#75706=CARTESIAN_POINT('Origin',(30.5,-30.1702883945039,23.1619558369422));
#75707=CARTESIAN_POINT('',(30.4955273645547,-29.8759744160904,23.562215640718));
#75708=CARTESIAN_POINT('Origin',(30.5,-29.8488945896607,23.5449780585017));
#75709=CARTESIAN_POINT('',(24.1012882089558,-29.6594674741542,23.893572647341));
#75710=CARTESIAN_POINT('Origin',(24.1,-29.5917795457861,23.8513958357493));
#75711=CARTESIAN_POINT('',(23.1004586919557,-29.7916028606322,23.6260497451375));
#75712=CARTESIAN_POINT('Origin',(23.1,-29.784615828692,23.6215825028136));
#75713=CARTESIAN_POINT('',(22.399682944576,-30.0370617130518,23.312172527411));
#75714=CARTESIAN_POINT('Origin',(22.4,-30.0417308725666,23.315164725566));
#75715=CARTESIAN_POINT('',(21.7998387845652,-30.1642348036977,23.1581731335784));
#75716=CARTESIAN_POINT('Origin',(21.8,-30.1702883945039,23.1619558369422));
#75717=CARTESIAN_POINT('',(13.2021921742626,-30.0879729141313,23.1105194160696));
#75718=CARTESIAN_POINT('Origin',(13.2,-30.1702883945039,23.1619558369422));
#75719=CARTESIAN_POINT('',(12.6002487187375,-30.038068082493,23.3128174522151));
#75720=CARTESIAN_POINT('Origin',(12.6,-30.0417308725666,23.315164725566));
#75721=CARTESIAN_POINT('',(11.8996457869536,-29.7900113841146,23.6250322156174));
#75722=CARTESIAN_POINT('Origin',(11.9,-29.784615828692,23.6215825028136));
#75723=CARTESIAN_POINT('',(10.899790263986,-29.6027999600046,23.8582627313001));
#75724=CARTESIAN_POINT('Origin',(10.9,-29.5917795457861,23.8513958357493));
#75725=CARTESIAN_POINT('',(4.55736144060343,-30.1961927037808,23.7660496304069));
#75726=CARTESIAN_POINT('Origin',(4.5,-29.8488945896607,23.5449780585017));
#75727=CARTESIAN_POINT('',(4.49524972087093,-30.1413426776676,23.1438685456221));
#75728=CARTESIAN_POINT('Origin',(4.5,-30.1702883945039,23.1619558369422));
#75729=CARTESIAN_POINT('',(1.90350512467335,-30.1131197861062,23.1262329256631));
#75730=CARTESIAN_POINT('Origin',(1.9,-30.1702883945039,23.1619558369422));
#75731=CARTESIAN_POINT('Ctrl Pts',(0.138207714141626,-33.3938750538235,
26.7099230322464));
#75732=CARTESIAN_POINT('Ctrl Pts',(0.370217470898796,-33.3145607080718,
26.4376444612465));
#75733=CARTESIAN_POINT('Ctrl Pts',(0.600000000000004,-33.234910440458,26.1673599741116));
#75734=CARTESIAN_POINT('Origin',(1.9,-28.0490892825384,25.6899024992348));
#75735=CARTESIAN_POINT('',(5.09593997529677,-30.9143101784803,28.872052684018));
#75736=CARTESIAN_POINT('',(17.5,-30.9143101784803,28.872052684018));
#75737=CARTESIAN_POINT('',(4.47529854852883,-27.9303271288835,25.5580037650976));
#75738=CARTESIAN_POINT('Origin',(4.5,-28.0490892825384,25.6899024992348));
#75739=CARTESIAN_POINT('',(5.09944803334083,-31.2759009022694,28.4799582645661));
#75740=CARTESIAN_POINT('Origin',(-0.840551718690874,0.,0.));
#75741=CARTESIAN_POINT('',(4.50447263544529,-28.3921611545025,25.3305554259542));
#75742=CARTESIAN_POINT('Origin',(4.5,-28.3704830873816,25.3068802776753));
#75743=CARTESIAN_POINT('',(10.8302042597752,-31.5148708405159,28.2152957791621));
#75744=CARTESIAN_POINT('Origin',(-62.7155570771054,0.,0.));
#75745=CARTESIAN_POINT('',(10.8987117910442,-28.6808880677203,25.0597981705973));
#75746=CARTESIAN_POINT('Origin',(10.9,-28.6275981312563,25.0004625004277));
#75747=CARTESIAN_POINT('',(11.6618634261911,-31.3486557215378,28.3998553597108));
#75748=CARTESIAN_POINT('Origin',(26.9856656232739,0.,0.));
#75749=CARTESIAN_POINT('',(11.8995413080444,-28.4403745085892,25.2363809880999));
#75750=CARTESIAN_POINT('Origin',(11.9,-28.4347618483503,25.2302758333634));
#75751=CARTESIAN_POINT('',(12.3548486633046,-31.0830181478507,28.6903465092421));
#75752=CARTESIAN_POINT('Origin',(20.8267261185512,0.,0.));
#75753=CARTESIAN_POINT('',(12.600317055424,-28.1738892734932,25.5326149758775));
#75754=CARTESIAN_POINT('Origin',(12.6,-28.1776468044757,25.536693610611));
#75755=CARTESIAN_POINT('',(13.103292255208,-30.9143101784803,28.872052684018));
#75756=CARTESIAN_POINT('Origin',(25.13830739299,0.,0.));
#75757=CARTESIAN_POINT('',(13.2001612154348,-28.0443128519265,25.684597735621));
#75758=CARTESIAN_POINT('Origin',(13.2,-28.0490892825384,25.6899024992348));
#75759=CARTESIAN_POINT('',(21.896707744792,-30.9143101784803,28.872052684018));
#75760=CARTESIAN_POINT('',(17.5,-30.9143101784803,28.872052684018));
#75761=CARTESIAN_POINT('',(21.7978078257374,-27.9841403633154,25.6177694167211));
#75762=CARTESIAN_POINT('Origin',(21.8,-28.0490892825384,25.6899024992348));
#75763=CARTESIAN_POINT('',(22.6451513366954,-31.0830181478507,28.6903465092421));
#75764=CARTESIAN_POINT('Origin',(9.86169260701004,0.,0.));
#75765=CARTESIAN_POINT('',(22.3997512812625,-28.1746991546599,25.5334940662887));
#75766=CARTESIAN_POINT('Origin',(22.4,-28.1776468044757,25.536693610611));
#75767=CARTESIAN_POINT('',(23.3381365738089,-31.3486557215378,28.3998553597108));
#75768=CARTESIAN_POINT('Origin',(14.1732738814488,0.,0.));
#75769=CARTESIAN_POINT('',(23.1003542130464,-28.4390960806318,25.2349903818335));
#75770=CARTESIAN_POINT('Origin',(23.1,-28.4347618483503,25.2302758333634));
#75771=CARTESIAN_POINT('',(24.1697957402248,-31.5148708405159,28.2152957791621));
#75772=CARTESIAN_POINT('Origin',(8.01433437672607,0.,0.));
#75773=CARTESIAN_POINT('',(24.100209736014,-28.63627437808,25.0101230658929));
#75774=CARTESIAN_POINT('Origin',(24.1,-28.6275981312563,25.0004625004277));
#75775=CARTESIAN_POINT('',(29.9005519666592,-31.2759009022694,28.4799582645661));
#75776=CARTESIAN_POINT('Origin',(97.7155570771055,0.,0.));
#75777=CARTESIAN_POINT('',(30.4426385593966,-28.6485037699886,25.610513477472));
#75778=CARTESIAN_POINT('Origin',(30.5,-28.3704830873816,25.3068802776753));
#75779=CARTESIAN_POINT('',(29.9040600247032,-30.9143101784803,28.872052684018));
#75780=CARTESIAN_POINT('Origin',(35.8405517186909,0.,0.));
#75781=CARTESIAN_POINT('',(30.5047502791291,-28.0262504068355,25.6645373580546));
#75782=CARTESIAN_POINT('Origin',(30.5,-28.0490892825384,25.6899024992348));
#75783=CARTESIAN_POINT('',(17.5,-30.9143101784803,28.872052684018));
#75784=CARTESIAN_POINT('Origin',(17.5,-32.7483999433363,27.4791703140996));
#75785=CARTESIAN_POINT('Origin',(17.5,0.,0.));
#75786=CARTESIAN_POINT('',(0.600000000000001,-28.1860830985703,31.5410006112756));
#75787=CARTESIAN_POINT('Origin',(0.600000000000001,0.,0.));
#75788=CARTESIAN_POINT('',(1.67735469196904,-28.872052684018,30.9143101784803));
#75789=CARTESIAN_POINT('Origin',(8.14497546096349,0.,0.));
#75790=CARTESIAN_POINT('',(5.09593997529677,-28.872052684018,30.9143101784803));
#75791=CARTESIAN_POINT('',(17.5,-28.872052684018,30.9143101784803));
#75792=CARTESIAN_POINT('',(5.09944803334083,-28.4799582645661,31.2759009022694));
#75793=CARTESIAN_POINT('Origin',(-0.840551718690872,0.,0.));
#75794=CARTESIAN_POINT('',(10.8302042597752,-28.2152957791621,31.5148708405159));
#75795=CARTESIAN_POINT('Origin',(-62.7155570771055,0.,0.));
#75796=CARTESIAN_POINT('',(11.6618634261911,-28.3998553597108,31.3486557215378));
#75797=CARTESIAN_POINT('Origin',(26.9856656232739,0.,0.));
#75798=CARTESIAN_POINT('',(12.3548486633046,-28.6903465092421,31.0830181478507));
#75799=CARTESIAN_POINT('Origin',(20.8267261185512,0.,0.));
#75800=CARTESIAN_POINT('',(13.103292255208,-28.872052684018,30.9143101784803));
#75801=CARTESIAN_POINT('Origin',(25.13830739299,0.,0.));
#75802=CARTESIAN_POINT('',(21.896707744792,-28.872052684018,30.9143101784803));
#75803=CARTESIAN_POINT('',(17.5,-28.872052684018,30.9143101784803));
#75804=CARTESIAN_POINT('',(22.6451513366954,-28.6903465092421,31.0830181478507));
#75805=CARTESIAN_POINT('Origin',(9.86169260701006,0.,0.));
#75806=CARTESIAN_POINT('',(23.3381365738089,-28.3998553597108,31.3486557215378));
#75807=CARTESIAN_POINT('Origin',(14.1732738814488,0.,0.));
#75808=CARTESIAN_POINT('',(24.1697957402248,-28.2152957791621,31.5148708405159));
#75809=CARTESIAN_POINT('Origin',(8.01433437672609,0.,0.));
#75810=CARTESIAN_POINT('',(29.9005519666592,-28.4799582645661,31.2759009022694));
#75811=CARTESIAN_POINT('Origin',(97.7155570771053,0.,0.));
#75812=CARTESIAN_POINT('',(29.9040600247032,-28.872052684018,30.9143101784803));
#75813=CARTESIAN_POINT('Origin',(35.8405517186909,0.,0.));
#75814=CARTESIAN_POINT('',(17.5,-28.872052684018,30.9143101784803));
#75815=CARTESIAN_POINT('Origin',(33.1,-25.6899024992348,28.0490892825384));
#75816=CARTESIAN_POINT('',(30.5247014514712,-25.5580037650976,27.9303271288835));
#75817=CARTESIAN_POINT('Origin',(30.5,-25.6899024992348,28.0490892825384));
#75818=CARTESIAN_POINT('',(30.4955273645547,-25.3305554259542,28.3921611545025));
#75819=CARTESIAN_POINT('Origin',(30.5,-25.3068802776753,28.3704830873816));
#75820=CARTESIAN_POINT('',(24.1012882089558,-25.0597981705973,28.6808880677203));
#75821=CARTESIAN_POINT('Origin',(24.1,-25.0004625004277,28.6275981312563));
#75822=CARTESIAN_POINT('',(23.1004586919557,-25.2363809880999,28.4403745085892));
#75823=CARTESIAN_POINT('Origin',(23.1,-25.2302758333634,28.4347618483503));
#75824=CARTESIAN_POINT('',(22.399682944576,-25.5326149758775,28.1738892734932));
#75825=CARTESIAN_POINT('Origin',(22.4,-25.536693610611,28.1776468044757));
#75826=CARTESIAN_POINT('',(21.7998387845652,-25.684597735621,28.0443128519265));
#75827=CARTESIAN_POINT('Origin',(21.8,-25.6899024992348,28.0490892825384));
#75828=CARTESIAN_POINT('',(13.2021921742626,-25.6177694167211,27.9841403633154));
#75829=CARTESIAN_POINT('Origin',(13.2,-25.6899024992348,28.0490892825384));
#75830=CARTESIAN_POINT('',(12.6002487187375,-25.5334940662887,28.1746991546599));
#75831=CARTESIAN_POINT('Origin',(12.6,-25.536693610611,28.1776468044757));
#75832=CARTESIAN_POINT('',(11.8996457869536,-25.2349903818335,28.4390960806318));
#75833=CARTESIAN_POINT('Origin',(11.9,-25.2302758333634,28.4347618483503));
#75834=CARTESIAN_POINT('',(10.899790263986,-25.0101230658929,28.63627437808));
#75835=CARTESIAN_POINT('Origin',(10.9,-25.0004625004277,28.6275981312563));
#75836=CARTESIAN_POINT('',(4.55736144060343,-25.610513477472,28.6485037699886));
#75837=CARTESIAN_POINT('Origin',(4.5,-25.3068802776753,28.3704830873816));
#75838=CARTESIAN_POINT('',(4.49524972087093,-25.6645373580546,28.0262504068355));
#75839=CARTESIAN_POINT('Origin',(4.5,-25.6899024992348,28.0490892825384));
#75840=CARTESIAN_POINT('',(1.90350512467335,-25.6398056289004,28.0039818578826));
#75841=CARTESIAN_POINT('Origin',(1.9,-25.6899024992348,28.0490892825384));
#75842=CARTESIAN_POINT('Ctrl Pts',(0.13820771414163,-28.2484175959528,32.1029248328492));
#75843=CARTESIAN_POINT('Ctrl Pts',(0.370217470902555,-28.2175888910028,
31.8210099935422));
#75844=CARTESIAN_POINT('Ctrl Pts',(0.600000000000005,-28.1860830985703,
31.5410006112756));
#75845=CARTESIAN_POINT('Origin',(1.9,-23.1619558369422,30.170288394504));
#75846=CARTESIAN_POINT('',(5.09593997529677,-25.4310730087083,33.8016349549212));
#75847=CARTESIAN_POINT('',(17.5,-25.4310730087083,33.8016349549212));
#75848=CARTESIAN_POINT('',(4.47529854852883,-23.0679019220779,30.0197706669552));
#75849=CARTESIAN_POINT('Origin',(4.5,-23.1619558369422,30.170288394504));
#75850=CARTESIAN_POINT('',(5.09944803334083,-25.8552568383243,33.4782869009794));
#75851=CARTESIAN_POINT('Origin',(-0.840551718690874,0.,0.));
#75852=CARTESIAN_POINT('',(4.50447263544529,-23.562215640718,29.8759744160904));
#75853=CARTESIAN_POINT('Origin',(4.5,-23.5449780585017,29.8488945896607));
#75854=CARTESIAN_POINT('',(10.8302042597752,-26.1365544445335,33.2591419277157));
#75855=CARTESIAN_POINT('Origin',(-62.7155570771055,0.,0.));
#75856=CARTESIAN_POINT('',(10.8987117910442,-23.893572647341,29.6594674741542));
#75857=CARTESIAN_POINT('Origin',(10.9,-23.8513958357493,29.5917795457861));
#75858=CARTESIAN_POINT('',(11.6618634261911,-25.9408160718628,33.4120346810215));
#75859=CARTESIAN_POINT('Origin',(26.9856656232739,0.,0.));
#75860=CARTESIAN_POINT('',(11.8995413080444,-23.6260497451375,29.7916028606322));
#75861=CARTESIAN_POINT('Origin',(11.9,-23.6215825028136,29.784615828692));
#75862=CARTESIAN_POINT('',(12.3548486633046,-25.6287708710599,33.6519851366708));
#75863=CARTESIAN_POINT('Origin',(20.8267261185512,0.,0.));
#75864=CARTESIAN_POINT('',(12.600317055424,-23.312172527411,30.0370617130518));
#75865=CARTESIAN_POINT('Origin',(12.6,-23.315164725566,30.0417308725666));
#75866=CARTESIAN_POINT('',(13.103292255208,-25.4310730087083,33.8016349549212));
#75867=CARTESIAN_POINT('Origin',(25.13830739299,0.,0.));
#75868=CARTESIAN_POINT('',(13.2001612154348,-23.1581731335784,30.1642348036977));
#75869=CARTESIAN_POINT('Origin',(13.2,-23.1619558369422,30.170288394504));
#75870=CARTESIAN_POINT('',(21.896707744792,-25.4310730087083,33.8016349549212));
#75871=CARTESIAN_POINT('',(17.5,-25.4310730087083,33.8016349549212));
#75872=CARTESIAN_POINT('',(21.7978078257374,-23.1105194160696,30.0879729141313));
#75873=CARTESIAN_POINT('Origin',(21.8,-23.1619558369422,30.170288394504));
#75874=CARTESIAN_POINT('',(22.6451513366954,-25.6287708710599,33.6519851366708));
#75875=CARTESIAN_POINT('Origin',(9.86169260701004,0.,0.));
#75876=CARTESIAN_POINT('',(22.3997512812625,-23.3128174522151,30.038068082493));
#75877=CARTESIAN_POINT('Origin',(22.4,-23.315164725566,30.0417308725666));
#75878=CARTESIAN_POINT('',(23.3381365738089,-25.9408160718628,33.4120346810215));
#75879=CARTESIAN_POINT('Origin',(14.1732738814488,0.,0.));
#75880=CARTESIAN_POINT('',(23.1003542130464,-23.6250322156174,29.7900113841146));
#75881=CARTESIAN_POINT('Origin',(23.1,-23.6215825028136,29.784615828692));
#75882=CARTESIAN_POINT('',(24.1697957402248,-26.1365544445335,33.2591419277157));
#75883=CARTESIAN_POINT('Origin',(8.01433437672608,0.,0.));
#75884=CARTESIAN_POINT('',(24.100209736014,-23.8582627313001,29.6027999600046));
#75885=CARTESIAN_POINT('Origin',(24.1,-23.8513958357493,29.5917795457861));
#75886=CARTESIAN_POINT('',(29.9005519666592,-25.8552568383243,33.4782869009794));
#75887=CARTESIAN_POINT('Origin',(97.7155570771056,0.,0.));
#75888=CARTESIAN_POINT('',(30.4426385593966,-23.7660496304069,30.1961927037808));
#75889=CARTESIAN_POINT('Origin',(30.5,-23.5449780585017,29.8488945896607));
#75890=CARTESIAN_POINT('',(29.9040600247032,-25.4310730087083,33.8016349549212));
#75891=CARTESIAN_POINT('Origin',(35.8405517186909,0.,0.));
#75892=CARTESIAN_POINT('',(30.5047502791291,-23.1438685456221,30.1413426776677));
#75893=CARTESIAN_POINT('Origin',(30.5,-23.1619558369422,30.170288394504));
#75894=CARTESIAN_POINT('',(17.5,-25.4310730087083,33.8016349549212));
#75895=CARTESIAN_POINT('Origin',(17.5,-27.4791703140996,32.7483999433363));
#75896=CARTESIAN_POINT('Origin',(17.5,0.,0.));
#75897=CARTESIAN_POINT('',(0.600000000000001,-22.2808358845789,35.9562839053824));
#75898=CARTESIAN_POINT('Origin',(0.600000000000001,0.,0.));
#75899=CARTESIAN_POINT('',(1.67735469196904,-23.0652077022745,35.4582316768749));
#75900=CARTESIAN_POINT('Origin',(8.14497546096349,0.,0.));
#75901=CARTESIAN_POINT('',(5.09593997529677,-23.0652077022745,35.4582316768749));
#75902=CARTESIAN_POINT('',(17.5,-23.0652077022745,35.4582316768749));
#75903=CARTESIAN_POINT('',(5.09944803334083,-22.6162805078382,35.7462425436685));
#75904=CARTESIAN_POINT('Origin',(-0.840551718690874,0.,0.));
#75905=CARTESIAN_POINT('',(10.8302042597752,-22.3141421459872,35.9356238333033));
#75906=CARTESIAN_POINT('Origin',(-62.7155570771055,0.,0.));
#75907=CARTESIAN_POINT('',(11.6618634261911,-22.5247608043154,35.8039823302992));
#75908=CARTESIAN_POINT('Origin',(26.9856656232739,0.,0.));
#75909=CARTESIAN_POINT('',(12.3548486633046,-22.856966221146,35.5928236469852));
#75910=CARTESIAN_POINT('Origin',(20.8267261185512,0.,0.));
#75911=CARTESIAN_POINT('',(13.103292255208,-23.0652077022745,35.4582316768749));
#75912=CARTESIAN_POINT('Origin',(25.13830739299,0.,0.));
#75913=CARTESIAN_POINT('',(21.896707744792,-23.0652077022745,35.4582316768749));
#75914=CARTESIAN_POINT('',(17.5,-23.0652077022745,35.4582316768749));
#75915=CARTESIAN_POINT('',(22.6451513366954,-22.856966221146,35.5928236469852));
#75916=CARTESIAN_POINT('Origin',(9.86169260701006,0.,0.));
#75917=CARTESIAN_POINT('',(23.3381365738089,-22.5247608043154,35.8039823302992));
#75918=CARTESIAN_POINT('Origin',(14.1732738814488,0.,0.));
#75919=CARTESIAN_POINT('',(24.1697957402248,-22.3141421459872,35.9356238333033));
#75920=CARTESIAN_POINT('Origin',(8.01433437672609,0.,0.));
#75921=CARTESIAN_POINT('',(29.9005519666592,-22.6162805078382,35.7462425436685));
#75922=CARTESIAN_POINT('Origin',(97.7155570771054,0.,0.));
#75923=CARTESIAN_POINT('',(29.9040600247032,-23.0652077022745,35.4582316768749));
#75924=CARTESIAN_POINT('Origin',(35.8405517186909,0.,0.));
#75925=CARTESIAN_POINT('',(17.5,-23.0652077022745,35.4582316768749));
#75926=CARTESIAN_POINT('Origin',(33.1,-20.4289419162443,32.0839653438087));
#75927=CARTESIAN_POINT('',(30.5247014514712,-20.3196698518115,31.9441034793054));
#75928=CARTESIAN_POINT('Origin',(30.5,-20.4289419162443,32.0839653438087));
#75929=CARTESIAN_POINT('',(30.4955273645547,-20.01548032708,32.3594252187343));
#75930=CARTESIAN_POINT('Origin',(30.5,-19.9959292143521,32.3339653438087));
#75931=CARTESIAN_POINT('',(24.1012882089558,-19.6986995804965,32.5967492173916));
#75932=CARTESIAN_POINT('Origin',(24.1,-19.6495190528383,32.5339653438087));
#75933=CARTESIAN_POINT('',(23.1004586919557,-19.9143644494691,32.3905528841213));
#75934=CARTESIAN_POINT('Origin',(23.1,-19.9093266739737,32.3839653438087));
#75935=CARTESIAN_POINT('',(22.399682944576,-20.2523726527878,32.1795566506761));
#75936=CARTESIAN_POINT('Origin',(22.4,-20.2557368354874,32.1839653438087));
#75937=CARTESIAN_POINT('',(21.7998387845652,-20.4245471623811,32.0783403153759));
#75938=CARTESIAN_POINT('Origin',(21.8,-20.4289419162443,32.0839653438087));
#75939=CARTESIAN_POINT('',(13.2021921742626,-20.3691829588007,32.0074773662801));
#75940=CARTESIAN_POINT('Origin',(13.2,-20.4289419162443,32.0839653438087));
#75941=CARTESIAN_POINT('',(12.6002487187375,-20.2530977534517,32.180506880376));
#75942=CARTESIAN_POINT('Origin',(12.6,-20.2557368354874,32.1839653438087));
#75943=CARTESIAN_POINT('',(11.8996457869536,-19.9132169663217,32.3890524021132));
#75944=CARTESIAN_POINT('Origin',(11.9,-19.9093266739737,32.3839653438087));
#75945=CARTESIAN_POINT('',(10.899790263986,-19.6575262381569,32.544187318536));
#75946=CARTESIAN_POINT('Origin',(10.9,-19.6495190528383,32.5339653438087));
#75947=CARTESIAN_POINT('',(4.55736144060343,-20.2466717586953,32.6604876193617));
#75948=CARTESIAN_POINT('Origin',(4.5,-19.9959292143521,32.3339653438087));
#75949=CARTESIAN_POINT('',(4.49524972087093,-20.4079280576995,32.0570688314042));
#75950=CARTESIAN_POINT('Origin',(4.5,-20.4289419162443,32.0839653438087));
#75951=CARTESIAN_POINT('',(1.90350512467335,-20.387438952028,32.0308439720488));
#75952=CARTESIAN_POINT('Origin',(1.9,-20.4289419162443,32.0839653438087));
#75953=CARTESIAN_POINT('Ctrl Pts',(0.138207714141625,-22.244646263818,36.5204955072697));
#75954=CARTESIAN_POINT('Ctrl Pts',(0.370217470898828,-22.2632399142706,
36.2375102394012));
#75955=CARTESIAN_POINT('Ctrl Pts',(0.600000000000003,-22.2808358845789,
35.9562839053824));
#75956=CARTESIAN_POINT('Origin',(1.9,-17.5710580837557,33.7339653438087));
#75957=CARTESIAN_POINT('',(5.09593997529677,-19.1751255543105,37.7041716521717));
#75958=CARTESIAN_POINT('',(17.5,-19.1751255543105,37.7041716521717));
#75959=CARTESIAN_POINT('',(4.47529854852883,-17.5045701882916,33.5694020278343));
#75960=CARTESIAN_POINT('Origin',(4.5,-17.5710580837557,33.7339653438087));
#75961=CARTESIAN_POINT('',(5.09944803334083,-19.6490138787379,37.459394730737));
#75962=CARTESIAN_POINT('Origin',(-0.840551718690876,0.,0.));
#75963=CARTESIAN_POINT('',(4.50447263544529,-18.0163441277467,33.5136270415661));
#75964=CARTESIAN_POINT('Origin',(4.5,-18.0040707856479,33.4839653438087));
#75965=CARTESIAN_POINT('',(10.8302042597752,-19.9640920674886,37.2924258787336));
#75966=CARTESIAN_POINT('Origin',(-62.7155570771054,0.,0.));
#75967=CARTESIAN_POINT('',(10.8987117910442,-18.3802631128033,33.3579488669236));
#75968=CARTESIAN_POINT('Origin',(10.9,-18.3504809471617,33.2839653438087));
#75969=CARTESIAN_POINT('',(11.6618634261911,-19.7447778525305,37.4090062358548));
#75970=CARTESIAN_POINT('Origin',(26.9856656232739,0.,0.));
#75971=CARTESIAN_POINT('',(11.8995413080444,-18.0938594155378,33.4416219555226));
#75972=CARTESIAN_POINT('Origin',(11.9,-18.0906733260263,33.4339653438087));
#75973=CARTESIAN_POINT('',(12.3548486633046,-19.3958063601357,37.5911252244478));
#75974=CARTESIAN_POINT('Origin',(20.8267261185512,0.,0.));
#75975=CARTESIAN_POINT('',(12.600317055424,-17.742127215612,33.6288475295616));
#75976=CARTESIAN_POINT('Origin',(12.6,-17.7442631645126,33.6339653438087));
#75977=CARTESIAN_POINT('',(13.103292255208,-19.1751255543105,37.7041716521717));
#75978=CARTESIAN_POINT('Origin',(25.13830739299,0.,0.));
#75979=CARTESIAN_POINT('',(13.2001612154348,-17.5683840431675,33.7273468611033));
#75980=CARTESIAN_POINT('Origin',(13.2,-17.5710580837557,33.7339653438087));
#75981=CARTESIAN_POINT('',(21.896707744792,-19.1751255543105,37.7041716521717));
#75982=CARTESIAN_POINT('',(17.5,-19.1751255543105,37.7041716521717));
#75983=CARTESIAN_POINT('',(21.7978078257374,-17.5346970308537,33.6439685797946));
#75984=CARTESIAN_POINT('Origin',(21.8,-17.5710580837557,33.7339653438087));
#75985=CARTESIAN_POINT('',(22.6451513366954,-19.3958063601357,37.5911252244479));
#75986=CARTESIAN_POINT('Origin',(9.86169260701005,0.,0.));
#75987=CARTESIAN_POINT('',(22.3997512812625,-17.7425875883397,33.6299506000067));
#75988=CARTESIAN_POINT('Origin',(22.4,-17.7442631645126,33.6339653438087));
#75989=CARTESIAN_POINT('',(23.3381365738089,-19.7447778525305,37.4090062358548));
#75990=CARTESIAN_POINT('Origin',(14.1732738814488,0.,0.));
#75991=CARTESIAN_POINT('',(23.1003542130464,-18.0931337015746,33.4398779649625));
#75992=CARTESIAN_POINT('Origin',(23.1,-18.0906733260263,33.4339653438087));
#75993=CARTESIAN_POINT('',(24.1697957402248,-19.9640920674886,37.2924258787336));
#75994=CARTESIAN_POINT('Origin',(8.01433437672606,0.,0.));
#75995=CARTESIAN_POINT('',(24.100209736014,-18.3553298442931,33.2960107570711));
#75996=CARTESIAN_POINT('Origin',(24.1,-18.3504809471617,33.2839653438087));
#75997=CARTESIAN_POINT('',(29.9005519666592,-19.6490138787379,37.459394730737));
#75998=CARTESIAN_POINT('Origin',(97.7155570771054,0.,0.));
#75999=CARTESIAN_POINT('',(30.4426385593966,-18.1614760990067,33.864375894796));
#76000=CARTESIAN_POINT('Origin',(30.5,-18.0040707856479,33.4839653438087));
#76001=CARTESIAN_POINT('',(29.9040600247032,-19.1751255543105,37.7041716521717));
#76002=CARTESIAN_POINT('Origin',(35.8405517186909,0.,0.));
#76003=CARTESIAN_POINT('',(30.5047502791291,-17.5582719500126,33.7023185522751));
#76004=CARTESIAN_POINT('Origin',(30.5,-17.5710580837557,33.7339653438087));
#76005=CARTESIAN_POINT('',(17.5,-19.1751255543105,37.7041716521717));
#76006=CARTESIAN_POINT('Origin',(17.5,-21.375,37.0225860117848));
#76007=CARTESIAN_POINT('Origin',(17.5,0.,0.));
#76008=CARTESIAN_POINT('',(0.600000000000001,-15.6985967468815,39.2790537077817));
#76009=CARTESIAN_POINT('Origin',(0.600000000000001,0.,0.));
#76010=CARTESIAN_POINT('',(1.67735469196904,-16.5575380560557,38.9247727484987));
#76011=CARTESIAN_POINT('Origin',(8.14497546096349,0.,0.));
#76012=CARTESIAN_POINT('',(5.09593997529677,-16.5575380560557,38.9247727484987));
#76013=CARTESIAN_POINT('',(17.5,-16.5575380560557,38.9247727484987));
#76014=CARTESIAN_POINT('',(5.09944803334083,-16.0654185122698,39.1304526938498));
#76015=CARTESIAN_POINT('Origin',(-0.840551718690872,0.,0.));
#76016=CARTESIAN_POINT('',(10.8302042597752,-15.7349845952072,39.2644910802189));
#76017=CARTESIAN_POINT('Origin',(-62.7155570771055,0.,0.));
#76018=CARTESIAN_POINT('',(11.6618634261911,-15.9652627899599,39.1714230536436));
#76019=CARTESIAN_POINT('Origin',(26.9856656232739,0.,0.));
#76020=CARTESIAN_POINT('',(12.3548486633046,-16.3290885806033,39.0211592104439));
#76021=CARTESIAN_POINT('Origin',(20.8267261185512,0.,0.));
#76022=CARTESIAN_POINT('',(13.103292255208,-16.5575380560557,38.9247727484987));
#76023=CARTESIAN_POINT('Origin',(25.13830739299,0.,0.));
#76024=CARTESIAN_POINT('',(21.896707744792,-16.5575380560557,38.9247727484987));
#76025=CARTESIAN_POINT('',(17.5,-16.5575380560557,38.9247727484987));
#76026=CARTESIAN_POINT('',(22.6451513366954,-16.3290885806033,39.0211592104439));
#76027=CARTESIAN_POINT('Origin',(9.86169260701006,0.,0.));
#76028=CARTESIAN_POINT('',(23.3381365738089,-15.9652627899599,39.1714230536436));
#76029=CARTESIAN_POINT('Origin',(14.1732738814488,0.,0.));
#76030=CARTESIAN_POINT('',(24.1697957402248,-15.7349845952072,39.2644910802189));
#76031=CARTESIAN_POINT('Origin',(8.01433437672609,0.,0.));
#76032=CARTESIAN_POINT('',(29.9005519666592,-16.0654185122698,39.1304526938498));
#76033=CARTESIAN_POINT('Origin',(97.7155570771054,0.,0.));
#76034=CARTESIAN_POINT('',(29.9040600247032,-16.5575380560557,38.9247727484987));
#76035=CARTESIAN_POINT('Origin',(35.8405517186909,0.,0.));
#76036=CARTESIAN_POINT('',(17.5,-16.5575380560557,38.9247727484987));
#76037=CARTESIAN_POINT('Origin',(33.1,-14.5472582706722,35.1439863533772));
#76038=CARTESIAN_POINT('',(30.5247014514712,-14.4639330523272,34.987274410005));
#76039=CARTESIAN_POINT('Origin',(30.5,-14.5472582706722,35.1439863533772));
#76040=CARTESIAN_POINT('',(30.4955273645547,-14.0922449867892,35.343464522354));
#76041=CARTESIAN_POINT('Origin',(30.5,-14.0774119602792,35.31499642504));
#76042=CARTESIAN_POINT('',(24.1012882089558,-13.7390659716653,35.5221746368434));
#76043=CARTESIAN_POINT('Origin',(24.1,-13.7015349119648,35.4518044823703));
#76044=CARTESIAN_POINT('',(23.1004586919557,-13.9872600241959,35.35656070068));
#76045=CARTESIAN_POINT('Origin',(23.1,-13.9834426982006,35.3491984393726));
#76046=CARTESIAN_POINT('',(22.399682944576,-14.3567722348382,35.2074644826695));
#76047=CARTESIAN_POINT('Origin',(22.4,-14.359319746515,35.2123903820423));
#76048=CARTESIAN_POINT('',(21.7998387845652,-14.5439070589317,35.137683640766));
#76049=CARTESIAN_POINT('Origin',(21.8,-14.5472582706722,35.1439863533772));
#76050=CARTESIAN_POINT('',(13.2021921742626,-14.501689183981,35.0582833660355));
#76051=CARTESIAN_POINT('Origin',(13.2,-14.5472582706722,35.1439863533772));
#76052=CARTESIAN_POINT('',(12.6002487187375,-14.3573213139379,35.208526188654));
#76053=CARTESIAN_POINT('Origin',(12.6,-14.359319746515,35.2123903820423));
#76054=CARTESIAN_POINT('',(11.8996457869536,-13.9863905298622,35.3548837560077));
#76055=CARTESIAN_POINT('Origin',(11.9,-13.9834426982006,35.3491984393726));
#76056=CARTESIAN_POINT('',(10.899790263986,-13.7076454228629,35.4632615954717));
#76057=CARTESIAN_POINT('Origin',(10.9,-13.7015349119648,35.4518044823703));
#76058=CARTESIAN_POINT('',(4.55736144060343,-14.267645163841,35.6800990794245));
#76059=CARTESIAN_POINT('Origin',(4.5,-14.0774119602792,35.31499642504));
#76060=CARTESIAN_POINT('',(4.49524972087093,-14.5312341902212,35.1138494411902));
#76061=CARTESIAN_POINT('Origin',(4.5,-14.5472582706722,35.1439863533772));
#76062=CARTESIAN_POINT('',(1.90350512467335,-14.5156102591402,35.0844651005135));
#76063=CARTESIAN_POINT('Origin',(1.9,-14.5472582706722,35.1439863533772));
#76064=CARTESIAN_POINT('Ctrl Pts',(0.138207714141622,-15.5649826112914,
39.8284094059642));
#76065=CARTESIAN_POINT('Ctrl Pts',(0.370217470894697,-15.6324336584846,
39.5529520737012));
#76066=CARTESIAN_POINT('Ctrl Pts',(0.600000000000004,-15.6985967468815,
39.2790537077817));
#76067=CARTESIAN_POINT('Origin',(1.9,-11.4462726220787,36.2726528263519));
#76068=CARTESIAN_POINT('',(5.09593997529677,-12.3365516130268,40.4610861730024));
#76069=CARTESIAN_POINT('',(17.5,-12.3365516130268,40.4610861730024));
#76070=CARTESIAN_POINT('',(4.47529854852883,-11.409370947074,36.0990440950346));
#76071=CARTESIAN_POINT('Origin',(4.5,-11.4462726220787,36.2726528263519));
#76072=CARTESIAN_POINT('',(5.09944803334083,-12.8457455753269,40.3023178069695));
#76073=CARTESIAN_POINT('Origin',(-0.840551718690874,0.,0.));
#76074=CARTESIAN_POINT('',(4.50447263544529,-11.9230551151638,36.1329850680974));
#76075=CARTESIAN_POINT('Origin',(4.5,-11.9161189324716,36.101642754689));
#76076=CARTESIAN_POINT('',(10.8302042597752,-13.1850308552911,40.1925983403042));
#76077=CARTESIAN_POINT('Origin',(-62.7155570771054,0.,0.));
#76078=CARTESIAN_POINT('',(10.8987117910442,-12.3084785844451,36.0428658633082));
#76079=CARTESIAN_POINT('Origin',(10.9,-12.291995980786,35.9648346973588));
#76080=CARTESIAN_POINT('',(11.6618634261911,-12.9488045494888,40.2693240660821));
#76081=CARTESIAN_POINT('Origin',(26.9856656232739,0.,0.));
#76082=CARTESIAN_POINT('',(11.8995413080444,-12.0118963235316,36.0755342895717));
#76083=CARTESIAN_POINT('Origin',(11.9,-12.0100881945502,36.0674407403565));
#76084=CARTESIAN_POINT('',(12.3548486633046,-12.5735100877104,40.3880779943072));
#76085=CARTESIAN_POINT('Origin',(20.8267261185512,0.,0.));
#76086=CARTESIAN_POINT('',(12.600317055424,-11.6329963463162,36.1988378309035));
#76087=CARTESIAN_POINT('Origin',(12.6,-11.6342111462358,36.2042487976867));
#76088=CARTESIAN_POINT('',(13.103292255208,-12.3365516130268,40.4610861730024));
#76089=CARTESIAN_POINT('Origin',(25.13830739299,0.,0.));
#76090=CARTESIAN_POINT('',(13.2001612154348,-11.4447884936362,36.2656705509953));
#76091=CARTESIAN_POINT('Origin',(13.2,-11.4462726220787,36.2726528263519));
#76092=CARTESIAN_POINT('',(21.896707744792,-12.3365516130268,40.4610861730024));
#76093=CARTESIAN_POINT('',(17.5,-12.3365516130268,40.4610861730024));
#76094=CARTESIAN_POINT('',(21.7978078257374,-11.4260917493401,36.1777092848303));
#76095=CARTESIAN_POINT('Origin',(21.8,-11.4462726220787,36.2726528263519));
#76096=CARTESIAN_POINT('',(22.6451513366954,-12.5735100877104,40.3880779943072));
#76097=CARTESIAN_POINT('Origin',(9.86169260701004,0.,0.));
#76098=CARTESIAN_POINT('',(22.3997512812625,-11.633258178775,36.2000040861152));
#76099=CARTESIAN_POINT('Origin',(22.4,-11.6342111462358,36.2042487976867));
#76100=CARTESIAN_POINT('',(23.3381365738089,-12.9488045494888,40.2693240660821));
#76101=CARTESIAN_POINT('Origin',(14.1732738814488,0.,0.));
#76102=CARTESIAN_POINT('',(23.1003542130464,-12.0114844755768,36.0736907752397));
#76103=CARTESIAN_POINT('Origin',(23.1,-12.0100881945502,36.0674407403565));
#76104=CARTESIAN_POINT('',(24.1697957402248,-13.1850308552911,40.1925983403042));
#76105=CARTESIAN_POINT('Origin',(8.01433437672608,0.,0.));
#76106=CARTESIAN_POINT('',(24.100209736014,-12.2946795482123,35.9775391158784));
#76107=CARTESIAN_POINT('Origin',(24.1,-12.291995980786,35.9648346973588));
#76108=CARTESIAN_POINT('',(29.9005519666592,-12.8457455753269,40.3023178069695));
#76109=CARTESIAN_POINT('Origin',(97.7155570771054,0.,0.));
#76110=CARTESIAN_POINT('',(30.4426385593966,-12.0050753064884,36.5036071604488));
#76111=CARTESIAN_POINT('Origin',(30.5,-11.9161189324716,36.101642754689));
#76112=CARTESIAN_POINT('',(29.9040600247032,-12.3365516130268,40.4610861730024));
#76113=CARTESIAN_POINT('Origin',(35.8405517186909,0.,0.));
#76114=CARTESIAN_POINT('',(30.5047502791291,-11.4391761461162,36.2392665318678));
#76115=CARTESIAN_POINT('Origin',(30.5,-11.4462726220787,36.2726528263519));
#76116=CARTESIAN_POINT('',(17.5,-12.3365516130268,40.4610861730024));
#76117=CARTESIAN_POINT('Origin',(17.5,-14.6213611271723,40.1718595385976));
#76118=CARTESIAN_POINT('Origin',(17.5,0.,0.));
#76119=CARTESIAN_POINT('',(0.600000000000001,-8.63936369090332,41.4083493394303));
#76120=CARTESIAN_POINT('Origin',(0.600000000000001,0.,0.));
#76121=CARTESIAN_POINT('',(1.67735469196904,-9.54677599452213,41.2086042970448));
#76122=CARTESIAN_POINT('Origin',(8.1449754609635,0.,0.));
#76123=CARTESIAN_POINT('',(5.09593997529677,-9.54677599452213,41.2086042970448));
#76124=CARTESIAN_POINT('',(17.5,-9.54677599452213,41.2086042970448));
#76125=CARTESIAN_POINT('',(5.09944803334083,-9.02641690470011,41.325703839893));
#76126=CARTESIAN_POINT('Origin',(-0.840551718690872,0.,0.));
#76127=CARTESIAN_POINT('',(10.8302042597752,-8.6777274997883,41.4003266344532));
#76128=CARTESIAN_POINT('Origin',(-62.7155570771055,0.,0.));
#76129=CARTESIAN_POINT('',(11.6618634261911,-8.92066834454427,41.3486599091996));
#76130=CARTESIAN_POINT('Origin',(26.9856656232739,0.,0.));
#76131=CARTESIAN_POINT('',(12.3548486633046,-9.30505984645652,41.2638565969525));
#76132=CARTESIAN_POINT('Origin',(20.8267261185512,0.,0.));
#76133=CARTESIAN_POINT('',(13.103292255208,-9.54677599452213,41.2086042970448));
#76134=CARTESIAN_POINT('Origin',(25.13830739299,0.,0.));
#76135=CARTESIAN_POINT('',(21.896707744792,-9.54677599452213,41.2086042970448));
#76136=CARTESIAN_POINT('',(17.5,-9.54677599452213,41.2086042970448));
#76137=CARTESIAN_POINT('',(22.6451513366954,-9.30505984645651,41.2638565969525));
#76138=CARTESIAN_POINT('Origin',(9.86169260701005,0.,0.));
#76139=CARTESIAN_POINT('',(23.3381365738089,-8.92066834454427,41.3486599091995));
#76140=CARTESIAN_POINT('Origin',(14.1732738814488,0.,0.));
#76141=CARTESIAN_POINT('',(24.1697957402248,-8.6777274997883,41.4003266344532));
#76142=CARTESIAN_POINT('Origin',(8.01433437672608,0.,0.));
#76143=CARTESIAN_POINT('',(29.9005519666592,-9.02641690470011,41.325703839893));
#76144=CARTESIAN_POINT('Origin',(97.7155570771054,0.,0.));
#76145=CARTESIAN_POINT('',(29.9040600247032,-9.54677599452213,41.2086042970448));
#76146=CARTESIAN_POINT('Origin',(35.8405517186909,0.,0.));
#76147=CARTESIAN_POINT('',(17.5,-9.54677599452213,41.2086042970448));
#76148=CARTESIAN_POINT('Origin',(33.1,-8.22356354381349,37.1361751213135));
#76149=CARTESIAN_POINT('',(30.5247014514712,-8.16871696615113,36.9673747121716));
#76150=CARTESIAN_POINT('Origin',(30.5,-8.22356354381349,37.1361751213135));
#76151=CARTESIAN_POINT('',(30.4955273645547,-7.74082391359484,37.253610541118));
#76152=CARTESIAN_POINT('Origin',(30.5,-7.73115966730739,37.2229992101469));
#76153=CARTESIAN_POINT('',(24.1012882089558,-7.36197779558791,37.3682767550424));
#76154=CARTESIAN_POINT('Origin',(24.1,-7.33723656610251,37.2924584812137));
#76155=CARTESIAN_POINT('',(23.1004586919557,-7.63515978098256,37.2482773116316));
#76156=CARTESIAN_POINT('Origin',(23.1,-7.63267889200617,37.2403640279136));
#76157=CARTESIAN_POINT('',(22.399682944576,-8.02494855741037,37.1656113221937));
#76158=CARTESIAN_POINT('Origin',(22.4,-8.02660199321105,37.1709047568469));
#76159=CARTESIAN_POINT('',(21.7998387845652,-8.22135769906884,37.1293862292573));
#76160=CARTESIAN_POINT('Origin',(21.8,-8.22356354381349,37.1361751213135));
#76161=CARTESIAN_POINT('',(13.2021921742626,-8.19356892151487,37.0438611660612));
#76162=CARTESIAN_POINT('Origin',(13.2,-8.22356354381349,37.1361751213135));
#76163=CARTESIAN_POINT('',(12.6002487187375,-8.02530493145534,37.1667522450638));
#76164=CARTESIAN_POINT('Origin',(12.6,-8.02660199321105,37.1709047568469));
#76165=CARTESIAN_POINT('',(11.8996457869536,-7.6345946946079,37.2464748574103));
#76166=CARTESIAN_POINT('Origin',(11.9,-7.63267889200617,37.2403640279136));
#76167=CARTESIAN_POINT('',(10.899790263986,-7.34126473779837,37.3048026141052));
#76168=CARTESIAN_POINT('Origin',(10.9,-7.33723656610251,37.2924584812137));
#76169=CARTESIAN_POINT('',(4.55736144060343,-7.85510339046016,37.6155887839604));
#76170=CARTESIAN_POINT('Origin',(4.5,-7.73115966730739,37.2229992101469));
#76171=CARTESIAN_POINT('',(4.49524972087093,-8.21301612503227,37.1037135041708));
#76172=CARTESIAN_POINT('Origin',(4.5,-8.22356354381349,37.1361751213135));
#76173=CARTESIAN_POINT('',(1.90350512467335,-8.20273209378168,37.0720625104951));
#76174=CARTESIAN_POINT('Origin',(1.9,-8.22356354381349,37.1361751213135));
#76175=CARTESIAN_POINT('Ctrl Pts',(0.138207714141624,-8.41238483838185,
41.9261572390061));
#76176=CARTESIAN_POINT('Ctrl Pts',(0.37021747089798,-8.52664381638061,41.6665974739926));
#76177=CARTESIAN_POINT('Ctrl Pts',(0.600000000000004,-8.63936369090332,
41.4083493394303));
#76178=CARTESIAN_POINT('Origin',(1.9,-4.97369795887321,37.7092141076143));
#76179=CARTESIAN_POINT('',(5.09593997529677,-5.12313779357752,41.9886110647639));
#76180=CARTESIAN_POINT('',(17.5,-5.12313779357752,41.9886110647639));
#76181=CARTESIAN_POINT('',(4.47529854852883,-4.96750374304976,37.5318349744051));
#76182=CARTESIAN_POINT('Origin',(4.5,-4.97369795887321,37.7092141076143));
#76183=CARTESIAN_POINT('',(5.09944803334083,-5.65216579287046,41.9206753505941));
#76184=CARTESIAN_POINT('Origin',(-0.840551718690874,0.,0.));
#76185=CARTESIAN_POINT('',(4.50447263544529,-5.46749010626366,37.6544606275072));
#76186=CARTESIAN_POINT('Origin',(4.5,-5.46610183537931,37.6223900187809));
#76187=CARTESIAN_POINT('',(10.8302042597752,-6.00534915250318,41.8715390397407));
#76188=CARTESIAN_POINT('Origin',(-62.7155570771055,0.,0.));
#76189=CARTESIAN_POINT('',(10.8987117910442,-5.86270716268919,37.6326386190063));
#76190=CARTESIAN_POINT('Origin',(10.9,-5.8600249365842,37.5529307477141));
#76191=CARTESIAN_POINT('',(11.6618634261911,-5.75938837262207,41.9060788618227));
#76192=CARTESIAN_POINT('Origin',(26.9856656232739,0.,0.));
#76193=CARTESIAN_POINT('',(11.8995413080444,-5.56495784004781,37.6133097693334));
#76194=CARTESIAN_POINT('Origin',(11.9,-5.56458261068053,37.6050252010142));
#76195=CARTESIAN_POINT('',(12.3548486633046,-5.3691740737731,41.9578594516632));
#76196=CARTESIAN_POINT('Origin',(20.8267261185512,0.,0.));
#76197=CARTESIAN_POINT('',(12.600317055424,-5.17040276961776,37.6689447622493));
#76198=CARTESIAN_POINT('Origin',(12.6,-5.17065950947565,37.674484472081));
#76199=CARTESIAN_POINT('',(13.103292255208,-5.12313779357752,41.9886110647639));
#76200=CARTESIAN_POINT('Origin',(25.13830739299,0.,0.));
#76201=CARTESIAN_POINT('',(13.2001612154348,-4.97344883706828,37.7020801925101));
#76202=CARTESIAN_POINT('Origin',(13.2,-4.97369795887321,37.7092141076143));
#76203=CARTESIAN_POINT('',(21.896707744792,-5.12313779357752,41.9886110647639));
#76204=CARTESIAN_POINT('',(17.5,-5.12313779357752,41.9886110647639));
#76205=CARTESIAN_POINT('',(21.7978078257374,-4.97031045190415,37.6122086000506));
#76206=CARTESIAN_POINT('Origin',(21.8,-4.97369795887321,37.7092141076143));
#76207=CARTESIAN_POINT('',(22.6451513366954,-5.3691740737731,41.9578594516632));
#76208=CARTESIAN_POINT('Origin',(9.86169260701005,0.,0.));
#76209=CARTESIAN_POINT('',(22.3997512812625,-5.17045810616098,37.6701387661531));
#76210=CARTESIAN_POINT('Origin',(22.4,-5.17065950947565,37.674484472081));
#76211=CARTESIAN_POINT('',(23.3381365738089,-5.75938837262207,41.9060788618227));
#76212=CARTESIAN_POINT('Origin',(14.1732738814488,0.,0.));
#76213=CARTESIAN_POINT('',(23.1003542130464,-5.56487237189312,37.6114227454796));
#76214=CARTESIAN_POINT('Origin',(23.1,-5.56458261068053,37.6050252010142));
#76215=CARTESIAN_POINT('',(24.1697957402248,-6.00534915250318,41.8715390397407));
#76216=CARTESIAN_POINT('Origin',(8.01433437672608,0.,0.));
#76217=CARTESIAN_POINT('',(24.100209736014,-5.8604616354671,37.565908154163));
#76218=CARTESIAN_POINT('Origin',(24.1,-5.8600249365842,37.5529307477141));
#76219=CARTESIAN_POINT('',(29.9005519666592,-5.65216579287046,41.9206753505941));
#76220=CARTESIAN_POINT('Origin',(97.7155570771054,0.,0.));
#76221=CARTESIAN_POINT('',(30.4426385593966,-5.48390637564377,38.0336947942479));
#76222=CARTESIAN_POINT('Origin',(30.5,-5.46610183537931,37.6223900187809));
#76223=CARTESIAN_POINT('',(29.9040600247032,-5.12313779357752,41.9886110647639));
#76224=CARTESIAN_POINT('Origin',(35.8405517186909,0.,0.));
#76225=CARTESIAN_POINT('',(30.5047502791291,-4.97250676352255,37.6751027358433));
#76226=CARTESIAN_POINT('Origin',(30.5,-4.97369795887321,37.7092141076143));
#76227=CARTESIAN_POINT('',(17.5,-5.12313779357752,41.9886110647639));
#76228=CARTESIAN_POINT('Origin',(17.5,-7.42345959526127,42.1005314412719));
#76229=CARTESIAN_POINT('Origin',(17.5,0.,0.));
#76230=CARTESIAN_POINT('',(0.600000000000001,-1.31762794090604,42.2794732300362));
#76231=CARTESIAN_POINT('Origin',(0.600000000000001,0.,0.));
#76232=CARTESIAN_POINT('',(1.67735469196904,-2.24593997529677,42.240333256585));
#76233=CARTESIAN_POINT('Origin',(8.14497546096349,0.,0.));
#76234=CARTESIAN_POINT('',(5.09593997529677,-2.24593997529677,42.240333256585));
#76235=CARTESIAN_POINT('',(17.5,-2.24593997529677,42.240333256585));
#76236=CARTESIAN_POINT('',(5.09944803334083,-1.71315218706844,42.2652943865761));
#76237=CARTESIAN_POINT('Origin',(-0.840551718690872,0.,0.));
#76238=CARTESIAN_POINT('',(10.8302042597752,-1.35680204543027,42.2782342134758));
#76239=CARTESIAN_POINT('Origin',(-62.7155570771055,0.,0.));
#76240=CARTESIAN_POINT('',(11.6618634261911,-1.60502390555561,42.269538656846));
#76241=CARTESIAN_POINT('Origin',(26.9856656232739,0.,0.));
#76242=CARTESIAN_POINT('',(12.3548486633046,-1.99830157746261,42.2527725812817));
#76243=CARTESIAN_POINT('Origin',(20.8267261185512,0.,0.));
#76244=CARTESIAN_POINT('',(13.103292255208,-2.24593997529677,42.240333256585));
#76245=CARTESIAN_POINT('Origin',(25.13830739299,0.,0.));
#76246=CARTESIAN_POINT('',(21.896707744792,-2.24593997529677,42.240333256585));
#76247=CARTESIAN_POINT('',(17.5,-2.24593997529677,42.240333256585));
#76248=CARTESIAN_POINT('',(22.6451513366954,-1.99830157746261,42.2527725812817));
#76249=CARTESIAN_POINT('Origin',(9.86169260701006,0.,0.));
#76250=CARTESIAN_POINT('',(23.3381365738089,-1.60502390555561,42.269538656846));
#76251=CARTESIAN_POINT('Origin',(14.1732738814488,0.,0.));
#76252=CARTESIAN_POINT('',(24.1697957402248,-1.35680204543027,42.2782342134758));
#76253=CARTESIAN_POINT('Origin',(8.01433437672608,0.,0.));
#76254=CARTESIAN_POINT('',(29.9005519666592,-1.71315218706844,42.2652943865761));
#76255=CARTESIAN_POINT('Origin',(97.7155570771054,0.,0.));
#76256=CARTESIAN_POINT('',(29.9040600247032,-2.24593997529677,42.240333256585));
#76257=CARTESIAN_POINT('Origin',(35.8405517186909,0.,0.));
#76258=CARTESIAN_POINT('',(17.5,-2.24593997529677,42.240333256585));
#76259=CARTESIAN_POINT('Origin',(33.1,-1.65,38.));
#76260=CARTESIAN_POINT('',(30.5247014514712,-1.62529854852883,37.8242400401031));
#76261=CARTESIAN_POINT('Origin',(30.5,-1.65,38.));
#76262=CARTESIAN_POINT('',(30.4955273645547,-1.15420182283181,38.0318244548267));
#76263=CARTESIAN_POINT('Origin',(30.5,-1.15,38.));
#76264=CARTESIAN_POINT('',(24.1012882089558,-0.761199649532069,38.0789626932999));
#76265=CARTESIAN_POINT('Origin',(24.1,-0.749999999999998,38.));
#76266=CARTESIAN_POINT('',(23.1004586919557,-1.05106907140133,38.0082238650069));
#76267=CARTESIAN_POINT('Origin',(23.1,-1.05,38.));
#76268=CARTESIAN_POINT('',(22.399682944576,-1.44929087888549,37.9944998683999));
#76269=CARTESIAN_POINT('Origin',(22.4,-1.45,38.));
#76270=CARTESIAN_POINT('',(21.7998387845652,-1.64900654572746,37.9929312055486));
#76271=CARTESIAN_POINT('Origin',(21.8,-1.65,38.));
#76272=CARTESIAN_POINT('',(13.2021921742626,-1.63649121351442,37.9038799896544));
#76273=CARTESIAN_POINT('Origin',(13.2,-1.65,38.));
#76274=CARTESIAN_POINT('',(12.6002487187375,-1.44944371963071,37.9956853417913));
#76275=CARTESIAN_POINT('Origin',(12.6,-1.45,38.));
#76276=CARTESIAN_POINT('',(11.8996457869536,-1.05082556284928,38.0063506678963));
#76277=CARTESIAN_POINT('Origin',(11.9,-1.05,38.));
#76278=CARTESIAN_POINT('',(10.899790263986,-0.751823438535066,38.01285608245));
#76279=CARTESIAN_POINT('Origin',(10.9,-0.749999999999998,38.));
#76280=CARTESIAN_POINT('',(4.55736144060343,-1.2038882754343,38.408147857702));
#76281=CARTESIAN_POINT('Origin',(4.5,-1.15,38.));
#76282=CARTESIAN_POINT('',(4.49524972087093,-1.64524972087093,37.9662000077121));
#76283=CARTESIAN_POINT('Origin',(4.5,-1.65,38.));
#76284=CARTESIAN_POINT('',(1.90350512467335,-1.64061806453626,37.933244060464));
#76285=CARTESIAN_POINT('Origin',(1.9,-1.65,38.));
#76286=CARTESIAN_POINT('Ctrl Pts',(0.13820771414162,-1.0041810090302,42.75));
#76287=CARTESIAN_POINT('Ctrl Pts',(0.370217470898037,-1.16177621660492,
42.5142243943562));
#76288=CARTESIAN_POINT('Ctrl Pts',(0.600000000000004,-1.31762794090604,
42.2794732300361));
#76289=CARTESIAN_POINT('Origin',(1.9,1.65,38.));
#76290=CARTESIAN_POINT('',(5.09593997529677,2.24593997529677,42.240333256585));
#76291=CARTESIAN_POINT('',(17.5,2.24593997529677,42.240333256585));
#76292=CARTESIAN_POINT('',(4.47529854852883,1.62529854852884,37.8242400401031));
#76293=CARTESIAN_POINT('Origin',(4.5,1.65,38.));
#76294=CARTESIAN_POINT('',(5.09944803334083,1.71315218706845,42.2652943865761));
#76295=CARTESIAN_POINT('Origin',(-0.840551718690874,0.,0.));
#76296=CARTESIAN_POINT('',(4.50447263544529,1.15420182283181,38.0318244548267));
#76297=CARTESIAN_POINT('Origin',(4.5,1.15,38.));
#76298=CARTESIAN_POINT('',(10.8302042597752,1.35680204543028,42.2782342134758));
#76299=CARTESIAN_POINT('Origin',(-62.7155570771055,0.,0.));
#76300=CARTESIAN_POINT('',(10.8987117910442,0.761199649532074,38.0789626932999));
#76301=CARTESIAN_POINT('Origin',(10.9,0.750000000000002,38.));
#76302=CARTESIAN_POINT('',(11.6618634261911,1.60502390555562,42.269538656846));
#76303=CARTESIAN_POINT('Origin',(26.9856656232739,0.,0.));
#76304=CARTESIAN_POINT('',(11.8995413080444,1.05106907140134,38.0082238650069));
#76305=CARTESIAN_POINT('Origin',(11.9,1.05,38.));
#76306=CARTESIAN_POINT('',(12.3548486633046,1.99830157746262,42.2527725812817));
#76307=CARTESIAN_POINT('Origin',(20.8267261185512,0.,0.));
#76308=CARTESIAN_POINT('',(12.600317055424,1.44929087888549,37.9944998683999));
#76309=CARTESIAN_POINT('Origin',(12.6,1.45,38.));
#76310=CARTESIAN_POINT('',(13.103292255208,2.24593997529677,42.240333256585));
#76311=CARTESIAN_POINT('Origin',(25.13830739299,0.,0.));
#76312=CARTESIAN_POINT('',(13.2001612154348,1.64900654572746,37.9929312055486));
#76313=CARTESIAN_POINT('Origin',(13.2,1.65,38.));
#76314=CARTESIAN_POINT('',(21.896707744792,2.24593997529677,42.240333256585));
#76315=CARTESIAN_POINT('',(17.5,2.24593997529677,42.240333256585));
#76316=CARTESIAN_POINT('',(21.7978078257374,1.63649121351443,37.9038799896544));
#76317=CARTESIAN_POINT('Origin',(21.8,1.65,38.));
#76318=CARTESIAN_POINT('',(22.6451513366954,1.99830157746262,42.2527725812817));
#76319=CARTESIAN_POINT('Origin',(9.86169260701005,0.,0.));
#76320=CARTESIAN_POINT('',(22.3997512812625,1.44944371963071,37.9956853417913));
#76321=CARTESIAN_POINT('Origin',(22.4,1.45,38.));
#76322=CARTESIAN_POINT('',(23.3381365738089,1.60502390555561,42.269538656846));
#76323=CARTESIAN_POINT('Origin',(14.1732738814488,0.,0.));
#76324=CARTESIAN_POINT('',(23.1003542130464,1.05082556284928,38.0063506678963));
#76325=CARTESIAN_POINT('Origin',(23.1,1.05,38.));
#76326=CARTESIAN_POINT('',(24.1697957402248,1.35680204543028,42.2782342134758));
#76327=CARTESIAN_POINT('Origin',(8.01433437672608,0.,0.));
#76328=CARTESIAN_POINT('',(24.100209736014,0.75182343853507,38.01285608245));
#76329=CARTESIAN_POINT('Origin',(24.1,0.750000000000002,38.));
#76330=CARTESIAN_POINT('',(29.9005519666592,1.71315218706845,42.2652943865761));
#76331=CARTESIAN_POINT('Origin',(97.7155570771054,0.,0.));
#76332=CARTESIAN_POINT('',(30.4426385593966,1.2038882754343,38.408147857702));
#76333=CARTESIAN_POINT('Origin',(30.5,1.15,38.));
#76334=CARTESIAN_POINT('',(29.9040600247032,2.24593997529677,42.240333256585));
#76335=CARTESIAN_POINT('Origin',(35.8405517186909,0.,0.));
#76336=CARTESIAN_POINT('',(30.5047502791291,1.64524972087093,37.9662000077121));
#76337=CARTESIAN_POINT('Origin',(30.5,1.65,38.));
#76338=CARTESIAN_POINT('',(17.5,2.24593997529677,42.240333256585));
#76339=CARTESIAN_POINT('Origin',(17.5,2.61768253317747E-15,42.75));
#76340=CARTESIAN_POINT('Origin',(17.5,0.,0.));
#76341=CARTESIAN_POINT('',(0.600000000000001,6.04414326732376,41.8659567209931));
#76342=CARTESIAN_POINT('Origin',(0.600000000000001,0.,0.));
#76343=CARTESIAN_POINT('',(1.67735469196905,5.12313779357752,41.9886110647639));
#76344=CARTESIAN_POINT('Origin',(8.14497546096349,0.,0.));
#76345=CARTESIAN_POINT('',(5.09593997529677,5.12313779357752,41.9886110647639));
#76346=CARTESIAN_POINT('',(17.5,5.12313779357752,41.9886110647639));
#76347=CARTESIAN_POINT('',(5.09944803334083,5.65216579287046,41.9206753505941));
#76348=CARTESIAN_POINT('Origin',(-0.840551718690872,0.,0.));
#76349=CARTESIAN_POINT('',(10.8302042597752,6.00534915250319,41.8715390397407));
#76350=CARTESIAN_POINT('Origin',(-62.7155570771055,0.,0.));
#76351=CARTESIAN_POINT('',(11.6618634261911,5.75938837262207,41.9060788618227));
#76352=CARTESIAN_POINT('Origin',(26.9856656232739,0.,0.));
#76353=CARTESIAN_POINT('',(12.3548486633046,5.3691740737731,41.9578594516632));
#76354=CARTESIAN_POINT('Origin',(20.8267261185512,0.,0.));
#76355=CARTESIAN_POINT('',(13.103292255208,5.12313779357752,41.9886110647639));
#76356=CARTESIAN_POINT('Origin',(25.13830739299,0.,0.));
#76357=CARTESIAN_POINT('',(21.896707744792,5.12313779357752,41.9886110647639));
#76358=CARTESIAN_POINT('',(17.5,5.12313779357752,41.9886110647639));
#76359=CARTESIAN_POINT('',(22.6451513366954,5.3691740737731,41.9578594516632));
#76360=CARTESIAN_POINT('Origin',(9.86169260701005,0.,0.));
#76361=CARTESIAN_POINT('',(23.3381365738089,5.75938837262207,41.9060788618227));
#76362=CARTESIAN_POINT('Origin',(14.1732738814488,0.,0.));
#76363=CARTESIAN_POINT('',(24.1697957402248,6.00534915250319,41.8715390397407));
#76364=CARTESIAN_POINT('Origin',(8.01433437672607,0.,0.));
#76365=CARTESIAN_POINT('',(29.9005519666592,5.65216579287046,41.9206753505941));
#76366=CARTESIAN_POINT('Origin',(97.7155570771054,0.,0.));
#76367=CARTESIAN_POINT('',(29.9040600247032,5.12313779357752,41.9886110647639));
#76368=CARTESIAN_POINT('Origin',(35.8405517186909,0.,0.));
#76369=CARTESIAN_POINT('',(17.5,5.12313779357752,41.9886110647639));
#76370=CARTESIAN_POINT('Origin',(33.1,4.97369795887321,37.7092141076143));
#76371=CARTESIAN_POINT('',(30.5247014514712,4.96750374304977,37.5318349744051));
#76372=CARTESIAN_POINT('Origin',(30.5,4.97369795887321,37.7092141076143));
#76373=CARTESIAN_POINT('',(30.4955273645547,5.46749010626367,37.6544606275072));
#76374=CARTESIAN_POINT('Origin',(30.5,5.46610183537932,37.6223900187809));
#76375=CARTESIAN_POINT('',(24.1012882089558,5.86270716268919,37.6326386190063));
#76376=CARTESIAN_POINT('Origin',(24.1,5.8600249365842,37.5529307477141));
#76377=CARTESIAN_POINT('',(23.1004586919557,5.56495784004782,37.6133097693334));
#76378=CARTESIAN_POINT('Origin',(23.1,5.56458261068054,37.6050252010142));
#76379=CARTESIAN_POINT('',(22.399682944576,5.17040276961776,37.6689447622493));
#76380=CARTESIAN_POINT('Origin',(22.4,5.17065950947566,37.674484472081));
#76381=CARTESIAN_POINT('',(21.7998387845652,4.97344883706828,37.7020801925101));
#76382=CARTESIAN_POINT('Origin',(21.8,4.97369795887321,37.7092141076143));
#76383=CARTESIAN_POINT('',(13.2021921742626,4.97031045190415,37.6122086000507));
#76384=CARTESIAN_POINT('Origin',(13.2,4.97369795887321,37.7092141076143));
#76385=CARTESIAN_POINT('',(12.6002487187375,5.17045810616099,37.6701387661531));
#76386=CARTESIAN_POINT('Origin',(12.6,5.17065950947566,37.674484472081));
#76387=CARTESIAN_POINT('',(11.8996457869536,5.56487237189312,37.6114227454796));
#76388=CARTESIAN_POINT('Origin',(11.9,5.56458261068054,37.6050252010142));
#76389=CARTESIAN_POINT('',(10.899790263986,5.86046163546711,37.565908154163));
#76390=CARTESIAN_POINT('Origin',(10.9,5.8600249365842,37.5529307477141));
#76391=CARTESIAN_POINT('',(4.55736144060343,5.48390637564378,38.0336947942479));
#76392=CARTESIAN_POINT('Origin',(4.5,5.46610183537932,37.6223900187809));
#76393=CARTESIAN_POINT('',(4.49524972087093,4.97250676352255,37.6751027358433));
#76394=CARTESIAN_POINT('Origin',(4.5,4.97369795887321,37.7092141076143));
#76395=CARTESIAN_POINT('',(1.90350512467335,4.97134531440729,37.6418431848034));
#76396=CARTESIAN_POINT('Origin',(1.9,4.97369795887321,37.7092141076143));
#76397=CARTESIAN_POINT('Ctrl Pts',(0.138207714141615,6.43453435214071,42.2749056435377));
#76398=CARTESIAN_POINT('Ctrl Pts',(0.370217470897385,6.23839136562575,42.0700781197336));
#76399=CARTESIAN_POINT('Ctrl Pts',(0.600000000000003,6.04414326732376,41.8659567209931));
#76400=CARTESIAN_POINT('Origin',(1.9,8.2235635438135,37.1361751213135));
#76401=CARTESIAN_POINT('',(5.09593997529677,9.54677599452213,41.2086042970448));
#76402=CARTESIAN_POINT('',(17.5,9.54677599452213,41.2086042970448));
#76403=CARTESIAN_POINT('',(4.47529854852883,8.16871696615114,36.9673747121716));
#76404=CARTESIAN_POINT('Origin',(4.5,8.2235635438135,37.1361751213135));
#76405=CARTESIAN_POINT('',(5.09944803334083,9.02641690470011,41.325703839893));
#76406=CARTESIAN_POINT('Origin',(-0.840551718690874,0.,0.));
#76407=CARTESIAN_POINT('',(4.50447263544529,7.74082391359485,37.253610541118));
#76408=CARTESIAN_POINT('Origin',(4.5,7.7311596673074,37.2229992101469));
#76409=CARTESIAN_POINT('',(10.8302042597752,8.6777274997883,41.4003266344532));
#76410=CARTESIAN_POINT('Origin',(-62.7155570771055,0.,0.));
#76411=CARTESIAN_POINT('',(10.8987117910442,7.36197779558791,37.3682767550424));
#76412=CARTESIAN_POINT('Origin',(10.9,7.33723656610251,37.2924584812137));
#76413=CARTESIAN_POINT('',(11.6618634261911,8.92066834454427,41.3486599091995));
#76414=CARTESIAN_POINT('Origin',(26.9856656232739,0.,0.));
#76415=CARTESIAN_POINT('',(11.8995413080444,7.63515978098257,37.2482773116316));
#76416=CARTESIAN_POINT('Origin',(11.9,7.63267889200617,37.2403640279136));
#76417=CARTESIAN_POINT('',(12.3548486633046,9.30505984645652,41.2638565969525));
#76418=CARTESIAN_POINT('Origin',(20.8267261185512,0.,0.));
#76419=CARTESIAN_POINT('',(12.600317055424,8.02494855741037,37.1656113221937));
#76420=CARTESIAN_POINT('Origin',(12.6,8.02660199321106,37.1709047568469));
#76421=CARTESIAN_POINT('',(13.103292255208,9.54677599452213,41.2086042970448));
#76422=CARTESIAN_POINT('Origin',(25.13830739299,0.,0.));
#76423=CARTESIAN_POINT('',(13.2001612154348,8.22135769906884,37.1293862292573));
#76424=CARTESIAN_POINT('Origin',(13.2,8.2235635438135,37.1361751213135));
#76425=CARTESIAN_POINT('',(21.896707744792,9.54677599452213,41.2086042970448));
#76426=CARTESIAN_POINT('',(17.5,9.54677599452213,41.2086042970448));
#76427=CARTESIAN_POINT('',(21.7978078257374,8.19356892151488,37.0438611660612));
#76428=CARTESIAN_POINT('Origin',(21.8,8.2235635438135,37.1361751213135));
#76429=CARTESIAN_POINT('',(22.6451513366954,9.30505984645652,41.2638565969525));
#76430=CARTESIAN_POINT('Origin',(9.86169260701005,0.,0.));
#76431=CARTESIAN_POINT('',(22.3997512812625,8.02530493145534,37.1667522450638));
#76432=CARTESIAN_POINT('Origin',(22.4,8.02660199321106,37.1709047568469));
#76433=CARTESIAN_POINT('',(23.3381365738089,8.92066834454427,41.3486599091995));
#76434=CARTESIAN_POINT('Origin',(14.1732738814488,0.,0.));
#76435=CARTESIAN_POINT('',(23.1003542130464,7.6345946946079,37.2464748574103));
#76436=CARTESIAN_POINT('Origin',(23.1,7.63267889200617,37.2403640279136));
#76437=CARTESIAN_POINT('',(24.1697957402248,8.6777274997883,41.4003266344532));
#76438=CARTESIAN_POINT('Origin',(8.01433437672608,0.,0.));
#76439=CARTESIAN_POINT('',(24.100209736014,7.34126473779837,37.3048026141052));
#76440=CARTESIAN_POINT('Origin',(24.1,7.33723656610251,37.2924584812137));
#76441=CARTESIAN_POINT('',(29.9005519666592,9.02641690470011,41.325703839893));
#76442=CARTESIAN_POINT('Origin',(97.7155570771055,0.,0.));
#76443=CARTESIAN_POINT('',(30.4426385593966,7.85510339046017,37.6155887839604));
#76444=CARTESIAN_POINT('Origin',(30.5,7.7311596673074,37.2229992101469));
#76445=CARTESIAN_POINT('',(29.9040600247032,9.54677599452213,41.2086042970448));
#76446=CARTESIAN_POINT('Origin',(35.8405517186909,0.,0.));
#76447=CARTESIAN_POINT('',(30.5047502791291,8.21301612503228,37.1037135041708));
#76448=CARTESIAN_POINT('Origin',(30.5,8.2235635438135,37.1361751213135));
#76449=CARTESIAN_POINT('',(17.5,9.54677599452213,41.2086042970448));
#76450=CARTESIAN_POINT('Origin',(17.5,7.42345959526128,42.1005314412719));
#76451=CARTESIAN_POINT('Origin',(17.5,0.,0.));
#76452=CARTESIAN_POINT('',(0.600000000000001,13.22226624086,40.1803643021789));
#76453=CARTESIAN_POINT('Origin',(0.600000000000001,0.,0.));
#76454=CARTESIAN_POINT('',(1.67735469196905,12.3365516130268,40.4610861730024));
#76455=CARTESIAN_POINT('Origin',(8.14497546096349,0.,0.));
#76456=CARTESIAN_POINT('',(5.09593997529677,12.3365516130268,40.4610861730024));
#76457=CARTESIAN_POINT('',(17.5,12.3365516130268,40.4610861730024));
#76458=CARTESIAN_POINT('',(5.09944803334083,12.8457455753269,40.3023178069695));
#76459=CARTESIAN_POINT('Origin',(-0.840551718690872,0.,0.));
#76460=CARTESIAN_POINT('',(10.8302042597752,13.1850308552911,40.1925983403042));
#76461=CARTESIAN_POINT('Origin',(-62.7155570771055,0.,0.));
#76462=CARTESIAN_POINT('',(11.6618634261911,12.9488045494888,40.2693240660821));
#76463=CARTESIAN_POINT('Origin',(26.9856656232739,0.,0.));
#76464=CARTESIAN_POINT('',(12.3548486633046,12.5735100877104,40.3880779943072));
#76465=CARTESIAN_POINT('Origin',(20.8267261185512,0.,0.));
#76466=CARTESIAN_POINT('',(13.103292255208,12.3365516130268,40.4610861730024));
#76467=CARTESIAN_POINT('Origin',(25.13830739299,0.,0.));
#76468=CARTESIAN_POINT('',(21.896707744792,12.3365516130268,40.4610861730024));
#76469=CARTESIAN_POINT('',(17.5,12.3365516130268,40.4610861730024));
#76470=CARTESIAN_POINT('',(22.6451513366954,12.5735100877104,40.3880779943072));
#76471=CARTESIAN_POINT('Origin',(9.86169260701005,0.,0.));
#76472=CARTESIAN_POINT('',(23.3381365738089,12.9488045494888,40.2693240660821));
#76473=CARTESIAN_POINT('Origin',(14.1732738814488,0.,0.));
#76474=CARTESIAN_POINT('',(24.1697957402248,13.1850308552911,40.1925983403042));
#76475=CARTESIAN_POINT('Origin',(8.01433437672608,0.,0.));
#76476=CARTESIAN_POINT('',(29.9005519666592,12.8457455753269,40.3023178069695));
#76477=CARTESIAN_POINT('Origin',(97.7155570771054,0.,0.));
#76478=CARTESIAN_POINT('',(29.9040600247032,12.3365516130268,40.4610861730024));
#76479=CARTESIAN_POINT('Origin',(35.8405517186909,0.,0.));
#76480=CARTESIAN_POINT('',(17.5,12.3365516130268,40.4610861730024));
#76481=CARTESIAN_POINT('Origin',(33.1,11.4462726220787,36.2726528263519));
#76482=CARTESIAN_POINT('',(30.5247014514712,11.409370947074,36.0990440950346));
#76483=CARTESIAN_POINT('Origin',(30.5,11.4462726220787,36.2726528263519));
#76484=CARTESIAN_POINT('',(30.4955273645547,11.9230551151638,36.1329850680974));
#76485=CARTESIAN_POINT('Origin',(30.5,11.9161189324716,36.101642754689));
#76486=CARTESIAN_POINT('',(24.1012882089558,12.3084785844451,36.0428658633082));
#76487=CARTESIAN_POINT('Origin',(24.1,12.291995980786,35.9648346973588));
#76488=CARTESIAN_POINT('',(23.1004586919557,12.0118963235317,36.0755342895717));
#76489=CARTESIAN_POINT('Origin',(23.1,12.0100881945502,36.0674407403565));
#76490=CARTESIAN_POINT('',(22.399682944576,11.6329963463162,36.1988378309035));
#76491=CARTESIAN_POINT('Origin',(22.4,11.6342111462359,36.2042487976867));
#76492=CARTESIAN_POINT('',(21.7998387845652,11.4447884936362,36.2656705509953));
#76493=CARTESIAN_POINT('Origin',(21.8,11.4462726220787,36.2726528263519));
#76494=CARTESIAN_POINT('',(13.2021921742626,11.4260917493401,36.1777092848303));
#76495=CARTESIAN_POINT('Origin',(13.2,11.4462726220787,36.2726528263519));
#76496=CARTESIAN_POINT('',(12.6002487187375,11.633258178775,36.2000040861152));
#76497=CARTESIAN_POINT('Origin',(12.6,11.6342111462359,36.2042487976867));
#76498=CARTESIAN_POINT('',(11.8996457869536,12.0114844755768,36.0736907752397));
#76499=CARTESIAN_POINT('Origin',(11.9,12.0100881945502,36.0674407403565));
#76500=CARTESIAN_POINT('',(10.899790263986,12.2946795482123,35.9775391158784));
#76501=CARTESIAN_POINT('Origin',(10.9,12.291995980786,35.9648346973588));
#76502=CARTESIAN_POINT('',(4.55736144060343,12.0050753064884,36.5036071604488));
#76503=CARTESIAN_POINT('Origin',(4.5,11.9161189324716,36.101642754689));
#76504=CARTESIAN_POINT('',(4.49524972087093,11.4391761461162,36.2392665318678));
#76505=CARTESIAN_POINT('Origin',(4.5,11.4462726220787,36.2726528263519));
#76506=CARTESIAN_POINT('',(1.90350512467335,11.4322568815947,36.2067139516643));
#76507=CARTESIAN_POINT('Origin',(1.9,11.4462726220787,36.2726528263519));
#76508=CARTESIAN_POINT('Ctrl Pts',(0.138207714141621,13.6777396430533,40.515309671231));
#76509=CARTESIAN_POINT('Ctrl Pts',(0.370217470897303,13.4490085829899,40.3476538099289));
#76510=CARTESIAN_POINT('Ctrl Pts',(0.600000000000004,13.22226624086,40.1803643021789));
#76511=CARTESIAN_POINT('Origin',(1.9,14.5472582706722,35.1439863533772));
#76512=CARTESIAN_POINT('',(5.09593997529677,16.5575380560557,38.9247727484987));
#76513=CARTESIAN_POINT('',(17.5,16.5575380560557,38.9247727484987));
#76514=CARTESIAN_POINT('',(4.47529854852883,14.4639330523272,34.987274410005));
#76515=CARTESIAN_POINT('Origin',(4.5,14.5472582706722,35.1439863533772));
#76516=CARTESIAN_POINT('',(5.09944803334083,16.0654185122698,39.1304526938498));
#76517=CARTESIAN_POINT('Origin',(-0.840551718690874,0.,0.));
#76518=CARTESIAN_POINT('',(4.50447263544529,14.0922449867892,35.343464522354));
#76519=CARTESIAN_POINT('Origin',(4.5,14.0774119602792,35.31499642504));
#76520=CARTESIAN_POINT('',(10.8302042597752,15.7349845952072,39.2644910802189));
#76521=CARTESIAN_POINT('Origin',(-62.7155570771055,0.,0.));
#76522=CARTESIAN_POINT('',(10.8987117910442,13.7390659716653,35.5221746368434));
#76523=CARTESIAN_POINT('Origin',(10.9,13.7015349119648,35.4518044823703));
#76524=CARTESIAN_POINT('',(11.6618634261911,15.9652627899599,39.1714230536436));
#76525=CARTESIAN_POINT('Origin',(26.9856656232739,0.,0.));
#76526=CARTESIAN_POINT('',(11.8995413080444,13.9872600241959,35.35656070068));
#76527=CARTESIAN_POINT('Origin',(11.9,13.9834426982006,35.3491984393726));
#76528=CARTESIAN_POINT('',(12.3548486633046,16.3290885806033,39.0211592104439));
#76529=CARTESIAN_POINT('Origin',(20.8267261185512,0.,0.));
#76530=CARTESIAN_POINT('',(12.600317055424,14.3567722348383,35.2074644826695));
#76531=CARTESIAN_POINT('Origin',(12.6,14.359319746515,35.2123903820423));
#76532=CARTESIAN_POINT('',(13.103292255208,16.5575380560557,38.9247727484987));
#76533=CARTESIAN_POINT('Origin',(25.13830739299,0.,0.));
#76534=CARTESIAN_POINT('',(13.2001612154348,14.5439070589318,35.137683640766));
#76535=CARTESIAN_POINT('Origin',(13.2,14.5472582706722,35.1439863533772));
#76536=CARTESIAN_POINT('',(21.896707744792,16.5575380560557,38.9247727484987));
#76537=CARTESIAN_POINT('',(17.5,16.5575380560557,38.9247727484987));
#76538=CARTESIAN_POINT('',(21.7978078257374,14.501689183981,35.0582833660355));
#76539=CARTESIAN_POINT('Origin',(21.8,14.5472582706722,35.1439863533772));
#76540=CARTESIAN_POINT('',(22.6451513366954,16.3290885806033,39.0211592104439));
#76541=CARTESIAN_POINT('Origin',(9.86169260701006,0.,0.));
#76542=CARTESIAN_POINT('',(22.3997512812625,14.3573213139379,35.208526188654));
#76543=CARTESIAN_POINT('Origin',(22.4,14.359319746515,35.2123903820423));
#76544=CARTESIAN_POINT('',(23.3381365738089,15.9652627899599,39.1714230536436));
#76545=CARTESIAN_POINT('Origin',(14.1732738814488,0.,0.));
#76546=CARTESIAN_POINT('',(23.1003542130464,13.9863905298622,35.3548837560077));
#76547=CARTESIAN_POINT('Origin',(23.1,13.9834426982006,35.3491984393726));
#76548=CARTESIAN_POINT('',(24.1697957402248,15.7349845952072,39.2644910802189));
#76549=CARTESIAN_POINT('Origin',(8.01433437672608,0.,0.));
#76550=CARTESIAN_POINT('',(24.100209736014,13.7076454228629,35.4632615954717));
#76551=CARTESIAN_POINT('Origin',(24.1,13.7015349119648,35.4518044823703));
#76552=CARTESIAN_POINT('',(29.9005519666592,16.0654185122698,39.1304526938498));
#76553=CARTESIAN_POINT('Origin',(97.7155570771054,0.,0.));
#76554=CARTESIAN_POINT('',(30.4426385593966,14.267645163841,35.6800990794245));
#76555=CARTESIAN_POINT('Origin',(30.5,14.0774119602792,35.31499642504));
#76556=CARTESIAN_POINT('',(29.9040600247032,16.5575380560557,38.9247727484987));
#76557=CARTESIAN_POINT('Origin',(35.8405517186909,0.,0.));
#76558=CARTESIAN_POINT('',(30.5047502791291,14.5312341902212,35.1138494411902));
#76559=CARTESIAN_POINT('Origin',(30.5,14.5472582706722,35.1439863533772));
#76560=CARTESIAN_POINT('',(17.5,16.5575380560557,38.9247727484987));
#76561=CARTESIAN_POINT('Origin',(17.5,14.6213611271723,40.1718595385976));
#76562=CARTESIAN_POINT('Origin',(17.5,0.,0.));
#76563=CARTESIAN_POINT('',(0.600000000000001,19.9986373454573,37.2739118462884));
#76564=CARTESIAN_POINT('Origin',(0.600000000000001,0.,0.));
#76565=CARTESIAN_POINT('',(1.67735469196905,19.1751255543105,37.7041716521717));
#76566=CARTESIAN_POINT('Origin',(8.14497546096349,0.,0.));
#76567=CARTESIAN_POINT('',(5.09593997529677,19.1751255543105,37.7041716521717));
#76568=CARTESIAN_POINT('',(17.5,19.1751255543105,37.7041716521717));
#76569=CARTESIAN_POINT('',(5.09944803334083,19.6490138787379,37.459394730737));
#76570=CARTESIAN_POINT('Origin',(-0.840551718690872,0.,0.));
#76571=CARTESIAN_POINT('',(10.8302042597752,19.9640920674886,37.2924258787336));
#76572=CARTESIAN_POINT('Origin',(-62.7155570771055,0.,0.));
#76573=CARTESIAN_POINT('',(11.6618634261911,19.7447778525305,37.4090062358548));
#76574=CARTESIAN_POINT('Origin',(26.9856656232739,0.,0.));
#76575=CARTESIAN_POINT('',(12.3548486633046,19.3958063601357,37.5911252244478));
#76576=CARTESIAN_POINT('Origin',(20.8267261185512,0.,0.));
#76577=CARTESIAN_POINT('',(13.103292255208,19.1751255543105,37.7041716521717));
#76578=CARTESIAN_POINT('Origin',(25.13830739299,0.,0.));
#76579=CARTESIAN_POINT('',(21.896707744792,19.1751255543105,37.7041716521717));
#76580=CARTESIAN_POINT('',(17.5,19.1751255543105,37.7041716521717));
#76581=CARTESIAN_POINT('',(22.6451513366954,19.3958063601357,37.5911252244478));
#76582=CARTESIAN_POINT('Origin',(9.86169260701005,0.,0.));
#76583=CARTESIAN_POINT('',(23.3381365738089,19.7447778525305,37.4090062358548));
#76584=CARTESIAN_POINT('Origin',(14.1732738814488,0.,0.));
#76585=CARTESIAN_POINT('',(24.1697957402248,19.9640920674886,37.2924258787336));
#76586=CARTESIAN_POINT('Origin',(8.01433437672609,0.,0.));
#76587=CARTESIAN_POINT('',(29.9005519666592,19.6490138787379,37.459394730737));
#76588=CARTESIAN_POINT('Origin',(97.7155570771053,0.,0.));
#76589=CARTESIAN_POINT('',(29.9040600247032,19.1751255543105,37.7041716521717));
#76590=CARTESIAN_POINT('Origin',(35.8405517186909,0.,0.));
#76591=CARTESIAN_POINT('',(17.5,19.1751255543105,37.7041716521717));
#76592=CARTESIAN_POINT('Origin',(33.1,17.5710580837557,33.7339653438087));
#76593=CARTESIAN_POINT('',(30.5247014514712,17.5045701882916,33.5694020278343));
#76594=CARTESIAN_POINT('Origin',(30.5,17.5710580837557,33.7339653438087));
#76595=CARTESIAN_POINT('',(30.4955273645547,18.0163441277467,33.5136270415661));
#76596=CARTESIAN_POINT('Origin',(30.5,18.0040707856479,33.4839653438087));
#76597=CARTESIAN_POINT('',(24.1012882089558,18.3802631128034,33.3579488669236));
#76598=CARTESIAN_POINT('Origin',(24.1,18.3504809471617,33.2839653438087));
#76599=CARTESIAN_POINT('',(23.1004586919557,18.0938594155378,33.4416219555226));
#76600=CARTESIAN_POINT('Origin',(23.1,18.0906733260263,33.4339653438087));
#76601=CARTESIAN_POINT('',(22.399682944576,17.742127215612,33.6288475295615));
#76602=CARTESIAN_POINT('Origin',(22.4,17.7442631645126,33.6339653438087));
#76603=CARTESIAN_POINT('',(21.7998387845652,17.5683840431675,33.7273468611033));
#76604=CARTESIAN_POINT('Origin',(21.8,17.5710580837557,33.7339653438087));
#76605=CARTESIAN_POINT('',(13.2021921742626,17.5346970308537,33.6439685797946));
#76606=CARTESIAN_POINT('Origin',(13.2,17.5710580837557,33.7339653438087));
#76607=CARTESIAN_POINT('',(12.6002487187375,17.7425875883397,33.6299506000067));
#76608=CARTESIAN_POINT('Origin',(12.6,17.7442631645126,33.6339653438087));
#76609=CARTESIAN_POINT('',(11.8996457869536,18.0931337015746,33.4398779649625));
#76610=CARTESIAN_POINT('Origin',(11.9,18.0906733260263,33.4339653438087));
#76611=CARTESIAN_POINT('',(10.899790263986,18.3553298442931,33.2960107570711));
#76612=CARTESIAN_POINT('Origin',(10.9,18.3504809471617,33.2839653438087));
#76613=CARTESIAN_POINT('',(4.55736144060343,18.1614760990067,33.864375894796));
#76614=CARTESIAN_POINT('Origin',(4.5,18.0040707856479,33.4839653438087));
#76615=CARTESIAN_POINT('',(4.49524972087093,17.5582719500126,33.7023185522751));
#76616=CARTESIAN_POINT('Origin',(4.5,17.5710580837557,33.7339653438087));
#76617=CARTESIAN_POINT('',(1.90350512467335,17.5458051084359,33.6714620365851));
#76618=CARTESIAN_POINT('Origin',(1.9,17.5710580837557,33.7339653438087));
#76619=CARTESIAN_POINT('Ctrl Pts',(0.138207714141623,20.505353736182,37.5246765162999));
#76620=CARTESIAN_POINT('Ctrl Pts',(0.370217470902976,20.2509844800803,37.3992864560044));
#76621=CARTESIAN_POINT('Ctrl Pts',(0.600000000000002,19.9986373454573,37.2739118462884));
#76622=CARTESIAN_POINT('Origin',(1.9,20.4289419162443,32.0839653438087));
#76623=CARTESIAN_POINT('',(5.09593997529677,23.0652077022745,35.4582316768749));
#76624=CARTESIAN_POINT('',(17.5,23.0652077022745,35.4582316768749));
#76625=CARTESIAN_POINT('',(4.47529854852883,20.3196698518115,31.9441034793054));
#76626=CARTESIAN_POINT('Origin',(4.5,20.4289419162443,32.0839653438087));
#76627=CARTESIAN_POINT('',(5.09944803334083,22.6162805078382,35.7462425436685));
#76628=CARTESIAN_POINT('Origin',(-0.840551718690874,0.,0.));
#76629=CARTESIAN_POINT('',(4.50447263544529,20.01548032708,32.3594252187343));
#76630=CARTESIAN_POINT('Origin',(4.5,19.9959292143521,32.3339653438087));
#76631=CARTESIAN_POINT('',(10.8302042597752,22.3141421459872,35.9356238333033));
#76632=CARTESIAN_POINT('Origin',(-62.7155570771054,0.,0.));
#76633=CARTESIAN_POINT('',(10.8987117910442,19.6986995804965,32.5967492173916));
#76634=CARTESIAN_POINT('Origin',(10.9,19.6495190528383,32.5339653438087));
#76635=CARTESIAN_POINT('',(11.6618634261911,22.5247608043155,35.8039823302991));
#76636=CARTESIAN_POINT('Origin',(26.9856656232739,0.,0.));
#76637=CARTESIAN_POINT('',(11.8995413080444,19.9143644494692,32.3905528841213));
#76638=CARTESIAN_POINT('Origin',(11.9,19.9093266739737,32.3839653438087));
#76639=CARTESIAN_POINT('',(12.3548486633046,22.856966221146,35.5928236469852));
#76640=CARTESIAN_POINT('Origin',(20.8267261185512,0.,0.));
#76641=CARTESIAN_POINT('',(12.600317055424,20.2523726527879,32.1795566506761));
#76642=CARTESIAN_POINT('Origin',(12.6,20.2557368354874,32.1839653438087));
#76643=CARTESIAN_POINT('',(13.103292255208,23.0652077022745,35.4582316768749));
#76644=CARTESIAN_POINT('Origin',(25.13830739299,0.,0.));
#76645=CARTESIAN_POINT('',(13.2001612154348,20.4245471623811,32.0783403153759));
#76646=CARTESIAN_POINT('Origin',(13.2,20.4289419162443,32.0839653438087));
#76647=CARTESIAN_POINT('',(21.896707744792,23.0652077022745,35.4582316768749));
#76648=CARTESIAN_POINT('',(17.5,23.0652077022745,35.4582316768749));
#76649=CARTESIAN_POINT('',(21.7978078257374,20.3691829588007,32.0074773662801));
#76650=CARTESIAN_POINT('Origin',(21.8,20.4289419162443,32.0839653438087));
#76651=CARTESIAN_POINT('',(22.6451513366954,22.856966221146,35.5928236469852));
#76652=CARTESIAN_POINT('Origin',(9.86169260701004,0.,0.));
#76653=CARTESIAN_POINT('',(22.3997512812625,20.2530977534517,32.180506880376));
#76654=CARTESIAN_POINT('Origin',(22.4,20.2557368354874,32.1839653438087));
#76655=CARTESIAN_POINT('',(23.3381365738089,22.5247608043155,35.8039823302992));
#76656=CARTESIAN_POINT('Origin',(14.1732738814488,0.,0.));
#76657=CARTESIAN_POINT('',(23.1003542130464,19.9132169663217,32.3890524021132));
#76658=CARTESIAN_POINT('Origin',(23.1,19.9093266739737,32.3839653438087));
#76659=CARTESIAN_POINT('',(24.1697957402248,22.3141421459872,35.9356238333033));
#76660=CARTESIAN_POINT('Origin',(8.01433437672608,0.,0.));
#76661=CARTESIAN_POINT('',(24.100209736014,19.657526238157,32.544187318536));
#76662=CARTESIAN_POINT('Origin',(24.1,19.6495190528383,32.5339653438087));
#76663=CARTESIAN_POINT('',(29.9005519666592,22.6162805078382,35.7462425436685));
#76664=CARTESIAN_POINT('Origin',(97.7155570771054,0.,0.));
#76665=CARTESIAN_POINT('',(30.4426385593966,20.2466717586954,32.6604876193617));
#76666=CARTESIAN_POINT('Origin',(30.5,19.9959292143521,32.3339653438087));
#76667=CARTESIAN_POINT('',(29.9040600247032,23.0652077022745,35.4582316768749));
#76668=CARTESIAN_POINT('Origin',(35.8405517186909,0.,0.));
#76669=CARTESIAN_POINT('',(30.5047502791291,20.4079280576996,32.0570688314042));
#76670=CARTESIAN_POINT('Origin',(30.5,20.4289419162443,32.0839653438087));
#76671=CARTESIAN_POINT('',(17.5,23.0652077022745,35.4582316768749));
#76672=CARTESIAN_POINT('Origin',(17.5,21.375,37.0225860117847));
#76673=CARTESIAN_POINT('Origin',(17.5,0.,0.));
#76674=CARTESIAN_POINT('',(0.600000000000001,26.1673599741116,33.234910440458));
#76675=CARTESIAN_POINT('Origin',(0.600000000000001,0.,0.));
#76676=CARTESIAN_POINT('',(1.67735469196904,25.4310730087083,33.8016349549212));
#76677=CARTESIAN_POINT('Origin',(8.14497546096349,0.,0.));
#76678=CARTESIAN_POINT('',(5.09593997529677,25.4310730087083,33.8016349549212));
#76679=CARTESIAN_POINT('',(17.5,25.4310730087083,33.8016349549212));
#76680=CARTESIAN_POINT('',(5.09944803334083,25.8552568383243,33.4782869009794));
#76681=CARTESIAN_POINT('Origin',(-0.840551718690872,0.,0.));
#76682=CARTESIAN_POINT('',(10.8302042597752,26.1365544445335,33.2591419277157));
#76683=CARTESIAN_POINT('Origin',(-62.7155570771055,0.,0.));
#76684=CARTESIAN_POINT('',(11.6618634261911,25.9408160718628,33.4120346810215));
#76685=CARTESIAN_POINT('Origin',(26.9856656232739,0.,0.));
#76686=CARTESIAN_POINT('',(12.3548486633046,25.6287708710599,33.6519851366708));
#76687=CARTESIAN_POINT('Origin',(20.8267261185512,0.,0.));
#76688=CARTESIAN_POINT('',(13.103292255208,25.4310730087083,33.8016349549212));
#76689=CARTESIAN_POINT('Origin',(25.13830739299,0.,0.));
#76690=CARTESIAN_POINT('',(21.896707744792,25.4310730087083,33.8016349549212));
#76691=CARTESIAN_POINT('',(17.5,25.4310730087083,33.8016349549212));
#76692=CARTESIAN_POINT('',(22.6451513366954,25.6287708710599,33.6519851366708));
#76693=CARTESIAN_POINT('Origin',(9.86169260701005,0.,0.));
#76694=CARTESIAN_POINT('',(23.3381365738089,25.9408160718628,33.4120346810215));
#76695=CARTESIAN_POINT('Origin',(14.1732738814488,0.,0.));
#76696=CARTESIAN_POINT('',(24.1697957402248,26.1365544445335,33.2591419277157));
#76697=CARTESIAN_POINT('Origin',(8.0143343767261,0.,0.));
#76698=CARTESIAN_POINT('',(29.9005519666592,25.8552568383243,33.4782869009794));
#76699=CARTESIAN_POINT('Origin',(97.7155570771055,0.,0.));
#76700=CARTESIAN_POINT('',(29.9040600247032,25.4310730087083,33.8016349549212));
#76701=CARTESIAN_POINT('Origin',(35.8405517186909,0.,0.));
#76702=CARTESIAN_POINT('',(17.5,25.4310730087083,33.8016349549212));
#76703=CARTESIAN_POINT('Origin',(33.1,23.1619558369422,30.170288394504));
#76704=CARTESIAN_POINT('',(30.5247014514712,23.0679019220779,30.0197706669552));
#76705=CARTESIAN_POINT('Origin',(30.5,23.1619558369422,30.170288394504));
#76706=CARTESIAN_POINT('',(30.4955273645547,23.562215640718,29.8759744160904));
#76707=CARTESIAN_POINT('Origin',(30.5,23.5449780585017,29.8488945896607));
#76708=CARTESIAN_POINT('',(24.1012882089558,23.893572647341,29.6594674741542));
#76709=CARTESIAN_POINT('Origin',(24.1,23.8513958357493,29.5917795457861));
#76710=CARTESIAN_POINT('',(23.1004586919557,23.6260497451375,29.7916028606322));
#76711=CARTESIAN_POINT('Origin',(23.1,23.6215825028136,29.784615828692));
#76712=CARTESIAN_POINT('',(22.399682944576,23.312172527411,30.0370617130518));
#76713=CARTESIAN_POINT('Origin',(22.4,23.315164725566,30.0417308725666));
#76714=CARTESIAN_POINT('',(21.7998387845652,23.1581731335784,30.1642348036977));
#76715=CARTESIAN_POINT('Origin',(21.8,23.1619558369422,30.170288394504));
#76716=CARTESIAN_POINT('',(13.2021921742626,23.1105194160696,30.0879729141313));
#76717=CARTESIAN_POINT('Origin',(13.2,23.1619558369422,30.170288394504));
#76718=CARTESIAN_POINT('',(12.6002487187375,23.3128174522151,30.038068082493));
#76719=CARTESIAN_POINT('Origin',(12.6,23.315164725566,30.0417308725666));
#76720=CARTESIAN_POINT('',(11.8996457869536,23.6250322156174,29.7900113841146));
#76721=CARTESIAN_POINT('Origin',(11.9,23.6215825028136,29.784615828692));
#76722=CARTESIAN_POINT('',(10.899790263986,23.8582627313001,29.6027999600046));
#76723=CARTESIAN_POINT('Origin',(10.9,23.8513958357493,29.5917795457861));
#76724=CARTESIAN_POINT('',(4.55736144060343,23.7660496304069,30.1961927037808));
#76725=CARTESIAN_POINT('Origin',(4.5,23.5449780585017,29.8488945896607));
#76726=CARTESIAN_POINT('',(4.49524972087093,23.1438685456221,30.1413426776677));
#76727=CARTESIAN_POINT('Origin',(4.5,23.1619558369422,30.170288394504));
#76728=CARTESIAN_POINT('',(1.90350512467335,23.1262329256631,30.1131197861062));
#76729=CARTESIAN_POINT('Origin',(1.9,23.1619558369422,30.170288394504));
#76730=CARTESIAN_POINT('Ctrl Pts',(0.138207714141625,26.7099230322463,33.3938750538235));
#76731=CARTESIAN_POINT('Ctrl Pts',(0.370217470894606,26.4376444612514,33.3145607080732));
#76732=CARTESIAN_POINT('Ctrl Pts',(0.600000000000002,26.1673599741116,33.234910440458));
#76733=CARTESIAN_POINT('Origin',(1.9,25.6899024992348,28.0490892825384));
#76734=CARTESIAN_POINT('',(5.09593997529677,28.872052684018,30.9143101784803));
#76735=CARTESIAN_POINT('',(17.5,28.872052684018,30.9143101784803));
#76736=CARTESIAN_POINT('',(4.47529854852883,25.5580037650976,27.9303271288835));
#76737=CARTESIAN_POINT('Origin',(4.5,25.6899024992348,28.0490892825384));
#76738=CARTESIAN_POINT('',(5.09944803334083,28.4799582645661,31.2759009022694));
#76739=CARTESIAN_POINT('Origin',(-0.840551718690874,0.,0.));
#76740=CARTESIAN_POINT('',(4.50447263544529,25.3305554259542,28.3921611545025));
#76741=CARTESIAN_POINT('Origin',(4.5,25.3068802776753,28.3704830873816));
#76742=CARTESIAN_POINT('',(10.8302042597752,28.2152957791621,31.5148708405159));
#76743=CARTESIAN_POINT('Origin',(-62.7155570771054,0.,0.));
#76744=CARTESIAN_POINT('',(10.8987117910442,25.0597981705973,28.6808880677203));
#76745=CARTESIAN_POINT('Origin',(10.9,25.0004625004277,28.6275981312563));
#76746=CARTESIAN_POINT('',(11.6618634261911,28.3998553597108,31.3486557215378));
#76747=CARTESIAN_POINT('Origin',(26.9856656232739,0.,0.));
#76748=CARTESIAN_POINT('',(11.8995413080444,25.2363809880999,28.4403745085892));
#76749=CARTESIAN_POINT('Origin',(11.9,25.2302758333634,28.4347618483503));
#76750=CARTESIAN_POINT('',(12.3548486633046,28.6903465092421,31.0830181478507));
#76751=CARTESIAN_POINT('Origin',(20.8267261185512,0.,0.));
#76752=CARTESIAN_POINT('',(12.600317055424,25.5326149758775,28.1738892734932));
#76753=CARTESIAN_POINT('Origin',(12.6,25.536693610611,28.1776468044757));
#76754=CARTESIAN_POINT('',(13.103292255208,28.872052684018,30.9143101784803));
#76755=CARTESIAN_POINT('Origin',(25.13830739299,0.,0.));
#76756=CARTESIAN_POINT('',(13.2001612154348,25.684597735621,28.0443128519265));
#76757=CARTESIAN_POINT('Origin',(13.2,25.6899024992348,28.0490892825384));
#76758=CARTESIAN_POINT('',(21.896707744792,28.872052684018,30.9143101784803));
#76759=CARTESIAN_POINT('',(17.5,28.872052684018,30.9143101784803));
#76760=CARTESIAN_POINT('',(21.7978078257374,25.6177694167211,27.9841403633154));
#76761=CARTESIAN_POINT('Origin',(21.8,25.6899024992348,28.0490892825384));
#76762=CARTESIAN_POINT('',(22.6451513366954,28.6903465092421,31.0830181478507));
#76763=CARTESIAN_POINT('Origin',(9.86169260701003,0.,0.));
#76764=CARTESIAN_POINT('',(22.3997512812625,25.5334940662887,28.1746991546599));
#76765=CARTESIAN_POINT('Origin',(22.4,25.536693610611,28.1776468044757));
#76766=CARTESIAN_POINT('',(23.3381365738089,28.3998553597108,31.3486557215378));
#76767=CARTESIAN_POINT('Origin',(14.1732738814488,0.,0.));
#76768=CARTESIAN_POINT('',(23.1003542130464,25.2349903818335,28.4390960806318));
#76769=CARTESIAN_POINT('Origin',(23.1,25.2302758333634,28.4347618483503));
#76770=CARTESIAN_POINT('',(24.1697957402248,28.2152957791621,31.5148708405159));
#76771=CARTESIAN_POINT('Origin',(8.01433437672607,0.,0.));
#76772=CARTESIAN_POINT('',(24.100209736014,25.0101230658929,28.63627437808));
#76773=CARTESIAN_POINT('Origin',(24.1,25.0004625004277,28.6275981312563));
#76774=CARTESIAN_POINT('',(29.9005519666592,28.4799582645661,31.2759009022694));
#76775=CARTESIAN_POINT('Origin',(97.7155570771054,0.,0.));
#76776=CARTESIAN_POINT('',(30.4426385593966,25.610513477472,28.6485037699886));
#76777=CARTESIAN_POINT('Origin',(30.5,25.3068802776753,28.3704830873816));
#76778=CARTESIAN_POINT('',(29.9040600247032,28.872052684018,30.9143101784803));
#76779=CARTESIAN_POINT('Origin',(35.8405517186909,0.,0.));
#76780=CARTESIAN_POINT('',(30.5047502791291,25.6645373580546,28.0262504068355));
#76781=CARTESIAN_POINT('Origin',(30.5,25.6899024992348,28.0490892825384));
#76782=CARTESIAN_POINT('',(17.5,28.872052684018,30.9143101784803));
#76783=CARTESIAN_POINT('Origin',(17.5,27.4791703140996,32.7483999433363));
#76784=CARTESIAN_POINT('Origin',(17.5,0.,0.));
#76785=CARTESIAN_POINT('',(0.600000000000001,31.5410006112756,28.1860830985703));
#76786=CARTESIAN_POINT('Origin',(0.600000000000001,0.,0.));
#76787=CARTESIAN_POINT('',(1.67735469196904,30.9143101784803,28.872052684018));
#76788=CARTESIAN_POINT('Origin',(8.14497546096349,0.,0.));
#76789=CARTESIAN_POINT('',(5.09593997529677,30.9143101784803,28.872052684018));
#76790=CARTESIAN_POINT('',(17.5,30.9143101784803,28.872052684018));
#76791=CARTESIAN_POINT('',(5.09944803334083,31.2759009022694,28.4799582645661));
#76792=CARTESIAN_POINT('Origin',(-0.840551718690872,0.,0.));
#76793=CARTESIAN_POINT('',(10.8302042597752,31.5148708405159,28.2152957791621));
#76794=CARTESIAN_POINT('Origin',(-62.7155570771055,0.,0.));
#76795=CARTESIAN_POINT('',(11.6618634261911,31.3486557215378,28.3998553597108));
#76796=CARTESIAN_POINT('Origin',(26.9856656232739,0.,0.));
#76797=CARTESIAN_POINT('',(12.3548486633046,31.0830181478507,28.6903465092421));
#76798=CARTESIAN_POINT('Origin',(20.8267261185512,0.,0.));
#76799=CARTESIAN_POINT('',(13.103292255208,30.9143101784803,28.872052684018));
#76800=CARTESIAN_POINT('Origin',(25.13830739299,0.,0.));
#76801=CARTESIAN_POINT('',(21.896707744792,30.9143101784803,28.872052684018));
#76802=CARTESIAN_POINT('',(17.5,30.9143101784803,28.872052684018));
#76803=CARTESIAN_POINT('',(22.6451513366954,31.0830181478507,28.6903465092421));
#76804=CARTESIAN_POINT('Origin',(9.86169260701006,0.,0.));
#76805=CARTESIAN_POINT('',(23.3381365738089,31.3486557215378,28.3998553597108));
#76806=CARTESIAN_POINT('Origin',(14.1732738814488,0.,0.));
#76807=CARTESIAN_POINT('',(24.1697957402248,31.5148708405159,28.2152957791621));
#76808=CARTESIAN_POINT('Origin',(8.01433437672608,0.,0.));
#76809=CARTESIAN_POINT('',(29.9005519666592,31.2759009022694,28.4799582645661));
#76810=CARTESIAN_POINT('Origin',(97.7155570771054,0.,0.));
#76811=CARTESIAN_POINT('',(29.9040600247032,30.9143101784803,28.872052684018));
#76812=CARTESIAN_POINT('Origin',(35.8405517186909,0.,0.));
#76813=CARTESIAN_POINT('',(17.5,30.9143101784803,28.872052684018));
#76814=CARTESIAN_POINT('Origin',(33.1,28.0490892825384,25.6899024992348));
#76815=CARTESIAN_POINT('',(30.5247014514712,27.9303271288835,25.5580037650976));
#76816=CARTESIAN_POINT('Origin',(30.5,28.0490892825384,25.6899024992348));
#76817=CARTESIAN_POINT('',(30.4955273645547,28.3921611545025,25.3305554259542));
#76818=CARTESIAN_POINT('Origin',(30.5,28.3704830873816,25.3068802776753));
#76819=CARTESIAN_POINT('',(24.1012882089558,28.6808880677203,25.0597981705973));
#76820=CARTESIAN_POINT('Origin',(24.1,28.6275981312563,25.0004625004277));
#76821=CARTESIAN_POINT('',(23.1004586919557,28.4403745085892,25.2363809880999));
#76822=CARTESIAN_POINT('Origin',(23.1,28.4347618483503,25.2302758333634));
#76823=CARTESIAN_POINT('',(22.399682944576,28.1738892734932,25.5326149758775));
#76824=CARTESIAN_POINT('Origin',(22.4,28.1776468044757,25.536693610611));
#76825=CARTESIAN_POINT('',(21.7998387845652,28.0443128519265,25.684597735621));
#76826=CARTESIAN_POINT('Origin',(21.8,28.0490892825384,25.6899024992348));
#76827=CARTESIAN_POINT('',(13.2021921742626,27.9841403633154,25.6177694167211));
#76828=CARTESIAN_POINT('Origin',(13.2,28.0490892825384,25.6899024992348));
#76829=CARTESIAN_POINT('',(12.6002487187375,28.1746991546599,25.5334940662887));
#76830=CARTESIAN_POINT('Origin',(12.6,28.1776468044757,25.536693610611));
#76831=CARTESIAN_POINT('',(11.8996457869536,28.4390960806318,25.2349903818335));
#76832=CARTESIAN_POINT('Origin',(11.9,28.4347618483503,25.2302758333634));
#76833=CARTESIAN_POINT('',(10.899790263986,28.63627437808,25.0101230658929));
#76834=CARTESIAN_POINT('Origin',(10.9,28.6275981312563,25.0004625004277));
#76835=CARTESIAN_POINT('',(4.55736144060343,28.6485037699886,25.610513477472));
#76836=CARTESIAN_POINT('Origin',(4.5,28.3704830873816,25.3068802776753));
#76837=CARTESIAN_POINT('',(4.49524972087093,28.0262504068355,25.6645373580546));
#76838=CARTESIAN_POINT('Origin',(4.5,28.0490892825384,25.6899024992348));
#76839=CARTESIAN_POINT('',(1.90350512467335,28.0039818578826,25.6398056289004));
#76840=CARTESIAN_POINT('Origin',(1.9,28.0490892825384,25.6899024992348));
#76841=CARTESIAN_POINT('Ctrl Pts',(0.138207714141624,32.1029248328492,28.2484175959527));
#76842=CARTESIAN_POINT('Ctrl Pts',(0.370217470898456,31.8210099935472,28.2175888910033));
#76843=CARTESIAN_POINT('Ctrl Pts',(0.600000000000002,31.5410006112756,28.1860830985703));
#76844=CARTESIAN_POINT('Origin',(1.9,30.170288394504,23.1619558369422));
#76845=CARTESIAN_POINT('',(5.09593997529677,33.8016349549212,25.4310730087083));
#76846=CARTESIAN_POINT('',(17.5,33.8016349549212,25.4310730087083));
#76847=CARTESIAN_POINT('',(4.47529854852883,30.0197706669552,23.0679019220779));
#76848=CARTESIAN_POINT('Origin',(4.5,30.170288394504,23.1619558369422));
#76849=CARTESIAN_POINT('',(5.09944803334083,33.4782869009794,25.8552568383243));
#76850=CARTESIAN_POINT('Origin',(-0.840551718690874,0.,0.));
#76851=CARTESIAN_POINT('',(4.50447263544529,29.8759744160904,23.562215640718));
#76852=CARTESIAN_POINT('Origin',(4.5,29.8488945896607,23.5449780585017));
#76853=CARTESIAN_POINT('',(10.8302042597752,33.2591419277157,26.1365544445334));
#76854=CARTESIAN_POINT('Origin',(-62.7155570771055,0.,0.));
#76855=CARTESIAN_POINT('',(10.8987117910442,29.6594674741542,23.893572647341));
#76856=CARTESIAN_POINT('Origin',(10.9,29.5917795457861,23.8513958357493));
#76857=CARTESIAN_POINT('',(11.6618634261911,33.4120346810215,25.9408160718628));
#76858=CARTESIAN_POINT('Origin',(26.9856656232739,0.,0.));
#76859=CARTESIAN_POINT('',(11.8995413080444,29.7916028606322,23.6260497451375));
#76860=CARTESIAN_POINT('Origin',(11.9,29.784615828692,23.6215825028136));
#76861=CARTESIAN_POINT('',(12.3548486633046,33.6519851366708,25.6287708710599));
#76862=CARTESIAN_POINT('Origin',(20.8267261185512,0.,0.));
#76863=CARTESIAN_POINT('',(12.600317055424,30.0370617130518,23.312172527411));
#76864=CARTESIAN_POINT('Origin',(12.6,30.0417308725667,23.315164725566));
#76865=CARTESIAN_POINT('',(13.103292255208,33.8016349549212,25.4310730087083));
#76866=CARTESIAN_POINT('Origin',(25.13830739299,0.,0.));
#76867=CARTESIAN_POINT('',(13.2001612154348,30.1642348036977,23.1581731335784));
#76868=CARTESIAN_POINT('Origin',(13.2,30.170288394504,23.1619558369422));
#76869=CARTESIAN_POINT('',(21.896707744792,33.8016349549212,25.4310730087083));
#76870=CARTESIAN_POINT('',(17.5,33.8016349549212,25.4310730087083));
#76871=CARTESIAN_POINT('',(21.7978078257374,30.0879729141313,23.1105194160696));
#76872=CARTESIAN_POINT('Origin',(21.8,30.170288394504,23.1619558369422));
#76873=CARTESIAN_POINT('',(22.6451513366954,33.6519851366708,25.6287708710599));
#76874=CARTESIAN_POINT('Origin',(9.86169260701005,0.,0.));
#76875=CARTESIAN_POINT('',(22.3997512812625,30.0380680824931,23.3128174522151));
#76876=CARTESIAN_POINT('Origin',(22.4,30.0417308725667,23.315164725566));
#76877=CARTESIAN_POINT('',(23.3381365738089,33.4120346810215,25.9408160718628));
#76878=CARTESIAN_POINT('Origin',(14.1732738814488,0.,0.));
#76879=CARTESIAN_POINT('',(23.1003542130464,29.7900113841146,23.6250322156174));
#76880=CARTESIAN_POINT('Origin',(23.1,29.784615828692,23.6215825028136));
#76881=CARTESIAN_POINT('',(24.1697957402248,33.2591419277157,26.1365544445335));
#76882=CARTESIAN_POINT('Origin',(8.01433437672607,0.,0.));
#76883=CARTESIAN_POINT('',(24.100209736014,29.6027999600046,23.8582627313001));
#76884=CARTESIAN_POINT('Origin',(24.1,29.5917795457861,23.8513958357493));
#76885=CARTESIAN_POINT('',(29.9005519666592,33.4782869009794,25.8552568383243));
#76886=CARTESIAN_POINT('Origin',(97.7155570771054,0.,0.));
#76887=CARTESIAN_POINT('',(30.4426385593966,30.1961927037808,23.7660496304069));
#76888=CARTESIAN_POINT('Origin',(30.5,29.8488945896607,23.5449780585017));
#76889=CARTESIAN_POINT('',(29.9040600247032,33.8016349549212,25.4310730087083));
#76890=CARTESIAN_POINT('Origin',(35.8405517186909,0.,0.));
#76891=CARTESIAN_POINT('',(30.5047502791291,30.1413426776677,23.1438685456221));
#76892=CARTESIAN_POINT('Origin',(30.5,30.170288394504,23.1619558369422));
#76893=CARTESIAN_POINT('',(17.5,33.8016349549212,25.4310730087083));
#76894=CARTESIAN_POINT('Origin',(17.5,32.7483999433363,27.4791703140996));
#76895=CARTESIAN_POINT('Origin',(17.5,0.,0.));
#76896=CARTESIAN_POINT('',(0.600000000000001,35.9562839053824,22.2808358845789));
#76897=CARTESIAN_POINT('Origin',(0.600000000000001,0.,0.));
#76898=CARTESIAN_POINT('',(1.67735469196904,35.4582316768749,23.0652077022745));
#76899=CARTESIAN_POINT('Origin',(8.14497546096349,0.,0.));
#76900=CARTESIAN_POINT('',(5.09593997529677,35.4582316768749,23.0652077022745));
#76901=CARTESIAN_POINT('',(17.5,35.4582316768749,23.0652077022745));
#76902=CARTESIAN_POINT('',(5.09944803334083,35.7462425436685,22.6162805078382));
#76903=CARTESIAN_POINT('Origin',(-0.840551718690872,0.,0.));
#76904=CARTESIAN_POINT('',(10.8302042597752,35.9356238333033,22.3141421459872));
#76905=CARTESIAN_POINT('Origin',(-62.7155570771055,0.,0.));
#76906=CARTESIAN_POINT('',(11.6618634261911,35.8039823302991,22.5247608043155));
#76907=CARTESIAN_POINT('Origin',(26.9856656232739,0.,0.));
#76908=CARTESIAN_POINT('',(12.3548486633046,35.5928236469852,22.856966221146));
#76909=CARTESIAN_POINT('Origin',(20.8267261185512,0.,0.));
#76910=CARTESIAN_POINT('',(13.103292255208,35.4582316768749,23.0652077022745));
#76911=CARTESIAN_POINT('Origin',(25.13830739299,0.,0.));
#76912=CARTESIAN_POINT('',(21.896707744792,35.4582316768749,23.0652077022745));
#76913=CARTESIAN_POINT('',(17.5,35.4582316768749,23.0652077022745));
#76914=CARTESIAN_POINT('',(22.6451513366954,35.5928236469852,22.856966221146));
#76915=CARTESIAN_POINT('Origin',(9.86169260701005,0.,0.));
#76916=CARTESIAN_POINT('',(23.3381365738089,35.8039823302992,22.5247608043155));
#76917=CARTESIAN_POINT('Origin',(14.1732738814488,0.,0.));
#76918=CARTESIAN_POINT('',(24.1697957402248,35.9356238333033,22.3141421459872));
#76919=CARTESIAN_POINT('Origin',(8.01433437672608,0.,0.));
#76920=CARTESIAN_POINT('',(29.9005519666592,35.7462425436685,22.6162805078382));
#76921=CARTESIAN_POINT('Origin',(97.7155570771054,0.,0.));
#76922=CARTESIAN_POINT('',(29.9040600247032,35.4582316768749,23.0652077022745));
#76923=CARTESIAN_POINT('Origin',(35.8405517186909,0.,0.));
#76924=CARTESIAN_POINT('',(17.5,35.4582316768749,23.0652077022745));
#76925=CARTESIAN_POINT('Origin',(33.1,32.0839653438087,20.4289419162443));
#76926=CARTESIAN_POINT('',(30.5247014514712,31.9441034793054,20.3196698518115));
#76927=CARTESIAN_POINT('Origin',(30.5,32.0839653438087,20.4289419162443));
#76928=CARTESIAN_POINT('',(30.4955273645547,32.3594252187343,20.01548032708));
#76929=CARTESIAN_POINT('Origin',(30.5,32.3339653438087,19.9959292143521));
#76930=CARTESIAN_POINT('',(24.1012882089558,32.5967492173916,19.6986995804965));
#76931=CARTESIAN_POINT('Origin',(24.1,32.5339653438087,19.6495190528383));
#76932=CARTESIAN_POINT('',(23.1004586919557,32.3905528841213,19.9143644494691));
#76933=CARTESIAN_POINT('Origin',(23.1,32.3839653438087,19.9093266739737));
#76934=CARTESIAN_POINT('',(22.399682944576,32.1795566506761,20.2523726527878));
#76935=CARTESIAN_POINT('Origin',(22.4,32.1839653438087,20.2557368354874));
#76936=CARTESIAN_POINT('',(21.7998387845652,32.0783403153759,20.4245471623811));
#76937=CARTESIAN_POINT('Origin',(21.8,32.0839653438087,20.4289419162443));
#76938=CARTESIAN_POINT('',(13.2021921742626,32.0074773662801,20.3691829588007));
#76939=CARTESIAN_POINT('Origin',(13.2,32.0839653438087,20.4289419162443));
#76940=CARTESIAN_POINT('',(12.6002487187375,32.180506880376,20.2530977534517));
#76941=CARTESIAN_POINT('Origin',(12.6,32.1839653438087,20.2557368354874));
#76942=CARTESIAN_POINT('',(11.8996457869536,32.3890524021132,19.9132169663217));
#76943=CARTESIAN_POINT('Origin',(11.9,32.3839653438087,19.9093266739737));
#76944=CARTESIAN_POINT('',(10.899790263986,32.544187318536,19.6575262381569));
#76945=CARTESIAN_POINT('Origin',(10.9,32.5339653438087,19.6495190528383));
#76946=CARTESIAN_POINT('',(4.55736144060343,32.6604876193617,20.2466717586953));
#76947=CARTESIAN_POINT('Origin',(4.5,32.3339653438087,19.9959292143521));
#76948=CARTESIAN_POINT('',(4.49524972087093,32.0570688314042,20.4079280576996));
#76949=CARTESIAN_POINT('Origin',(4.5,32.0839653438087,20.4289419162443));
#76950=CARTESIAN_POINT('',(1.90350512467335,32.0308439720488,20.387438952028));
#76951=CARTESIAN_POINT('Origin',(1.9,32.0839653438087,20.4289419162443));
#76952=CARTESIAN_POINT('Ctrl Pts',(0.138207714141628,36.5204955072696,22.2446462638181));
#76953=CARTESIAN_POINT('Ctrl Pts',(0.370217470898585,36.2375102394015,22.2632399142706));
#76954=CARTESIAN_POINT('Ctrl Pts',(0.600000000000001,35.9562839053824,22.2808358845789));
#76955=CARTESIAN_POINT('Origin',(1.9,33.7339653438087,17.5710580837557));
#76956=CARTESIAN_POINT('',(5.09593997529677,37.7041716521717,19.1751255543105));
#76957=CARTESIAN_POINT('',(17.5,37.7041716521717,19.1751255543105));
#76958=CARTESIAN_POINT('',(4.47529854852883,33.5694020278343,17.5045701882916));
#76959=CARTESIAN_POINT('Origin',(4.5,33.7339653438087,17.5710580837557));
#76960=CARTESIAN_POINT('',(5.09944803334083,37.459394730737,19.6490138787379));
#76961=CARTESIAN_POINT('Origin',(-0.840551718690874,0.,0.));
#76962=CARTESIAN_POINT('',(4.50447263544529,33.5136270415661,18.0163441277467));
#76963=CARTESIAN_POINT('Origin',(4.5,33.4839653438087,18.0040707856479));
#76964=CARTESIAN_POINT('',(10.8302042597752,37.2924258787336,19.9640920674886));
#76965=CARTESIAN_POINT('Origin',(-62.7155570771054,0.,0.));
#76966=CARTESIAN_POINT('',(10.8987117910442,33.3579488669236,18.3802631128033));
#76967=CARTESIAN_POINT('Origin',(10.9,33.2839653438087,18.3504809471617));
#76968=CARTESIAN_POINT('',(11.6618634261911,37.4090062358548,19.7447778525305));
#76969=CARTESIAN_POINT('Origin',(26.9856656232739,0.,0.));
#76970=CARTESIAN_POINT('',(11.8995413080444,33.4416219555226,18.0938594155378));
#76971=CARTESIAN_POINT('Origin',(11.9,33.4339653438087,18.0906733260263));
#76972=CARTESIAN_POINT('',(12.3548486633046,37.5911252244478,19.3958063601357));
#76973=CARTESIAN_POINT('Origin',(20.8267261185512,0.,0.));
#76974=CARTESIAN_POINT('',(12.600317055424,33.6288475295615,17.742127215612));
#76975=CARTESIAN_POINT('Origin',(12.6,33.6339653438087,17.7442631645126));
#76976=CARTESIAN_POINT('',(13.103292255208,37.7041716521717,19.1751255543105));
#76977=CARTESIAN_POINT('Origin',(25.13830739299,0.,0.));
#76978=CARTESIAN_POINT('',(13.2001612154348,33.7273468611033,17.5683840431675));
#76979=CARTESIAN_POINT('Origin',(13.2,33.7339653438087,17.5710580837557));
#76980=CARTESIAN_POINT('',(21.896707744792,37.7041716521717,19.1751255543105));
#76981=CARTESIAN_POINT('',(17.5,37.7041716521717,19.1751255543105));
#76982=CARTESIAN_POINT('',(21.7978078257374,33.6439685797946,17.5346970308537));
#76983=CARTESIAN_POINT('Origin',(21.8,33.7339653438087,17.5710580837557));
#76984=CARTESIAN_POINT('',(22.6451513366954,37.5911252244478,19.3958063601357));
#76985=CARTESIAN_POINT('Origin',(9.86169260701005,0.,0.));
#76986=CARTESIAN_POINT('',(22.3997512812625,33.6299506000067,17.7425875883397));
#76987=CARTESIAN_POINT('Origin',(22.4,33.6339653438087,17.7442631645126));
#76988=CARTESIAN_POINT('',(23.3381365738089,37.4090062358548,19.7447778525305));
#76989=CARTESIAN_POINT('Origin',(14.1732738814488,0.,0.));
#76990=CARTESIAN_POINT('',(23.1003542130464,33.4398779649625,18.0931337015746));
#76991=CARTESIAN_POINT('Origin',(23.1,33.4339653438087,18.0906733260263));
#76992=CARTESIAN_POINT('',(24.1697957402248,37.2924258787336,19.9640920674886));
#76993=CARTESIAN_POINT('Origin',(8.01433437672608,0.,0.));
#76994=CARTESIAN_POINT('',(24.100209736014,33.2960107570711,18.3553298442931));
#76995=CARTESIAN_POINT('Origin',(24.1,33.2839653438087,18.3504809471617));
#76996=CARTESIAN_POINT('',(29.9005519666592,37.459394730737,19.6490138787379));
#76997=CARTESIAN_POINT('Origin',(97.7155570771054,0.,0.));
#76998=CARTESIAN_POINT('',(30.4426385593966,33.864375894796,18.1614760990067));
#76999=CARTESIAN_POINT('Origin',(30.5,33.4839653438087,18.0040707856479));
#77000=CARTESIAN_POINT('',(29.9040600247032,37.7041716521717,19.1751255543105));
#77001=CARTESIAN_POINT('Origin',(35.8405517186909,0.,0.));
#77002=CARTESIAN_POINT('',(30.5047502791291,33.7023185522751,17.5582719500126));
#77003=CARTESIAN_POINT('Origin',(30.5,33.7339653438087,17.5710580837557));
#77004=CARTESIAN_POINT('',(17.5,37.7041716521717,19.1751255543105));
#77005=CARTESIAN_POINT('Origin',(17.5,37.0225860117848,21.375));
#77006=CARTESIAN_POINT('Origin',(17.5,0.,0.));
#77007=CARTESIAN_POINT('',(0.600000000000001,39.2790537077817,15.6985967468815));
#77008=CARTESIAN_POINT('Origin',(0.600000000000001,0.,0.));
#77009=CARTESIAN_POINT('',(1.67735469196904,38.9247727484987,16.5575380560557));
#77010=CARTESIAN_POINT('Origin',(8.14497546096349,0.,0.));
#77011=CARTESIAN_POINT('',(5.09593997529677,38.9247727484987,16.5575380560557));
#77012=CARTESIAN_POINT('',(17.5,38.9247727484987,16.5575380560557));
#77013=CARTESIAN_POINT('',(5.09944803334083,39.1304526938498,16.0654185122698));
#77014=CARTESIAN_POINT('Origin',(-0.840551718690872,0.,0.));
#77015=CARTESIAN_POINT('',(10.8302042597752,39.2644910802189,15.7349845952072));
#77016=CARTESIAN_POINT('Origin',(-62.7155570771055,0.,0.));
#77017=CARTESIAN_POINT('',(11.6618634261911,39.1714230536436,15.9652627899599));
#77018=CARTESIAN_POINT('Origin',(26.9856656232739,0.,0.));
#77019=CARTESIAN_POINT('',(12.3548486633046,39.0211592104439,16.3290885806033));
#77020=CARTESIAN_POINT('Origin',(20.8267261185512,0.,0.));
#77021=CARTESIAN_POINT('',(13.103292255208,38.9247727484987,16.5575380560557));
#77022=CARTESIAN_POINT('Origin',(25.13830739299,0.,0.));
#77023=CARTESIAN_POINT('',(21.896707744792,38.9247727484987,16.5575380560557));
#77024=CARTESIAN_POINT('',(17.5,38.9247727484987,16.5575380560557));
#77025=CARTESIAN_POINT('',(22.6451513366954,39.0211592104439,16.3290885806033));
#77026=CARTESIAN_POINT('Origin',(9.86169260701006,0.,0.));
#77027=CARTESIAN_POINT('',(23.3381365738089,39.1714230536436,15.9652627899599));
#77028=CARTESIAN_POINT('Origin',(14.1732738814488,0.,0.));
#77029=CARTESIAN_POINT('',(24.1697957402248,39.2644910802189,15.7349845952072));
#77030=CARTESIAN_POINT('Origin',(8.01433437672609,0.,0.));
#77031=CARTESIAN_POINT('',(29.9005519666592,39.1304526938498,16.0654185122698));
#77032=CARTESIAN_POINT('Origin',(97.7155570771054,0.,0.));
#77033=CARTESIAN_POINT('',(29.9040600247032,38.9247727484987,16.5575380560557));
#77034=CARTESIAN_POINT('Origin',(35.8405517186909,0.,0.));
#77035=CARTESIAN_POINT('',(17.5,38.9247727484987,16.5575380560557));
#77036=CARTESIAN_POINT('Origin',(33.1,35.1439863533772,14.5472582706722));
#77037=CARTESIAN_POINT('',(30.5247014514712,34.987274410005,14.4639330523272));
#77038=CARTESIAN_POINT('Origin',(30.5,35.1439863533772,14.5472582706722));
#77039=CARTESIAN_POINT('',(30.4955273645547,35.343464522354,14.0922449867892));
#77040=CARTESIAN_POINT('Origin',(30.5,35.31499642504,14.0774119602792));
#77041=CARTESIAN_POINT('',(24.1012882089558,35.5221746368434,13.7390659716653));
#77042=CARTESIAN_POINT('Origin',(24.1,35.4518044823703,13.7015349119648));
#77043=CARTESIAN_POINT('',(23.1004586919557,35.35656070068,13.9872600241959));
#77044=CARTESIAN_POINT('Origin',(23.1,35.3491984393726,13.9834426982006));
#77045=CARTESIAN_POINT('',(22.399682944576,35.2074644826695,14.3567722348382));
#77046=CARTESIAN_POINT('Origin',(22.4,35.2123903820423,14.359319746515));
#77047=CARTESIAN_POINT('',(21.7998387845652,35.137683640766,14.5439070589317));
#77048=CARTESIAN_POINT('Origin',(21.8,35.1439863533772,14.5472582706722));
#77049=CARTESIAN_POINT('',(13.2021921742626,35.0582833660355,14.501689183981));
#77050=CARTESIAN_POINT('Origin',(13.2,35.1439863533772,14.5472582706722));
#77051=CARTESIAN_POINT('',(12.6002487187375,35.208526188654,14.3573213139379));
#77052=CARTESIAN_POINT('Origin',(12.6,35.2123903820423,14.359319746515));
#77053=CARTESIAN_POINT('',(11.8996457869536,35.3548837560077,13.9863905298622));
#77054=CARTESIAN_POINT('Origin',(11.9,35.3491984393726,13.9834426982006));
#77055=CARTESIAN_POINT('',(10.899790263986,35.4632615954717,13.7076454228629));
#77056=CARTESIAN_POINT('Origin',(10.9,35.4518044823703,13.7015349119648));
#77057=CARTESIAN_POINT('',(4.55736144060343,35.6800990794245,14.267645163841));
#77058=CARTESIAN_POINT('Origin',(4.5,35.31499642504,14.0774119602792));
#77059=CARTESIAN_POINT('',(4.49524972087093,35.1138494411902,14.5312341902212));
#77060=CARTESIAN_POINT('Origin',(4.5,35.1439863533772,14.5472582706722));
#77061=CARTESIAN_POINT('',(1.90350512467335,35.0844651005135,14.5156102591402));
#77062=CARTESIAN_POINT('Origin',(1.9,35.1439863533772,14.5472582706722));
#77063=CARTESIAN_POINT('Ctrl Pts',(0.138207714141622,39.8284094059642,15.5649826112914));
#77064=CARTESIAN_POINT('Ctrl Pts',(0.37021747089279,39.5529520737035,15.6324336584841));
#77065=CARTESIAN_POINT('Ctrl Pts',(0.600000000000001,39.2790537077817,15.6985967468815));
#77066=CARTESIAN_POINT('Origin',(1.9,36.2726528263519,11.4462726220787));
#77067=CARTESIAN_POINT('',(5.09593997529677,40.4610861730024,12.3365516130268));
#77068=CARTESIAN_POINT('',(17.5,40.4610861730024,12.3365516130268));
#77069=CARTESIAN_POINT('',(4.47529854852883,36.0990440950346,11.409370947074));
#77070=CARTESIAN_POINT('Origin',(4.5,36.2726528263519,11.4462726220787));
#77071=CARTESIAN_POINT('',(5.09944803334083,40.3023178069695,12.8457455753269));
#77072=CARTESIAN_POINT('Origin',(-0.840551718690874,0.,0.));
#77073=CARTESIAN_POINT('',(4.50447263544529,36.1329850680974,11.9230551151638));
#77074=CARTESIAN_POINT('Origin',(4.5,36.101642754689,11.9161189324716));
#77075=CARTESIAN_POINT('',(10.8302042597752,40.1925983403042,13.1850308552911));
#77076=CARTESIAN_POINT('Origin',(-62.7155570771055,0.,0.));
#77077=CARTESIAN_POINT('',(10.8987117910442,36.0428658633082,12.3084785844451));
#77078=CARTESIAN_POINT('Origin',(10.9,35.9648346973588,12.291995980786));
#77079=CARTESIAN_POINT('',(11.6618634261911,40.2693240660821,12.9488045494888));
#77080=CARTESIAN_POINT('Origin',(26.9856656232739,0.,0.));
#77081=CARTESIAN_POINT('',(11.8995413080444,36.0755342895717,12.0118963235316));
#77082=CARTESIAN_POINT('Origin',(11.9,36.0674407403565,12.0100881945502));
#77083=CARTESIAN_POINT('',(12.3548486633046,40.3880779943072,12.5735100877104));
#77084=CARTESIAN_POINT('Origin',(20.8267261185512,0.,0.));
#77085=CARTESIAN_POINT('',(12.600317055424,36.1988378309035,11.6329963463162));
#77086=CARTESIAN_POINT('Origin',(12.6,36.2042487976867,11.6342111462358));
#77087=CARTESIAN_POINT('',(13.103292255208,40.4610861730024,12.3365516130268));
#77088=CARTESIAN_POINT('Origin',(25.13830739299,0.,0.));
#77089=CARTESIAN_POINT('',(13.2001612154348,36.2656705509953,11.4447884936362));
#77090=CARTESIAN_POINT('Origin',(13.2,36.2726528263519,11.4462726220787));
#77091=CARTESIAN_POINT('',(21.896707744792,40.4610861730024,12.3365516130268));
#77092=CARTESIAN_POINT('',(17.5,40.4610861730024,12.3365516130268));
#77093=CARTESIAN_POINT('',(21.7978078257374,36.1777092848303,11.4260917493401));
#77094=CARTESIAN_POINT('Origin',(21.8,36.2726528263519,11.4462726220787));
#77095=CARTESIAN_POINT('',(22.6451513366954,40.3880779943072,12.5735100877104));
#77096=CARTESIAN_POINT('Origin',(9.86169260701004,0.,0.));
#77097=CARTESIAN_POINT('',(22.3997512812625,36.2000040861152,11.633258178775));
#77098=CARTESIAN_POINT('Origin',(22.4,36.2042487976867,11.6342111462358));
#77099=CARTESIAN_POINT('',(23.3381365738089,40.2693240660821,12.9488045494888));
#77100=CARTESIAN_POINT('Origin',(14.1732738814488,0.,0.));
#77101=CARTESIAN_POINT('',(23.1003542130464,36.0736907752397,12.0114844755768));
#77102=CARTESIAN_POINT('Origin',(23.1,36.0674407403565,12.0100881945502));
#77103=CARTESIAN_POINT('',(24.1697957402248,40.1925983403042,13.1850308552911));
#77104=CARTESIAN_POINT('Origin',(8.01433437672608,0.,0.));
#77105=CARTESIAN_POINT('',(24.100209736014,35.9775391158784,12.2946795482123));
#77106=CARTESIAN_POINT('Origin',(24.1,35.9648346973588,12.291995980786));
#77107=CARTESIAN_POINT('',(29.9005519666592,40.3023178069695,12.8457455753269));
#77108=CARTESIAN_POINT('Origin',(97.7155570771054,0.,0.));
#77109=CARTESIAN_POINT('',(30.4426385593966,36.5036071604488,12.0050753064884));
#77110=CARTESIAN_POINT('Origin',(30.5,36.101642754689,11.9161189324716));
#77111=CARTESIAN_POINT('',(29.9040600247032,40.4610861730024,12.3365516130268));
#77112=CARTESIAN_POINT('Origin',(35.8405517186909,0.,0.));
#77113=CARTESIAN_POINT('',(30.5047502791291,36.2392665318678,11.4391761461162));
#77114=CARTESIAN_POINT('Origin',(30.5,36.2726528263519,11.4462726220787));
#77115=CARTESIAN_POINT('',(17.5,40.4610861730024,12.3365516130268));
#77116=CARTESIAN_POINT('Origin',(17.5,40.1718595385976,14.6213611271723));
#77117=CARTESIAN_POINT('Origin',(17.5,0.,0.));
#77118=CARTESIAN_POINT('',(0.600000000000001,41.4083493394303,8.63936369090332));
#77119=CARTESIAN_POINT('Origin',(0.600000000000001,0.,0.));
#77120=CARTESIAN_POINT('',(1.67735469196904,41.2086042970448,9.54677599452213));
#77121=CARTESIAN_POINT('Origin',(8.14497546096349,0.,0.));
#77122=CARTESIAN_POINT('',(5.09593997529677,41.2086042970448,9.54677599452213));
#77123=CARTESIAN_POINT('',(17.5,41.2086042970448,9.54677599452213));
#77124=CARTESIAN_POINT('',(5.09944803334083,41.325703839893,9.02641690470011));
#77125=CARTESIAN_POINT('Origin',(-0.840551718690872,0.,0.));
#77126=CARTESIAN_POINT('',(10.8302042597752,41.4003266344532,8.6777274997883));
#77127=CARTESIAN_POINT('Origin',(-62.7155570771055,0.,0.));
#77128=CARTESIAN_POINT('',(11.6618634261911,41.3486599091995,8.92066834454426));
#77129=CARTESIAN_POINT('Origin',(26.9856656232739,0.,0.));
#77130=CARTESIAN_POINT('',(12.3548486633046,41.2638565969525,9.30505984645652));
#77131=CARTESIAN_POINT('Origin',(20.8267261185512,0.,0.));
#77132=CARTESIAN_POINT('',(13.103292255208,41.2086042970448,9.54677599452213));
#77133=CARTESIAN_POINT('Origin',(25.13830739299,0.,0.));
#77134=CARTESIAN_POINT('',(21.896707744792,41.2086042970448,9.54677599452213));
#77135=CARTESIAN_POINT('',(17.5,41.2086042970448,9.54677599452213));
#77136=CARTESIAN_POINT('',(22.6451513366954,41.2638565969525,9.30505984645652));
#77137=CARTESIAN_POINT('Origin',(9.86169260701005,0.,0.));
#77138=CARTESIAN_POINT('',(23.3381365738089,41.3486599091995,8.92066834454427));
#77139=CARTESIAN_POINT('Origin',(14.1732738814488,0.,0.));
#77140=CARTESIAN_POINT('',(24.1697957402248,41.4003266344532,8.6777274997883));
#77141=CARTESIAN_POINT('Origin',(8.01433437672608,0.,0.));
#77142=CARTESIAN_POINT('',(29.9005519666592,41.325703839893,9.02641690470011));
#77143=CARTESIAN_POINT('Origin',(97.7155570771054,0.,0.));
#77144=CARTESIAN_POINT('',(29.9040600247032,41.2086042970448,9.54677599452213));
#77145=CARTESIAN_POINT('Origin',(35.8405517186909,0.,0.));
#77146=CARTESIAN_POINT('',(17.5,41.2086042970448,9.54677599452213));
#77147=CARTESIAN_POINT('Origin',(33.1,37.1361751213135,8.2235635438135));
#77148=CARTESIAN_POINT('',(30.5247014514712,36.9673747121716,8.16871696615113));
#77149=CARTESIAN_POINT('Origin',(30.5,37.1361751213135,8.2235635438135));
#77150=CARTESIAN_POINT('',(30.4955273645547,37.253610541118,7.74082391359484));
#77151=CARTESIAN_POINT('Origin',(30.5,37.2229992101469,7.73115966730739));
#77152=CARTESIAN_POINT('',(24.1012882089558,37.3682767550424,7.36197779558791));
#77153=CARTESIAN_POINT('Origin',(24.1,37.2924584812137,7.33723656610251));
#77154=CARTESIAN_POINT('',(23.1004586919557,37.2482773116316,7.63515978098256));
#77155=CARTESIAN_POINT('Origin',(23.1,37.2403640279136,7.63267889200617));
#77156=CARTESIAN_POINT('',(22.399682944576,37.1656113221937,8.02494855741037));
#77157=CARTESIAN_POINT('Origin',(22.4,37.1709047568469,8.02660199321105));
#77158=CARTESIAN_POINT('',(21.7998387845652,37.1293862292573,8.22135769906884));
#77159=CARTESIAN_POINT('Origin',(21.8,37.1361751213135,8.2235635438135));
#77160=CARTESIAN_POINT('',(13.2021921742626,37.0438611660612,8.19356892151487));
#77161=CARTESIAN_POINT('Origin',(13.2,37.1361751213135,8.2235635438135));
#77162=CARTESIAN_POINT('',(12.6002487187375,37.1667522450638,8.02530493145534));
#77163=CARTESIAN_POINT('Origin',(12.6,37.1709047568469,8.02660199321105));
#77164=CARTESIAN_POINT('',(11.8996457869536,37.2464748574103,7.6345946946079));
#77165=CARTESIAN_POINT('Origin',(11.9,37.2403640279136,7.63267889200617));
#77166=CARTESIAN_POINT('',(10.899790263986,37.3048026141052,7.34126473779837));
#77167=CARTESIAN_POINT('Origin',(10.9,37.2924584812137,7.33723656610251));
#77168=CARTESIAN_POINT('',(4.55736144060343,37.6155887839604,7.85510339046017));
#77169=CARTESIAN_POINT('Origin',(4.5,37.2229992101469,7.73115966730739));
#77170=CARTESIAN_POINT('',(4.49524972087093,37.1037135041708,8.21301612503227));
#77171=CARTESIAN_POINT('Origin',(4.5,37.1361751213135,8.2235635438135));
#77172=CARTESIAN_POINT('',(1.90350512467335,37.0720625104951,8.20273209378168));
#77173=CARTESIAN_POINT('Origin',(1.9,37.1361751213135,8.2235635438135));
#77174=CARTESIAN_POINT('Ctrl Pts',(0.138207714141622,41.9261572390061,8.41238483838184));
#77175=CARTESIAN_POINT('Ctrl Pts',(0.37021747089976,41.6665974739906,8.52664381638148));
#77176=CARTESIAN_POINT('Ctrl Pts',(0.600000000000001,41.4083493394303,8.63936369090332));
#77177=CARTESIAN_POINT('Origin',(1.9,37.7092141076143,4.97369795887321));
#77178=CARTESIAN_POINT('',(5.09593997529677,41.9886110647639,5.12313779357752));
#77179=CARTESIAN_POINT('',(17.5,41.9886110647639,5.12313779357752));
#77180=CARTESIAN_POINT('',(4.47529854852883,37.5318349744051,4.96750374304976));
#77181=CARTESIAN_POINT('Origin',(4.5,37.7092141076143,4.97369795887321));
#77182=CARTESIAN_POINT('',(5.09944803334083,41.9206753505941,5.65216579287046));
#77183=CARTESIAN_POINT('Origin',(-0.840551718690874,0.,0.));
#77184=CARTESIAN_POINT('',(4.50447263544529,37.6544606275072,5.46749010626366));
#77185=CARTESIAN_POINT('Origin',(4.5,37.6223900187809,5.46610183537931));
#77186=CARTESIAN_POINT('',(10.8302042597752,41.8715390397407,6.00534915250318));
#77187=CARTESIAN_POINT('Origin',(-62.7155570771055,0.,0.));
#77188=CARTESIAN_POINT('',(10.8987117910442,37.6326386190063,5.86270716268919));
#77189=CARTESIAN_POINT('Origin',(10.9,37.5529307477141,5.8600249365842));
#77190=CARTESIAN_POINT('',(11.6618634261911,41.9060788618227,5.75938837262207));
#77191=CARTESIAN_POINT('Origin',(26.9856656232739,0.,0.));
#77192=CARTESIAN_POINT('',(11.8995413080444,37.6133097693334,5.56495784004781));
#77193=CARTESIAN_POINT('Origin',(11.9,37.6050252010142,5.56458261068053));
#77194=CARTESIAN_POINT('',(12.3548486633046,41.9578594516632,5.3691740737731));
#77195=CARTESIAN_POINT('Origin',(20.8267261185512,0.,0.));
#77196=CARTESIAN_POINT('',(12.600317055424,37.6689447622493,5.17040276961776));
#77197=CARTESIAN_POINT('Origin',(12.6,37.674484472081,5.17065950947565));
#77198=CARTESIAN_POINT('',(13.103292255208,41.9886110647639,5.12313779357752));
#77199=CARTESIAN_POINT('Origin',(25.13830739299,0.,0.));
#77200=CARTESIAN_POINT('',(13.2001612154348,37.7020801925101,4.97344883706828));
#77201=CARTESIAN_POINT('Origin',(13.2,37.7092141076143,4.97369795887321));
#77202=CARTESIAN_POINT('',(21.896707744792,41.9886110647639,5.12313779357752));
#77203=CARTESIAN_POINT('',(17.5,41.9886110647639,5.12313779357752));
#77204=CARTESIAN_POINT('',(21.7978078257374,37.6122086000506,4.97031045190415));
#77205=CARTESIAN_POINT('Origin',(21.8,37.7092141076143,4.97369795887321));
#77206=CARTESIAN_POINT('',(22.6451513366954,41.9578594516632,5.3691740737731));
#77207=CARTESIAN_POINT('Origin',(9.86169260701005,0.,0.));
#77208=CARTESIAN_POINT('',(22.3997512812625,37.6701387661531,5.17045810616099));
#77209=CARTESIAN_POINT('Origin',(22.4,37.674484472081,5.17065950947565));
#77210=CARTESIAN_POINT('',(23.3381365738089,41.9060788618227,5.75938837262207));
#77211=CARTESIAN_POINT('Origin',(14.1732738814488,0.,0.));
#77212=CARTESIAN_POINT('',(23.1003542130464,37.6114227454796,5.56487237189312));
#77213=CARTESIAN_POINT('Origin',(23.1,37.6050252010142,5.56458261068053));
#77214=CARTESIAN_POINT('',(24.1697957402248,41.8715390397407,6.00534915250318));
#77215=CARTESIAN_POINT('Origin',(8.01433437672607,0.,0.));
#77216=CARTESIAN_POINT('',(24.100209736014,37.565908154163,5.8604616354671));
#77217=CARTESIAN_POINT('Origin',(24.1,37.5529307477141,5.8600249365842));
#77218=CARTESIAN_POINT('',(29.9005519666592,41.9206753505941,5.65216579287046));
#77219=CARTESIAN_POINT('Origin',(97.7155570771054,0.,0.));
#77220=CARTESIAN_POINT('',(30.4426385593966,38.0336947942479,5.48390637564377));
#77221=CARTESIAN_POINT('Origin',(30.5,37.6223900187809,5.46610183537931));
#77222=CARTESIAN_POINT('',(29.9040600247032,41.9886110647639,5.12313779357752));
#77223=CARTESIAN_POINT('Origin',(35.8405517186909,0.,0.));
#77224=CARTESIAN_POINT('',(30.5047502791291,37.6751027358433,4.97250676352255));
#77225=CARTESIAN_POINT('Origin',(30.5,37.7092141076143,4.97369795887321));
#77226=CARTESIAN_POINT('',(17.5,41.9886110647639,5.12313779357752));
#77227=CARTESIAN_POINT('Origin',(17.5,42.1005314412719,7.42345959526127));
#77228=CARTESIAN_POINT('Origin',(17.5,0.,0.));
#77229=CARTESIAN_POINT('',(0.600000000000001,42.2794732300362,1.31762794090604));
#77230=CARTESIAN_POINT('Origin',(0.600000000000001,0.,0.));
#77231=CARTESIAN_POINT('',(1.67735469196904,42.240333256585,2.24593997529677));
#77232=CARTESIAN_POINT('Origin',(8.14497546096349,0.,0.));
#77233=CARTESIAN_POINT('',(5.09593997529677,42.240333256585,2.24593997529677));
#77234=CARTESIAN_POINT('',(17.5,42.240333256585,2.24593997529677));
#77235=CARTESIAN_POINT('',(5.09944803334083,42.2652943865761,1.71315218706844));
#77236=CARTESIAN_POINT('Origin',(-0.840551718690872,0.,0.));
#77237=CARTESIAN_POINT('',(10.8302042597752,42.2782342134758,1.35680204543027));
#77238=CARTESIAN_POINT('Origin',(-62.7155570771055,0.,0.));
#77239=CARTESIAN_POINT('',(11.6618634261911,42.269538656846,1.60502390555561));
#77240=CARTESIAN_POINT('Origin',(26.9856656232739,0.,0.));
#77241=CARTESIAN_POINT('',(12.3548486633046,42.2527725812817,1.99830157746262));
#77242=CARTESIAN_POINT('Origin',(20.8267261185512,0.,0.));
#77243=CARTESIAN_POINT('',(13.103292255208,42.240333256585,2.24593997529677));
#77244=CARTESIAN_POINT('Origin',(25.13830739299,0.,0.));
#77245=CARTESIAN_POINT('',(21.896707744792,42.240333256585,2.24593997529677));
#77246=CARTESIAN_POINT('',(17.5,42.240333256585,2.24593997529677));
#77247=CARTESIAN_POINT('',(22.6451513366954,42.2527725812817,1.99830157746261));
#77248=CARTESIAN_POINT('Origin',(9.86169260701005,0.,0.));
#77249=CARTESIAN_POINT('',(23.3381365738089,42.269538656846,1.60502390555561));
#77250=CARTESIAN_POINT('Origin',(14.1732738814488,0.,0.));
#77251=CARTESIAN_POINT('',(24.1697957402248,42.2782342134758,1.35680204543027));
#77252=CARTESIAN_POINT('Origin',(8.01433437672608,0.,0.));
#77253=CARTESIAN_POINT('',(29.9005519666592,42.2652943865761,1.71315218706844));
#77254=CARTESIAN_POINT('Origin',(97.7155570771054,0.,0.));
#77255=CARTESIAN_POINT('',(29.9040600247032,42.240333256585,2.24593997529677));
#77256=CARTESIAN_POINT('Origin',(35.8405517186909,0.,0.));
#77257=CARTESIAN_POINT('',(17.5,42.240333256585,2.24593997529677));
#77258=CARTESIAN_POINT('Origin',(1.9,38.,-1.65));
#77259=CARTESIAN_POINT('',(5.09593997529677,42.240333256585,-2.24593997529677));
#77260=CARTESIAN_POINT('',(17.5,42.240333256585,-2.24593997529677));
#77261=CARTESIAN_POINT('',(4.47529854852883,37.8242400401031,-1.62529854852883));
#77262=CARTESIAN_POINT('Origin',(4.5,38.,-1.65));
#77263=CARTESIAN_POINT('',(5.09944803334083,42.2652943865761,-1.71315218706844));
#77264=CARTESIAN_POINT('Origin',(-0.840551718690874,0.,0.));
#77265=CARTESIAN_POINT('',(4.50447263544529,38.0318244548267,-1.15420182283181));
#77266=CARTESIAN_POINT('Origin',(4.5,38.,-1.15));
#77267=CARTESIAN_POINT('',(10.8302042597752,42.2782342134758,-1.35680204543028));
#77268=CARTESIAN_POINT('Origin',(-62.7155570771055,0.,0.));
#77269=CARTESIAN_POINT('',(10.8987117910442,38.0789626932999,-0.761199649532072));
#77270=CARTESIAN_POINT('Origin',(10.9,38.,-0.75));
#77271=CARTESIAN_POINT('',(11.6618634261911,42.269538656846,-1.60502390555561));
#77272=CARTESIAN_POINT('Origin',(26.9856656232739,0.,0.));
#77273=CARTESIAN_POINT('',(11.8995413080444,38.0082238650069,-1.05106907140133));
#77274=CARTESIAN_POINT('Origin',(11.9,38.,-1.05));
#77275=CARTESIAN_POINT('',(12.3548486633046,42.2527725812817,-1.99830157746261));
#77276=CARTESIAN_POINT('Origin',(20.8267261185512,0.,0.));
#77277=CARTESIAN_POINT('',(12.600317055424,37.9944998683999,-1.44929087888549));
#77278=CARTESIAN_POINT('Origin',(12.6,38.,-1.45));
#77279=CARTESIAN_POINT('',(13.103292255208,42.240333256585,-2.24593997529677));
#77280=CARTESIAN_POINT('Origin',(25.13830739299,0.,0.));
#77281=CARTESIAN_POINT('',(13.2001612154348,37.9929312055486,-1.64900654572746));
#77282=CARTESIAN_POINT('Origin',(13.2,38.,-1.65));
#77283=CARTESIAN_POINT('',(21.896707744792,42.240333256585,-2.24593997529677));
#77284=CARTESIAN_POINT('',(17.5,42.240333256585,-2.24593997529677));
#77285=CARTESIAN_POINT('',(21.7978078257374,37.9038799896544,-1.63649121351442));
#77286=CARTESIAN_POINT('Origin',(21.8,38.,-1.65));
#77287=CARTESIAN_POINT('',(22.6451513366954,42.2527725812817,-1.99830157746261));
#77288=CARTESIAN_POINT('Origin',(9.86169260701005,0.,0.));
#77289=CARTESIAN_POINT('',(22.3997512812625,37.9956853417913,-1.44944371963071));
#77290=CARTESIAN_POINT('Origin',(22.4,38.,-1.45));
#77291=CARTESIAN_POINT('',(23.3381365738089,42.269538656846,-1.60502390555561));
#77292=CARTESIAN_POINT('Origin',(14.1732738814488,0.,0.));
#77293=CARTESIAN_POINT('',(23.1003542130464,38.0063506678963,-1.05082556284928));
#77294=CARTESIAN_POINT('Origin',(23.1,38.,-1.05));
#77295=CARTESIAN_POINT('',(24.1697957402248,42.2782342134758,-1.35680204543027));
#77296=CARTESIAN_POINT('Origin',(8.01433437672608,0.,0.));
#77297=CARTESIAN_POINT('',(24.100209736014,38.01285608245,-0.751823438535068));
#77298=CARTESIAN_POINT('Origin',(24.1,38.,-0.75));
#77299=CARTESIAN_POINT('',(29.9005519666592,42.2652943865761,-1.71315218706844));
#77300=CARTESIAN_POINT('Origin',(97.7155570771054,0.,0.));
#77301=CARTESIAN_POINT('',(30.4426385593966,38.408147857702,-1.2038882754343));
#77302=CARTESIAN_POINT('Origin',(30.5,38.,-1.15));
#77303=CARTESIAN_POINT('',(29.9040600247032,42.240333256585,-2.24593997529677));
#77304=CARTESIAN_POINT('Origin',(35.8405517186909,0.,0.));
#77305=CARTESIAN_POINT('',(30.5047502791291,37.9662000077121,-1.64524972087093));
#77306=CARTESIAN_POINT('Origin',(30.5,38.,-1.65));
#77307=CARTESIAN_POINT('',(33.3226453080309,42.240333256585,-2.24593997529677));
#77308=CARTESIAN_POINT('',(17.5,42.240333256585,-2.24593997529677));
#77309=CARTESIAN_POINT('',(33.0964948753266,37.933244060464,-1.64061806453627));
#77310=CARTESIAN_POINT('Origin',(33.1,38.,-1.65));
#77311=CARTESIAN_POINT('Origin',(26.8550245390365,0.,0.));
#77312=CARTESIAN_POINT('Origin',(33.1,38.,1.65));
#77313=CARTESIAN_POINT('',(30.5247014514712,37.8242400401031,1.62529854852883));
#77314=CARTESIAN_POINT('Origin',(30.5,38.,1.65));
#77315=CARTESIAN_POINT('',(30.4955273645547,38.0318244548267,1.15420182283181));
#77316=CARTESIAN_POINT('Origin',(30.5,38.,1.15));
#77317=CARTESIAN_POINT('',(24.1012882089558,38.0789626932999,0.761199649532072));
#77318=CARTESIAN_POINT('Origin',(24.1,38.,0.75));
#77319=CARTESIAN_POINT('',(23.1004586919557,38.0082238650069,1.05106907140133));
#77320=CARTESIAN_POINT('Origin',(23.1,38.,1.05));
#77321=CARTESIAN_POINT('',(22.399682944576,37.9944998683999,1.44929087888549));
#77322=CARTESIAN_POINT('Origin',(22.4,38.,1.45));
#77323=CARTESIAN_POINT('',(21.7998387845652,37.9929312055486,1.64900654572746));
#77324=CARTESIAN_POINT('Origin',(21.8,38.,1.65));
#77325=CARTESIAN_POINT('',(13.2021921742626,37.9038799896544,1.63649121351442));
#77326=CARTESIAN_POINT('Origin',(13.2,38.,1.65));
#77327=CARTESIAN_POINT('',(12.6002487187375,37.9956853417913,1.44944371963071));
#77328=CARTESIAN_POINT('Origin',(12.6,38.,1.45));
#77329=CARTESIAN_POINT('',(11.8996457869536,38.0063506678963,1.05082556284928));
#77330=CARTESIAN_POINT('Origin',(11.9,38.,1.05));
#77331=CARTESIAN_POINT('',(10.899790263986,38.01285608245,0.751823438535068));
#77332=CARTESIAN_POINT('Origin',(10.9,38.,0.75));
#77333=CARTESIAN_POINT('',(4.55736144060343,38.408147857702,1.2038882754343));
#77334=CARTESIAN_POINT('Origin',(4.5,38.,1.15));
#77335=CARTESIAN_POINT('',(4.49524972087093,37.9662000077121,1.64524972087093));
#77336=CARTESIAN_POINT('Origin',(4.5,38.,1.65));
#77337=CARTESIAN_POINT('',(1.90350512467335,37.933244060464,1.64061806453627));
#77338=CARTESIAN_POINT('Origin',(1.9,38.,1.65));
#77339=CARTESIAN_POINT('Ctrl Pts',(0.138207714141622,42.75,1.00418100903021));
#77340=CARTESIAN_POINT('Ctrl Pts',(0.37021747090124,42.514224394353,1.1617762166071));
#77341=CARTESIAN_POINT('Ctrl Pts',(0.6,42.2794732300361,1.31762794090604));
#77342=CARTESIAN_POINT('Origin',(0.299999999999998,0.,0.));
#77343=CARTESIAN_POINT('Origin',(0.600000000000001,0.,0.));
#77344=CARTESIAN_POINT('',(-2.8796409701215E-15,-42.9,-5.25373476834215E-15));
#77345=CARTESIAN_POINT('',(0.299999999999998,-42.6,-5.21699536436772E-15));
#77346=CARTESIAN_POINT('Origin',(0.,0.,0.));
#77347=CARTESIAN_POINT('Origin',(34.8112283287268,0.,-1.45831369988988E-15));
#77348=CARTESIAN_POINT('',(35.,47.1,-5.76808642398403E-15));
#77349=CARTESIAN_POINT('Origin',(35.,0.,0.));
#77350=CARTESIAN_POINT('',(34.6224566574536,47.6321401698912,5.83325479955954E-15));
#77351=CARTESIAN_POINT('',(34.8112283287268,47.3660700849456,5.80067061177179E-15));
#77352=CARTESIAN_POINT('',(34.6224566574536,-47.6321401698912,-5.83325479955954E-15));
#77353=CARTESIAN_POINT('Origin',(34.6224566574536,0.,-2.91662739977977E-15));
#77354=CARTESIAN_POINT('Origin',(34.6224566574536,0.,-2.91662739977977E-15));
#77355=CARTESIAN_POINT('Origin',(30.,0.,0.));
#77356=CARTESIAN_POINT('',(25.9624281765825,-50.6631501381961,-6.20444646514636E-15));
#77357=CARTESIAN_POINT('',(30.,-49.25,-6.03138548580071E-15));
#77358=CARTESIAN_POINT('',(25.9624281765825,-6.20444646514636E-15,50.6631501381961));
#77359=CARTESIAN_POINT('Origin',(25.9624281765825,0.,-7.75555808143296E-15));
#77360=CARTESIAN_POINT('Origin',(25.9624281765825,0.,-7.75555808143296E-15));
#77361=CARTESIAN_POINT('Origin',(35.,42.9,0.));
#77362=CARTESIAN_POINT('Origin',(23.9803256282139,0.,0.));
#77363=CARTESIAN_POINT('',(23.9803256282139,-6.2456986756515E-15,51.));
#77364=CARTESIAN_POINT('Origin',(23.9803256282139,-5.51091059616309E-15,
45.));
#77365=CARTESIAN_POINT('',(23.9803256282139,-51.,-6.2456986756515E-15));
#77366=CARTESIAN_POINT('Origin',(23.9803256282139,0.,0.));
#77367=CARTESIAN_POINT('Origin',(23.9803256282139,0.,0.));
#77368=CARTESIAN_POINT('Origin',(19.9,0.,0.));
#77369=CARTESIAN_POINT('',(14.8,-51.,-6.2456986756515E-15));
#77370=CARTESIAN_POINT('',(19.9,-51.,-6.2456986756515E-15));
#77371=CARTESIAN_POINT('Origin',(14.8,0.,0.));
#77372=CARTESIAN_POINT('Origin',(12.6,0.,0.));
#77373=CARTESIAN_POINT('',(12.6,-46.5,-5.69460761603519E-15));
#77374=CARTESIAN_POINT('',(12.6,-5.69460761603519E-15,46.5));
#77375=CARTESIAN_POINT('Origin',(12.6,0.,0.));
#77376=CARTESIAN_POINT('',(13.,-5.74359348800109E-15,46.9));
#77377=CARTESIAN_POINT('Origin',(12.6,-5.74359348800109E-15,46.9));
#77378=CARTESIAN_POINT('Origin',(13.,0.,0.));
#77379=CARTESIAN_POINT('Origin',(12.6,0.,0.));
#77380=CARTESIAN_POINT('Origin',(9.25,0.,0.));
#77381=CARTESIAN_POINT('',(5.9,-46.5,-5.69460761603519E-15));
#77382=CARTESIAN_POINT('',(9.25,-46.5,-5.69460761603519E-15));
#77383=CARTESIAN_POINT('',(5.9,-5.69460761603519E-15,46.5));
#77384=CARTESIAN_POINT('Origin',(5.9,0.,0.));
#77385=CARTESIAN_POINT('Origin',(5.9,0.,0.));
#77386=CARTESIAN_POINT('Origin',(13.,50.4,0.));
#77387=CARTESIAN_POINT('',(13.,-50.4,-6.17221986770266E-15));
#77388=CARTESIAN_POINT('Origin',(13.,0.,0.));
#77389=CARTESIAN_POINT('Origin',(5.9,0.,0.));
#77390=CARTESIAN_POINT('',(5.5,-5.74359348800109E-15,46.9));
#77391=CARTESIAN_POINT('Origin',(5.5,0.,0.));
#77392=CARTESIAN_POINT('Origin',(5.9,-5.74359348800109E-15,46.9));
#77393=CARTESIAN_POINT('Origin',(5.5,46.5,0.));
#77394=CARTESIAN_POINT('',(5.5,-50.,-6.12323399573677E-15));
#77395=CARTESIAN_POINT('Origin',(5.5,0.,0.));
#77396=CARTESIAN_POINT('Origin',(17.5,0.,0.));
#77397=CARTESIAN_POINT('Origin',(0.,49.7,0.));
#77398=CARTESIAN_POINT('',(1.31838984174237E-15,-49.7,-6.08649459176235E-15));
#77399=CARTESIAN_POINT('Origin',(0.,0.,0.));
#77400=CARTESIAN_POINT('Origin',(0.4,0.,0.));
#77401=CARTESIAN_POINT('',(0.800000000000004,-50.5,-6.18446633569413E-15));
#77402=CARTESIAN_POINT('Origin',(0.800000000000001,0.,0.));
#77403=CARTESIAN_POINT('',(0.4,-50.1,-6.13548046372824E-15));
#77404=CARTESIAN_POINT('Origin',(2.9,0.,0.));
#77405=CARTESIAN_POINT('',(5.,-50.5,-6.18446633569413E-15));
#77406=CARTESIAN_POINT('Origin',(5.,0.,0.));
#77407=CARTESIAN_POINT('',(2.9,-50.5,-6.18446633569413E-15));
#77408=CARTESIAN_POINT('Origin',(5.25,0.,0.));
#77409=CARTESIAN_POINT('',(5.25,-50.25,-6.15385016571545E-15));
#77410=CARTESIAN_POINT('Origin',(13.75,0.,0.));
#77411=CARTESIAN_POINT('',(14.5,-50.4,-6.17221986770266E-15));
#77412=CARTESIAN_POINT('Origin',(14.5,0.,0.));
#77413=CARTESIAN_POINT('',(13.75,-50.4,-6.17221986770266E-15));
#77414=CARTESIAN_POINT('Origin',(14.65,0.,0.));
#77415=CARTESIAN_POINT('',(14.65,-50.7,-6.20895927167708E-15));
#94271=UNCERTAINTY_MEASURE_WITH_UNIT(LENGTH_MEASURE(0.01),#94302,
'DISTANCE_ACCURACY_VALUE',
'Maximum model space distance between geometric entities at asserted c
onnectivities');
#94285=UNCERTAINTY_MEASURE_WITH_UNIT(LENGTH_MEASURE(0.01),#94302,
'DISTANCE_ACCURACY_VALUE',
'Maximum model space distance between geometric entities at asserted c
onnectivities');
#94287=(
GEOMETRIC_REPRESENTATION_CONTEXT(3)
GLOBAL_UNCERTAINTY_ASSIGNED_CONTEXT((#94271))
GLOBAL_UNIT_ASSIGNED_CONTEXT((#94302,#94304,#94305))
REPRESENTATION_CONTEXT('','3D')
);
#94301=(
GEOMETRIC_REPRESENTATION_CONTEXT(3)
GLOBAL_UNCERTAINTY_ASSIGNED_CONTEXT((#94285))
GLOBAL_UNIT_ASSIGNED_CONTEXT((#94302,#94304,#94305))
REPRESENTATION_CONTEXT('','3D')
);
#94302=(
LENGTH_UNIT()
NAMED_UNIT(*)
SI_UNIT(.MILLI.,.METRE.)
);
#94304=(
NAMED_UNIT(*)
PLANE_ANGLE_UNIT()
SI_UNIT($,.RADIAN.)
);
#94305=(
NAMED_UNIT(*)
SI_UNIT($,.STERADIAN.)
SOLID_ANGLE_UNIT()
);
#94307=SHAPE_DEFINITION_REPRESENTATION(#94322,#94371);
#94322=PRODUCT_DEFINITION_SHAPE('',$,#94387);
#94371=SHAPE_REPRESENTATION('',(#51188),#94287);
#94385=PRODUCT_DEFINITION_CONTEXT('part definition',#94432,'design');
#94387=PRODUCT_DEFINITION('2026-10-11-08-26-31-288',
'01_Synchro_Sleeve_Torque-Lock_T10-15_WT297-15',#94402,#94385);
#94402=PRODUCT_DEFINITION_FORMATION('',$,#94435);
#94432=APPLICATION_CONTEXT(
'Core Data for Automotive Mechanical Design Process');
#94433=PRODUCT_CONTEXT('part definition',#94432,'mechanical');
#94435=PRODUCT('2026-10-11-08-26-31-288',
'01_Synchro_Sleeve_Torque-Lock_T10-15_WT297-15',$,(#94433));
#94561=COLOUR_RGB('Light Blue',0.38,0.62,0.78);
#94562=FILL_AREA_STYLE_COLOUR('',#94561);
#94563=FILL_AREA_STYLE('',(#94562));
#94564=SURFACE_STYLE_FILL_AREA(#94563);
#94565=SURFACE_SIDE_STYLE('',(#94564));
#94566=SURFACE_STYLE_USAGE(.BOTH.,#94565);
#94567=PRESENTATION_STYLE_ASSIGNMENT((#94566));
ENDSEC;
END-ISO-10303-21;
